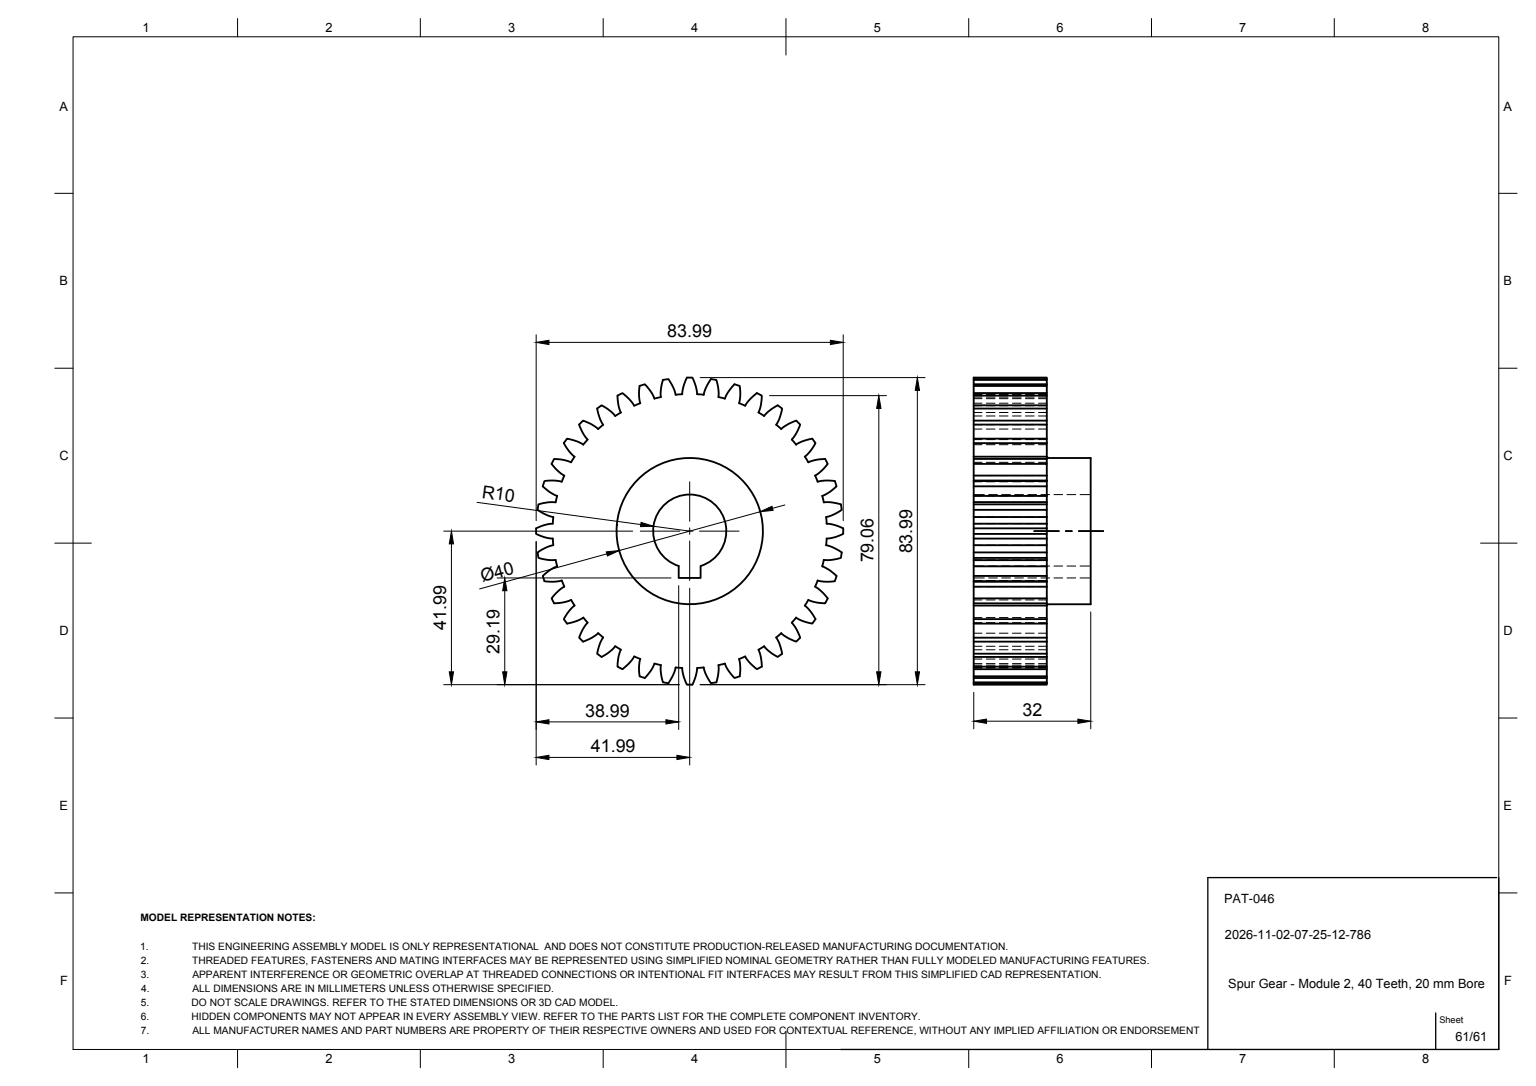
ISO-10303-21;
HEADER;
/* Generated by software containing ST-Developer
 * from STEP Tools, Inc. (www.steptools.com) 
 */

FILE_DESCRIPTION(
/* description */ ('Gear mesh backlash fixture'),
/* implementation_level */ '2;1');

FILE_NAME(
/* name */ 'Spur Gear - Module 2, 40 Teeth, 20 mm Bore.step',
/* time_stamp */ '2026-10-28T03:26:00-07:00',
/* author */ (''),
/* organization */ (''),
/* preprocessor_version */ 'ST-DEVELOPER v20.2',
/* originating_system */ 'Autodesk Translation Framework v15.17.0.0',
/* authorisation */ '');

FILE_SCHEMA (('AUTOMOTIVE_DESIGN { 1 0 10303 214 3 1 1 }'));
ENDSEC;

DATA;
#10=MECHANICAL_DESIGN_GEOMETRIC_PRESENTATION_REPRESENTATION('',(#1079),#57900);
#51=(
BOUNDED_SURFACE()
B_SPLINE_SURFACE(5,1,((#39961,#39962),(#39963,#39964),(#39965,#39966),(#39967,
#39968),(#39969,#39970),(#39971,#39972),(#39973,#39974),(#39975,#39976),
(#39977,#39978),(#39979,#39980),(#39981,#39982),(#39983,#39984),(#39985,
#39986),(#39987,#39988),(#39989,#39990),(#39991,#39992),(#39993,#39994),
(#39995,#39996),(#39997,#39998),(#39999,#40000),(#40001,#40002),(#40003,
#40004),(#40005,#40006),(#40007,#40008),(#40009,#40010),(#40011,#40012),
(#40013,#40014),(#40015,#40016),(#40017,#40018),(#40019,#40020),(#40021,
#40022),(#40023,#40024),(#40025,#40026),(#40027,#40028),(#40029,#40030),
(#40031,#40032),(#40033,#40034),(#40035,#40036),(#40037,#40038),(#40039,
#40040),(#40041,#40042),(#40043,#40044),(#40045,#40046),(#40047,#40048),
(#40049,#40050),(#40051,#40052),(#40053,#40054),(#40055,#40056),(#40057,
#40058),(#40059,#40060),(#40061,#40062),(#40063,#40064),(#40065,#40066),
(#40067,#40068),(#40069,#40070),(#40071,#40072),(#40073,#40074),(#40075,
#40076),(#40077,#40078),(#40079,#40080),(#40081,#40082),(#40083,#40084),
(#40085,#40086),(#40087,#40088),(#40089,#40090),(#40091,#40092),(#40093,
#40094),(#40095,#40096),(#40097,#40098),(#40099,#40100)),.UNSPECIFIED.,
 .F.,.F.,.F.)
B_SPLINE_SURFACE_WITH_KNOTS((6,1,1,1,1,1,1,1,1,1,1,1,1,1,1,1,1,1,1,1,1,
1,1,1,1,1,1,1,1,1,1,1,1,1,1,1,1,1,1,1,1,1,1,1,1,1,1,1,1,1,1,1,1,1,1,1,1,
1,1,1,1,1,1,1,1,6),(2,2),(-1.,-0.984615384615383,-0.969230769230768,-0.953846153846152,
-0.938461538461537,-0.923076923076922,-0.907692307692306,-0.892307692307691,
-0.876923076923076,-0.86153846153846,-0.846153846153845,-0.83076923076923,
-0.815384615384614,-0.799999999999999,-0.784615384615384,-0.769230769230768,
-0.753846153846153,-0.738461538461538,-0.723076923076922,-0.707692307692307,
-0.692307692307692,-0.676923076923076,-0.661538461538461,-0.646153846153846,
-0.63076923076923,-0.615384615384615,-0.6,-0.584615384615384,-0.569230769230769,
-0.553846153846154,-0.538461538461538,-0.523076923076923,-0.507692307692308,
-0.492307692307692,-0.476923076923077,-0.461538461538462,-0.446153846153846,
-0.430769230769231,-0.415384615384615,-0.4,-0.384615384615385,-0.369230769230769,
-0.353846153846154,-0.338461538461538,-0.323076923076923,-0.307692307692308,
-0.292307692307692,-0.276923076923077,-0.261538461538462,-0.246153846153846,
-0.230769230769231,-0.215384615384615,-0.2,-0.184615384615385,-0.169230769230769,
-0.153846153846154,-0.138461538461538,-0.123076923076923,-0.107692307692308,
-0.0923076923076923,-0.0769230769230769,-0.0615384615384615,-0.0461538461538462,
-0.0307692307692308,-0.0153846153846154,0.),(-1.,1.),.UNSPECIFIED.)
GEOMETRIC_REPRESENTATION_ITEM()
RATIONAL_B_SPLINE_SURFACE(((1.,1.),(1.,1.),(1.,1.),(1.,1.),(1.,1.),(1.,
1.),(1.,1.),(1.,1.),(1.,1.),(1.,1.),(1.,1.),(1.,1.),(1.,1.),(1.,1.),(1.,
1.),(1.,1.),(1.,1.),(1.,1.),(1.,1.),(1.,1.),(1.,1.),(1.,1.),(1.,1.),(1.,
1.),(1.,1.),(1.,1.),(1.,1.),(1.,1.),(1.,1.),(1.,1.),(1.,1.),(1.,1.),(1.,
1.),(1.,1.),(1.,1.),(1.,1.),(1.,1.),(1.,1.),(1.,1.),(1.,1.),(1.,1.),(1.,
1.),(1.,1.),(1.,1.),(1.,1.),(1.,1.),(1.,1.),(1.,1.),(1.,1.),(1.,1.),(1.,
1.),(1.,1.),(1.,1.),(1.,1.),(1.,1.),(1.,1.),(1.,1.),(1.,1.),(1.,1.),(1.,
1.),(1.,1.),(1.,1.),(1.,1.),(1.,1.),(1.,1.),(1.,1.),(1.,1.),(1.,1.),(1.,
1.),(1.,1.)))
REPRESENTATION_ITEM('')
SURFACE()
);
#52=(
BOUNDED_SURFACE()
B_SPLINE_SURFACE(5,1,((#40180,#40181),(#40182,#40183),(#40184,#40185),(#40186,
#40187),(#40188,#40189),(#40190,#40191),(#40192,#40193),(#40194,#40195),
(#40196,#40197),(#40198,#40199),(#40200,#40201),(#40202,#40203),(#40204,
#40205),(#40206,#40207),(#40208,#40209),(#40210,#40211),(#40212,#40213),
(#40214,#40215),(#40216,#40217),(#40218,#40219),(#40220,#40221),(#40222,
#40223),(#40224,#40225),(#40226,#40227),(#40228,#40229),(#40230,#40231),
(#40232,#40233),(#40234,#40235),(#40236,#40237),(#40238,#40239),(#40240,
#40241),(#40242,#40243),(#40244,#40245),(#40246,#40247),(#40248,#40249),
(#40250,#40251),(#40252,#40253),(#40254,#40255),(#40256,#40257),(#40258,
#40259),(#40260,#40261),(#40262,#40263),(#40264,#40265),(#40266,#40267),
(#40268,#40269),(#40270,#40271),(#40272,#40273),(#40274,#40275),(#40276,
#40277),(#40278,#40279),(#40280,#40281),(#40282,#40283),(#40284,#40285),
(#40286,#40287),(#40288,#40289),(#40290,#40291),(#40292,#40293),(#40294,
#40295),(#40296,#40297),(#40298,#40299),(#40300,#40301),(#40302,#40303),
(#40304,#40305),(#40306,#40307),(#40308,#40309),(#40310,#40311),(#40312,
#40313),(#40314,#40315),(#40316,#40317),(#40318,#40319)),.UNSPECIFIED.,
 .F.,.F.,.F.)
B_SPLINE_SURFACE_WITH_KNOTS((6,1,1,1,1,1,1,1,1,1,1,1,1,1,1,1,1,1,1,1,1,
1,1,1,1,1,1,1,1,1,1,1,1,1,1,1,1,1,1,1,1,1,1,1,1,1,1,1,1,1,1,1,1,1,1,1,1,
1,1,1,1,1,1,1,1,6),(2,2),(-1.,-0.984615384615383,-0.969230769230768,-0.953846153846152,
-0.938461538461537,-0.923076923076922,-0.907692307692306,-0.892307692307691,
-0.876923076923076,-0.86153846153846,-0.846153846153845,-0.83076923076923,
-0.815384615384614,-0.799999999999999,-0.784615384615384,-0.769230769230768,
-0.753846153846153,-0.738461538461538,-0.723076923076922,-0.707692307692307,
-0.692307692307692,-0.676923076923076,-0.661538461538461,-0.646153846153846,
-0.63076923076923,-0.615384615384615,-0.6,-0.584615384615384,-0.569230769230769,
-0.553846153846154,-0.538461538461538,-0.523076923076923,-0.507692307692308,
-0.492307692307692,-0.476923076923077,-0.461538461538462,-0.446153846153846,
-0.430769230769231,-0.415384615384615,-0.4,-0.384615384615385,-0.369230769230769,
-0.353846153846154,-0.338461538461538,-0.323076923076923,-0.307692307692308,
-0.292307692307692,-0.276923076923077,-0.261538461538462,-0.246153846153846,
-0.230769230769231,-0.215384615384615,-0.2,-0.184615384615385,-0.169230769230769,
-0.153846153846154,-0.138461538461538,-0.123076923076923,-0.107692307692308,
-0.0923076923076923,-0.0769230769230769,-0.0615384615384615,-0.0461538461538462,
-0.0307692307692308,-0.0153846153846154,0.),(-1.,1.),.UNSPECIFIED.)
GEOMETRIC_REPRESENTATION_ITEM()
RATIONAL_B_SPLINE_SURFACE(((1.,1.),(1.,1.),(1.,1.),(1.,1.),(1.,1.),(1.,
1.),(1.,1.),(1.,1.),(1.,1.),(1.,1.),(1.,1.),(1.,1.),(1.,1.),(1.,1.),(1.,
1.),(1.,1.),(1.,1.),(1.,1.),(1.,1.),(1.,1.),(1.,1.),(1.,1.),(1.,1.),(1.,
1.),(1.,1.),(1.,1.),(1.,1.),(1.,1.),(1.,1.),(1.,1.),(1.,1.),(1.,1.),(1.,
1.),(1.,1.),(1.,1.),(1.,1.),(1.,1.),(1.,1.),(1.,1.),(1.,1.),(1.,1.),(1.,
1.),(1.,1.),(1.,1.),(1.,1.),(1.,1.),(1.,1.),(1.,1.),(1.,1.),(1.,1.),(1.,
1.),(1.,1.),(1.,1.),(1.,1.),(1.,1.),(1.,1.),(1.,1.),(1.,1.),(1.,1.),(1.,
1.),(1.,1.),(1.,1.),(1.,1.),(1.,1.),(1.,1.),(1.,1.),(1.,1.),(1.,1.),(1.,
1.),(1.,1.)))
REPRESENTATION_ITEM('')
SURFACE()
);
#53=(
BOUNDED_SURFACE()
B_SPLINE_SURFACE(5,1,((#40410,#40411),(#40412,#40413),(#40414,#40415),(#40416,
#40417),(#40418,#40419),(#40420,#40421),(#40422,#40423),(#40424,#40425),
(#40426,#40427),(#40428,#40429),(#40430,#40431),(#40432,#40433),(#40434,
#40435),(#40436,#40437),(#40438,#40439),(#40440,#40441),(#40442,#40443),
(#40444,#40445),(#40446,#40447),(#40448,#40449),(#40450,#40451),(#40452,
#40453),(#40454,#40455),(#40456,#40457),(#40458,#40459),(#40460,#40461),
(#40462,#40463),(#40464,#40465),(#40466,#40467),(#40468,#40469),(#40470,
#40471),(#40472,#40473),(#40474,#40475),(#40476,#40477),(#40478,#40479),
(#40480,#40481),(#40482,#40483),(#40484,#40485),(#40486,#40487),(#40488,
#40489),(#40490,#40491),(#40492,#40493),(#40494,#40495),(#40496,#40497),
(#40498,#40499),(#40500,#40501),(#40502,#40503),(#40504,#40505),(#40506,
#40507),(#40508,#40509),(#40510,#40511),(#40512,#40513),(#40514,#40515),
(#40516,#40517),(#40518,#40519),(#40520,#40521),(#40522,#40523),(#40524,
#40525),(#40526,#40527),(#40528,#40529),(#40530,#40531),(#40532,#40533),
(#40534,#40535),(#40536,#40537),(#40538,#40539),(#40540,#40541),(#40542,
#40543),(#40544,#40545),(#40546,#40547),(#40548,#40549)),.UNSPECIFIED.,
 .F.,.F.,.F.)
B_SPLINE_SURFACE_WITH_KNOTS((6,1,1,1,1,1,1,1,1,1,1,1,1,1,1,1,1,1,1,1,1,
1,1,1,1,1,1,1,1,1,1,1,1,1,1,1,1,1,1,1,1,1,1,1,1,1,1,1,1,1,1,1,1,1,1,1,1,
1,1,1,1,1,1,1,1,6),(2,2),(-1.,-0.984615384615383,-0.969230769230768,-0.953846153846152,
-0.938461538461537,-0.923076923076922,-0.907692307692306,-0.892307692307691,
-0.876923076923076,-0.86153846153846,-0.846153846153845,-0.83076923076923,
-0.815384615384614,-0.799999999999999,-0.784615384615384,-0.769230769230768,
-0.753846153846153,-0.738461538461538,-0.723076923076922,-0.707692307692307,
-0.692307692307692,-0.676923076923076,-0.661538461538461,-0.646153846153846,
-0.63076923076923,-0.615384615384615,-0.6,-0.584615384615384,-0.569230769230769,
-0.553846153846154,-0.538461538461538,-0.523076923076923,-0.507692307692308,
-0.492307692307692,-0.476923076923077,-0.461538461538462,-0.446153846153846,
-0.430769230769231,-0.415384615384615,-0.4,-0.384615384615385,-0.369230769230769,
-0.353846153846154,-0.338461538461538,-0.323076923076923,-0.307692307692308,
-0.292307692307692,-0.276923076923077,-0.261538461538462,-0.246153846153846,
-0.230769230769231,-0.215384615384615,-0.2,-0.184615384615385,-0.169230769230769,
-0.153846153846154,-0.138461538461538,-0.123076923076923,-0.107692307692308,
-0.0923076923076923,-0.0769230769230769,-0.0615384615384615,-0.0461538461538462,
-0.0307692307692308,-0.0153846153846154,0.),(-1.,1.),.UNSPECIFIED.)
GEOMETRIC_REPRESENTATION_ITEM()
RATIONAL_B_SPLINE_SURFACE(((1.,1.),(1.,1.),(1.,1.),(1.,1.),(1.,1.),(1.,
1.),(1.,1.),(1.,1.),(1.,1.),(1.,1.),(1.,1.),(1.,1.),(1.,1.),(1.,1.),(1.,
1.),(1.,1.),(1.,1.),(1.,1.),(1.,1.),(1.,1.),(1.,1.),(1.,1.),(1.,1.),(1.,
1.),(1.,1.),(1.,1.),(1.,1.),(1.,1.),(1.,1.),(1.,1.),(1.,1.),(1.,1.),(1.,
1.),(1.,1.),(1.,1.),(1.,1.),(1.,1.),(1.,1.),(1.,1.),(1.,1.),(1.,1.),(1.,
1.),(1.,1.),(1.,1.),(1.,1.),(1.,1.),(1.,1.),(1.,1.),(1.,1.),(1.,1.),(1.,
1.),(1.,1.),(1.,1.),(1.,1.),(1.,1.),(1.,1.),(1.,1.),(1.,1.),(1.,1.),(1.,
1.),(1.,1.),(1.,1.),(1.,1.),(1.,1.),(1.,1.),(1.,1.),(1.,1.),(1.,1.),(1.,
1.),(1.,1.)))
REPRESENTATION_ITEM('')
SURFACE()
);
#54=(
BOUNDED_SURFACE()
B_SPLINE_SURFACE(5,1,((#40622,#40623),(#40624,#40625),(#40626,#40627),(#40628,
#40629),(#40630,#40631),(#40632,#40633),(#40634,#40635),(#40636,#40637),
(#40638,#40639),(#40640,#40641),(#40642,#40643),(#40644,#40645),(#40646,
#40647),(#40648,#40649),(#40650,#40651),(#40652,#40653),(#40654,#40655),
(#40656,#40657),(#40658,#40659),(#40660,#40661),(#40662,#40663),(#40664,
#40665),(#40666,#40667),(#40668,#40669),(#40670,#40671),(#40672,#40673),
(#40674,#40675),(#40676,#40677),(#40678,#40679),(#40680,#40681),(#40682,
#40683),(#40684,#40685),(#40686,#40687),(#40688,#40689),(#40690,#40691),
(#40692,#40693),(#40694,#40695),(#40696,#40697),(#40698,#40699),(#40700,
#40701),(#40702,#40703),(#40704,#40705),(#40706,#40707),(#40708,#40709),
(#40710,#40711),(#40712,#40713),(#40714,#40715),(#40716,#40717),(#40718,
#40719),(#40720,#40721),(#40722,#40723),(#40724,#40725),(#40726,#40727),
(#40728,#40729),(#40730,#40731),(#40732,#40733),(#40734,#40735),(#40736,
#40737),(#40738,#40739),(#40740,#40741),(#40742,#40743),(#40744,#40745),
(#40746,#40747),(#40748,#40749),(#40750,#40751),(#40752,#40753),(#40754,
#40755),(#40756,#40757),(#40758,#40759),(#40760,#40761)),.UNSPECIFIED.,
 .F.,.F.,.F.)
B_SPLINE_SURFACE_WITH_KNOTS((6,1,1,1,1,1,1,1,1,1,1,1,1,1,1,1,1,1,1,1,1,
1,1,1,1,1,1,1,1,1,1,1,1,1,1,1,1,1,1,1,1,1,1,1,1,1,1,1,1,1,1,1,1,1,1,1,1,
1,1,1,1,1,1,1,1,6),(2,2),(-1.,-0.984615384615383,-0.969230769230768,-0.953846153846152,
-0.938461538461537,-0.923076923076922,-0.907692307692306,-0.892307692307691,
-0.876923076923076,-0.86153846153846,-0.846153846153845,-0.83076923076923,
-0.815384615384614,-0.799999999999999,-0.784615384615384,-0.769230769230768,
-0.753846153846153,-0.738461538461538,-0.723076923076922,-0.707692307692307,
-0.692307692307692,-0.676923076923076,-0.661538461538461,-0.646153846153846,
-0.63076923076923,-0.615384615384615,-0.6,-0.584615384615384,-0.569230769230769,
-0.553846153846154,-0.538461538461538,-0.523076923076923,-0.507692307692308,
-0.492307692307692,-0.476923076923077,-0.461538461538462,-0.446153846153846,
-0.430769230769231,-0.415384615384615,-0.4,-0.384615384615385,-0.369230769230769,
-0.353846153846154,-0.338461538461538,-0.323076923076923,-0.307692307692308,
-0.292307692307692,-0.276923076923077,-0.261538461538462,-0.246153846153846,
-0.230769230769231,-0.215384615384615,-0.2,-0.184615384615385,-0.169230769230769,
-0.153846153846154,-0.138461538461538,-0.123076923076923,-0.107692307692308,
-0.0923076923076923,-0.0769230769230769,-0.0615384615384615,-0.0461538461538462,
-0.0307692307692308,-0.0153846153846154,0.),(-1.,1.),.UNSPECIFIED.)
GEOMETRIC_REPRESENTATION_ITEM()
RATIONAL_B_SPLINE_SURFACE(((1.,1.),(1.,1.),(1.,1.),(1.,1.),(1.,1.),(1.,
1.),(1.,1.),(1.,1.),(1.,1.),(1.,1.),(1.,1.),(1.,1.),(1.,1.),(1.,1.),(1.,
1.),(1.,1.),(1.,1.),(1.,1.),(1.,1.),(1.,1.),(1.,1.),(1.,1.),(1.,1.),(1.,
1.),(1.,1.),(1.,1.),(1.,1.),(1.,1.),(1.,1.),(1.,1.),(1.,1.),(1.,1.),(1.,
1.),(1.,1.),(1.,1.),(1.,1.),(1.,1.),(1.,1.),(1.,1.),(1.,1.),(1.,1.),(1.,
1.),(1.,1.),(1.,1.),(1.,1.),(1.,1.),(1.,1.),(1.,1.),(1.,1.),(1.,1.),(1.,
1.),(1.,1.),(1.,1.),(1.,1.),(1.,1.),(1.,1.),(1.,1.),(1.,1.),(1.,1.),(1.,
1.),(1.,1.),(1.,1.),(1.,1.),(1.,1.),(1.,1.),(1.,1.),(1.,1.),(1.,1.),(1.,
1.),(1.,1.)))
REPRESENTATION_ITEM('')
SURFACE()
);
#55=(
BOUNDED_SURFACE()
B_SPLINE_SURFACE(5,1,((#40852,#40853),(#40854,#40855),(#40856,#40857),(#40858,
#40859),(#40860,#40861),(#40862,#40863),(#40864,#40865),(#40866,#40867),
(#40868,#40869),(#40870,#40871),(#40872,#40873),(#40874,#40875),(#40876,
#40877),(#40878,#40879),(#40880,#40881),(#40882,#40883),(#40884,#40885),
(#40886,#40887),(#40888,#40889),(#40890,#40891),(#40892,#40893),(#40894,
#40895),(#40896,#40897),(#40898,#40899),(#40900,#40901),(#40902,#40903),
(#40904,#40905),(#40906,#40907),(#40908,#40909),(#40910,#40911),(#40912,
#40913),(#40914,#40915),(#40916,#40917),(#40918,#40919),(#40920,#40921),
(#40922,#40923),(#40924,#40925),(#40926,#40927),(#40928,#40929),(#40930,
#40931),(#40932,#40933),(#40934,#40935),(#40936,#40937),(#40938,#40939),
(#40940,#40941),(#40942,#40943),(#40944,#40945),(#40946,#40947),(#40948,
#40949),(#40950,#40951),(#40952,#40953),(#40954,#40955),(#40956,#40957),
(#40958,#40959),(#40960,#40961),(#40962,#40963),(#40964,#40965),(#40966,
#40967),(#40968,#40969),(#40970,#40971),(#40972,#40973),(#40974,#40975),
(#40976,#40977),(#40978,#40979),(#40980,#40981),(#40982,#40983),(#40984,
#40985),(#40986,#40987),(#40988,#40989),(#40990,#40991)),.UNSPECIFIED.,
 .F.,.F.,.F.)
B_SPLINE_SURFACE_WITH_KNOTS((6,1,1,1,1,1,1,1,1,1,1,1,1,1,1,1,1,1,1,1,1,
1,1,1,1,1,1,1,1,1,1,1,1,1,1,1,1,1,1,1,1,1,1,1,1,1,1,1,1,1,1,1,1,1,1,1,1,
1,1,1,1,1,1,1,1,6),(2,2),(-1.,-0.984615384615383,-0.969230769230768,-0.953846153846152,
-0.938461538461537,-0.923076923076922,-0.907692307692306,-0.892307692307691,
-0.876923076923076,-0.86153846153846,-0.846153846153845,-0.83076923076923,
-0.815384615384614,-0.799999999999999,-0.784615384615384,-0.769230769230768,
-0.753846153846153,-0.738461538461538,-0.723076923076922,-0.707692307692307,
-0.692307692307692,-0.676923076923076,-0.661538461538461,-0.646153846153846,
-0.63076923076923,-0.615384615384615,-0.6,-0.584615384615384,-0.569230769230769,
-0.553846153846154,-0.538461538461538,-0.523076923076923,-0.507692307692308,
-0.492307692307692,-0.476923076923077,-0.461538461538462,-0.446153846153846,
-0.430769230769231,-0.415384615384615,-0.4,-0.384615384615385,-0.369230769230769,
-0.353846153846154,-0.338461538461538,-0.323076923076923,-0.307692307692308,
-0.292307692307692,-0.276923076923077,-0.261538461538462,-0.246153846153846,
-0.230769230769231,-0.215384615384615,-0.2,-0.184615384615385,-0.169230769230769,
-0.153846153846154,-0.138461538461538,-0.123076923076923,-0.107692307692308,
-0.0923076923076923,-0.0769230769230769,-0.0615384615384615,-0.0461538461538462,
-0.0307692307692308,-0.0153846153846154,0.),(-1.,1.),.UNSPECIFIED.)
GEOMETRIC_REPRESENTATION_ITEM()
RATIONAL_B_SPLINE_SURFACE(((1.,1.),(1.,1.),(1.,1.),(1.,1.),(1.,1.),(1.,
1.),(1.,1.),(1.,1.),(1.,1.),(1.,1.),(1.,1.),(1.,1.),(1.,1.),(1.,1.),(1.,
1.),(1.,1.),(1.,1.),(1.,1.),(1.,1.),(1.,1.),(1.,1.),(1.,1.),(1.,1.),(1.,
1.),(1.,1.),(1.,1.),(1.,1.),(1.,1.),(1.,1.),(1.,1.),(1.,1.),(1.,1.),(1.,
1.),(1.,1.),(1.,1.),(1.,1.),(1.,1.),(1.,1.),(1.,1.),(1.,1.),(1.,1.),(1.,
1.),(1.,1.),(1.,1.),(1.,1.),(1.,1.),(1.,1.),(1.,1.),(1.,1.),(1.,1.),(1.,
1.),(1.,1.),(1.,1.),(1.,1.),(1.,1.),(1.,1.),(1.,1.),(1.,1.),(1.,1.),(1.,
1.),(1.,1.),(1.,1.),(1.,1.),(1.,1.),(1.,1.),(1.,1.),(1.,1.),(1.,1.),(1.,
1.),(1.,1.)))
REPRESENTATION_ITEM('')
SURFACE()
);
#56=(
BOUNDED_SURFACE()
B_SPLINE_SURFACE(5,1,((#41064,#41065),(#41066,#41067),(#41068,#41069),(#41070,
#41071),(#41072,#41073),(#41074,#41075),(#41076,#41077),(#41078,#41079),
(#41080,#41081),(#41082,#41083),(#41084,#41085),(#41086,#41087),(#41088,
#41089),(#41090,#41091),(#41092,#41093),(#41094,#41095),(#41096,#41097),
(#41098,#41099),(#41100,#41101),(#41102,#41103),(#41104,#41105),(#41106,
#41107),(#41108,#41109),(#41110,#41111),(#41112,#41113),(#41114,#41115),
(#41116,#41117),(#41118,#41119),(#41120,#41121),(#41122,#41123),(#41124,
#41125),(#41126,#41127),(#41128,#41129),(#41130,#41131),(#41132,#41133),
(#41134,#41135),(#41136,#41137),(#41138,#41139),(#41140,#41141),(#41142,
#41143),(#41144,#41145),(#41146,#41147),(#41148,#41149),(#41150,#41151),
(#41152,#41153),(#41154,#41155),(#41156,#41157),(#41158,#41159),(#41160,
#41161),(#41162,#41163),(#41164,#41165),(#41166,#41167),(#41168,#41169),
(#41170,#41171),(#41172,#41173),(#41174,#41175),(#41176,#41177),(#41178,
#41179),(#41180,#41181),(#41182,#41183),(#41184,#41185),(#41186,#41187),
(#41188,#41189),(#41190,#41191),(#41192,#41193),(#41194,#41195),(#41196,
#41197),(#41198,#41199),(#41200,#41201),(#41202,#41203)),.UNSPECIFIED.,
 .F.,.F.,.F.)
B_SPLINE_SURFACE_WITH_KNOTS((6,1,1,1,1,1,1,1,1,1,1,1,1,1,1,1,1,1,1,1,1,
1,1,1,1,1,1,1,1,1,1,1,1,1,1,1,1,1,1,1,1,1,1,1,1,1,1,1,1,1,1,1,1,1,1,1,1,
1,1,1,1,1,1,1,1,6),(2,2),(-1.,-0.984615384615383,-0.969230769230768,-0.953846153846152,
-0.938461538461537,-0.923076923076922,-0.907692307692306,-0.892307692307691,
-0.876923076923076,-0.86153846153846,-0.846153846153845,-0.83076923076923,
-0.815384615384614,-0.799999999999999,-0.784615384615384,-0.769230769230768,
-0.753846153846153,-0.738461538461538,-0.723076923076922,-0.707692307692307,
-0.692307692307692,-0.676923076923076,-0.661538461538461,-0.646153846153846,
-0.63076923076923,-0.615384615384615,-0.6,-0.584615384615384,-0.569230769230769,
-0.553846153846154,-0.538461538461538,-0.523076923076923,-0.507692307692308,
-0.492307692307692,-0.476923076923077,-0.461538461538462,-0.446153846153846,
-0.430769230769231,-0.415384615384615,-0.4,-0.384615384615385,-0.369230769230769,
-0.353846153846154,-0.338461538461538,-0.323076923076923,-0.307692307692308,
-0.292307692307692,-0.276923076923077,-0.261538461538462,-0.246153846153846,
-0.230769230769231,-0.215384615384615,-0.2,-0.184615384615385,-0.169230769230769,
-0.153846153846154,-0.138461538461538,-0.123076923076923,-0.107692307692308,
-0.0923076923076923,-0.0769230769230769,-0.0615384615384615,-0.0461538461538462,
-0.0307692307692308,-0.0153846153846154,0.),(-1.,1.),.UNSPECIFIED.)
GEOMETRIC_REPRESENTATION_ITEM()
RATIONAL_B_SPLINE_SURFACE(((1.,1.),(1.,1.),(1.,1.),(1.,1.),(1.,1.),(1.,
1.),(1.,1.),(1.,1.),(1.,1.),(1.,1.),(1.,1.),(1.,1.),(1.,1.),(1.,1.),(1.,
1.),(1.,1.),(1.,1.),(1.,1.),(1.,1.),(1.,1.),(1.,1.),(1.,1.),(1.,1.),(1.,
1.),(1.,1.),(1.,1.),(1.,1.),(1.,1.),(1.,1.),(1.,1.),(1.,1.),(1.,1.),(1.,
1.),(1.,1.),(1.,1.),(1.,1.),(1.,1.),(1.,1.),(1.,1.),(1.,1.),(1.,1.),(1.,
1.),(1.,1.),(1.,1.),(1.,1.),(1.,1.),(1.,1.),(1.,1.),(1.,1.),(1.,1.),(1.,
1.),(1.,1.),(1.,1.),(1.,1.),(1.,1.),(1.,1.),(1.,1.),(1.,1.),(1.,1.),(1.,
1.),(1.,1.),(1.,1.),(1.,1.),(1.,1.),(1.,1.),(1.,1.),(1.,1.),(1.,1.),(1.,
1.),(1.,1.)))
REPRESENTATION_ITEM('')
SURFACE()
);
#57=(
BOUNDED_SURFACE()
B_SPLINE_SURFACE(5,1,((#41294,#41295),(#41296,#41297),(#41298,#41299),(#41300,
#41301),(#41302,#41303),(#41304,#41305),(#41306,#41307),(#41308,#41309),
(#41310,#41311),(#41312,#41313),(#41314,#41315),(#41316,#41317),(#41318,
#41319),(#41320,#41321),(#41322,#41323),(#41324,#41325),(#41326,#41327),
(#41328,#41329),(#41330,#41331),(#41332,#41333),(#41334,#41335),(#41336,
#41337),(#41338,#41339),(#41340,#41341),(#41342,#41343),(#41344,#41345),
(#41346,#41347),(#41348,#41349),(#41350,#41351),(#41352,#41353),(#41354,
#41355),(#41356,#41357),(#41358,#41359),(#41360,#41361),(#41362,#41363),
(#41364,#41365),(#41366,#41367),(#41368,#41369),(#41370,#41371),(#41372,
#41373),(#41374,#41375),(#41376,#41377),(#41378,#41379),(#41380,#41381),
(#41382,#41383),(#41384,#41385),(#41386,#41387),(#41388,#41389),(#41390,
#41391),(#41392,#41393),(#41394,#41395),(#41396,#41397),(#41398,#41399),
(#41400,#41401),(#41402,#41403),(#41404,#41405),(#41406,#41407),(#41408,
#41409),(#41410,#41411),(#41412,#41413),(#41414,#41415),(#41416,#41417),
(#41418,#41419),(#41420,#41421),(#41422,#41423),(#41424,#41425),(#41426,
#41427),(#41428,#41429),(#41430,#41431),(#41432,#41433)),.UNSPECIFIED.,
 .F.,.F.,.F.)
B_SPLINE_SURFACE_WITH_KNOTS((6,1,1,1,1,1,1,1,1,1,1,1,1,1,1,1,1,1,1,1,1,
1,1,1,1,1,1,1,1,1,1,1,1,1,1,1,1,1,1,1,1,1,1,1,1,1,1,1,1,1,1,1,1,1,1,1,1,
1,1,1,1,1,1,1,1,6),(2,2),(-1.,-0.984615384615383,-0.969230769230768,-0.953846153846152,
-0.938461538461537,-0.923076923076922,-0.907692307692306,-0.892307692307691,
-0.876923076923076,-0.86153846153846,-0.846153846153845,-0.83076923076923,
-0.815384615384614,-0.799999999999999,-0.784615384615384,-0.769230769230768,
-0.753846153846153,-0.738461538461538,-0.723076923076922,-0.707692307692307,
-0.692307692307692,-0.676923076923076,-0.661538461538461,-0.646153846153846,
-0.63076923076923,-0.615384615384615,-0.6,-0.584615384615384,-0.569230769230769,
-0.553846153846154,-0.538461538461538,-0.523076923076923,-0.507692307692308,
-0.492307692307692,-0.476923076923077,-0.461538461538462,-0.446153846153846,
-0.430769230769231,-0.415384615384615,-0.4,-0.384615384615385,-0.369230769230769,
-0.353846153846154,-0.338461538461538,-0.323076923076923,-0.307692307692308,
-0.292307692307692,-0.276923076923077,-0.261538461538462,-0.246153846153846,
-0.230769230769231,-0.215384615384615,-0.2,-0.184615384615385,-0.169230769230769,
-0.153846153846154,-0.138461538461538,-0.123076923076923,-0.107692307692308,
-0.0923076923076923,-0.0769230769230769,-0.0615384615384615,-0.0461538461538462,
-0.0307692307692308,-0.0153846153846154,0.),(-1.,1.),.UNSPECIFIED.)
GEOMETRIC_REPRESENTATION_ITEM()
RATIONAL_B_SPLINE_SURFACE(((1.,1.),(1.,1.),(1.,1.),(1.,1.),(1.,1.),(1.,
1.),(1.,1.),(1.,1.),(1.,1.),(1.,1.),(1.,1.),(1.,1.),(1.,1.),(1.,1.),(1.,
1.),(1.,1.),(1.,1.),(1.,1.),(1.,1.),(1.,1.),(1.,1.),(1.,1.),(1.,1.),(1.,
1.),(1.,1.),(1.,1.),(1.,1.),(1.,1.),(1.,1.),(1.,1.),(1.,1.),(1.,1.),(1.,
1.),(1.,1.),(1.,1.),(1.,1.),(1.,1.),(1.,1.),(1.,1.),(1.,1.),(1.,1.),(1.,
1.),(1.,1.),(1.,1.),(1.,1.),(1.,1.),(1.,1.),(1.,1.),(1.,1.),(1.,1.),(1.,
1.),(1.,1.),(1.,1.),(1.,1.),(1.,1.),(1.,1.),(1.,1.),(1.,1.),(1.,1.),(1.,
1.),(1.,1.),(1.,1.),(1.,1.),(1.,1.),(1.,1.),(1.,1.),(1.,1.),(1.,1.),(1.,
1.),(1.,1.)))
REPRESENTATION_ITEM('')
SURFACE()
);
#58=(
BOUNDED_SURFACE()
B_SPLINE_SURFACE(5,1,((#41506,#41507),(#41508,#41509),(#41510,#41511),(#41512,
#41513),(#41514,#41515),(#41516,#41517),(#41518,#41519),(#41520,#41521),
(#41522,#41523),(#41524,#41525),(#41526,#41527),(#41528,#41529),(#41530,
#41531),(#41532,#41533),(#41534,#41535),(#41536,#41537),(#41538,#41539),
(#41540,#41541),(#41542,#41543),(#41544,#41545),(#41546,#41547),(#41548,
#41549),(#41550,#41551),(#41552,#41553),(#41554,#41555),(#41556,#41557),
(#41558,#41559),(#41560,#41561),(#41562,#41563),(#41564,#41565),(#41566,
#41567),(#41568,#41569),(#41570,#41571),(#41572,#41573),(#41574,#41575),
(#41576,#41577),(#41578,#41579),(#41580,#41581),(#41582,#41583),(#41584,
#41585),(#41586,#41587),(#41588,#41589),(#41590,#41591),(#41592,#41593),
(#41594,#41595),(#41596,#41597),(#41598,#41599),(#41600,#41601),(#41602,
#41603),(#41604,#41605),(#41606,#41607),(#41608,#41609),(#41610,#41611),
(#41612,#41613),(#41614,#41615),(#41616,#41617),(#41618,#41619),(#41620,
#41621),(#41622,#41623),(#41624,#41625),(#41626,#41627),(#41628,#41629),
(#41630,#41631),(#41632,#41633),(#41634,#41635),(#41636,#41637),(#41638,
#41639),(#41640,#41641),(#41642,#41643),(#41644,#41645)),.UNSPECIFIED.,
 .F.,.F.,.F.)
B_SPLINE_SURFACE_WITH_KNOTS((6,1,1,1,1,1,1,1,1,1,1,1,1,1,1,1,1,1,1,1,1,
1,1,1,1,1,1,1,1,1,1,1,1,1,1,1,1,1,1,1,1,1,1,1,1,1,1,1,1,1,1,1,1,1,1,1,1,
1,1,1,1,1,1,1,1,6),(2,2),(-1.,-0.984615384615383,-0.969230769230768,-0.953846153846152,
-0.938461538461537,-0.923076923076922,-0.907692307692306,-0.892307692307691,
-0.876923076923076,-0.86153846153846,-0.846153846153845,-0.83076923076923,
-0.815384615384614,-0.799999999999999,-0.784615384615384,-0.769230769230768,
-0.753846153846153,-0.738461538461538,-0.723076923076922,-0.707692307692307,
-0.692307692307692,-0.676923076923076,-0.661538461538461,-0.646153846153846,
-0.63076923076923,-0.615384615384615,-0.6,-0.584615384615384,-0.569230769230769,
-0.553846153846154,-0.538461538461538,-0.523076923076923,-0.507692307692308,
-0.492307692307692,-0.476923076923077,-0.461538461538462,-0.446153846153846,
-0.430769230769231,-0.415384615384615,-0.4,-0.384615384615385,-0.369230769230769,
-0.353846153846154,-0.338461538461538,-0.323076923076923,-0.307692307692308,
-0.292307692307692,-0.276923076923077,-0.261538461538462,-0.246153846153846,
-0.230769230769231,-0.215384615384615,-0.2,-0.184615384615385,-0.169230769230769,
-0.153846153846154,-0.138461538461538,-0.123076923076923,-0.107692307692308,
-0.0923076923076923,-0.0769230769230769,-0.0615384615384615,-0.0461538461538462,
-0.0307692307692308,-0.0153846153846154,0.),(-1.,1.),.UNSPECIFIED.)
GEOMETRIC_REPRESENTATION_ITEM()
RATIONAL_B_SPLINE_SURFACE(((1.,1.),(1.,1.),(1.,1.),(1.,1.),(1.,1.),(1.,
1.),(1.,1.),(1.,1.),(1.,1.),(1.,1.),(1.,1.),(1.,1.),(1.,1.),(1.,1.),(1.,
1.),(1.,1.),(1.,1.),(1.,1.),(1.,1.),(1.,1.),(1.,1.),(1.,1.),(1.,1.),(1.,
1.),(1.,1.),(1.,1.),(1.,1.),(1.,1.),(1.,1.),(1.,1.),(1.,1.),(1.,1.),(1.,
1.),(1.,1.),(1.,1.),(1.,1.),(1.,1.),(1.,1.),(1.,1.),(1.,1.),(1.,1.),(1.,
1.),(1.,1.),(1.,1.),(1.,1.),(1.,1.),(1.,1.),(1.,1.),(1.,1.),(1.,1.),(1.,
1.),(1.,1.),(1.,1.),(1.,1.),(1.,1.),(1.,1.),(1.,1.),(1.,1.),(1.,1.),(1.,
1.),(1.,1.),(1.,1.),(1.,1.),(1.,1.),(1.,1.),(1.,1.),(1.,1.),(1.,1.),(1.,
1.),(1.,1.)))
REPRESENTATION_ITEM('')
SURFACE()
);
#59=(
BOUNDED_SURFACE()
B_SPLINE_SURFACE(5,1,((#41736,#41737),(#41738,#41739),(#41740,#41741),(#41742,
#41743),(#41744,#41745),(#41746,#41747),(#41748,#41749),(#41750,#41751),
(#41752,#41753),(#41754,#41755),(#41756,#41757),(#41758,#41759),(#41760,
#41761),(#41762,#41763),(#41764,#41765),(#41766,#41767),(#41768,#41769),
(#41770,#41771),(#41772,#41773),(#41774,#41775),(#41776,#41777),(#41778,
#41779),(#41780,#41781),(#41782,#41783),(#41784,#41785),(#41786,#41787),
(#41788,#41789),(#41790,#41791),(#41792,#41793),(#41794,#41795),(#41796,
#41797),(#41798,#41799),(#41800,#41801),(#41802,#41803),(#41804,#41805),
(#41806,#41807),(#41808,#41809),(#41810,#41811),(#41812,#41813),(#41814,
#41815),(#41816,#41817),(#41818,#41819),(#41820,#41821),(#41822,#41823),
(#41824,#41825),(#41826,#41827),(#41828,#41829),(#41830,#41831),(#41832,
#41833),(#41834,#41835),(#41836,#41837),(#41838,#41839),(#41840,#41841),
(#41842,#41843),(#41844,#41845),(#41846,#41847),(#41848,#41849),(#41850,
#41851),(#41852,#41853),(#41854,#41855),(#41856,#41857),(#41858,#41859),
(#41860,#41861),(#41862,#41863),(#41864,#41865),(#41866,#41867),(#41868,
#41869),(#41870,#41871),(#41872,#41873),(#41874,#41875)),.UNSPECIFIED.,
 .F.,.F.,.F.)
B_SPLINE_SURFACE_WITH_KNOTS((6,1,1,1,1,1,1,1,1,1,1,1,1,1,1,1,1,1,1,1,1,
1,1,1,1,1,1,1,1,1,1,1,1,1,1,1,1,1,1,1,1,1,1,1,1,1,1,1,1,1,1,1,1,1,1,1,1,
1,1,1,1,1,1,1,1,6),(2,2),(-1.,-0.984615384615383,-0.969230769230768,-0.953846153846152,
-0.938461538461537,-0.923076923076922,-0.907692307692306,-0.892307692307691,
-0.876923076923076,-0.86153846153846,-0.846153846153845,-0.83076923076923,
-0.815384615384614,-0.799999999999999,-0.784615384615384,-0.769230769230768,
-0.753846153846153,-0.738461538461538,-0.723076923076922,-0.707692307692307,
-0.692307692307692,-0.676923076923076,-0.661538461538461,-0.646153846153846,
-0.63076923076923,-0.615384615384615,-0.6,-0.584615384615384,-0.569230769230769,
-0.553846153846154,-0.538461538461538,-0.523076923076923,-0.507692307692308,
-0.492307692307692,-0.476923076923077,-0.461538461538462,-0.446153846153846,
-0.430769230769231,-0.415384615384615,-0.4,-0.384615384615385,-0.369230769230769,
-0.353846153846154,-0.338461538461538,-0.323076923076923,-0.307692307692308,
-0.292307692307692,-0.276923076923077,-0.261538461538462,-0.246153846153846,
-0.230769230769231,-0.215384615384615,-0.2,-0.184615384615385,-0.169230769230769,
-0.153846153846154,-0.138461538461538,-0.123076923076923,-0.107692307692308,
-0.0923076923076923,-0.0769230769230769,-0.0615384615384615,-0.0461538461538462,
-0.0307692307692308,-0.0153846153846154,0.),(-1.,1.),.UNSPECIFIED.)
GEOMETRIC_REPRESENTATION_ITEM()
RATIONAL_B_SPLINE_SURFACE(((1.,1.),(1.,1.),(1.,1.),(1.,1.),(1.,1.),(1.,
1.),(1.,1.),(1.,1.),(1.,1.),(1.,1.),(1.,1.),(1.,1.),(1.,1.),(1.,1.),(1.,
1.),(1.,1.),(1.,1.),(1.,1.),(1.,1.),(1.,1.),(1.,1.),(1.,1.),(1.,1.),(1.,
1.),(1.,1.),(1.,1.),(1.,1.),(1.,1.),(1.,1.),(1.,1.),(1.,1.),(1.,1.),(1.,
1.),(1.,1.),(1.,1.),(1.,1.),(1.,1.),(1.,1.),(1.,1.),(1.,1.),(1.,1.),(1.,
1.),(1.,1.),(1.,1.),(1.,1.),(1.,1.),(1.,1.),(1.,1.),(1.,1.),(1.,1.),(1.,
1.),(1.,1.),(1.,1.),(1.,1.),(1.,1.),(1.,1.),(1.,1.),(1.,1.),(1.,1.),(1.,
1.),(1.,1.),(1.,1.),(1.,1.),(1.,1.),(1.,1.),(1.,1.),(1.,1.),(1.,1.),(1.,
1.),(1.,1.)))
REPRESENTATION_ITEM('')
SURFACE()
);
#60=(
BOUNDED_SURFACE()
B_SPLINE_SURFACE(5,1,((#41948,#41949),(#41950,#41951),(#41952,#41953),(#41954,
#41955),(#41956,#41957),(#41958,#41959),(#41960,#41961),(#41962,#41963),
(#41964,#41965),(#41966,#41967),(#41968,#41969),(#41970,#41971),(#41972,
#41973),(#41974,#41975),(#41976,#41977),(#41978,#41979),(#41980,#41981),
(#41982,#41983),(#41984,#41985),(#41986,#41987),(#41988,#41989),(#41990,
#41991),(#41992,#41993),(#41994,#41995),(#41996,#41997),(#41998,#41999),
(#42000,#42001),(#42002,#42003),(#42004,#42005),(#42006,#42007),(#42008,
#42009),(#42010,#42011),(#42012,#42013),(#42014,#42015),(#42016,#42017),
(#42018,#42019),(#42020,#42021),(#42022,#42023),(#42024,#42025),(#42026,
#42027),(#42028,#42029),(#42030,#42031),(#42032,#42033),(#42034,#42035),
(#42036,#42037),(#42038,#42039),(#42040,#42041),(#42042,#42043),(#42044,
#42045),(#42046,#42047),(#42048,#42049),(#42050,#42051),(#42052,#42053),
(#42054,#42055),(#42056,#42057),(#42058,#42059),(#42060,#42061),(#42062,
#42063),(#42064,#42065),(#42066,#42067),(#42068,#42069),(#42070,#42071),
(#42072,#42073),(#42074,#42075),(#42076,#42077),(#42078,#42079),(#42080,
#42081),(#42082,#42083),(#42084,#42085),(#42086,#42087)),.UNSPECIFIED.,
 .F.,.F.,.F.)
B_SPLINE_SURFACE_WITH_KNOTS((6,1,1,1,1,1,1,1,1,1,1,1,1,1,1,1,1,1,1,1,1,
1,1,1,1,1,1,1,1,1,1,1,1,1,1,1,1,1,1,1,1,1,1,1,1,1,1,1,1,1,1,1,1,1,1,1,1,
1,1,1,1,1,1,1,1,6),(2,2),(-1.,-0.984615384615383,-0.969230769230768,-0.953846153846152,
-0.938461538461537,-0.923076923076922,-0.907692307692306,-0.892307692307691,
-0.876923076923076,-0.86153846153846,-0.846153846153845,-0.83076923076923,
-0.815384615384614,-0.799999999999999,-0.784615384615384,-0.769230769230768,
-0.753846153846153,-0.738461538461538,-0.723076923076922,-0.707692307692307,
-0.692307692307692,-0.676923076923076,-0.661538461538461,-0.646153846153846,
-0.63076923076923,-0.615384615384615,-0.6,-0.584615384615384,-0.569230769230769,
-0.553846153846154,-0.538461538461538,-0.523076923076923,-0.507692307692308,
-0.492307692307692,-0.476923076923077,-0.461538461538462,-0.446153846153846,
-0.430769230769231,-0.415384615384615,-0.4,-0.384615384615385,-0.369230769230769,
-0.353846153846154,-0.338461538461538,-0.323076923076923,-0.307692307692308,
-0.292307692307692,-0.276923076923077,-0.261538461538462,-0.246153846153846,
-0.230769230769231,-0.215384615384615,-0.2,-0.184615384615385,-0.169230769230769,
-0.153846153846154,-0.138461538461538,-0.123076923076923,-0.107692307692308,
-0.0923076923076923,-0.0769230769230769,-0.0615384615384615,-0.0461538461538462,
-0.0307692307692308,-0.0153846153846154,0.),(-1.,1.),.UNSPECIFIED.)
GEOMETRIC_REPRESENTATION_ITEM()
RATIONAL_B_SPLINE_SURFACE(((1.,1.),(1.,1.),(1.,1.),(1.,1.),(1.,1.),(1.,
1.),(1.,1.),(1.,1.),(1.,1.),(1.,1.),(1.,1.),(1.,1.),(1.,1.),(1.,1.),(1.,
1.),(1.,1.),(1.,1.),(1.,1.),(1.,1.),(1.,1.),(1.,1.),(1.,1.),(1.,1.),(1.,
1.),(1.,1.),(1.,1.),(1.,1.),(1.,1.),(1.,1.),(1.,1.),(1.,1.),(1.,1.),(1.,
1.),(1.,1.),(1.,1.),(1.,1.),(1.,1.),(1.,1.),(1.,1.),(1.,1.),(1.,1.),(1.,
1.),(1.,1.),(1.,1.),(1.,1.),(1.,1.),(1.,1.),(1.,1.),(1.,1.),(1.,1.),(1.,
1.),(1.,1.),(1.,1.),(1.,1.),(1.,1.),(1.,1.),(1.,1.),(1.,1.),(1.,1.),(1.,
1.),(1.,1.),(1.,1.),(1.,1.),(1.,1.),(1.,1.),(1.,1.),(1.,1.),(1.,1.),(1.,
1.),(1.,1.)))
REPRESENTATION_ITEM('')
SURFACE()
);
#61=(
BOUNDED_SURFACE()
B_SPLINE_SURFACE(5,1,((#42178,#42179),(#42180,#42181),(#42182,#42183),(#42184,
#42185),(#42186,#42187),(#42188,#42189),(#42190,#42191),(#42192,#42193),
(#42194,#42195),(#42196,#42197),(#42198,#42199),(#42200,#42201),(#42202,
#42203),(#42204,#42205),(#42206,#42207),(#42208,#42209),(#42210,#42211),
(#42212,#42213),(#42214,#42215),(#42216,#42217),(#42218,#42219),(#42220,
#42221),(#42222,#42223),(#42224,#42225),(#42226,#42227),(#42228,#42229),
(#42230,#42231),(#42232,#42233),(#42234,#42235),(#42236,#42237),(#42238,
#42239),(#42240,#42241),(#42242,#42243),(#42244,#42245),(#42246,#42247),
(#42248,#42249),(#42250,#42251),(#42252,#42253),(#42254,#42255),(#42256,
#42257),(#42258,#42259),(#42260,#42261),(#42262,#42263),(#42264,#42265),
(#42266,#42267),(#42268,#42269),(#42270,#42271),(#42272,#42273),(#42274,
#42275),(#42276,#42277),(#42278,#42279),(#42280,#42281),(#42282,#42283),
(#42284,#42285),(#42286,#42287),(#42288,#42289),(#42290,#42291),(#42292,
#42293),(#42294,#42295),(#42296,#42297),(#42298,#42299),(#42300,#42301),
(#42302,#42303),(#42304,#42305),(#42306,#42307),(#42308,#42309),(#42310,
#42311),(#42312,#42313),(#42314,#42315),(#42316,#42317)),.UNSPECIFIED.,
 .F.,.F.,.F.)
B_SPLINE_SURFACE_WITH_KNOTS((6,1,1,1,1,1,1,1,1,1,1,1,1,1,1,1,1,1,1,1,1,
1,1,1,1,1,1,1,1,1,1,1,1,1,1,1,1,1,1,1,1,1,1,1,1,1,1,1,1,1,1,1,1,1,1,1,1,
1,1,1,1,1,1,1,1,6),(2,2),(-1.,-0.984615384615383,-0.969230769230768,-0.953846153846152,
-0.938461538461537,-0.923076923076922,-0.907692307692306,-0.892307692307691,
-0.876923076923076,-0.86153846153846,-0.846153846153845,-0.83076923076923,
-0.815384615384614,-0.799999999999999,-0.784615384615384,-0.769230769230768,
-0.753846153846153,-0.738461538461538,-0.723076923076922,-0.707692307692307,
-0.692307692307692,-0.676923076923076,-0.661538461538461,-0.646153846153846,
-0.63076923076923,-0.615384615384615,-0.6,-0.584615384615384,-0.569230769230769,
-0.553846153846154,-0.538461538461538,-0.523076923076923,-0.507692307692308,
-0.492307692307692,-0.476923076923077,-0.461538461538462,-0.446153846153846,
-0.430769230769231,-0.415384615384615,-0.4,-0.384615384615385,-0.369230769230769,
-0.353846153846154,-0.338461538461538,-0.323076923076923,-0.307692307692308,
-0.292307692307692,-0.276923076923077,-0.261538461538462,-0.246153846153846,
-0.230769230769231,-0.215384615384615,-0.2,-0.184615384615385,-0.169230769230769,
-0.153846153846154,-0.138461538461538,-0.123076923076923,-0.107692307692308,
-0.0923076923076923,-0.0769230769230769,-0.0615384615384615,-0.0461538461538462,
-0.0307692307692308,-0.0153846153846154,0.),(-1.,1.),.UNSPECIFIED.)
GEOMETRIC_REPRESENTATION_ITEM()
RATIONAL_B_SPLINE_SURFACE(((1.,1.),(1.,1.),(1.,1.),(1.,1.),(1.,1.),(1.,
1.),(1.,1.),(1.,1.),(1.,1.),(1.,1.),(1.,1.),(1.,1.),(1.,1.),(1.,1.),(1.,
1.),(1.,1.),(1.,1.),(1.,1.),(1.,1.),(1.,1.),(1.,1.),(1.,1.),(1.,1.),(1.,
1.),(1.,1.),(1.,1.),(1.,1.),(1.,1.),(1.,1.),(1.,1.),(1.,1.),(1.,1.),(1.,
1.),(1.,1.),(1.,1.),(1.,1.),(1.,1.),(1.,1.),(1.,1.),(1.,1.),(1.,1.),(1.,
1.),(1.,1.),(1.,1.),(1.,1.),(1.,1.),(1.,1.),(1.,1.),(1.,1.),(1.,1.),(1.,
1.),(1.,1.),(1.,1.),(1.,1.),(1.,1.),(1.,1.),(1.,1.),(1.,1.),(1.,1.),(1.,
1.),(1.,1.),(1.,1.),(1.,1.),(1.,1.),(1.,1.),(1.,1.),(1.,1.),(1.,1.),(1.,
1.),(1.,1.)))
REPRESENTATION_ITEM('')
SURFACE()
);
#62=(
BOUNDED_SURFACE()
B_SPLINE_SURFACE(5,1,((#42390,#42391),(#42392,#42393),(#42394,#42395),(#42396,
#42397),(#42398,#42399),(#42400,#42401),(#42402,#42403),(#42404,#42405),
(#42406,#42407),(#42408,#42409),(#42410,#42411),(#42412,#42413),(#42414,
#42415),(#42416,#42417),(#42418,#42419),(#42420,#42421),(#42422,#42423),
(#42424,#42425),(#42426,#42427),(#42428,#42429),(#42430,#42431),(#42432,
#42433),(#42434,#42435),(#42436,#42437),(#42438,#42439),(#42440,#42441),
(#42442,#42443),(#42444,#42445),(#42446,#42447),(#42448,#42449),(#42450,
#42451),(#42452,#42453),(#42454,#42455),(#42456,#42457),(#42458,#42459),
(#42460,#42461),(#42462,#42463),(#42464,#42465),(#42466,#42467),(#42468,
#42469),(#42470,#42471),(#42472,#42473),(#42474,#42475),(#42476,#42477),
(#42478,#42479),(#42480,#42481),(#42482,#42483),(#42484,#42485),(#42486,
#42487),(#42488,#42489),(#42490,#42491),(#42492,#42493),(#42494,#42495),
(#42496,#42497),(#42498,#42499),(#42500,#42501),(#42502,#42503),(#42504,
#42505),(#42506,#42507),(#42508,#42509),(#42510,#42511),(#42512,#42513),
(#42514,#42515),(#42516,#42517),(#42518,#42519),(#42520,#42521),(#42522,
#42523),(#42524,#42525),(#42526,#42527),(#42528,#42529)),.UNSPECIFIED.,
 .F.,.F.,.F.)
B_SPLINE_SURFACE_WITH_KNOTS((6,1,1,1,1,1,1,1,1,1,1,1,1,1,1,1,1,1,1,1,1,
1,1,1,1,1,1,1,1,1,1,1,1,1,1,1,1,1,1,1,1,1,1,1,1,1,1,1,1,1,1,1,1,1,1,1,1,
1,1,1,1,1,1,1,1,6),(2,2),(-1.,-0.984615384615383,-0.969230769230768,-0.953846153846152,
-0.938461538461537,-0.923076923076922,-0.907692307692306,-0.892307692307691,
-0.876923076923076,-0.86153846153846,-0.846153846153845,-0.83076923076923,
-0.815384615384614,-0.799999999999999,-0.784615384615384,-0.769230769230768,
-0.753846153846153,-0.738461538461538,-0.723076923076922,-0.707692307692307,
-0.692307692307692,-0.676923076923076,-0.661538461538461,-0.646153846153846,
-0.63076923076923,-0.615384615384615,-0.6,-0.584615384615384,-0.569230769230769,
-0.553846153846154,-0.538461538461538,-0.523076923076923,-0.507692307692308,
-0.492307692307692,-0.476923076923077,-0.461538461538462,-0.446153846153846,
-0.430769230769231,-0.415384615384615,-0.4,-0.384615384615385,-0.369230769230769,
-0.353846153846154,-0.338461538461538,-0.323076923076923,-0.307692307692308,
-0.292307692307692,-0.276923076923077,-0.261538461538462,-0.246153846153846,
-0.230769230769231,-0.215384615384615,-0.2,-0.184615384615385,-0.169230769230769,
-0.153846153846154,-0.138461538461538,-0.123076923076923,-0.107692307692308,
-0.0923076923076923,-0.0769230769230769,-0.0615384615384615,-0.0461538461538462,
-0.0307692307692308,-0.0153846153846154,0.),(-1.,1.),.UNSPECIFIED.)
GEOMETRIC_REPRESENTATION_ITEM()
RATIONAL_B_SPLINE_SURFACE(((1.,1.),(1.,1.),(1.,1.),(1.,1.),(1.,1.),(1.,
1.),(1.,1.),(1.,1.),(1.,1.),(1.,1.),(1.,1.),(1.,1.),(1.,1.),(1.,1.),(1.,
1.),(1.,1.),(1.,1.),(1.,1.),(1.,1.),(1.,1.),(1.,1.),(1.,1.),(1.,1.),(1.,
1.),(1.,1.),(1.,1.),(1.,1.),(1.,1.),(1.,1.),(1.,1.),(1.,1.),(1.,1.),(1.,
1.),(1.,1.),(1.,1.),(1.,1.),(1.,1.),(1.,1.),(1.,1.),(1.,1.),(1.,1.),(1.,
1.),(1.,1.),(1.,1.),(1.,1.),(1.,1.),(1.,1.),(1.,1.),(1.,1.),(1.,1.),(1.,
1.),(1.,1.),(1.,1.),(1.,1.),(1.,1.),(1.,1.),(1.,1.),(1.,1.),(1.,1.),(1.,
1.),(1.,1.),(1.,1.),(1.,1.),(1.,1.),(1.,1.),(1.,1.),(1.,1.),(1.,1.),(1.,
1.),(1.,1.)))
REPRESENTATION_ITEM('')
SURFACE()
);
#63=(
BOUNDED_SURFACE()
B_SPLINE_SURFACE(5,1,((#42620,#42621),(#42622,#42623),(#42624,#42625),(#42626,
#42627),(#42628,#42629),(#42630,#42631),(#42632,#42633),(#42634,#42635),
(#42636,#42637),(#42638,#42639),(#42640,#42641),(#42642,#42643),(#42644,
#42645),(#42646,#42647),(#42648,#42649),(#42650,#42651),(#42652,#42653),
(#42654,#42655),(#42656,#42657),(#42658,#42659),(#42660,#42661),(#42662,
#42663),(#42664,#42665),(#42666,#42667),(#42668,#42669),(#42670,#42671),
(#42672,#42673),(#42674,#42675),(#42676,#42677),(#42678,#42679),(#42680,
#42681),(#42682,#42683),(#42684,#42685),(#42686,#42687),(#42688,#42689),
(#42690,#42691),(#42692,#42693),(#42694,#42695),(#42696,#42697),(#42698,
#42699),(#42700,#42701),(#42702,#42703),(#42704,#42705),(#42706,#42707),
(#42708,#42709),(#42710,#42711),(#42712,#42713),(#42714,#42715),(#42716,
#42717),(#42718,#42719),(#42720,#42721),(#42722,#42723),(#42724,#42725),
(#42726,#42727),(#42728,#42729),(#42730,#42731),(#42732,#42733),(#42734,
#42735),(#42736,#42737),(#42738,#42739),(#42740,#42741),(#42742,#42743),
(#42744,#42745),(#42746,#42747),(#42748,#42749),(#42750,#42751),(#42752,
#42753),(#42754,#42755),(#42756,#42757),(#42758,#42759)),.UNSPECIFIED.,
 .F.,.F.,.F.)
B_SPLINE_SURFACE_WITH_KNOTS((6,1,1,1,1,1,1,1,1,1,1,1,1,1,1,1,1,1,1,1,1,
1,1,1,1,1,1,1,1,1,1,1,1,1,1,1,1,1,1,1,1,1,1,1,1,1,1,1,1,1,1,1,1,1,1,1,1,
1,1,1,1,1,1,1,1,6),(2,2),(-1.,-0.984615384615383,-0.969230769230768,-0.953846153846152,
-0.938461538461537,-0.923076923076922,-0.907692307692306,-0.892307692307691,
-0.876923076923076,-0.86153846153846,-0.846153846153845,-0.83076923076923,
-0.815384615384614,-0.799999999999999,-0.784615384615384,-0.769230769230768,
-0.753846153846153,-0.738461538461538,-0.723076923076922,-0.707692307692307,
-0.692307692307692,-0.676923076923076,-0.661538461538461,-0.646153846153846,
-0.63076923076923,-0.615384615384615,-0.6,-0.584615384615384,-0.569230769230769,
-0.553846153846154,-0.538461538461538,-0.523076923076923,-0.507692307692308,
-0.492307692307692,-0.476923076923077,-0.461538461538462,-0.446153846153846,
-0.430769230769231,-0.415384615384615,-0.4,-0.384615384615385,-0.369230769230769,
-0.353846153846154,-0.338461538461538,-0.323076923076923,-0.307692307692308,
-0.292307692307692,-0.276923076923077,-0.261538461538462,-0.246153846153846,
-0.230769230769231,-0.215384615384615,-0.2,-0.184615384615385,-0.169230769230769,
-0.153846153846154,-0.138461538461538,-0.123076923076923,-0.107692307692308,
-0.0923076923076923,-0.0769230769230769,-0.0615384615384615,-0.0461538461538462,
-0.0307692307692308,-0.0153846153846154,0.),(-1.,1.),.UNSPECIFIED.)
GEOMETRIC_REPRESENTATION_ITEM()
RATIONAL_B_SPLINE_SURFACE(((1.,1.),(1.,1.),(1.,1.),(1.,1.),(1.,1.),(1.,
1.),(1.,1.),(1.,1.),(1.,1.),(1.,1.),(1.,1.),(1.,1.),(1.,1.),(1.,1.),(1.,
1.),(1.,1.),(1.,1.),(1.,1.),(1.,1.),(1.,1.),(1.,1.),(1.,1.),(1.,1.),(1.,
1.),(1.,1.),(1.,1.),(1.,1.),(1.,1.),(1.,1.),(1.,1.),(1.,1.),(1.,1.),(1.,
1.),(1.,1.),(1.,1.),(1.,1.),(1.,1.),(1.,1.),(1.,1.),(1.,1.),(1.,1.),(1.,
1.),(1.,1.),(1.,1.),(1.,1.),(1.,1.),(1.,1.),(1.,1.),(1.,1.),(1.,1.),(1.,
1.),(1.,1.),(1.,1.),(1.,1.),(1.,1.),(1.,1.),(1.,1.),(1.,1.),(1.,1.),(1.,
1.),(1.,1.),(1.,1.),(1.,1.),(1.,1.),(1.,1.),(1.,1.),(1.,1.),(1.,1.),(1.,
1.),(1.,1.)))
REPRESENTATION_ITEM('')
SURFACE()
);
#64=(
BOUNDED_SURFACE()
B_SPLINE_SURFACE(5,1,((#42832,#42833),(#42834,#42835),(#42836,#42837),(#42838,
#42839),(#42840,#42841),(#42842,#42843),(#42844,#42845),(#42846,#42847),
(#42848,#42849),(#42850,#42851),(#42852,#42853),(#42854,#42855),(#42856,
#42857),(#42858,#42859),(#42860,#42861),(#42862,#42863),(#42864,#42865),
(#42866,#42867),(#42868,#42869),(#42870,#42871),(#42872,#42873),(#42874,
#42875),(#42876,#42877),(#42878,#42879),(#42880,#42881),(#42882,#42883),
(#42884,#42885),(#42886,#42887),(#42888,#42889),(#42890,#42891),(#42892,
#42893),(#42894,#42895),(#42896,#42897),(#42898,#42899),(#42900,#42901),
(#42902,#42903),(#42904,#42905),(#42906,#42907),(#42908,#42909),(#42910,
#42911),(#42912,#42913),(#42914,#42915),(#42916,#42917),(#42918,#42919),
(#42920,#42921),(#42922,#42923),(#42924,#42925),(#42926,#42927),(#42928,
#42929),(#42930,#42931),(#42932,#42933),(#42934,#42935),(#42936,#42937),
(#42938,#42939),(#42940,#42941),(#42942,#42943),(#42944,#42945),(#42946,
#42947),(#42948,#42949),(#42950,#42951),(#42952,#42953),(#42954,#42955),
(#42956,#42957),(#42958,#42959),(#42960,#42961),(#42962,#42963),(#42964,
#42965),(#42966,#42967),(#42968,#42969),(#42970,#42971)),.UNSPECIFIED.,
 .F.,.F.,.F.)
B_SPLINE_SURFACE_WITH_KNOTS((6,1,1,1,1,1,1,1,1,1,1,1,1,1,1,1,1,1,1,1,1,
1,1,1,1,1,1,1,1,1,1,1,1,1,1,1,1,1,1,1,1,1,1,1,1,1,1,1,1,1,1,1,1,1,1,1,1,
1,1,1,1,1,1,1,1,6),(2,2),(-1.,-0.984615384615383,-0.969230769230768,-0.953846153846152,
-0.938461538461537,-0.923076923076922,-0.907692307692306,-0.892307692307691,
-0.876923076923076,-0.86153846153846,-0.846153846153845,-0.83076923076923,
-0.815384615384614,-0.799999999999999,-0.784615384615384,-0.769230769230768,
-0.753846153846153,-0.738461538461538,-0.723076923076922,-0.707692307692307,
-0.692307692307692,-0.676923076923076,-0.661538461538461,-0.646153846153846,
-0.63076923076923,-0.615384615384615,-0.6,-0.584615384615384,-0.569230769230769,
-0.553846153846154,-0.538461538461538,-0.523076923076923,-0.507692307692308,
-0.492307692307692,-0.476923076923077,-0.461538461538462,-0.446153846153846,
-0.430769230769231,-0.415384615384615,-0.4,-0.384615384615385,-0.369230769230769,
-0.353846153846154,-0.338461538461538,-0.323076923076923,-0.307692307692308,
-0.292307692307692,-0.276923076923077,-0.261538461538462,-0.246153846153846,
-0.230769230769231,-0.215384615384615,-0.2,-0.184615384615385,-0.169230769230769,
-0.153846153846154,-0.138461538461538,-0.123076923076923,-0.107692307692308,
-0.0923076923076923,-0.0769230769230769,-0.0615384615384615,-0.0461538461538462,
-0.0307692307692308,-0.0153846153846154,0.),(-1.,1.),.UNSPECIFIED.)
GEOMETRIC_REPRESENTATION_ITEM()
RATIONAL_B_SPLINE_SURFACE(((1.,1.),(1.,1.),(1.,1.),(1.,1.),(1.,1.),(1.,
1.),(1.,1.),(1.,1.),(1.,1.),(1.,1.),(1.,1.),(1.,1.),(1.,1.),(1.,1.),(1.,
1.),(1.,1.),(1.,1.),(1.,1.),(1.,1.),(1.,1.),(1.,1.),(1.,1.),(1.,1.),(1.,
1.),(1.,1.),(1.,1.),(1.,1.),(1.,1.),(1.,1.),(1.,1.),(1.,1.),(1.,1.),(1.,
1.),(1.,1.),(1.,1.),(1.,1.),(1.,1.),(1.,1.),(1.,1.),(1.,1.),(1.,1.),(1.,
1.),(1.,1.),(1.,1.),(1.,1.),(1.,1.),(1.,1.),(1.,1.),(1.,1.),(1.,1.),(1.,
1.),(1.,1.),(1.,1.),(1.,1.),(1.,1.),(1.,1.),(1.,1.),(1.,1.),(1.,1.),(1.,
1.),(1.,1.),(1.,1.),(1.,1.),(1.,1.),(1.,1.),(1.,1.),(1.,1.),(1.,1.),(1.,
1.),(1.,1.)))
REPRESENTATION_ITEM('')
SURFACE()
);
#65=(
BOUNDED_SURFACE()
B_SPLINE_SURFACE(5,1,((#43062,#43063),(#43064,#43065),(#43066,#43067),(#43068,
#43069),(#43070,#43071),(#43072,#43073),(#43074,#43075),(#43076,#43077),
(#43078,#43079),(#43080,#43081),(#43082,#43083),(#43084,#43085),(#43086,
#43087),(#43088,#43089),(#43090,#43091),(#43092,#43093),(#43094,#43095),
(#43096,#43097),(#43098,#43099),(#43100,#43101),(#43102,#43103),(#43104,
#43105),(#43106,#43107),(#43108,#43109),(#43110,#43111),(#43112,#43113),
(#43114,#43115),(#43116,#43117),(#43118,#43119),(#43120,#43121),(#43122,
#43123),(#43124,#43125),(#43126,#43127),(#43128,#43129),(#43130,#43131),
(#43132,#43133),(#43134,#43135),(#43136,#43137),(#43138,#43139),(#43140,
#43141),(#43142,#43143),(#43144,#43145),(#43146,#43147),(#43148,#43149),
(#43150,#43151),(#43152,#43153),(#43154,#43155),(#43156,#43157),(#43158,
#43159),(#43160,#43161),(#43162,#43163),(#43164,#43165),(#43166,#43167),
(#43168,#43169),(#43170,#43171),(#43172,#43173),(#43174,#43175),(#43176,
#43177),(#43178,#43179),(#43180,#43181),(#43182,#43183),(#43184,#43185),
(#43186,#43187),(#43188,#43189),(#43190,#43191),(#43192,#43193),(#43194,
#43195),(#43196,#43197),(#43198,#43199),(#43200,#43201)),.UNSPECIFIED.,
 .F.,.F.,.F.)
B_SPLINE_SURFACE_WITH_KNOTS((6,1,1,1,1,1,1,1,1,1,1,1,1,1,1,1,1,1,1,1,1,
1,1,1,1,1,1,1,1,1,1,1,1,1,1,1,1,1,1,1,1,1,1,1,1,1,1,1,1,1,1,1,1,1,1,1,1,
1,1,1,1,1,1,1,1,6),(2,2),(-1.,-0.984615384615383,-0.969230769230768,-0.953846153846152,
-0.938461538461537,-0.923076923076922,-0.907692307692306,-0.892307692307691,
-0.876923076923076,-0.86153846153846,-0.846153846153845,-0.83076923076923,
-0.815384615384614,-0.799999999999999,-0.784615384615384,-0.769230769230768,
-0.753846153846153,-0.738461538461538,-0.723076923076922,-0.707692307692307,
-0.692307692307692,-0.676923076923076,-0.661538461538461,-0.646153846153846,
-0.63076923076923,-0.615384615384615,-0.6,-0.584615384615384,-0.569230769230769,
-0.553846153846154,-0.538461538461538,-0.523076923076923,-0.507692307692308,
-0.492307692307692,-0.476923076923077,-0.461538461538462,-0.446153846153846,
-0.430769230769231,-0.415384615384615,-0.4,-0.384615384615385,-0.369230769230769,
-0.353846153846154,-0.338461538461538,-0.323076923076923,-0.307692307692308,
-0.292307692307692,-0.276923076923077,-0.261538461538462,-0.246153846153846,
-0.230769230769231,-0.215384615384615,-0.2,-0.184615384615385,-0.169230769230769,
-0.153846153846154,-0.138461538461538,-0.123076923076923,-0.107692307692308,
-0.0923076923076923,-0.0769230769230769,-0.0615384615384615,-0.0461538461538462,
-0.0307692307692308,-0.0153846153846154,0.),(-1.,1.),.UNSPECIFIED.)
GEOMETRIC_REPRESENTATION_ITEM()
RATIONAL_B_SPLINE_SURFACE(((1.,1.),(1.,1.),(1.,1.),(1.,1.),(1.,1.),(1.,
1.),(1.,1.),(1.,1.),(1.,1.),(1.,1.),(1.,1.),(1.,1.),(1.,1.),(1.,1.),(1.,
1.),(1.,1.),(1.,1.),(1.,1.),(1.,1.),(1.,1.),(1.,1.),(1.,1.),(1.,1.),(1.,
1.),(1.,1.),(1.,1.),(1.,1.),(1.,1.),(1.,1.),(1.,1.),(1.,1.),(1.,1.),(1.,
1.),(1.,1.),(1.,1.),(1.,1.),(1.,1.),(1.,1.),(1.,1.),(1.,1.),(1.,1.),(1.,
1.),(1.,1.),(1.,1.),(1.,1.),(1.,1.),(1.,1.),(1.,1.),(1.,1.),(1.,1.),(1.,
1.),(1.,1.),(1.,1.),(1.,1.),(1.,1.),(1.,1.),(1.,1.),(1.,1.),(1.,1.),(1.,
1.),(1.,1.),(1.,1.),(1.,1.),(1.,1.),(1.,1.),(1.,1.),(1.,1.),(1.,1.),(1.,
1.),(1.,1.)))
REPRESENTATION_ITEM('')
SURFACE()
);
#66=(
BOUNDED_SURFACE()
B_SPLINE_SURFACE(5,1,((#43274,#43275),(#43276,#43277),(#43278,#43279),(#43280,
#43281),(#43282,#43283),(#43284,#43285),(#43286,#43287),(#43288,#43289),
(#43290,#43291),(#43292,#43293),(#43294,#43295),(#43296,#43297),(#43298,
#43299),(#43300,#43301),(#43302,#43303),(#43304,#43305),(#43306,#43307),
(#43308,#43309),(#43310,#43311),(#43312,#43313),(#43314,#43315),(#43316,
#43317),(#43318,#43319),(#43320,#43321),(#43322,#43323),(#43324,#43325),
(#43326,#43327),(#43328,#43329),(#43330,#43331),(#43332,#43333),(#43334,
#43335),(#43336,#43337),(#43338,#43339),(#43340,#43341),(#43342,#43343),
(#43344,#43345),(#43346,#43347),(#43348,#43349),(#43350,#43351),(#43352,
#43353),(#43354,#43355),(#43356,#43357),(#43358,#43359),(#43360,#43361),
(#43362,#43363),(#43364,#43365),(#43366,#43367),(#43368,#43369),(#43370,
#43371),(#43372,#43373),(#43374,#43375),(#43376,#43377),(#43378,#43379),
(#43380,#43381),(#43382,#43383),(#43384,#43385),(#43386,#43387),(#43388,
#43389),(#43390,#43391),(#43392,#43393),(#43394,#43395),(#43396,#43397),
(#43398,#43399),(#43400,#43401),(#43402,#43403),(#43404,#43405),(#43406,
#43407),(#43408,#43409),(#43410,#43411),(#43412,#43413)),.UNSPECIFIED.,
 .F.,.F.,.F.)
B_SPLINE_SURFACE_WITH_KNOTS((6,1,1,1,1,1,1,1,1,1,1,1,1,1,1,1,1,1,1,1,1,
1,1,1,1,1,1,1,1,1,1,1,1,1,1,1,1,1,1,1,1,1,1,1,1,1,1,1,1,1,1,1,1,1,1,1,1,
1,1,1,1,1,1,1,1,6),(2,2),(-1.,-0.984615384615383,-0.969230769230768,-0.953846153846152,
-0.938461538461537,-0.923076923076922,-0.907692307692306,-0.892307692307691,
-0.876923076923076,-0.86153846153846,-0.846153846153845,-0.83076923076923,
-0.815384615384614,-0.799999999999999,-0.784615384615384,-0.769230769230768,
-0.753846153846153,-0.738461538461538,-0.723076923076922,-0.707692307692307,
-0.692307692307692,-0.676923076923076,-0.661538461538461,-0.646153846153846,
-0.63076923076923,-0.615384615384615,-0.6,-0.584615384615384,-0.569230769230769,
-0.553846153846154,-0.538461538461538,-0.523076923076923,-0.507692307692308,
-0.492307692307692,-0.476923076923077,-0.461538461538462,-0.446153846153846,
-0.430769230769231,-0.415384615384615,-0.4,-0.384615384615385,-0.369230769230769,
-0.353846153846154,-0.338461538461538,-0.323076923076923,-0.307692307692308,
-0.292307692307692,-0.276923076923077,-0.261538461538462,-0.246153846153846,
-0.230769230769231,-0.215384615384615,-0.2,-0.184615384615385,-0.169230769230769,
-0.153846153846154,-0.138461538461538,-0.123076923076923,-0.107692307692308,
-0.0923076923076923,-0.0769230769230769,-0.0615384615384615,-0.0461538461538462,
-0.0307692307692308,-0.0153846153846154,0.),(-1.,1.),.UNSPECIFIED.)
GEOMETRIC_REPRESENTATION_ITEM()
RATIONAL_B_SPLINE_SURFACE(((1.,1.),(1.,1.),(1.,1.),(1.,1.),(1.,1.),(1.,
1.),(1.,1.),(1.,1.),(1.,1.),(1.,1.),(1.,1.),(1.,1.),(1.,1.),(1.,1.),(1.,
1.),(1.,1.),(1.,1.),(1.,1.),(1.,1.),(1.,1.),(1.,1.),(1.,1.),(1.,1.),(1.,
1.),(1.,1.),(1.,1.),(1.,1.),(1.,1.),(1.,1.),(1.,1.),(1.,1.),(1.,1.),(1.,
1.),(1.,1.),(1.,1.),(1.,1.),(1.,1.),(1.,1.),(1.,1.),(1.,1.),(1.,1.),(1.,
1.),(1.,1.),(1.,1.),(1.,1.),(1.,1.),(1.,1.),(1.,1.),(1.,1.),(1.,1.),(1.,
1.),(1.,1.),(1.,1.),(1.,1.),(1.,1.),(1.,1.),(1.,1.),(1.,1.),(1.,1.),(1.,
1.),(1.,1.),(1.,1.),(1.,1.),(1.,1.),(1.,1.),(1.,1.),(1.,1.),(1.,1.),(1.,
1.),(1.,1.)))
REPRESENTATION_ITEM('')
SURFACE()
);
#67=(
BOUNDED_SURFACE()
B_SPLINE_SURFACE(5,1,((#43504,#43505),(#43506,#43507),(#43508,#43509),(#43510,
#43511),(#43512,#43513),(#43514,#43515),(#43516,#43517),(#43518,#43519),
(#43520,#43521),(#43522,#43523),(#43524,#43525),(#43526,#43527),(#43528,
#43529),(#43530,#43531),(#43532,#43533),(#43534,#43535),(#43536,#43537),
(#43538,#43539),(#43540,#43541),(#43542,#43543),(#43544,#43545),(#43546,
#43547),(#43548,#43549),(#43550,#43551),(#43552,#43553),(#43554,#43555),
(#43556,#43557),(#43558,#43559),(#43560,#43561),(#43562,#43563),(#43564,
#43565),(#43566,#43567),(#43568,#43569),(#43570,#43571),(#43572,#43573),
(#43574,#43575),(#43576,#43577),(#43578,#43579),(#43580,#43581),(#43582,
#43583),(#43584,#43585),(#43586,#43587),(#43588,#43589),(#43590,#43591),
(#43592,#43593),(#43594,#43595),(#43596,#43597),(#43598,#43599),(#43600,
#43601),(#43602,#43603),(#43604,#43605),(#43606,#43607),(#43608,#43609),
(#43610,#43611),(#43612,#43613),(#43614,#43615),(#43616,#43617),(#43618,
#43619),(#43620,#43621),(#43622,#43623),(#43624,#43625),(#43626,#43627),
(#43628,#43629),(#43630,#43631),(#43632,#43633),(#43634,#43635),(#43636,
#43637),(#43638,#43639),(#43640,#43641),(#43642,#43643)),.UNSPECIFIED.,
 .F.,.F.,.F.)
B_SPLINE_SURFACE_WITH_KNOTS((6,1,1,1,1,1,1,1,1,1,1,1,1,1,1,1,1,1,1,1,1,
1,1,1,1,1,1,1,1,1,1,1,1,1,1,1,1,1,1,1,1,1,1,1,1,1,1,1,1,1,1,1,1,1,1,1,1,
1,1,1,1,1,1,1,1,6),(2,2),(-1.,-0.984615384615383,-0.969230769230768,-0.953846153846152,
-0.938461538461537,-0.923076923076922,-0.907692307692306,-0.892307692307691,
-0.876923076923076,-0.86153846153846,-0.846153846153845,-0.83076923076923,
-0.815384615384614,-0.799999999999999,-0.784615384615384,-0.769230769230768,
-0.753846153846153,-0.738461538461538,-0.723076923076922,-0.707692307692307,
-0.692307692307692,-0.676923076923076,-0.661538461538461,-0.646153846153846,
-0.63076923076923,-0.615384615384615,-0.6,-0.584615384615384,-0.569230769230769,
-0.553846153846154,-0.538461538461538,-0.523076923076923,-0.507692307692308,
-0.492307692307692,-0.476923076923077,-0.461538461538462,-0.446153846153846,
-0.430769230769231,-0.415384615384615,-0.4,-0.384615384615385,-0.369230769230769,
-0.353846153846154,-0.338461538461538,-0.323076923076923,-0.307692307692308,
-0.292307692307692,-0.276923076923077,-0.261538461538462,-0.246153846153846,
-0.230769230769231,-0.215384615384615,-0.2,-0.184615384615385,-0.169230769230769,
-0.153846153846154,-0.138461538461538,-0.123076923076923,-0.107692307692308,
-0.0923076923076923,-0.0769230769230769,-0.0615384615384615,-0.0461538461538462,
-0.0307692307692308,-0.0153846153846154,0.),(-1.,1.),.UNSPECIFIED.)
GEOMETRIC_REPRESENTATION_ITEM()
RATIONAL_B_SPLINE_SURFACE(((1.,1.),(1.,1.),(1.,1.),(1.,1.),(1.,1.),(1.,
1.),(1.,1.),(1.,1.),(1.,1.),(1.,1.),(1.,1.),(1.,1.),(1.,1.),(1.,1.),(1.,
1.),(1.,1.),(1.,1.),(1.,1.),(1.,1.),(1.,1.),(1.,1.),(1.,1.),(1.,1.),(1.,
1.),(1.,1.),(1.,1.),(1.,1.),(1.,1.),(1.,1.),(1.,1.),(1.,1.),(1.,1.),(1.,
1.),(1.,1.),(1.,1.),(1.,1.),(1.,1.),(1.,1.),(1.,1.),(1.,1.),(1.,1.),(1.,
1.),(1.,1.),(1.,1.),(1.,1.),(1.,1.),(1.,1.),(1.,1.),(1.,1.),(1.,1.),(1.,
1.),(1.,1.),(1.,1.),(1.,1.),(1.,1.),(1.,1.),(1.,1.),(1.,1.),(1.,1.),(1.,
1.),(1.,1.),(1.,1.),(1.,1.),(1.,1.),(1.,1.),(1.,1.),(1.,1.),(1.,1.),(1.,
1.),(1.,1.)))
REPRESENTATION_ITEM('')
SURFACE()
);
#68=(
BOUNDED_SURFACE()
B_SPLINE_SURFACE(5,1,((#43716,#43717),(#43718,#43719),(#43720,#43721),(#43722,
#43723),(#43724,#43725),(#43726,#43727),(#43728,#43729),(#43730,#43731),
(#43732,#43733),(#43734,#43735),(#43736,#43737),(#43738,#43739),(#43740,
#43741),(#43742,#43743),(#43744,#43745),(#43746,#43747),(#43748,#43749),
(#43750,#43751),(#43752,#43753),(#43754,#43755),(#43756,#43757),(#43758,
#43759),(#43760,#43761),(#43762,#43763),(#43764,#43765),(#43766,#43767),
(#43768,#43769),(#43770,#43771),(#43772,#43773),(#43774,#43775),(#43776,
#43777),(#43778,#43779),(#43780,#43781),(#43782,#43783),(#43784,#43785),
(#43786,#43787),(#43788,#43789),(#43790,#43791),(#43792,#43793),(#43794,
#43795),(#43796,#43797),(#43798,#43799),(#43800,#43801),(#43802,#43803),
(#43804,#43805),(#43806,#43807),(#43808,#43809),(#43810,#43811),(#43812,
#43813),(#43814,#43815),(#43816,#43817),(#43818,#43819),(#43820,#43821),
(#43822,#43823),(#43824,#43825),(#43826,#43827),(#43828,#43829),(#43830,
#43831),(#43832,#43833),(#43834,#43835),(#43836,#43837),(#43838,#43839),
(#43840,#43841),(#43842,#43843),(#43844,#43845),(#43846,#43847),(#43848,
#43849),(#43850,#43851),(#43852,#43853),(#43854,#43855)),.UNSPECIFIED.,
 .F.,.F.,.F.)
B_SPLINE_SURFACE_WITH_KNOTS((6,1,1,1,1,1,1,1,1,1,1,1,1,1,1,1,1,1,1,1,1,
1,1,1,1,1,1,1,1,1,1,1,1,1,1,1,1,1,1,1,1,1,1,1,1,1,1,1,1,1,1,1,1,1,1,1,1,
1,1,1,1,1,1,1,1,6),(2,2),(-1.,-0.984615384615383,-0.969230769230768,-0.953846153846152,
-0.938461538461537,-0.923076923076922,-0.907692307692306,-0.892307692307691,
-0.876923076923076,-0.86153846153846,-0.846153846153845,-0.83076923076923,
-0.815384615384614,-0.799999999999999,-0.784615384615384,-0.769230769230768,
-0.753846153846153,-0.738461538461538,-0.723076923076922,-0.707692307692307,
-0.692307692307692,-0.676923076923076,-0.661538461538461,-0.646153846153846,
-0.63076923076923,-0.615384615384615,-0.6,-0.584615384615384,-0.569230769230769,
-0.553846153846154,-0.538461538461538,-0.523076923076923,-0.507692307692308,
-0.492307692307692,-0.476923076923077,-0.461538461538462,-0.446153846153846,
-0.430769230769231,-0.415384615384615,-0.4,-0.384615384615385,-0.369230769230769,
-0.353846153846154,-0.338461538461538,-0.323076923076923,-0.307692307692308,
-0.292307692307692,-0.276923076923077,-0.261538461538462,-0.246153846153846,
-0.230769230769231,-0.215384615384615,-0.2,-0.184615384615385,-0.169230769230769,
-0.153846153846154,-0.138461538461538,-0.123076923076923,-0.107692307692308,
-0.0923076923076923,-0.0769230769230769,-0.0615384615384615,-0.0461538461538462,
-0.0307692307692308,-0.0153846153846154,0.),(-1.,1.),.UNSPECIFIED.)
GEOMETRIC_REPRESENTATION_ITEM()
RATIONAL_B_SPLINE_SURFACE(((1.,1.),(1.,1.),(1.,1.),(1.,1.),(1.,1.),(1.,
1.),(1.,1.),(1.,1.),(1.,1.),(1.,1.),(1.,1.),(1.,1.),(1.,1.),(1.,1.),(1.,
1.),(1.,1.),(1.,1.),(1.,1.),(1.,1.),(1.,1.),(1.,1.),(1.,1.),(1.,1.),(1.,
1.),(1.,1.),(1.,1.),(1.,1.),(1.,1.),(1.,1.),(1.,1.),(1.,1.),(1.,1.),(1.,
1.),(1.,1.),(1.,1.),(1.,1.),(1.,1.),(1.,1.),(1.,1.),(1.,1.),(1.,1.),(1.,
1.),(1.,1.),(1.,1.),(1.,1.),(1.,1.),(1.,1.),(1.,1.),(1.,1.),(1.,1.),(1.,
1.),(1.,1.),(1.,1.),(1.,1.),(1.,1.),(1.,1.),(1.,1.),(1.,1.),(1.,1.),(1.,
1.),(1.,1.),(1.,1.),(1.,1.),(1.,1.),(1.,1.),(1.,1.),(1.,1.),(1.,1.),(1.,
1.),(1.,1.)))
REPRESENTATION_ITEM('')
SURFACE()
);
#69=(
BOUNDED_SURFACE()
B_SPLINE_SURFACE(5,1,((#43946,#43947),(#43948,#43949),(#43950,#43951),(#43952,
#43953),(#43954,#43955),(#43956,#43957),(#43958,#43959),(#43960,#43961),
(#43962,#43963),(#43964,#43965),(#43966,#43967),(#43968,#43969),(#43970,
#43971),(#43972,#43973),(#43974,#43975),(#43976,#43977),(#43978,#43979),
(#43980,#43981),(#43982,#43983),(#43984,#43985),(#43986,#43987),(#43988,
#43989),(#43990,#43991),(#43992,#43993),(#43994,#43995),(#43996,#43997),
(#43998,#43999),(#44000,#44001),(#44002,#44003),(#44004,#44005),(#44006,
#44007),(#44008,#44009),(#44010,#44011),(#44012,#44013),(#44014,#44015),
(#44016,#44017),(#44018,#44019),(#44020,#44021),(#44022,#44023),(#44024,
#44025),(#44026,#44027),(#44028,#44029),(#44030,#44031),(#44032,#44033),
(#44034,#44035),(#44036,#44037),(#44038,#44039),(#44040,#44041),(#44042,
#44043),(#44044,#44045),(#44046,#44047),(#44048,#44049),(#44050,#44051),
(#44052,#44053),(#44054,#44055),(#44056,#44057),(#44058,#44059),(#44060,
#44061),(#44062,#44063),(#44064,#44065),(#44066,#44067),(#44068,#44069),
(#44070,#44071),(#44072,#44073),(#44074,#44075),(#44076,#44077),(#44078,
#44079),(#44080,#44081),(#44082,#44083),(#44084,#44085)),.UNSPECIFIED.,
 .F.,.F.,.F.)
B_SPLINE_SURFACE_WITH_KNOTS((6,1,1,1,1,1,1,1,1,1,1,1,1,1,1,1,1,1,1,1,1,
1,1,1,1,1,1,1,1,1,1,1,1,1,1,1,1,1,1,1,1,1,1,1,1,1,1,1,1,1,1,1,1,1,1,1,1,
1,1,1,1,1,1,1,1,6),(2,2),(-1.,-0.984615384615383,-0.969230769230768,-0.953846153846152,
-0.938461538461537,-0.923076923076922,-0.907692307692306,-0.892307692307691,
-0.876923076923076,-0.86153846153846,-0.846153846153845,-0.83076923076923,
-0.815384615384614,-0.799999999999999,-0.784615384615384,-0.769230769230768,
-0.753846153846153,-0.738461538461538,-0.723076923076922,-0.707692307692307,
-0.692307692307692,-0.676923076923076,-0.661538461538461,-0.646153846153846,
-0.63076923076923,-0.615384615384615,-0.6,-0.584615384615384,-0.569230769230769,
-0.553846153846154,-0.538461538461538,-0.523076923076923,-0.507692307692308,
-0.492307692307692,-0.476923076923077,-0.461538461538462,-0.446153846153846,
-0.430769230769231,-0.415384615384615,-0.4,-0.384615384615385,-0.369230769230769,
-0.353846153846154,-0.338461538461538,-0.323076923076923,-0.307692307692308,
-0.292307692307692,-0.276923076923077,-0.261538461538462,-0.246153846153846,
-0.230769230769231,-0.215384615384615,-0.2,-0.184615384615385,-0.169230769230769,
-0.153846153846154,-0.138461538461538,-0.123076923076923,-0.107692307692308,
-0.0923076923076923,-0.0769230769230769,-0.0615384615384615,-0.0461538461538462,
-0.0307692307692308,-0.0153846153846154,0.),(-1.,1.),.UNSPECIFIED.)
GEOMETRIC_REPRESENTATION_ITEM()
RATIONAL_B_SPLINE_SURFACE(((1.,1.),(1.,1.),(1.,1.),(1.,1.),(1.,1.),(1.,
1.),(1.,1.),(1.,1.),(1.,1.),(1.,1.),(1.,1.),(1.,1.),(1.,1.),(1.,1.),(1.,
1.),(1.,1.),(1.,1.),(1.,1.),(1.,1.),(1.,1.),(1.,1.),(1.,1.),(1.,1.),(1.,
1.),(1.,1.),(1.,1.),(1.,1.),(1.,1.),(1.,1.),(1.,1.),(1.,1.),(1.,1.),(1.,
1.),(1.,1.),(1.,1.),(1.,1.),(1.,1.),(1.,1.),(1.,1.),(1.,1.),(1.,1.),(1.,
1.),(1.,1.),(1.,1.),(1.,1.),(1.,1.),(1.,1.),(1.,1.),(1.,1.),(1.,1.),(1.,
1.),(1.,1.),(1.,1.),(1.,1.),(1.,1.),(1.,1.),(1.,1.),(1.,1.),(1.,1.),(1.,
1.),(1.,1.),(1.,1.),(1.,1.),(1.,1.),(1.,1.),(1.,1.),(1.,1.),(1.,1.),(1.,
1.),(1.,1.)))
REPRESENTATION_ITEM('')
SURFACE()
);
#70=(
BOUNDED_SURFACE()
B_SPLINE_SURFACE(5,1,((#44158,#44159),(#44160,#44161),(#44162,#44163),(#44164,
#44165),(#44166,#44167),(#44168,#44169),(#44170,#44171),(#44172,#44173),
(#44174,#44175),(#44176,#44177),(#44178,#44179),(#44180,#44181),(#44182,
#44183),(#44184,#44185),(#44186,#44187),(#44188,#44189),(#44190,#44191),
(#44192,#44193),(#44194,#44195),(#44196,#44197),(#44198,#44199),(#44200,
#44201),(#44202,#44203),(#44204,#44205),(#44206,#44207),(#44208,#44209),
(#44210,#44211),(#44212,#44213),(#44214,#44215),(#44216,#44217),(#44218,
#44219),(#44220,#44221),(#44222,#44223),(#44224,#44225),(#44226,#44227),
(#44228,#44229),(#44230,#44231),(#44232,#44233),(#44234,#44235),(#44236,
#44237),(#44238,#44239),(#44240,#44241),(#44242,#44243),(#44244,#44245),
(#44246,#44247),(#44248,#44249),(#44250,#44251),(#44252,#44253),(#44254,
#44255),(#44256,#44257),(#44258,#44259),(#44260,#44261),(#44262,#44263),
(#44264,#44265),(#44266,#44267),(#44268,#44269),(#44270,#44271),(#44272,
#44273),(#44274,#44275),(#44276,#44277),(#44278,#44279),(#44280,#44281),
(#44282,#44283),(#44284,#44285),(#44286,#44287),(#44288,#44289),(#44290,
#44291),(#44292,#44293),(#44294,#44295),(#44296,#44297)),.UNSPECIFIED.,
 .F.,.F.,.F.)
B_SPLINE_SURFACE_WITH_KNOTS((6,1,1,1,1,1,1,1,1,1,1,1,1,1,1,1,1,1,1,1,1,
1,1,1,1,1,1,1,1,1,1,1,1,1,1,1,1,1,1,1,1,1,1,1,1,1,1,1,1,1,1,1,1,1,1,1,1,
1,1,1,1,1,1,1,1,6),(2,2),(-1.,-0.984615384615383,-0.969230769230768,-0.953846153846152,
-0.938461538461537,-0.923076923076922,-0.907692307692306,-0.892307692307691,
-0.876923076923076,-0.86153846153846,-0.846153846153845,-0.83076923076923,
-0.815384615384614,-0.799999999999999,-0.784615384615384,-0.769230769230768,
-0.753846153846153,-0.738461538461538,-0.723076923076922,-0.707692307692307,
-0.692307692307692,-0.676923076923076,-0.661538461538461,-0.646153846153846,
-0.63076923076923,-0.615384615384615,-0.6,-0.584615384615384,-0.569230769230769,
-0.553846153846154,-0.538461538461538,-0.523076923076923,-0.507692307692308,
-0.492307692307692,-0.476923076923077,-0.461538461538462,-0.446153846153846,
-0.430769230769231,-0.415384615384615,-0.4,-0.384615384615385,-0.369230769230769,
-0.353846153846154,-0.338461538461538,-0.323076923076923,-0.307692307692308,
-0.292307692307692,-0.276923076923077,-0.261538461538462,-0.246153846153846,
-0.230769230769231,-0.215384615384615,-0.2,-0.184615384615385,-0.169230769230769,
-0.153846153846154,-0.138461538461538,-0.123076923076923,-0.107692307692308,
-0.0923076923076923,-0.0769230769230769,-0.0615384615384615,-0.0461538461538462,
-0.0307692307692308,-0.0153846153846154,0.),(-1.,1.),.UNSPECIFIED.)
GEOMETRIC_REPRESENTATION_ITEM()
RATIONAL_B_SPLINE_SURFACE(((1.,1.),(1.,1.),(1.,1.),(1.,1.),(1.,1.),(1.,
1.),(1.,1.),(1.,1.),(1.,1.),(1.,1.),(1.,1.),(1.,1.),(1.,1.),(1.,1.),(1.,
1.),(1.,1.),(1.,1.),(1.,1.),(1.,1.),(1.,1.),(1.,1.),(1.,1.),(1.,1.),(1.,
1.),(1.,1.),(1.,1.),(1.,1.),(1.,1.),(1.,1.),(1.,1.),(1.,1.),(1.,1.),(1.,
1.),(1.,1.),(1.,1.),(1.,1.),(1.,1.),(1.,1.),(1.,1.),(1.,1.),(1.,1.),(1.,
1.),(1.,1.),(1.,1.),(1.,1.),(1.,1.),(1.,1.),(1.,1.),(1.,1.),(1.,1.),(1.,
1.),(1.,1.),(1.,1.),(1.,1.),(1.,1.),(1.,1.),(1.,1.),(1.,1.),(1.,1.),(1.,
1.),(1.,1.),(1.,1.),(1.,1.),(1.,1.),(1.,1.),(1.,1.),(1.,1.),(1.,1.),(1.,
1.),(1.,1.)))
REPRESENTATION_ITEM('')
SURFACE()
);
#71=(
BOUNDED_SURFACE()
B_SPLINE_SURFACE(5,1,((#44388,#44389),(#44390,#44391),(#44392,#44393),(#44394,
#44395),(#44396,#44397),(#44398,#44399),(#44400,#44401),(#44402,#44403),
(#44404,#44405),(#44406,#44407),(#44408,#44409),(#44410,#44411),(#44412,
#44413),(#44414,#44415),(#44416,#44417),(#44418,#44419),(#44420,#44421),
(#44422,#44423),(#44424,#44425),(#44426,#44427),(#44428,#44429),(#44430,
#44431),(#44432,#44433),(#44434,#44435),(#44436,#44437),(#44438,#44439),
(#44440,#44441),(#44442,#44443),(#44444,#44445),(#44446,#44447),(#44448,
#44449),(#44450,#44451),(#44452,#44453),(#44454,#44455),(#44456,#44457),
(#44458,#44459),(#44460,#44461),(#44462,#44463),(#44464,#44465),(#44466,
#44467),(#44468,#44469),(#44470,#44471),(#44472,#44473),(#44474,#44475),
(#44476,#44477),(#44478,#44479),(#44480,#44481),(#44482,#44483),(#44484,
#44485),(#44486,#44487),(#44488,#44489),(#44490,#44491),(#44492,#44493),
(#44494,#44495),(#44496,#44497),(#44498,#44499),(#44500,#44501),(#44502,
#44503),(#44504,#44505),(#44506,#44507),(#44508,#44509),(#44510,#44511),
(#44512,#44513),(#44514,#44515),(#44516,#44517),(#44518,#44519),(#44520,
#44521),(#44522,#44523),(#44524,#44525),(#44526,#44527)),.UNSPECIFIED.,
 .F.,.F.,.F.)
B_SPLINE_SURFACE_WITH_KNOTS((6,1,1,1,1,1,1,1,1,1,1,1,1,1,1,1,1,1,1,1,1,
1,1,1,1,1,1,1,1,1,1,1,1,1,1,1,1,1,1,1,1,1,1,1,1,1,1,1,1,1,1,1,1,1,1,1,1,
1,1,1,1,1,1,1,1,6),(2,2),(-1.,-0.984615384615383,-0.969230769230768,-0.953846153846152,
-0.938461538461537,-0.923076923076922,-0.907692307692306,-0.892307692307691,
-0.876923076923076,-0.86153846153846,-0.846153846153845,-0.83076923076923,
-0.815384615384614,-0.799999999999999,-0.784615384615384,-0.769230769230768,
-0.753846153846153,-0.738461538461538,-0.723076923076922,-0.707692307692307,
-0.692307692307692,-0.676923076923076,-0.661538461538461,-0.646153846153846,
-0.63076923076923,-0.615384615384615,-0.6,-0.584615384615384,-0.569230769230769,
-0.553846153846154,-0.538461538461538,-0.523076923076923,-0.507692307692308,
-0.492307692307692,-0.476923076923077,-0.461538461538462,-0.446153846153846,
-0.430769230769231,-0.415384615384615,-0.4,-0.384615384615385,-0.369230769230769,
-0.353846153846154,-0.338461538461538,-0.323076923076923,-0.307692307692308,
-0.292307692307692,-0.276923076923077,-0.261538461538462,-0.246153846153846,
-0.230769230769231,-0.215384615384615,-0.2,-0.184615384615385,-0.169230769230769,
-0.153846153846154,-0.138461538461538,-0.123076923076923,-0.107692307692308,
-0.0923076923076923,-0.0769230769230769,-0.0615384615384615,-0.0461538461538462,
-0.0307692307692308,-0.0153846153846154,0.),(-1.,1.),.UNSPECIFIED.)
GEOMETRIC_REPRESENTATION_ITEM()
RATIONAL_B_SPLINE_SURFACE(((1.,1.),(1.,1.),(1.,1.),(1.,1.),(1.,1.),(1.,
1.),(1.,1.),(1.,1.),(1.,1.),(1.,1.),(1.,1.),(1.,1.),(1.,1.),(1.,1.),(1.,
1.),(1.,1.),(1.,1.),(1.,1.),(1.,1.),(1.,1.),(1.,1.),(1.,1.),(1.,1.),(1.,
1.),(1.,1.),(1.,1.),(1.,1.),(1.,1.),(1.,1.),(1.,1.),(1.,1.),(1.,1.),(1.,
1.),(1.,1.),(1.,1.),(1.,1.),(1.,1.),(1.,1.),(1.,1.),(1.,1.),(1.,1.),(1.,
1.),(1.,1.),(1.,1.),(1.,1.),(1.,1.),(1.,1.),(1.,1.),(1.,1.),(1.,1.),(1.,
1.),(1.,1.),(1.,1.),(1.,1.),(1.,1.),(1.,1.),(1.,1.),(1.,1.),(1.,1.),(1.,
1.),(1.,1.),(1.,1.),(1.,1.),(1.,1.),(1.,1.),(1.,1.),(1.,1.),(1.,1.),(1.,
1.),(1.,1.)))
REPRESENTATION_ITEM('')
SURFACE()
);
#72=(
BOUNDED_SURFACE()
B_SPLINE_SURFACE(5,1,((#44600,#44601),(#44602,#44603),(#44604,#44605),(#44606,
#44607),(#44608,#44609),(#44610,#44611),(#44612,#44613),(#44614,#44615),
(#44616,#44617),(#44618,#44619),(#44620,#44621),(#44622,#44623),(#44624,
#44625),(#44626,#44627),(#44628,#44629),(#44630,#44631),(#44632,#44633),
(#44634,#44635),(#44636,#44637),(#44638,#44639),(#44640,#44641),(#44642,
#44643),(#44644,#44645),(#44646,#44647),(#44648,#44649),(#44650,#44651),
(#44652,#44653),(#44654,#44655),(#44656,#44657),(#44658,#44659),(#44660,
#44661),(#44662,#44663),(#44664,#44665),(#44666,#44667),(#44668,#44669),
(#44670,#44671),(#44672,#44673),(#44674,#44675),(#44676,#44677),(#44678,
#44679),(#44680,#44681),(#44682,#44683),(#44684,#44685),(#44686,#44687),
(#44688,#44689),(#44690,#44691),(#44692,#44693),(#44694,#44695),(#44696,
#44697),(#44698,#44699),(#44700,#44701),(#44702,#44703),(#44704,#44705),
(#44706,#44707),(#44708,#44709),(#44710,#44711),(#44712,#44713),(#44714,
#44715),(#44716,#44717),(#44718,#44719),(#44720,#44721),(#44722,#44723),
(#44724,#44725),(#44726,#44727),(#44728,#44729),(#44730,#44731),(#44732,
#44733),(#44734,#44735),(#44736,#44737),(#44738,#44739)),.UNSPECIFIED.,
 .F.,.F.,.F.)
B_SPLINE_SURFACE_WITH_KNOTS((6,1,1,1,1,1,1,1,1,1,1,1,1,1,1,1,1,1,1,1,1,
1,1,1,1,1,1,1,1,1,1,1,1,1,1,1,1,1,1,1,1,1,1,1,1,1,1,1,1,1,1,1,1,1,1,1,1,
1,1,1,1,1,1,1,1,6),(2,2),(-1.,-0.984615384615383,-0.969230769230768,-0.953846153846152,
-0.938461538461537,-0.923076923076922,-0.907692307692306,-0.892307692307691,
-0.876923076923076,-0.86153846153846,-0.846153846153845,-0.83076923076923,
-0.815384615384614,-0.799999999999999,-0.784615384615384,-0.769230769230768,
-0.753846153846153,-0.738461538461538,-0.723076923076922,-0.707692307692307,
-0.692307692307692,-0.676923076923076,-0.661538461538461,-0.646153846153846,
-0.63076923076923,-0.615384615384615,-0.6,-0.584615384615384,-0.569230769230769,
-0.553846153846154,-0.538461538461538,-0.523076923076923,-0.507692307692308,
-0.492307692307692,-0.476923076923077,-0.461538461538462,-0.446153846153846,
-0.430769230769231,-0.415384615384615,-0.4,-0.384615384615385,-0.369230769230769,
-0.353846153846154,-0.338461538461538,-0.323076923076923,-0.307692307692308,
-0.292307692307692,-0.276923076923077,-0.261538461538462,-0.246153846153846,
-0.230769230769231,-0.215384615384615,-0.2,-0.184615384615385,-0.169230769230769,
-0.153846153846154,-0.138461538461538,-0.123076923076923,-0.107692307692308,
-0.0923076923076923,-0.0769230769230769,-0.0615384615384615,-0.0461538461538462,
-0.0307692307692308,-0.0153846153846154,0.),(-1.,1.),.UNSPECIFIED.)
GEOMETRIC_REPRESENTATION_ITEM()
RATIONAL_B_SPLINE_SURFACE(((1.,1.),(1.,1.),(1.,1.),(1.,1.),(1.,1.),(1.,
1.),(1.,1.),(1.,1.),(1.,1.),(1.,1.),(1.,1.),(1.,1.),(1.,1.),(1.,1.),(1.,
1.),(1.,1.),(1.,1.),(1.,1.),(1.,1.),(1.,1.),(1.,1.),(1.,1.),(1.,1.),(1.,
1.),(1.,1.),(1.,1.),(1.,1.),(1.,1.),(1.,1.),(1.,1.),(1.,1.),(1.,1.),(1.,
1.),(1.,1.),(1.,1.),(1.,1.),(1.,1.),(1.,1.),(1.,1.),(1.,1.),(1.,1.),(1.,
1.),(1.,1.),(1.,1.),(1.,1.),(1.,1.),(1.,1.),(1.,1.),(1.,1.),(1.,1.),(1.,
1.),(1.,1.),(1.,1.),(1.,1.),(1.,1.),(1.,1.),(1.,1.),(1.,1.),(1.,1.),(1.,
1.),(1.,1.),(1.,1.),(1.,1.),(1.,1.),(1.,1.),(1.,1.),(1.,1.),(1.,1.),(1.,
1.),(1.,1.)))
REPRESENTATION_ITEM('')
SURFACE()
);
#73=(
BOUNDED_SURFACE()
B_SPLINE_SURFACE(5,1,((#44830,#44831),(#44832,#44833),(#44834,#44835),(#44836,
#44837),(#44838,#44839),(#44840,#44841),(#44842,#44843),(#44844,#44845),
(#44846,#44847),(#44848,#44849),(#44850,#44851),(#44852,#44853),(#44854,
#44855),(#44856,#44857),(#44858,#44859),(#44860,#44861),(#44862,#44863),
(#44864,#44865),(#44866,#44867),(#44868,#44869),(#44870,#44871),(#44872,
#44873),(#44874,#44875),(#44876,#44877),(#44878,#44879),(#44880,#44881),
(#44882,#44883),(#44884,#44885),(#44886,#44887),(#44888,#44889),(#44890,
#44891),(#44892,#44893),(#44894,#44895),(#44896,#44897),(#44898,#44899),
(#44900,#44901),(#44902,#44903),(#44904,#44905),(#44906,#44907),(#44908,
#44909),(#44910,#44911),(#44912,#44913),(#44914,#44915),(#44916,#44917),
(#44918,#44919),(#44920,#44921),(#44922,#44923),(#44924,#44925),(#44926,
#44927),(#44928,#44929),(#44930,#44931),(#44932,#44933),(#44934,#44935),
(#44936,#44937),(#44938,#44939),(#44940,#44941),(#44942,#44943),(#44944,
#44945),(#44946,#44947),(#44948,#44949),(#44950,#44951),(#44952,#44953),
(#44954,#44955),(#44956,#44957),(#44958,#44959),(#44960,#44961),(#44962,
#44963),(#44964,#44965),(#44966,#44967),(#44968,#44969)),.UNSPECIFIED.,
 .F.,.F.,.F.)
B_SPLINE_SURFACE_WITH_KNOTS((6,1,1,1,1,1,1,1,1,1,1,1,1,1,1,1,1,1,1,1,1,
1,1,1,1,1,1,1,1,1,1,1,1,1,1,1,1,1,1,1,1,1,1,1,1,1,1,1,1,1,1,1,1,1,1,1,1,
1,1,1,1,1,1,1,1,6),(2,2),(-1.,-0.984615384615383,-0.969230769230768,-0.953846153846152,
-0.938461538461537,-0.923076923076922,-0.907692307692306,-0.892307692307691,
-0.876923076923076,-0.86153846153846,-0.846153846153845,-0.83076923076923,
-0.815384615384614,-0.799999999999999,-0.784615384615384,-0.769230769230768,
-0.753846153846153,-0.738461538461538,-0.723076923076922,-0.707692307692307,
-0.692307692307692,-0.676923076923076,-0.661538461538461,-0.646153846153846,
-0.63076923076923,-0.615384615384615,-0.6,-0.584615384615384,-0.569230769230769,
-0.553846153846154,-0.538461538461538,-0.523076923076923,-0.507692307692308,
-0.492307692307692,-0.476923076923077,-0.461538461538462,-0.446153846153846,
-0.430769230769231,-0.415384615384615,-0.4,-0.384615384615385,-0.369230769230769,
-0.353846153846154,-0.338461538461538,-0.323076923076923,-0.307692307692308,
-0.292307692307692,-0.276923076923077,-0.261538461538462,-0.246153846153846,
-0.230769230769231,-0.215384615384615,-0.2,-0.184615384615385,-0.169230769230769,
-0.153846153846154,-0.138461538461538,-0.123076923076923,-0.107692307692308,
-0.0923076923076923,-0.0769230769230769,-0.0615384615384615,-0.0461538461538462,
-0.0307692307692308,-0.0153846153846154,0.),(-1.,1.),.UNSPECIFIED.)
GEOMETRIC_REPRESENTATION_ITEM()
RATIONAL_B_SPLINE_SURFACE(((1.,1.),(1.,1.),(1.,1.),(1.,1.),(1.,1.),(1.,
1.),(1.,1.),(1.,1.),(1.,1.),(1.,1.),(1.,1.),(1.,1.),(1.,1.),(1.,1.),(1.,
1.),(1.,1.),(1.,1.),(1.,1.),(1.,1.),(1.,1.),(1.,1.),(1.,1.),(1.,1.),(1.,
1.),(1.,1.),(1.,1.),(1.,1.),(1.,1.),(1.,1.),(1.,1.),(1.,1.),(1.,1.),(1.,
1.),(1.,1.),(1.,1.),(1.,1.),(1.,1.),(1.,1.),(1.,1.),(1.,1.),(1.,1.),(1.,
1.),(1.,1.),(1.,1.),(1.,1.),(1.,1.),(1.,1.),(1.,1.),(1.,1.),(1.,1.),(1.,
1.),(1.,1.),(1.,1.),(1.,1.),(1.,1.),(1.,1.),(1.,1.),(1.,1.),(1.,1.),(1.,
1.),(1.,1.),(1.,1.),(1.,1.),(1.,1.),(1.,1.),(1.,1.),(1.,1.),(1.,1.),(1.,
1.),(1.,1.)))
REPRESENTATION_ITEM('')
SURFACE()
);
#74=(
BOUNDED_SURFACE()
B_SPLINE_SURFACE(5,1,((#45042,#45043),(#45044,#45045),(#45046,#45047),(#45048,
#45049),(#45050,#45051),(#45052,#45053),(#45054,#45055),(#45056,#45057),
(#45058,#45059),(#45060,#45061),(#45062,#45063),(#45064,#45065),(#45066,
#45067),(#45068,#45069),(#45070,#45071),(#45072,#45073),(#45074,#45075),
(#45076,#45077),(#45078,#45079),(#45080,#45081),(#45082,#45083),(#45084,
#45085),(#45086,#45087),(#45088,#45089),(#45090,#45091),(#45092,#45093),
(#45094,#45095),(#45096,#45097),(#45098,#45099),(#45100,#45101),(#45102,
#45103),(#45104,#45105),(#45106,#45107),(#45108,#45109),(#45110,#45111),
(#45112,#45113),(#45114,#45115),(#45116,#45117),(#45118,#45119),(#45120,
#45121),(#45122,#45123),(#45124,#45125),(#45126,#45127),(#45128,#45129),
(#45130,#45131),(#45132,#45133),(#45134,#45135),(#45136,#45137),(#45138,
#45139),(#45140,#45141),(#45142,#45143),(#45144,#45145),(#45146,#45147),
(#45148,#45149),(#45150,#45151),(#45152,#45153),(#45154,#45155),(#45156,
#45157),(#45158,#45159),(#45160,#45161),(#45162,#45163),(#45164,#45165),
(#45166,#45167),(#45168,#45169),(#45170,#45171),(#45172,#45173),(#45174,
#45175),(#45176,#45177),(#45178,#45179),(#45180,#45181)),.UNSPECIFIED.,
 .F.,.F.,.F.)
B_SPLINE_SURFACE_WITH_KNOTS((6,1,1,1,1,1,1,1,1,1,1,1,1,1,1,1,1,1,1,1,1,
1,1,1,1,1,1,1,1,1,1,1,1,1,1,1,1,1,1,1,1,1,1,1,1,1,1,1,1,1,1,1,1,1,1,1,1,
1,1,1,1,1,1,1,1,6),(2,2),(-1.,-0.984615384615383,-0.969230769230768,-0.953846153846152,
-0.938461538461537,-0.923076923076922,-0.907692307692306,-0.892307692307691,
-0.876923076923076,-0.86153846153846,-0.846153846153845,-0.83076923076923,
-0.815384615384614,-0.799999999999999,-0.784615384615384,-0.769230769230768,
-0.753846153846153,-0.738461538461538,-0.723076923076922,-0.707692307692307,
-0.692307692307692,-0.676923076923076,-0.661538461538461,-0.646153846153846,
-0.63076923076923,-0.615384615384615,-0.6,-0.584615384615384,-0.569230769230769,
-0.553846153846154,-0.538461538461538,-0.523076923076923,-0.507692307692308,
-0.492307692307692,-0.476923076923077,-0.461538461538462,-0.446153846153846,
-0.430769230769231,-0.415384615384615,-0.4,-0.384615384615385,-0.369230769230769,
-0.353846153846154,-0.338461538461538,-0.323076923076923,-0.307692307692308,
-0.292307692307692,-0.276923076923077,-0.261538461538462,-0.246153846153846,
-0.230769230769231,-0.215384615384615,-0.2,-0.184615384615385,-0.169230769230769,
-0.153846153846154,-0.138461538461538,-0.123076923076923,-0.107692307692308,
-0.0923076923076923,-0.0769230769230769,-0.0615384615384615,-0.0461538461538462,
-0.0307692307692308,-0.0153846153846154,0.),(-1.,1.),.UNSPECIFIED.)
GEOMETRIC_REPRESENTATION_ITEM()
RATIONAL_B_SPLINE_SURFACE(((1.,1.),(1.,1.),(1.,1.),(1.,1.),(1.,1.),(1.,
1.),(1.,1.),(1.,1.),(1.,1.),(1.,1.),(1.,1.),(1.,1.),(1.,1.),(1.,1.),(1.,
1.),(1.,1.),(1.,1.),(1.,1.),(1.,1.),(1.,1.),(1.,1.),(1.,1.),(1.,1.),(1.,
1.),(1.,1.),(1.,1.),(1.,1.),(1.,1.),(1.,1.),(1.,1.),(1.,1.),(1.,1.),(1.,
1.),(1.,1.),(1.,1.),(1.,1.),(1.,1.),(1.,1.),(1.,1.),(1.,1.),(1.,1.),(1.,
1.),(1.,1.),(1.,1.),(1.,1.),(1.,1.),(1.,1.),(1.,1.),(1.,1.),(1.,1.),(1.,
1.),(1.,1.),(1.,1.),(1.,1.),(1.,1.),(1.,1.),(1.,1.),(1.,1.),(1.,1.),(1.,
1.),(1.,1.),(1.,1.),(1.,1.),(1.,1.),(1.,1.),(1.,1.),(1.,1.),(1.,1.),(1.,
1.),(1.,1.)))
REPRESENTATION_ITEM('')
SURFACE()
);
#75=(
BOUNDED_SURFACE()
B_SPLINE_SURFACE(5,1,((#45272,#45273),(#45274,#45275),(#45276,#45277),(#45278,
#45279),(#45280,#45281),(#45282,#45283),(#45284,#45285),(#45286,#45287),
(#45288,#45289),(#45290,#45291),(#45292,#45293),(#45294,#45295),(#45296,
#45297),(#45298,#45299),(#45300,#45301),(#45302,#45303),(#45304,#45305),
(#45306,#45307),(#45308,#45309),(#45310,#45311),(#45312,#45313),(#45314,
#45315),(#45316,#45317),(#45318,#45319),(#45320,#45321),(#45322,#45323),
(#45324,#45325),(#45326,#45327),(#45328,#45329),(#45330,#45331),(#45332,
#45333),(#45334,#45335),(#45336,#45337),(#45338,#45339),(#45340,#45341),
(#45342,#45343),(#45344,#45345),(#45346,#45347),(#45348,#45349),(#45350,
#45351),(#45352,#45353),(#45354,#45355),(#45356,#45357),(#45358,#45359),
(#45360,#45361),(#45362,#45363),(#45364,#45365),(#45366,#45367),(#45368,
#45369),(#45370,#45371),(#45372,#45373),(#45374,#45375),(#45376,#45377),
(#45378,#45379),(#45380,#45381),(#45382,#45383),(#45384,#45385),(#45386,
#45387),(#45388,#45389),(#45390,#45391),(#45392,#45393),(#45394,#45395),
(#45396,#45397),(#45398,#45399),(#45400,#45401),(#45402,#45403),(#45404,
#45405),(#45406,#45407),(#45408,#45409),(#45410,#45411)),.UNSPECIFIED.,
 .F.,.F.,.F.)
B_SPLINE_SURFACE_WITH_KNOTS((6,1,1,1,1,1,1,1,1,1,1,1,1,1,1,1,1,1,1,1,1,
1,1,1,1,1,1,1,1,1,1,1,1,1,1,1,1,1,1,1,1,1,1,1,1,1,1,1,1,1,1,1,1,1,1,1,1,
1,1,1,1,1,1,1,1,6),(2,2),(-1.,-0.984615384615383,-0.969230769230768,-0.953846153846152,
-0.938461538461537,-0.923076923076922,-0.907692307692306,-0.892307692307691,
-0.876923076923076,-0.86153846153846,-0.846153846153845,-0.83076923076923,
-0.815384615384614,-0.799999999999999,-0.784615384615384,-0.769230769230768,
-0.753846153846153,-0.738461538461538,-0.723076923076922,-0.707692307692307,
-0.692307692307692,-0.676923076923076,-0.661538461538461,-0.646153846153846,
-0.63076923076923,-0.615384615384615,-0.6,-0.584615384615384,-0.569230769230769,
-0.553846153846154,-0.538461538461538,-0.523076923076923,-0.507692307692308,
-0.492307692307692,-0.476923076923077,-0.461538461538462,-0.446153846153846,
-0.430769230769231,-0.415384615384615,-0.4,-0.384615384615385,-0.369230769230769,
-0.353846153846154,-0.338461538461538,-0.323076923076923,-0.307692307692308,
-0.292307692307692,-0.276923076923077,-0.261538461538462,-0.246153846153846,
-0.230769230769231,-0.215384615384615,-0.2,-0.184615384615385,-0.169230769230769,
-0.153846153846154,-0.138461538461538,-0.123076923076923,-0.107692307692308,
-0.0923076923076923,-0.0769230769230769,-0.0615384615384615,-0.0461538461538462,
-0.0307692307692308,-0.0153846153846154,0.),(-1.,1.),.UNSPECIFIED.)
GEOMETRIC_REPRESENTATION_ITEM()
RATIONAL_B_SPLINE_SURFACE(((1.,1.),(1.,1.),(1.,1.),(1.,1.),(1.,1.),(1.,
1.),(1.,1.),(1.,1.),(1.,1.),(1.,1.),(1.,1.),(1.,1.),(1.,1.),(1.,1.),(1.,
1.),(1.,1.),(1.,1.),(1.,1.),(1.,1.),(1.,1.),(1.,1.),(1.,1.),(1.,1.),(1.,
1.),(1.,1.),(1.,1.),(1.,1.),(1.,1.),(1.,1.),(1.,1.),(1.,1.),(1.,1.),(1.,
1.),(1.,1.),(1.,1.),(1.,1.),(1.,1.),(1.,1.),(1.,1.),(1.,1.),(1.,1.),(1.,
1.),(1.,1.),(1.,1.),(1.,1.),(1.,1.),(1.,1.),(1.,1.),(1.,1.),(1.,1.),(1.,
1.),(1.,1.),(1.,1.),(1.,1.),(1.,1.),(1.,1.),(1.,1.),(1.,1.),(1.,1.),(1.,
1.),(1.,1.),(1.,1.),(1.,1.),(1.,1.),(1.,1.),(1.,1.),(1.,1.),(1.,1.),(1.,
1.),(1.,1.)))
REPRESENTATION_ITEM('')
SURFACE()
);
#76=(
BOUNDED_SURFACE()
B_SPLINE_SURFACE(5,1,((#45484,#45485),(#45486,#45487),(#45488,#45489),(#45490,
#45491),(#45492,#45493),(#45494,#45495),(#45496,#45497),(#45498,#45499),
(#45500,#45501),(#45502,#45503),(#45504,#45505),(#45506,#45507),(#45508,
#45509),(#45510,#45511),(#45512,#45513),(#45514,#45515),(#45516,#45517),
(#45518,#45519),(#45520,#45521),(#45522,#45523),(#45524,#45525),(#45526,
#45527),(#45528,#45529),(#45530,#45531),(#45532,#45533),(#45534,#45535),
(#45536,#45537),(#45538,#45539),(#45540,#45541),(#45542,#45543),(#45544,
#45545),(#45546,#45547),(#45548,#45549),(#45550,#45551),(#45552,#45553),
(#45554,#45555),(#45556,#45557),(#45558,#45559),(#45560,#45561),(#45562,
#45563),(#45564,#45565),(#45566,#45567),(#45568,#45569),(#45570,#45571),
(#45572,#45573),(#45574,#45575),(#45576,#45577),(#45578,#45579),(#45580,
#45581),(#45582,#45583),(#45584,#45585),(#45586,#45587),(#45588,#45589),
(#45590,#45591),(#45592,#45593),(#45594,#45595),(#45596,#45597),(#45598,
#45599),(#45600,#45601),(#45602,#45603),(#45604,#45605),(#45606,#45607),
(#45608,#45609),(#45610,#45611),(#45612,#45613),(#45614,#45615),(#45616,
#45617),(#45618,#45619),(#45620,#45621),(#45622,#45623)),.UNSPECIFIED.,
 .F.,.F.,.F.)
B_SPLINE_SURFACE_WITH_KNOTS((6,1,1,1,1,1,1,1,1,1,1,1,1,1,1,1,1,1,1,1,1,
1,1,1,1,1,1,1,1,1,1,1,1,1,1,1,1,1,1,1,1,1,1,1,1,1,1,1,1,1,1,1,1,1,1,1,1,
1,1,1,1,1,1,1,1,6),(2,2),(-1.,-0.984615384615383,-0.969230769230768,-0.953846153846152,
-0.938461538461537,-0.923076923076922,-0.907692307692306,-0.892307692307691,
-0.876923076923076,-0.86153846153846,-0.846153846153845,-0.83076923076923,
-0.815384615384614,-0.799999999999999,-0.784615384615384,-0.769230769230768,
-0.753846153846153,-0.738461538461538,-0.723076923076922,-0.707692307692307,
-0.692307692307692,-0.676923076923076,-0.661538461538461,-0.646153846153846,
-0.63076923076923,-0.615384615384615,-0.6,-0.584615384615384,-0.569230769230769,
-0.553846153846154,-0.538461538461538,-0.523076923076923,-0.507692307692308,
-0.492307692307692,-0.476923076923077,-0.461538461538462,-0.446153846153846,
-0.430769230769231,-0.415384615384615,-0.4,-0.384615384615385,-0.369230769230769,
-0.353846153846154,-0.338461538461538,-0.323076923076923,-0.307692307692308,
-0.292307692307692,-0.276923076923077,-0.261538461538462,-0.246153846153846,
-0.230769230769231,-0.215384615384615,-0.2,-0.184615384615385,-0.169230769230769,
-0.153846153846154,-0.138461538461538,-0.123076923076923,-0.107692307692308,
-0.0923076923076923,-0.0769230769230769,-0.0615384615384615,-0.0461538461538462,
-0.0307692307692308,-0.0153846153846154,0.),(-1.,1.),.UNSPECIFIED.)
GEOMETRIC_REPRESENTATION_ITEM()
RATIONAL_B_SPLINE_SURFACE(((1.,1.),(1.,1.),(1.,1.),(1.,1.),(1.,1.),(1.,
1.),(1.,1.),(1.,1.),(1.,1.),(1.,1.),(1.,1.),(1.,1.),(1.,1.),(1.,1.),(1.,
1.),(1.,1.),(1.,1.),(1.,1.),(1.,1.),(1.,1.),(1.,1.),(1.,1.),(1.,1.),(1.,
1.),(1.,1.),(1.,1.),(1.,1.),(1.,1.),(1.,1.),(1.,1.),(1.,1.),(1.,1.),(1.,
1.),(1.,1.),(1.,1.),(1.,1.),(1.,1.),(1.,1.),(1.,1.),(1.,1.),(1.,1.),(1.,
1.),(1.,1.),(1.,1.),(1.,1.),(1.,1.),(1.,1.),(1.,1.),(1.,1.),(1.,1.),(1.,
1.),(1.,1.),(1.,1.),(1.,1.),(1.,1.),(1.,1.),(1.,1.),(1.,1.),(1.,1.),(1.,
1.),(1.,1.),(1.,1.),(1.,1.),(1.,1.),(1.,1.),(1.,1.),(1.,1.),(1.,1.),(1.,
1.),(1.,1.)))
REPRESENTATION_ITEM('')
SURFACE()
);
#77=(
BOUNDED_SURFACE()
B_SPLINE_SURFACE(5,1,((#45714,#45715),(#45716,#45717),(#45718,#45719),(#45720,
#45721),(#45722,#45723),(#45724,#45725),(#45726,#45727),(#45728,#45729),
(#45730,#45731),(#45732,#45733),(#45734,#45735),(#45736,#45737),(#45738,
#45739),(#45740,#45741),(#45742,#45743),(#45744,#45745),(#45746,#45747),
(#45748,#45749),(#45750,#45751),(#45752,#45753),(#45754,#45755),(#45756,
#45757),(#45758,#45759),(#45760,#45761),(#45762,#45763),(#45764,#45765),
(#45766,#45767),(#45768,#45769),(#45770,#45771),(#45772,#45773),(#45774,
#45775),(#45776,#45777),(#45778,#45779),(#45780,#45781),(#45782,#45783),
(#45784,#45785),(#45786,#45787),(#45788,#45789),(#45790,#45791),(#45792,
#45793),(#45794,#45795),(#45796,#45797),(#45798,#45799),(#45800,#45801),
(#45802,#45803),(#45804,#45805),(#45806,#45807),(#45808,#45809),(#45810,
#45811),(#45812,#45813),(#45814,#45815),(#45816,#45817),(#45818,#45819),
(#45820,#45821),(#45822,#45823),(#45824,#45825),(#45826,#45827),(#45828,
#45829),(#45830,#45831),(#45832,#45833),(#45834,#45835),(#45836,#45837),
(#45838,#45839),(#45840,#45841),(#45842,#45843),(#45844,#45845),(#45846,
#45847),(#45848,#45849),(#45850,#45851),(#45852,#45853)),.UNSPECIFIED.,
 .F.,.F.,.F.)
B_SPLINE_SURFACE_WITH_KNOTS((6,1,1,1,1,1,1,1,1,1,1,1,1,1,1,1,1,1,1,1,1,
1,1,1,1,1,1,1,1,1,1,1,1,1,1,1,1,1,1,1,1,1,1,1,1,1,1,1,1,1,1,1,1,1,1,1,1,
1,1,1,1,1,1,1,1,6),(2,2),(-1.,-0.984615384615383,-0.969230769230768,-0.953846153846152,
-0.938461538461537,-0.923076923076922,-0.907692307692306,-0.892307692307691,
-0.876923076923076,-0.86153846153846,-0.846153846153845,-0.83076923076923,
-0.815384615384614,-0.799999999999999,-0.784615384615384,-0.769230769230768,
-0.753846153846153,-0.738461538461538,-0.723076923076922,-0.707692307692307,
-0.692307692307692,-0.676923076923076,-0.661538461538461,-0.646153846153846,
-0.63076923076923,-0.615384615384615,-0.6,-0.584615384615384,-0.569230769230769,
-0.553846153846154,-0.538461538461538,-0.523076923076923,-0.507692307692308,
-0.492307692307692,-0.476923076923077,-0.461538461538462,-0.446153846153846,
-0.430769230769231,-0.415384615384615,-0.4,-0.384615384615385,-0.369230769230769,
-0.353846153846154,-0.338461538461538,-0.323076923076923,-0.307692307692308,
-0.292307692307692,-0.276923076923077,-0.261538461538462,-0.246153846153846,
-0.230769230769231,-0.215384615384615,-0.2,-0.184615384615385,-0.169230769230769,
-0.153846153846154,-0.138461538461538,-0.123076923076923,-0.107692307692308,
-0.0923076923076923,-0.0769230769230769,-0.0615384615384615,-0.0461538461538462,
-0.0307692307692308,-0.0153846153846154,0.),(-1.,1.),.UNSPECIFIED.)
GEOMETRIC_REPRESENTATION_ITEM()
RATIONAL_B_SPLINE_SURFACE(((1.,1.),(1.,1.),(1.,1.),(1.,1.),(1.,1.),(1.,
1.),(1.,1.),(1.,1.),(1.,1.),(1.,1.),(1.,1.),(1.,1.),(1.,1.),(1.,1.),(1.,
1.),(1.,1.),(1.,1.),(1.,1.),(1.,1.),(1.,1.),(1.,1.),(1.,1.),(1.,1.),(1.,
1.),(1.,1.),(1.,1.),(1.,1.),(1.,1.),(1.,1.),(1.,1.),(1.,1.),(1.,1.),(1.,
1.),(1.,1.),(1.,1.),(1.,1.),(1.,1.),(1.,1.),(1.,1.),(1.,1.),(1.,1.),(1.,
1.),(1.,1.),(1.,1.),(1.,1.),(1.,1.),(1.,1.),(1.,1.),(1.,1.),(1.,1.),(1.,
1.),(1.,1.),(1.,1.),(1.,1.),(1.,1.),(1.,1.),(1.,1.),(1.,1.),(1.,1.),(1.,
1.),(1.,1.),(1.,1.),(1.,1.),(1.,1.),(1.,1.),(1.,1.),(1.,1.),(1.,1.),(1.,
1.),(1.,1.)))
REPRESENTATION_ITEM('')
SURFACE()
);
#78=(
BOUNDED_SURFACE()
B_SPLINE_SURFACE(5,1,((#45926,#45927),(#45928,#45929),(#45930,#45931),(#45932,
#45933),(#45934,#45935),(#45936,#45937),(#45938,#45939),(#45940,#45941),
(#45942,#45943),(#45944,#45945),(#45946,#45947),(#45948,#45949),(#45950,
#45951),(#45952,#45953),(#45954,#45955),(#45956,#45957),(#45958,#45959),
(#45960,#45961),(#45962,#45963),(#45964,#45965),(#45966,#45967),(#45968,
#45969),(#45970,#45971),(#45972,#45973),(#45974,#45975),(#45976,#45977),
(#45978,#45979),(#45980,#45981),(#45982,#45983),(#45984,#45985),(#45986,
#45987),(#45988,#45989),(#45990,#45991),(#45992,#45993),(#45994,#45995),
(#45996,#45997),(#45998,#45999),(#46000,#46001),(#46002,#46003),(#46004,
#46005),(#46006,#46007),(#46008,#46009),(#46010,#46011),(#46012,#46013),
(#46014,#46015),(#46016,#46017),(#46018,#46019),(#46020,#46021),(#46022,
#46023),(#46024,#46025),(#46026,#46027),(#46028,#46029),(#46030,#46031),
(#46032,#46033),(#46034,#46035),(#46036,#46037),(#46038,#46039),(#46040,
#46041),(#46042,#46043),(#46044,#46045),(#46046,#46047),(#46048,#46049),
(#46050,#46051),(#46052,#46053),(#46054,#46055),(#46056,#46057),(#46058,
#46059),(#46060,#46061),(#46062,#46063),(#46064,#46065)),.UNSPECIFIED.,
 .F.,.F.,.F.)
B_SPLINE_SURFACE_WITH_KNOTS((6,1,1,1,1,1,1,1,1,1,1,1,1,1,1,1,1,1,1,1,1,
1,1,1,1,1,1,1,1,1,1,1,1,1,1,1,1,1,1,1,1,1,1,1,1,1,1,1,1,1,1,1,1,1,1,1,1,
1,1,1,1,1,1,1,1,6),(2,2),(-1.,-0.984615384615383,-0.969230769230768,-0.953846153846152,
-0.938461538461537,-0.923076923076922,-0.907692307692306,-0.892307692307691,
-0.876923076923076,-0.86153846153846,-0.846153846153845,-0.83076923076923,
-0.815384615384614,-0.799999999999999,-0.784615384615384,-0.769230769230768,
-0.753846153846153,-0.738461538461538,-0.723076923076922,-0.707692307692307,
-0.692307692307692,-0.676923076923076,-0.661538461538461,-0.646153846153846,
-0.63076923076923,-0.615384615384615,-0.6,-0.584615384615384,-0.569230769230769,
-0.553846153846154,-0.538461538461538,-0.523076923076923,-0.507692307692308,
-0.492307692307692,-0.476923076923077,-0.461538461538462,-0.446153846153846,
-0.430769230769231,-0.415384615384615,-0.4,-0.384615384615385,-0.369230769230769,
-0.353846153846154,-0.338461538461538,-0.323076923076923,-0.307692307692308,
-0.292307692307692,-0.276923076923077,-0.261538461538462,-0.246153846153846,
-0.230769230769231,-0.215384615384615,-0.2,-0.184615384615385,-0.169230769230769,
-0.153846153846154,-0.138461538461538,-0.123076923076923,-0.107692307692308,
-0.0923076923076923,-0.0769230769230769,-0.0615384615384615,-0.0461538461538462,
-0.0307692307692308,-0.0153846153846154,0.),(-1.,1.),.UNSPECIFIED.)
GEOMETRIC_REPRESENTATION_ITEM()
RATIONAL_B_SPLINE_SURFACE(((1.,1.),(1.,1.),(1.,1.),(1.,1.),(1.,1.),(1.,
1.),(1.,1.),(1.,1.),(1.,1.),(1.,1.),(1.,1.),(1.,1.),(1.,1.),(1.,1.),(1.,
1.),(1.,1.),(1.,1.),(1.,1.),(1.,1.),(1.,1.),(1.,1.),(1.,1.),(1.,1.),(1.,
1.),(1.,1.),(1.,1.),(1.,1.),(1.,1.),(1.,1.),(1.,1.),(1.,1.),(1.,1.),(1.,
1.),(1.,1.),(1.,1.),(1.,1.),(1.,1.),(1.,1.),(1.,1.),(1.,1.),(1.,1.),(1.,
1.),(1.,1.),(1.,1.),(1.,1.),(1.,1.),(1.,1.),(1.,1.),(1.,1.),(1.,1.),(1.,
1.),(1.,1.),(1.,1.),(1.,1.),(1.,1.),(1.,1.),(1.,1.),(1.,1.),(1.,1.),(1.,
1.),(1.,1.),(1.,1.),(1.,1.),(1.,1.),(1.,1.),(1.,1.),(1.,1.),(1.,1.),(1.,
1.),(1.,1.)))
REPRESENTATION_ITEM('')
SURFACE()
);
#79=(
BOUNDED_SURFACE()
B_SPLINE_SURFACE(5,1,((#46156,#46157),(#46158,#46159),(#46160,#46161),(#46162,
#46163),(#46164,#46165),(#46166,#46167),(#46168,#46169),(#46170,#46171),
(#46172,#46173),(#46174,#46175),(#46176,#46177),(#46178,#46179),(#46180,
#46181),(#46182,#46183),(#46184,#46185),(#46186,#46187),(#46188,#46189),
(#46190,#46191),(#46192,#46193),(#46194,#46195),(#46196,#46197),(#46198,
#46199),(#46200,#46201),(#46202,#46203),(#46204,#46205),(#46206,#46207),
(#46208,#46209),(#46210,#46211),(#46212,#46213),(#46214,#46215),(#46216,
#46217),(#46218,#46219),(#46220,#46221),(#46222,#46223),(#46224,#46225),
(#46226,#46227),(#46228,#46229),(#46230,#46231),(#46232,#46233),(#46234,
#46235),(#46236,#46237),(#46238,#46239),(#46240,#46241),(#46242,#46243),
(#46244,#46245),(#46246,#46247),(#46248,#46249),(#46250,#46251),(#46252,
#46253),(#46254,#46255),(#46256,#46257),(#46258,#46259),(#46260,#46261),
(#46262,#46263),(#46264,#46265),(#46266,#46267),(#46268,#46269),(#46270,
#46271),(#46272,#46273),(#46274,#46275),(#46276,#46277),(#46278,#46279),
(#46280,#46281),(#46282,#46283),(#46284,#46285),(#46286,#46287),(#46288,
#46289),(#46290,#46291),(#46292,#46293),(#46294,#46295)),.UNSPECIFIED.,
 .F.,.F.,.F.)
B_SPLINE_SURFACE_WITH_KNOTS((6,1,1,1,1,1,1,1,1,1,1,1,1,1,1,1,1,1,1,1,1,
1,1,1,1,1,1,1,1,1,1,1,1,1,1,1,1,1,1,1,1,1,1,1,1,1,1,1,1,1,1,1,1,1,1,1,1,
1,1,1,1,1,1,1,1,6),(2,2),(-1.,-0.984615384615383,-0.969230769230768,-0.953846153846152,
-0.938461538461537,-0.923076923076922,-0.907692307692306,-0.892307692307691,
-0.876923076923076,-0.86153846153846,-0.846153846153845,-0.83076923076923,
-0.815384615384614,-0.799999999999999,-0.784615384615384,-0.769230769230768,
-0.753846153846153,-0.738461538461538,-0.723076923076922,-0.707692307692307,
-0.692307692307692,-0.676923076923076,-0.661538461538461,-0.646153846153846,
-0.63076923076923,-0.615384615384615,-0.6,-0.584615384615384,-0.569230769230769,
-0.553846153846154,-0.538461538461538,-0.523076923076923,-0.507692307692308,
-0.492307692307692,-0.476923076923077,-0.461538461538462,-0.446153846153846,
-0.430769230769231,-0.415384615384615,-0.4,-0.384615384615385,-0.369230769230769,
-0.353846153846154,-0.338461538461538,-0.323076923076923,-0.307692307692308,
-0.292307692307692,-0.276923076923077,-0.261538461538462,-0.246153846153846,
-0.230769230769231,-0.215384615384615,-0.2,-0.184615384615385,-0.169230769230769,
-0.153846153846154,-0.138461538461538,-0.123076923076923,-0.107692307692308,
-0.0923076923076923,-0.0769230769230769,-0.0615384615384615,-0.0461538461538462,
-0.0307692307692308,-0.0153846153846154,0.),(-1.,1.),.UNSPECIFIED.)
GEOMETRIC_REPRESENTATION_ITEM()
RATIONAL_B_SPLINE_SURFACE(((1.,1.),(1.,1.),(1.,1.),(1.,1.),(1.,1.),(1.,
1.),(1.,1.),(1.,1.),(1.,1.),(1.,1.),(1.,1.),(1.,1.),(1.,1.),(1.,1.),(1.,
1.),(1.,1.),(1.,1.),(1.,1.),(1.,1.),(1.,1.),(1.,1.),(1.,1.),(1.,1.),(1.,
1.),(1.,1.),(1.,1.),(1.,1.),(1.,1.),(1.,1.),(1.,1.),(1.,1.),(1.,1.),(1.,
1.),(1.,1.),(1.,1.),(1.,1.),(1.,1.),(1.,1.),(1.,1.),(1.,1.),(1.,1.),(1.,
1.),(1.,1.),(1.,1.),(1.,1.),(1.,1.),(1.,1.),(1.,1.),(1.,1.),(1.,1.),(1.,
1.),(1.,1.),(1.,1.),(1.,1.),(1.,1.),(1.,1.),(1.,1.),(1.,1.),(1.,1.),(1.,
1.),(1.,1.),(1.,1.),(1.,1.),(1.,1.),(1.,1.),(1.,1.),(1.,1.),(1.,1.),(1.,
1.),(1.,1.)))
REPRESENTATION_ITEM('')
SURFACE()
);
#80=(
BOUNDED_SURFACE()
B_SPLINE_SURFACE(5,1,((#46368,#46369),(#46370,#46371),(#46372,#46373),(#46374,
#46375),(#46376,#46377),(#46378,#46379),(#46380,#46381),(#46382,#46383),
(#46384,#46385),(#46386,#46387),(#46388,#46389),(#46390,#46391),(#46392,
#46393),(#46394,#46395),(#46396,#46397),(#46398,#46399),(#46400,#46401),
(#46402,#46403),(#46404,#46405),(#46406,#46407),(#46408,#46409),(#46410,
#46411),(#46412,#46413),(#46414,#46415),(#46416,#46417),(#46418,#46419),
(#46420,#46421),(#46422,#46423),(#46424,#46425),(#46426,#46427),(#46428,
#46429),(#46430,#46431),(#46432,#46433),(#46434,#46435),(#46436,#46437),
(#46438,#46439),(#46440,#46441),(#46442,#46443),(#46444,#46445),(#46446,
#46447),(#46448,#46449),(#46450,#46451),(#46452,#46453),(#46454,#46455),
(#46456,#46457),(#46458,#46459),(#46460,#46461),(#46462,#46463),(#46464,
#46465),(#46466,#46467),(#46468,#46469),(#46470,#46471),(#46472,#46473),
(#46474,#46475),(#46476,#46477),(#46478,#46479),(#46480,#46481),(#46482,
#46483),(#46484,#46485),(#46486,#46487),(#46488,#46489),(#46490,#46491),
(#46492,#46493),(#46494,#46495),(#46496,#46497),(#46498,#46499),(#46500,
#46501),(#46502,#46503),(#46504,#46505),(#46506,#46507)),.UNSPECIFIED.,
 .F.,.F.,.F.)
B_SPLINE_SURFACE_WITH_KNOTS((6,1,1,1,1,1,1,1,1,1,1,1,1,1,1,1,1,1,1,1,1,
1,1,1,1,1,1,1,1,1,1,1,1,1,1,1,1,1,1,1,1,1,1,1,1,1,1,1,1,1,1,1,1,1,1,1,1,
1,1,1,1,1,1,1,1,6),(2,2),(-1.,-0.984615384615383,-0.969230769230768,-0.953846153846152,
-0.938461538461537,-0.923076923076922,-0.907692307692306,-0.892307692307691,
-0.876923076923076,-0.86153846153846,-0.846153846153845,-0.83076923076923,
-0.815384615384614,-0.799999999999999,-0.784615384615384,-0.769230769230768,
-0.753846153846153,-0.738461538461538,-0.723076923076922,-0.707692307692307,
-0.692307692307692,-0.676923076923076,-0.661538461538461,-0.646153846153846,
-0.63076923076923,-0.615384615384615,-0.6,-0.584615384615384,-0.569230769230769,
-0.553846153846154,-0.538461538461538,-0.523076923076923,-0.507692307692308,
-0.492307692307692,-0.476923076923077,-0.461538461538462,-0.446153846153846,
-0.430769230769231,-0.415384615384615,-0.4,-0.384615384615385,-0.369230769230769,
-0.353846153846154,-0.338461538461538,-0.323076923076923,-0.307692307692308,
-0.292307692307692,-0.276923076923077,-0.261538461538462,-0.246153846153846,
-0.230769230769231,-0.215384615384615,-0.2,-0.184615384615385,-0.169230769230769,
-0.153846153846154,-0.138461538461538,-0.123076923076923,-0.107692307692308,
-0.0923076923076923,-0.0769230769230769,-0.0615384615384615,-0.0461538461538462,
-0.0307692307692308,-0.0153846153846154,0.),(-1.,1.),.UNSPECIFIED.)
GEOMETRIC_REPRESENTATION_ITEM()
RATIONAL_B_SPLINE_SURFACE(((1.,1.),(1.,1.),(1.,1.),(1.,1.),(1.,1.),(1.,
1.),(1.,1.),(1.,1.),(1.,1.),(1.,1.),(1.,1.),(1.,1.),(1.,1.),(1.,1.),(1.,
1.),(1.,1.),(1.,1.),(1.,1.),(1.,1.),(1.,1.),(1.,1.),(1.,1.),(1.,1.),(1.,
1.),(1.,1.),(1.,1.),(1.,1.),(1.,1.),(1.,1.),(1.,1.),(1.,1.),(1.,1.),(1.,
1.),(1.,1.),(1.,1.),(1.,1.),(1.,1.),(1.,1.),(1.,1.),(1.,1.),(1.,1.),(1.,
1.),(1.,1.),(1.,1.),(1.,1.),(1.,1.),(1.,1.),(1.,1.),(1.,1.),(1.,1.),(1.,
1.),(1.,1.),(1.,1.),(1.,1.),(1.,1.),(1.,1.),(1.,1.),(1.,1.),(1.,1.),(1.,
1.),(1.,1.),(1.,1.),(1.,1.),(1.,1.),(1.,1.),(1.,1.),(1.,1.),(1.,1.),(1.,
1.),(1.,1.)))
REPRESENTATION_ITEM('')
SURFACE()
);
#81=(
BOUNDED_SURFACE()
B_SPLINE_SURFACE(5,1,((#46598,#46599),(#46600,#46601),(#46602,#46603),(#46604,
#46605),(#46606,#46607),(#46608,#46609),(#46610,#46611),(#46612,#46613),
(#46614,#46615),(#46616,#46617),(#46618,#46619),(#46620,#46621),(#46622,
#46623),(#46624,#46625),(#46626,#46627),(#46628,#46629),(#46630,#46631),
(#46632,#46633),(#46634,#46635),(#46636,#46637),(#46638,#46639),(#46640,
#46641),(#46642,#46643),(#46644,#46645),(#46646,#46647),(#46648,#46649),
(#46650,#46651),(#46652,#46653),(#46654,#46655),(#46656,#46657),(#46658,
#46659),(#46660,#46661),(#46662,#46663),(#46664,#46665),(#46666,#46667),
(#46668,#46669),(#46670,#46671),(#46672,#46673),(#46674,#46675),(#46676,
#46677),(#46678,#46679),(#46680,#46681),(#46682,#46683),(#46684,#46685),
(#46686,#46687),(#46688,#46689),(#46690,#46691),(#46692,#46693),(#46694,
#46695),(#46696,#46697),(#46698,#46699),(#46700,#46701),(#46702,#46703),
(#46704,#46705),(#46706,#46707),(#46708,#46709),(#46710,#46711),(#46712,
#46713),(#46714,#46715),(#46716,#46717),(#46718,#46719),(#46720,#46721),
(#46722,#46723),(#46724,#46725),(#46726,#46727),(#46728,#46729),(#46730,
#46731),(#46732,#46733),(#46734,#46735),(#46736,#46737)),.UNSPECIFIED.,
 .F.,.F.,.F.)
B_SPLINE_SURFACE_WITH_KNOTS((6,1,1,1,1,1,1,1,1,1,1,1,1,1,1,1,1,1,1,1,1,
1,1,1,1,1,1,1,1,1,1,1,1,1,1,1,1,1,1,1,1,1,1,1,1,1,1,1,1,1,1,1,1,1,1,1,1,
1,1,1,1,1,1,1,1,6),(2,2),(-1.,-0.984615384615383,-0.969230769230768,-0.953846153846152,
-0.938461538461537,-0.923076923076922,-0.907692307692306,-0.892307692307691,
-0.876923076923076,-0.86153846153846,-0.846153846153845,-0.83076923076923,
-0.815384615384614,-0.799999999999999,-0.784615384615384,-0.769230769230768,
-0.753846153846153,-0.738461538461538,-0.723076923076922,-0.707692307692307,
-0.692307692307692,-0.676923076923076,-0.661538461538461,-0.646153846153846,
-0.63076923076923,-0.615384615384615,-0.6,-0.584615384615384,-0.569230769230769,
-0.553846153846154,-0.538461538461538,-0.523076923076923,-0.507692307692308,
-0.492307692307692,-0.476923076923077,-0.461538461538462,-0.446153846153846,
-0.430769230769231,-0.415384615384615,-0.4,-0.384615384615385,-0.369230769230769,
-0.353846153846154,-0.338461538461538,-0.323076923076923,-0.307692307692308,
-0.292307692307692,-0.276923076923077,-0.261538461538462,-0.246153846153846,
-0.230769230769231,-0.215384615384615,-0.2,-0.184615384615385,-0.169230769230769,
-0.153846153846154,-0.138461538461538,-0.123076923076923,-0.107692307692308,
-0.0923076923076923,-0.0769230769230769,-0.0615384615384615,-0.0461538461538462,
-0.0307692307692308,-0.0153846153846154,0.),(-1.,1.),.UNSPECIFIED.)
GEOMETRIC_REPRESENTATION_ITEM()
RATIONAL_B_SPLINE_SURFACE(((1.,1.),(1.,1.),(1.,1.),(1.,1.),(1.,1.),(1.,
1.),(1.,1.),(1.,1.),(1.,1.),(1.,1.),(1.,1.),(1.,1.),(1.,1.),(1.,1.),(1.,
1.),(1.,1.),(1.,1.),(1.,1.),(1.,1.),(1.,1.),(1.,1.),(1.,1.),(1.,1.),(1.,
1.),(1.,1.),(1.,1.),(1.,1.),(1.,1.),(1.,1.),(1.,1.),(1.,1.),(1.,1.),(1.,
1.),(1.,1.),(1.,1.),(1.,1.),(1.,1.),(1.,1.),(1.,1.),(1.,1.),(1.,1.),(1.,
1.),(1.,1.),(1.,1.),(1.,1.),(1.,1.),(1.,1.),(1.,1.),(1.,1.),(1.,1.),(1.,
1.),(1.,1.),(1.,1.),(1.,1.),(1.,1.),(1.,1.),(1.,1.),(1.,1.),(1.,1.),(1.,
1.),(1.,1.),(1.,1.),(1.,1.),(1.,1.),(1.,1.),(1.,1.),(1.,1.),(1.,1.),(1.,
1.),(1.,1.)))
REPRESENTATION_ITEM('')
SURFACE()
);
#82=(
BOUNDED_SURFACE()
B_SPLINE_SURFACE(5,1,((#46810,#46811),(#46812,#46813),(#46814,#46815),(#46816,
#46817),(#46818,#46819),(#46820,#46821),(#46822,#46823),(#46824,#46825),
(#46826,#46827),(#46828,#46829),(#46830,#46831),(#46832,#46833),(#46834,
#46835),(#46836,#46837),(#46838,#46839),(#46840,#46841),(#46842,#46843),
(#46844,#46845),(#46846,#46847),(#46848,#46849),(#46850,#46851),(#46852,
#46853),(#46854,#46855),(#46856,#46857),(#46858,#46859),(#46860,#46861),
(#46862,#46863),(#46864,#46865),(#46866,#46867),(#46868,#46869),(#46870,
#46871),(#46872,#46873),(#46874,#46875),(#46876,#46877),(#46878,#46879),
(#46880,#46881),(#46882,#46883),(#46884,#46885),(#46886,#46887),(#46888,
#46889),(#46890,#46891),(#46892,#46893),(#46894,#46895),(#46896,#46897),
(#46898,#46899),(#46900,#46901),(#46902,#46903),(#46904,#46905),(#46906,
#46907),(#46908,#46909),(#46910,#46911),(#46912,#46913),(#46914,#46915),
(#46916,#46917),(#46918,#46919),(#46920,#46921),(#46922,#46923),(#46924,
#46925),(#46926,#46927),(#46928,#46929),(#46930,#46931),(#46932,#46933),
(#46934,#46935),(#46936,#46937),(#46938,#46939),(#46940,#46941),(#46942,
#46943),(#46944,#46945),(#46946,#46947),(#46948,#46949)),.UNSPECIFIED.,
 .F.,.F.,.F.)
B_SPLINE_SURFACE_WITH_KNOTS((6,1,1,1,1,1,1,1,1,1,1,1,1,1,1,1,1,1,1,1,1,
1,1,1,1,1,1,1,1,1,1,1,1,1,1,1,1,1,1,1,1,1,1,1,1,1,1,1,1,1,1,1,1,1,1,1,1,
1,1,1,1,1,1,1,1,6),(2,2),(-1.,-0.984615384615383,-0.969230769230768,-0.953846153846152,
-0.938461538461537,-0.923076923076922,-0.907692307692306,-0.892307692307691,
-0.876923076923076,-0.86153846153846,-0.846153846153845,-0.83076923076923,
-0.815384615384614,-0.799999999999999,-0.784615384615384,-0.769230769230768,
-0.753846153846153,-0.738461538461538,-0.723076923076922,-0.707692307692307,
-0.692307692307692,-0.676923076923076,-0.661538461538461,-0.646153846153846,
-0.63076923076923,-0.615384615384615,-0.6,-0.584615384615384,-0.569230769230769,
-0.553846153846154,-0.538461538461538,-0.523076923076923,-0.507692307692308,
-0.492307692307692,-0.476923076923077,-0.461538461538462,-0.446153846153846,
-0.430769230769231,-0.415384615384615,-0.4,-0.384615384615385,-0.369230769230769,
-0.353846153846154,-0.338461538461538,-0.323076923076923,-0.307692307692308,
-0.292307692307692,-0.276923076923077,-0.261538461538462,-0.246153846153846,
-0.230769230769231,-0.215384615384615,-0.2,-0.184615384615385,-0.169230769230769,
-0.153846153846154,-0.138461538461538,-0.123076923076923,-0.107692307692308,
-0.0923076923076923,-0.0769230769230769,-0.0615384615384615,-0.0461538461538462,
-0.0307692307692308,-0.0153846153846154,0.),(-1.,1.),.UNSPECIFIED.)
GEOMETRIC_REPRESENTATION_ITEM()
RATIONAL_B_SPLINE_SURFACE(((1.,1.),(1.,1.),(1.,1.),(1.,1.),(1.,1.),(1.,
1.),(1.,1.),(1.,1.),(1.,1.),(1.,1.),(1.,1.),(1.,1.),(1.,1.),(1.,1.),(1.,
1.),(1.,1.),(1.,1.),(1.,1.),(1.,1.),(1.,1.),(1.,1.),(1.,1.),(1.,1.),(1.,
1.),(1.,1.),(1.,1.),(1.,1.),(1.,1.),(1.,1.),(1.,1.),(1.,1.),(1.,1.),(1.,
1.),(1.,1.),(1.,1.),(1.,1.),(1.,1.),(1.,1.),(1.,1.),(1.,1.),(1.,1.),(1.,
1.),(1.,1.),(1.,1.),(1.,1.),(1.,1.),(1.,1.),(1.,1.),(1.,1.),(1.,1.),(1.,
1.),(1.,1.),(1.,1.),(1.,1.),(1.,1.),(1.,1.),(1.,1.),(1.,1.),(1.,1.),(1.,
1.),(1.,1.),(1.,1.),(1.,1.),(1.,1.),(1.,1.),(1.,1.),(1.,1.),(1.,1.),(1.,
1.),(1.,1.)))
REPRESENTATION_ITEM('')
SURFACE()
);
#83=(
BOUNDED_SURFACE()
B_SPLINE_SURFACE(5,1,((#47040,#47041),(#47042,#47043),(#47044,#47045),(#47046,
#47047),(#47048,#47049),(#47050,#47051),(#47052,#47053),(#47054,#47055),
(#47056,#47057),(#47058,#47059),(#47060,#47061),(#47062,#47063),(#47064,
#47065),(#47066,#47067),(#47068,#47069),(#47070,#47071),(#47072,#47073),
(#47074,#47075),(#47076,#47077),(#47078,#47079),(#47080,#47081),(#47082,
#47083),(#47084,#47085),(#47086,#47087),(#47088,#47089),(#47090,#47091),
(#47092,#47093),(#47094,#47095),(#47096,#47097),(#47098,#47099),(#47100,
#47101),(#47102,#47103),(#47104,#47105),(#47106,#47107),(#47108,#47109),
(#47110,#47111),(#47112,#47113),(#47114,#47115),(#47116,#47117),(#47118,
#47119),(#47120,#47121),(#47122,#47123),(#47124,#47125),(#47126,#47127),
(#47128,#47129),(#47130,#47131),(#47132,#47133),(#47134,#47135),(#47136,
#47137),(#47138,#47139),(#47140,#47141),(#47142,#47143),(#47144,#47145),
(#47146,#47147),(#47148,#47149),(#47150,#47151),(#47152,#47153),(#47154,
#47155),(#47156,#47157),(#47158,#47159),(#47160,#47161),(#47162,#47163),
(#47164,#47165),(#47166,#47167),(#47168,#47169),(#47170,#47171),(#47172,
#47173),(#47174,#47175),(#47176,#47177),(#47178,#47179)),.UNSPECIFIED.,
 .F.,.F.,.F.)
B_SPLINE_SURFACE_WITH_KNOTS((6,1,1,1,1,1,1,1,1,1,1,1,1,1,1,1,1,1,1,1,1,
1,1,1,1,1,1,1,1,1,1,1,1,1,1,1,1,1,1,1,1,1,1,1,1,1,1,1,1,1,1,1,1,1,1,1,1,
1,1,1,1,1,1,1,1,6),(2,2),(-1.,-0.984615384615383,-0.969230769230768,-0.953846153846152,
-0.938461538461537,-0.923076923076922,-0.907692307692306,-0.892307692307691,
-0.876923076923076,-0.86153846153846,-0.846153846153845,-0.83076923076923,
-0.815384615384614,-0.799999999999999,-0.784615384615384,-0.769230769230768,
-0.753846153846153,-0.738461538461538,-0.723076923076922,-0.707692307692307,
-0.692307692307692,-0.676923076923076,-0.661538461538461,-0.646153846153846,
-0.63076923076923,-0.615384615384615,-0.6,-0.584615384615384,-0.569230769230769,
-0.553846153846154,-0.538461538461538,-0.523076923076923,-0.507692307692308,
-0.492307692307692,-0.476923076923077,-0.461538461538462,-0.446153846153846,
-0.430769230769231,-0.415384615384615,-0.4,-0.384615384615385,-0.369230769230769,
-0.353846153846154,-0.338461538461538,-0.323076923076923,-0.307692307692308,
-0.292307692307692,-0.276923076923077,-0.261538461538462,-0.246153846153846,
-0.230769230769231,-0.215384615384615,-0.2,-0.184615384615385,-0.169230769230769,
-0.153846153846154,-0.138461538461538,-0.123076923076923,-0.107692307692308,
-0.0923076923076923,-0.0769230769230769,-0.0615384615384615,-0.0461538461538462,
-0.0307692307692308,-0.0153846153846154,0.),(-1.,1.),.UNSPECIFIED.)
GEOMETRIC_REPRESENTATION_ITEM()
RATIONAL_B_SPLINE_SURFACE(((1.,1.),(1.,1.),(1.,1.),(1.,1.),(1.,1.),(1.,
1.),(1.,1.),(1.,1.),(1.,1.),(1.,1.),(1.,1.),(1.,1.),(1.,1.),(1.,1.),(1.,
1.),(1.,1.),(1.,1.),(1.,1.),(1.,1.),(1.,1.),(1.,1.),(1.,1.),(1.,1.),(1.,
1.),(1.,1.),(1.,1.),(1.,1.),(1.,1.),(1.,1.),(1.,1.),(1.,1.),(1.,1.),(1.,
1.),(1.,1.),(1.,1.),(1.,1.),(1.,1.),(1.,1.),(1.,1.),(1.,1.),(1.,1.),(1.,
1.),(1.,1.),(1.,1.),(1.,1.),(1.,1.),(1.,1.),(1.,1.),(1.,1.),(1.,1.),(1.,
1.),(1.,1.),(1.,1.),(1.,1.),(1.,1.),(1.,1.),(1.,1.),(1.,1.),(1.,1.),(1.,
1.),(1.,1.),(1.,1.),(1.,1.),(1.,1.),(1.,1.),(1.,1.),(1.,1.),(1.,1.),(1.,
1.),(1.,1.)))
REPRESENTATION_ITEM('')
SURFACE()
);
#84=(
BOUNDED_SURFACE()
B_SPLINE_SURFACE(5,1,((#47252,#47253),(#47254,#47255),(#47256,#47257),(#47258,
#47259),(#47260,#47261),(#47262,#47263),(#47264,#47265),(#47266,#47267),
(#47268,#47269),(#47270,#47271),(#47272,#47273),(#47274,#47275),(#47276,
#47277),(#47278,#47279),(#47280,#47281),(#47282,#47283),(#47284,#47285),
(#47286,#47287),(#47288,#47289),(#47290,#47291),(#47292,#47293),(#47294,
#47295),(#47296,#47297),(#47298,#47299),(#47300,#47301),(#47302,#47303),
(#47304,#47305),(#47306,#47307),(#47308,#47309),(#47310,#47311),(#47312,
#47313),(#47314,#47315),(#47316,#47317),(#47318,#47319),(#47320,#47321),
(#47322,#47323),(#47324,#47325),(#47326,#47327),(#47328,#47329),(#47330,
#47331),(#47332,#47333),(#47334,#47335),(#47336,#47337),(#47338,#47339),
(#47340,#47341),(#47342,#47343),(#47344,#47345),(#47346,#47347),(#47348,
#47349),(#47350,#47351),(#47352,#47353),(#47354,#47355),(#47356,#47357),
(#47358,#47359),(#47360,#47361),(#47362,#47363),(#47364,#47365),(#47366,
#47367),(#47368,#47369),(#47370,#47371),(#47372,#47373),(#47374,#47375),
(#47376,#47377),(#47378,#47379),(#47380,#47381),(#47382,#47383),(#47384,
#47385),(#47386,#47387),(#47388,#47389),(#47390,#47391)),.UNSPECIFIED.,
 .F.,.F.,.F.)
B_SPLINE_SURFACE_WITH_KNOTS((6,1,1,1,1,1,1,1,1,1,1,1,1,1,1,1,1,1,1,1,1,
1,1,1,1,1,1,1,1,1,1,1,1,1,1,1,1,1,1,1,1,1,1,1,1,1,1,1,1,1,1,1,1,1,1,1,1,
1,1,1,1,1,1,1,1,6),(2,2),(-1.,-0.984615384615383,-0.969230769230768,-0.953846153846152,
-0.938461538461537,-0.923076923076922,-0.907692307692306,-0.892307692307691,
-0.876923076923076,-0.86153846153846,-0.846153846153845,-0.83076923076923,
-0.815384615384614,-0.799999999999999,-0.784615384615384,-0.769230769230768,
-0.753846153846153,-0.738461538461538,-0.723076923076922,-0.707692307692307,
-0.692307692307692,-0.676923076923076,-0.661538461538461,-0.646153846153846,
-0.63076923076923,-0.615384615384615,-0.6,-0.584615384615384,-0.569230769230769,
-0.553846153846154,-0.538461538461538,-0.523076923076923,-0.507692307692308,
-0.492307692307692,-0.476923076923077,-0.461538461538462,-0.446153846153846,
-0.430769230769231,-0.415384615384615,-0.4,-0.384615384615385,-0.369230769230769,
-0.353846153846154,-0.338461538461538,-0.323076923076923,-0.307692307692308,
-0.292307692307692,-0.276923076923077,-0.261538461538462,-0.246153846153846,
-0.230769230769231,-0.215384615384615,-0.2,-0.184615384615385,-0.169230769230769,
-0.153846153846154,-0.138461538461538,-0.123076923076923,-0.107692307692308,
-0.0923076923076923,-0.0769230769230769,-0.0615384615384615,-0.0461538461538462,
-0.0307692307692308,-0.0153846153846154,0.),(-1.,1.),.UNSPECIFIED.)
GEOMETRIC_REPRESENTATION_ITEM()
RATIONAL_B_SPLINE_SURFACE(((1.,1.),(1.,1.),(1.,1.),(1.,1.),(1.,1.),(1.,
1.),(1.,1.),(1.,1.),(1.,1.),(1.,1.),(1.,1.),(1.,1.),(1.,1.),(1.,1.),(1.,
1.),(1.,1.),(1.,1.),(1.,1.),(1.,1.),(1.,1.),(1.,1.),(1.,1.),(1.,1.),(1.,
1.),(1.,1.),(1.,1.),(1.,1.),(1.,1.),(1.,1.),(1.,1.),(1.,1.),(1.,1.),(1.,
1.),(1.,1.),(1.,1.),(1.,1.),(1.,1.),(1.,1.),(1.,1.),(1.,1.),(1.,1.),(1.,
1.),(1.,1.),(1.,1.),(1.,1.),(1.,1.),(1.,1.),(1.,1.),(1.,1.),(1.,1.),(1.,
1.),(1.,1.),(1.,1.),(1.,1.),(1.,1.),(1.,1.),(1.,1.),(1.,1.),(1.,1.),(1.,
1.),(1.,1.),(1.,1.),(1.,1.),(1.,1.),(1.,1.),(1.,1.),(1.,1.),(1.,1.),(1.,
1.),(1.,1.)))
REPRESENTATION_ITEM('')
SURFACE()
);
#85=(
BOUNDED_SURFACE()
B_SPLINE_SURFACE(5,1,((#47482,#47483),(#47484,#47485),(#47486,#47487),(#47488,
#47489),(#47490,#47491),(#47492,#47493),(#47494,#47495),(#47496,#47497),
(#47498,#47499),(#47500,#47501),(#47502,#47503),(#47504,#47505),(#47506,
#47507),(#47508,#47509),(#47510,#47511),(#47512,#47513),(#47514,#47515),
(#47516,#47517),(#47518,#47519),(#47520,#47521),(#47522,#47523),(#47524,
#47525),(#47526,#47527),(#47528,#47529),(#47530,#47531),(#47532,#47533),
(#47534,#47535),(#47536,#47537),(#47538,#47539),(#47540,#47541),(#47542,
#47543),(#47544,#47545),(#47546,#47547),(#47548,#47549),(#47550,#47551),
(#47552,#47553),(#47554,#47555),(#47556,#47557),(#47558,#47559),(#47560,
#47561),(#47562,#47563),(#47564,#47565),(#47566,#47567),(#47568,#47569),
(#47570,#47571),(#47572,#47573),(#47574,#47575),(#47576,#47577),(#47578,
#47579),(#47580,#47581),(#47582,#47583),(#47584,#47585),(#47586,#47587),
(#47588,#47589),(#47590,#47591),(#47592,#47593),(#47594,#47595),(#47596,
#47597),(#47598,#47599),(#47600,#47601),(#47602,#47603),(#47604,#47605),
(#47606,#47607),(#47608,#47609),(#47610,#47611),(#47612,#47613),(#47614,
#47615),(#47616,#47617),(#47618,#47619),(#47620,#47621)),.UNSPECIFIED.,
 .F.,.F.,.F.)
B_SPLINE_SURFACE_WITH_KNOTS((6,1,1,1,1,1,1,1,1,1,1,1,1,1,1,1,1,1,1,1,1,
1,1,1,1,1,1,1,1,1,1,1,1,1,1,1,1,1,1,1,1,1,1,1,1,1,1,1,1,1,1,1,1,1,1,1,1,
1,1,1,1,1,1,1,1,6),(2,2),(-1.,-0.984615384615383,-0.969230769230768,-0.953846153846152,
-0.938461538461537,-0.923076923076922,-0.907692307692306,-0.892307692307691,
-0.876923076923076,-0.86153846153846,-0.846153846153845,-0.83076923076923,
-0.815384615384614,-0.799999999999999,-0.784615384615384,-0.769230769230768,
-0.753846153846153,-0.738461538461538,-0.723076923076922,-0.707692307692307,
-0.692307692307692,-0.676923076923076,-0.661538461538461,-0.646153846153846,
-0.63076923076923,-0.615384615384615,-0.6,-0.584615384615384,-0.569230769230769,
-0.553846153846154,-0.538461538461538,-0.523076923076923,-0.507692307692308,
-0.492307692307692,-0.476923076923077,-0.461538461538462,-0.446153846153846,
-0.430769230769231,-0.415384615384615,-0.4,-0.384615384615385,-0.369230769230769,
-0.353846153846154,-0.338461538461538,-0.323076923076923,-0.307692307692308,
-0.292307692307692,-0.276923076923077,-0.261538461538462,-0.246153846153846,
-0.230769230769231,-0.215384615384615,-0.2,-0.184615384615385,-0.169230769230769,
-0.153846153846154,-0.138461538461538,-0.123076923076923,-0.107692307692308,
-0.0923076923076923,-0.0769230769230769,-0.0615384615384615,-0.0461538461538462,
-0.0307692307692308,-0.0153846153846154,0.),(-1.,1.),.UNSPECIFIED.)
GEOMETRIC_REPRESENTATION_ITEM()
RATIONAL_B_SPLINE_SURFACE(((1.,1.),(1.,1.),(1.,1.),(1.,1.),(1.,1.),(1.,
1.),(1.,1.),(1.,1.),(1.,1.),(1.,1.),(1.,1.),(1.,1.),(1.,1.),(1.,1.),(1.,
1.),(1.,1.),(1.,1.),(1.,1.),(1.,1.),(1.,1.),(1.,1.),(1.,1.),(1.,1.),(1.,
1.),(1.,1.),(1.,1.),(1.,1.),(1.,1.),(1.,1.),(1.,1.),(1.,1.),(1.,1.),(1.,
1.),(1.,1.),(1.,1.),(1.,1.),(1.,1.),(1.,1.),(1.,1.),(1.,1.),(1.,1.),(1.,
1.),(1.,1.),(1.,1.),(1.,1.),(1.,1.),(1.,1.),(1.,1.),(1.,1.),(1.,1.),(1.,
1.),(1.,1.),(1.,1.),(1.,1.),(1.,1.),(1.,1.),(1.,1.),(1.,1.),(1.,1.),(1.,
1.),(1.,1.),(1.,1.),(1.,1.),(1.,1.),(1.,1.),(1.,1.),(1.,1.),(1.,1.),(1.,
1.),(1.,1.)))
REPRESENTATION_ITEM('')
SURFACE()
);
#86=(
BOUNDED_SURFACE()
B_SPLINE_SURFACE(5,1,((#47694,#47695),(#47696,#47697),(#47698,#47699),(#47700,
#47701),(#47702,#47703),(#47704,#47705),(#47706,#47707),(#47708,#47709),
(#47710,#47711),(#47712,#47713),(#47714,#47715),(#47716,#47717),(#47718,
#47719),(#47720,#47721),(#47722,#47723),(#47724,#47725),(#47726,#47727),
(#47728,#47729),(#47730,#47731),(#47732,#47733),(#47734,#47735),(#47736,
#47737),(#47738,#47739),(#47740,#47741),(#47742,#47743),(#47744,#47745),
(#47746,#47747),(#47748,#47749),(#47750,#47751),(#47752,#47753),(#47754,
#47755),(#47756,#47757),(#47758,#47759),(#47760,#47761),(#47762,#47763),
(#47764,#47765),(#47766,#47767),(#47768,#47769),(#47770,#47771),(#47772,
#47773),(#47774,#47775),(#47776,#47777),(#47778,#47779),(#47780,#47781),
(#47782,#47783),(#47784,#47785),(#47786,#47787),(#47788,#47789),(#47790,
#47791),(#47792,#47793),(#47794,#47795),(#47796,#47797),(#47798,#47799),
(#47800,#47801),(#47802,#47803),(#47804,#47805),(#47806,#47807),(#47808,
#47809),(#47810,#47811),(#47812,#47813),(#47814,#47815),(#47816,#47817),
(#47818,#47819),(#47820,#47821),(#47822,#47823),(#47824,#47825),(#47826,
#47827),(#47828,#47829),(#47830,#47831),(#47832,#47833)),.UNSPECIFIED.,
 .F.,.F.,.F.)
B_SPLINE_SURFACE_WITH_KNOTS((6,1,1,1,1,1,1,1,1,1,1,1,1,1,1,1,1,1,1,1,1,
1,1,1,1,1,1,1,1,1,1,1,1,1,1,1,1,1,1,1,1,1,1,1,1,1,1,1,1,1,1,1,1,1,1,1,1,
1,1,1,1,1,1,1,1,6),(2,2),(-1.,-0.984615384615383,-0.969230769230768,-0.953846153846152,
-0.938461538461537,-0.923076923076922,-0.907692307692306,-0.892307692307691,
-0.876923076923076,-0.86153846153846,-0.846153846153845,-0.83076923076923,
-0.815384615384614,-0.799999999999999,-0.784615384615384,-0.769230769230768,
-0.753846153846153,-0.738461538461538,-0.723076923076922,-0.707692307692307,
-0.692307692307692,-0.676923076923076,-0.661538461538461,-0.646153846153846,
-0.63076923076923,-0.615384615384615,-0.6,-0.584615384615384,-0.569230769230769,
-0.553846153846154,-0.538461538461538,-0.523076923076923,-0.507692307692308,
-0.492307692307692,-0.476923076923077,-0.461538461538462,-0.446153846153846,
-0.430769230769231,-0.415384615384615,-0.4,-0.384615384615385,-0.369230769230769,
-0.353846153846154,-0.338461538461538,-0.323076923076923,-0.307692307692308,
-0.292307692307692,-0.276923076923077,-0.261538461538462,-0.246153846153846,
-0.230769230769231,-0.215384615384615,-0.2,-0.184615384615385,-0.169230769230769,
-0.153846153846154,-0.138461538461538,-0.123076923076923,-0.107692307692308,
-0.0923076923076923,-0.0769230769230769,-0.0615384615384615,-0.0461538461538462,
-0.0307692307692308,-0.0153846153846154,0.),(-1.,1.),.UNSPECIFIED.)
GEOMETRIC_REPRESENTATION_ITEM()
RATIONAL_B_SPLINE_SURFACE(((1.,1.),(1.,1.),(1.,1.),(1.,1.),(1.,1.),(1.,
1.),(1.,1.),(1.,1.),(1.,1.),(1.,1.),(1.,1.),(1.,1.),(1.,1.),(1.,1.),(1.,
1.),(1.,1.),(1.,1.),(1.,1.),(1.,1.),(1.,1.),(1.,1.),(1.,1.),(1.,1.),(1.,
1.),(1.,1.),(1.,1.),(1.,1.),(1.,1.),(1.,1.),(1.,1.),(1.,1.),(1.,1.),(1.,
1.),(1.,1.),(1.,1.),(1.,1.),(1.,1.),(1.,1.),(1.,1.),(1.,1.),(1.,1.),(1.,
1.),(1.,1.),(1.,1.),(1.,1.),(1.,1.),(1.,1.),(1.,1.),(1.,1.),(1.,1.),(1.,
1.),(1.,1.),(1.,1.),(1.,1.),(1.,1.),(1.,1.),(1.,1.),(1.,1.),(1.,1.),(1.,
1.),(1.,1.),(1.,1.),(1.,1.),(1.,1.),(1.,1.),(1.,1.),(1.,1.),(1.,1.),(1.,
1.),(1.,1.)))
REPRESENTATION_ITEM('')
SURFACE()
);
#87=(
BOUNDED_SURFACE()
B_SPLINE_SURFACE(5,1,((#47924,#47925),(#47926,#47927),(#47928,#47929),(#47930,
#47931),(#47932,#47933),(#47934,#47935),(#47936,#47937),(#47938,#47939),
(#47940,#47941),(#47942,#47943),(#47944,#47945),(#47946,#47947),(#47948,
#47949),(#47950,#47951),(#47952,#47953),(#47954,#47955),(#47956,#47957),
(#47958,#47959),(#47960,#47961),(#47962,#47963),(#47964,#47965),(#47966,
#47967),(#47968,#47969),(#47970,#47971),(#47972,#47973),(#47974,#47975),
(#47976,#47977),(#47978,#47979),(#47980,#47981),(#47982,#47983),(#47984,
#47985),(#47986,#47987),(#47988,#47989),(#47990,#47991),(#47992,#47993),
(#47994,#47995),(#47996,#47997),(#47998,#47999),(#48000,#48001),(#48002,
#48003),(#48004,#48005),(#48006,#48007),(#48008,#48009),(#48010,#48011),
(#48012,#48013),(#48014,#48015),(#48016,#48017),(#48018,#48019),(#48020,
#48021),(#48022,#48023),(#48024,#48025),(#48026,#48027),(#48028,#48029),
(#48030,#48031),(#48032,#48033),(#48034,#48035),(#48036,#48037),(#48038,
#48039),(#48040,#48041),(#48042,#48043),(#48044,#48045),(#48046,#48047),
(#48048,#48049),(#48050,#48051),(#48052,#48053),(#48054,#48055),(#48056,
#48057),(#48058,#48059),(#48060,#48061),(#48062,#48063)),.UNSPECIFIED.,
 .F.,.F.,.F.)
B_SPLINE_SURFACE_WITH_KNOTS((6,1,1,1,1,1,1,1,1,1,1,1,1,1,1,1,1,1,1,1,1,
1,1,1,1,1,1,1,1,1,1,1,1,1,1,1,1,1,1,1,1,1,1,1,1,1,1,1,1,1,1,1,1,1,1,1,1,
1,1,1,1,1,1,1,1,6),(2,2),(-1.,-0.984615384615383,-0.969230769230768,-0.953846153846152,
-0.938461538461537,-0.923076923076922,-0.907692307692306,-0.892307692307691,
-0.876923076923076,-0.86153846153846,-0.846153846153845,-0.83076923076923,
-0.815384615384614,-0.799999999999999,-0.784615384615384,-0.769230769230768,
-0.753846153846153,-0.738461538461538,-0.723076923076922,-0.707692307692307,
-0.692307692307692,-0.676923076923076,-0.661538461538461,-0.646153846153846,
-0.63076923076923,-0.615384615384615,-0.6,-0.584615384615384,-0.569230769230769,
-0.553846153846154,-0.538461538461538,-0.523076923076923,-0.507692307692308,
-0.492307692307692,-0.476923076923077,-0.461538461538462,-0.446153846153846,
-0.430769230769231,-0.415384615384615,-0.4,-0.384615384615385,-0.369230769230769,
-0.353846153846154,-0.338461538461538,-0.323076923076923,-0.307692307692308,
-0.292307692307692,-0.276923076923077,-0.261538461538462,-0.246153846153846,
-0.230769230769231,-0.215384615384615,-0.2,-0.184615384615385,-0.169230769230769,
-0.153846153846154,-0.138461538461538,-0.123076923076923,-0.107692307692308,
-0.0923076923076923,-0.0769230769230769,-0.0615384615384615,-0.0461538461538462,
-0.0307692307692308,-0.0153846153846154,0.),(-1.,1.),.UNSPECIFIED.)
GEOMETRIC_REPRESENTATION_ITEM()
RATIONAL_B_SPLINE_SURFACE(((1.,1.),(1.,1.),(1.,1.),(1.,1.),(1.,1.),(1.,
1.),(1.,1.),(1.,1.),(1.,1.),(1.,1.),(1.,1.),(1.,1.),(1.,1.),(1.,1.),(1.,
1.),(1.,1.),(1.,1.),(1.,1.),(1.,1.),(1.,1.),(1.,1.),(1.,1.),(1.,1.),(1.,
1.),(1.,1.),(1.,1.),(1.,1.),(1.,1.),(1.,1.),(1.,1.),(1.,1.),(1.,1.),(1.,
1.),(1.,1.),(1.,1.),(1.,1.),(1.,1.),(1.,1.),(1.,1.),(1.,1.),(1.,1.),(1.,
1.),(1.,1.),(1.,1.),(1.,1.),(1.,1.),(1.,1.),(1.,1.),(1.,1.),(1.,1.),(1.,
1.),(1.,1.),(1.,1.),(1.,1.),(1.,1.),(1.,1.),(1.,1.),(1.,1.),(1.,1.),(1.,
1.),(1.,1.),(1.,1.),(1.,1.),(1.,1.),(1.,1.),(1.,1.),(1.,1.),(1.,1.),(1.,
1.),(1.,1.)))
REPRESENTATION_ITEM('')
SURFACE()
);
#88=(
BOUNDED_SURFACE()
B_SPLINE_SURFACE(5,1,((#48136,#48137),(#48138,#48139),(#48140,#48141),(#48142,
#48143),(#48144,#48145),(#48146,#48147),(#48148,#48149),(#48150,#48151),
(#48152,#48153),(#48154,#48155),(#48156,#48157),(#48158,#48159),(#48160,
#48161),(#48162,#48163),(#48164,#48165),(#48166,#48167),(#48168,#48169),
(#48170,#48171),(#48172,#48173),(#48174,#48175),(#48176,#48177),(#48178,
#48179),(#48180,#48181),(#48182,#48183),(#48184,#48185),(#48186,#48187),
(#48188,#48189),(#48190,#48191),(#48192,#48193),(#48194,#48195),(#48196,
#48197),(#48198,#48199),(#48200,#48201),(#48202,#48203),(#48204,#48205),
(#48206,#48207),(#48208,#48209),(#48210,#48211),(#48212,#48213),(#48214,
#48215),(#48216,#48217),(#48218,#48219),(#48220,#48221),(#48222,#48223),
(#48224,#48225),(#48226,#48227),(#48228,#48229),(#48230,#48231),(#48232,
#48233),(#48234,#48235),(#48236,#48237),(#48238,#48239),(#48240,#48241),
(#48242,#48243),(#48244,#48245),(#48246,#48247),(#48248,#48249),(#48250,
#48251),(#48252,#48253),(#48254,#48255),(#48256,#48257),(#48258,#48259),
(#48260,#48261),(#48262,#48263),(#48264,#48265),(#48266,#48267),(#48268,
#48269),(#48270,#48271),(#48272,#48273),(#48274,#48275)),.UNSPECIFIED.,
 .F.,.F.,.F.)
B_SPLINE_SURFACE_WITH_KNOTS((6,1,1,1,1,1,1,1,1,1,1,1,1,1,1,1,1,1,1,1,1,
1,1,1,1,1,1,1,1,1,1,1,1,1,1,1,1,1,1,1,1,1,1,1,1,1,1,1,1,1,1,1,1,1,1,1,1,
1,1,1,1,1,1,1,1,6),(2,2),(-1.,-0.984615384615383,-0.969230769230768,-0.953846153846152,
-0.938461538461537,-0.923076923076922,-0.907692307692306,-0.892307692307691,
-0.876923076923076,-0.86153846153846,-0.846153846153845,-0.83076923076923,
-0.815384615384614,-0.799999999999999,-0.784615384615384,-0.769230769230768,
-0.753846153846153,-0.738461538461538,-0.723076923076922,-0.707692307692307,
-0.692307692307692,-0.676923076923076,-0.661538461538461,-0.646153846153846,
-0.63076923076923,-0.615384615384615,-0.6,-0.584615384615384,-0.569230769230769,
-0.553846153846154,-0.538461538461538,-0.523076923076923,-0.507692307692308,
-0.492307692307692,-0.476923076923077,-0.461538461538462,-0.446153846153846,
-0.430769230769231,-0.415384615384615,-0.4,-0.384615384615385,-0.369230769230769,
-0.353846153846154,-0.338461538461538,-0.323076923076923,-0.307692307692308,
-0.292307692307692,-0.276923076923077,-0.261538461538462,-0.246153846153846,
-0.230769230769231,-0.215384615384615,-0.2,-0.184615384615385,-0.169230769230769,
-0.153846153846154,-0.138461538461538,-0.123076923076923,-0.107692307692308,
-0.0923076923076923,-0.0769230769230769,-0.0615384615384615,-0.0461538461538462,
-0.0307692307692308,-0.0153846153846154,0.),(-1.,1.),.UNSPECIFIED.)
GEOMETRIC_REPRESENTATION_ITEM()
RATIONAL_B_SPLINE_SURFACE(((1.,1.),(1.,1.),(1.,1.),(1.,1.),(1.,1.),(1.,
1.),(1.,1.),(1.,1.),(1.,1.),(1.,1.),(1.,1.),(1.,1.),(1.,1.),(1.,1.),(1.,
1.),(1.,1.),(1.,1.),(1.,1.),(1.,1.),(1.,1.),(1.,1.),(1.,1.),(1.,1.),(1.,
1.),(1.,1.),(1.,1.),(1.,1.),(1.,1.),(1.,1.),(1.,1.),(1.,1.),(1.,1.),(1.,
1.),(1.,1.),(1.,1.),(1.,1.),(1.,1.),(1.,1.),(1.,1.),(1.,1.),(1.,1.),(1.,
1.),(1.,1.),(1.,1.),(1.,1.),(1.,1.),(1.,1.),(1.,1.),(1.,1.),(1.,1.),(1.,
1.),(1.,1.),(1.,1.),(1.,1.),(1.,1.),(1.,1.),(1.,1.),(1.,1.),(1.,1.),(1.,
1.),(1.,1.),(1.,1.),(1.,1.),(1.,1.),(1.,1.),(1.,1.),(1.,1.),(1.,1.),(1.,
1.),(1.,1.)))
REPRESENTATION_ITEM('')
SURFACE()
);
#89=(
BOUNDED_SURFACE()
B_SPLINE_SURFACE(5,1,((#48366,#48367),(#48368,#48369),(#48370,#48371),(#48372,
#48373),(#48374,#48375),(#48376,#48377),(#48378,#48379),(#48380,#48381),
(#48382,#48383),(#48384,#48385),(#48386,#48387),(#48388,#48389),(#48390,
#48391),(#48392,#48393),(#48394,#48395),(#48396,#48397),(#48398,#48399),
(#48400,#48401),(#48402,#48403),(#48404,#48405),(#48406,#48407),(#48408,
#48409),(#48410,#48411),(#48412,#48413),(#48414,#48415),(#48416,#48417),
(#48418,#48419),(#48420,#48421),(#48422,#48423),(#48424,#48425),(#48426,
#48427),(#48428,#48429),(#48430,#48431),(#48432,#48433),(#48434,#48435),
(#48436,#48437),(#48438,#48439),(#48440,#48441),(#48442,#48443),(#48444,
#48445),(#48446,#48447),(#48448,#48449),(#48450,#48451),(#48452,#48453),
(#48454,#48455),(#48456,#48457),(#48458,#48459),(#48460,#48461),(#48462,
#48463),(#48464,#48465),(#48466,#48467),(#48468,#48469),(#48470,#48471),
(#48472,#48473),(#48474,#48475),(#48476,#48477),(#48478,#48479),(#48480,
#48481),(#48482,#48483),(#48484,#48485),(#48486,#48487),(#48488,#48489),
(#48490,#48491),(#48492,#48493),(#48494,#48495),(#48496,#48497),(#48498,
#48499),(#48500,#48501),(#48502,#48503),(#48504,#48505)),.UNSPECIFIED.,
 .F.,.F.,.F.)
B_SPLINE_SURFACE_WITH_KNOTS((6,1,1,1,1,1,1,1,1,1,1,1,1,1,1,1,1,1,1,1,1,
1,1,1,1,1,1,1,1,1,1,1,1,1,1,1,1,1,1,1,1,1,1,1,1,1,1,1,1,1,1,1,1,1,1,1,1,
1,1,1,1,1,1,1,1,6),(2,2),(-1.,-0.984615384615383,-0.969230769230768,-0.953846153846152,
-0.938461538461537,-0.923076923076922,-0.907692307692306,-0.892307692307691,
-0.876923076923076,-0.86153846153846,-0.846153846153845,-0.83076923076923,
-0.815384615384614,-0.799999999999999,-0.784615384615384,-0.769230769230768,
-0.753846153846153,-0.738461538461538,-0.723076923076922,-0.707692307692307,
-0.692307692307692,-0.676923076923076,-0.661538461538461,-0.646153846153846,
-0.63076923076923,-0.615384615384615,-0.6,-0.584615384615384,-0.569230769230769,
-0.553846153846154,-0.538461538461538,-0.523076923076923,-0.507692307692308,
-0.492307692307692,-0.476923076923077,-0.461538461538462,-0.446153846153846,
-0.430769230769231,-0.415384615384615,-0.4,-0.384615384615385,-0.369230769230769,
-0.353846153846154,-0.338461538461538,-0.323076923076923,-0.307692307692308,
-0.292307692307692,-0.276923076923077,-0.261538461538462,-0.246153846153846,
-0.230769230769231,-0.215384615384615,-0.2,-0.184615384615385,-0.169230769230769,
-0.153846153846154,-0.138461538461538,-0.123076923076923,-0.107692307692308,
-0.0923076923076923,-0.0769230769230769,-0.0615384615384615,-0.0461538461538462,
-0.0307692307692308,-0.0153846153846154,0.),(-1.,1.),.UNSPECIFIED.)
GEOMETRIC_REPRESENTATION_ITEM()
RATIONAL_B_SPLINE_SURFACE(((1.,1.),(1.,1.),(1.,1.),(1.,1.),(1.,1.),(1.,
1.),(1.,1.),(1.,1.),(1.,1.),(1.,1.),(1.,1.),(1.,1.),(1.,1.),(1.,1.),(1.,
1.),(1.,1.),(1.,1.),(1.,1.),(1.,1.),(1.,1.),(1.,1.),(1.,1.),(1.,1.),(1.,
1.),(1.,1.),(1.,1.),(1.,1.),(1.,1.),(1.,1.),(1.,1.),(1.,1.),(1.,1.),(1.,
1.),(1.,1.),(1.,1.),(1.,1.),(1.,1.),(1.,1.),(1.,1.),(1.,1.),(1.,1.),(1.,
1.),(1.,1.),(1.,1.),(1.,1.),(1.,1.),(1.,1.),(1.,1.),(1.,1.),(1.,1.),(1.,
1.),(1.,1.),(1.,1.),(1.,1.),(1.,1.),(1.,1.),(1.,1.),(1.,1.),(1.,1.),(1.,
1.),(1.,1.),(1.,1.),(1.,1.),(1.,1.),(1.,1.),(1.,1.),(1.,1.),(1.,1.),(1.,
1.),(1.,1.)))
REPRESENTATION_ITEM('')
SURFACE()
);
#90=(
BOUNDED_SURFACE()
B_SPLINE_SURFACE(5,1,((#48578,#48579),(#48580,#48581),(#48582,#48583),(#48584,
#48585),(#48586,#48587),(#48588,#48589),(#48590,#48591),(#48592,#48593),
(#48594,#48595),(#48596,#48597),(#48598,#48599),(#48600,#48601),(#48602,
#48603),(#48604,#48605),(#48606,#48607),(#48608,#48609),(#48610,#48611),
(#48612,#48613),(#48614,#48615),(#48616,#48617),(#48618,#48619),(#48620,
#48621),(#48622,#48623),(#48624,#48625),(#48626,#48627),(#48628,#48629),
(#48630,#48631),(#48632,#48633),(#48634,#48635),(#48636,#48637),(#48638,
#48639),(#48640,#48641),(#48642,#48643),(#48644,#48645),(#48646,#48647),
(#48648,#48649),(#48650,#48651),(#48652,#48653),(#48654,#48655),(#48656,
#48657),(#48658,#48659),(#48660,#48661),(#48662,#48663),(#48664,#48665),
(#48666,#48667),(#48668,#48669),(#48670,#48671),(#48672,#48673),(#48674,
#48675),(#48676,#48677),(#48678,#48679),(#48680,#48681),(#48682,#48683),
(#48684,#48685),(#48686,#48687),(#48688,#48689),(#48690,#48691),(#48692,
#48693),(#48694,#48695),(#48696,#48697),(#48698,#48699),(#48700,#48701),
(#48702,#48703),(#48704,#48705),(#48706,#48707),(#48708,#48709),(#48710,
#48711),(#48712,#48713),(#48714,#48715),(#48716,#48717)),.UNSPECIFIED.,
 .F.,.F.,.F.)
B_SPLINE_SURFACE_WITH_KNOTS((6,1,1,1,1,1,1,1,1,1,1,1,1,1,1,1,1,1,1,1,1,
1,1,1,1,1,1,1,1,1,1,1,1,1,1,1,1,1,1,1,1,1,1,1,1,1,1,1,1,1,1,1,1,1,1,1,1,
1,1,1,1,1,1,1,1,6),(2,2),(-1.,-0.984615384615383,-0.969230769230768,-0.953846153846152,
-0.938461538461537,-0.923076923076922,-0.907692307692306,-0.892307692307691,
-0.876923076923076,-0.86153846153846,-0.846153846153845,-0.83076923076923,
-0.815384615384614,-0.799999999999999,-0.784615384615384,-0.769230769230768,
-0.753846153846153,-0.738461538461538,-0.723076923076922,-0.707692307692307,
-0.692307692307692,-0.676923076923076,-0.661538461538461,-0.646153846153846,
-0.63076923076923,-0.615384615384615,-0.6,-0.584615384615384,-0.569230769230769,
-0.553846153846154,-0.538461538461538,-0.523076923076923,-0.507692307692308,
-0.492307692307692,-0.476923076923077,-0.461538461538462,-0.446153846153846,
-0.430769230769231,-0.415384615384615,-0.4,-0.384615384615385,-0.369230769230769,
-0.353846153846154,-0.338461538461538,-0.323076923076923,-0.307692307692308,
-0.292307692307692,-0.276923076923077,-0.261538461538462,-0.246153846153846,
-0.230769230769231,-0.215384615384615,-0.2,-0.184615384615385,-0.169230769230769,
-0.153846153846154,-0.138461538461538,-0.123076923076923,-0.107692307692308,
-0.0923076923076923,-0.0769230769230769,-0.0615384615384615,-0.0461538461538462,
-0.0307692307692308,-0.0153846153846154,0.),(-1.,1.),.UNSPECIFIED.)
GEOMETRIC_REPRESENTATION_ITEM()
RATIONAL_B_SPLINE_SURFACE(((1.,1.),(1.,1.),(1.,1.),(1.,1.),(1.,1.),(1.,
1.),(1.,1.),(1.,1.),(1.,1.),(1.,1.),(1.,1.),(1.,1.),(1.,1.),(1.,1.),(1.,
1.),(1.,1.),(1.,1.),(1.,1.),(1.,1.),(1.,1.),(1.,1.),(1.,1.),(1.,1.),(1.,
1.),(1.,1.),(1.,1.),(1.,1.),(1.,1.),(1.,1.),(1.,1.),(1.,1.),(1.,1.),(1.,
1.),(1.,1.),(1.,1.),(1.,1.),(1.,1.),(1.,1.),(1.,1.),(1.,1.),(1.,1.),(1.,
1.),(1.,1.),(1.,1.),(1.,1.),(1.,1.),(1.,1.),(1.,1.),(1.,1.),(1.,1.),(1.,
1.),(1.,1.),(1.,1.),(1.,1.),(1.,1.),(1.,1.),(1.,1.),(1.,1.),(1.,1.),(1.,
1.),(1.,1.),(1.,1.),(1.,1.),(1.,1.),(1.,1.),(1.,1.),(1.,1.),(1.,1.),(1.,
1.),(1.,1.)))
REPRESENTATION_ITEM('')
SURFACE()
);
#91=(
BOUNDED_SURFACE()
B_SPLINE_SURFACE(5,1,((#48808,#48809),(#48810,#48811),(#48812,#48813),(#48814,
#48815),(#48816,#48817),(#48818,#48819),(#48820,#48821),(#48822,#48823),
(#48824,#48825),(#48826,#48827),(#48828,#48829),(#48830,#48831),(#48832,
#48833),(#48834,#48835),(#48836,#48837),(#48838,#48839),(#48840,#48841),
(#48842,#48843),(#48844,#48845),(#48846,#48847),(#48848,#48849),(#48850,
#48851),(#48852,#48853),(#48854,#48855),(#48856,#48857),(#48858,#48859),
(#48860,#48861),(#48862,#48863),(#48864,#48865),(#48866,#48867),(#48868,
#48869),(#48870,#48871),(#48872,#48873),(#48874,#48875),(#48876,#48877),
(#48878,#48879),(#48880,#48881),(#48882,#48883),(#48884,#48885),(#48886,
#48887),(#48888,#48889),(#48890,#48891),(#48892,#48893),(#48894,#48895),
(#48896,#48897),(#48898,#48899),(#48900,#48901),(#48902,#48903),(#48904,
#48905),(#48906,#48907),(#48908,#48909),(#48910,#48911),(#48912,#48913),
(#48914,#48915),(#48916,#48917),(#48918,#48919),(#48920,#48921),(#48922,
#48923),(#48924,#48925),(#48926,#48927),(#48928,#48929),(#48930,#48931),
(#48932,#48933),(#48934,#48935),(#48936,#48937),(#48938,#48939),(#48940,
#48941),(#48942,#48943),(#48944,#48945),(#48946,#48947)),.UNSPECIFIED.,
 .F.,.F.,.F.)
B_SPLINE_SURFACE_WITH_KNOTS((6,1,1,1,1,1,1,1,1,1,1,1,1,1,1,1,1,1,1,1,1,
1,1,1,1,1,1,1,1,1,1,1,1,1,1,1,1,1,1,1,1,1,1,1,1,1,1,1,1,1,1,1,1,1,1,1,1,
1,1,1,1,1,1,1,1,6),(2,2),(-1.,-0.984615384615383,-0.969230769230768,-0.953846153846152,
-0.938461538461537,-0.923076923076922,-0.907692307692306,-0.892307692307691,
-0.876923076923076,-0.86153846153846,-0.846153846153845,-0.83076923076923,
-0.815384615384614,-0.799999999999999,-0.784615384615384,-0.769230769230768,
-0.753846153846153,-0.738461538461538,-0.723076923076922,-0.707692307692307,
-0.692307692307692,-0.676923076923076,-0.661538461538461,-0.646153846153846,
-0.63076923076923,-0.615384615384615,-0.6,-0.584615384615384,-0.569230769230769,
-0.553846153846154,-0.538461538461538,-0.523076923076923,-0.507692307692308,
-0.492307692307692,-0.476923076923077,-0.461538461538462,-0.446153846153846,
-0.430769230769231,-0.415384615384615,-0.4,-0.384615384615385,-0.369230769230769,
-0.353846153846154,-0.338461538461538,-0.323076923076923,-0.307692307692308,
-0.292307692307692,-0.276923076923077,-0.261538461538462,-0.246153846153846,
-0.230769230769231,-0.215384615384615,-0.2,-0.184615384615385,-0.169230769230769,
-0.153846153846154,-0.138461538461538,-0.123076923076923,-0.107692307692308,
-0.0923076923076923,-0.0769230769230769,-0.0615384615384615,-0.0461538461538462,
-0.0307692307692308,-0.0153846153846154,0.),(-1.,1.),.UNSPECIFIED.)
GEOMETRIC_REPRESENTATION_ITEM()
RATIONAL_B_SPLINE_SURFACE(((1.,1.),(1.,1.),(1.,1.),(1.,1.),(1.,1.),(1.,
1.),(1.,1.),(1.,1.),(1.,1.),(1.,1.),(1.,1.),(1.,1.),(1.,1.),(1.,1.),(1.,
1.),(1.,1.),(1.,1.),(1.,1.),(1.,1.),(1.,1.),(1.,1.),(1.,1.),(1.,1.),(1.,
1.),(1.,1.),(1.,1.),(1.,1.),(1.,1.),(1.,1.),(1.,1.),(1.,1.),(1.,1.),(1.,
1.),(1.,1.),(1.,1.),(1.,1.),(1.,1.),(1.,1.),(1.,1.),(1.,1.),(1.,1.),(1.,
1.),(1.,1.),(1.,1.),(1.,1.),(1.,1.),(1.,1.),(1.,1.),(1.,1.),(1.,1.),(1.,
1.),(1.,1.),(1.,1.),(1.,1.),(1.,1.),(1.,1.),(1.,1.),(1.,1.),(1.,1.),(1.,
1.),(1.,1.),(1.,1.),(1.,1.),(1.,1.),(1.,1.),(1.,1.),(1.,1.),(1.,1.),(1.,
1.),(1.,1.)))
REPRESENTATION_ITEM('')
SURFACE()
);
#92=(
BOUNDED_SURFACE()
B_SPLINE_SURFACE(5,1,((#49020,#49021),(#49022,#49023),(#49024,#49025),(#49026,
#49027),(#49028,#49029),(#49030,#49031),(#49032,#49033),(#49034,#49035),
(#49036,#49037),(#49038,#49039),(#49040,#49041),(#49042,#49043),(#49044,
#49045),(#49046,#49047),(#49048,#49049),(#49050,#49051),(#49052,#49053),
(#49054,#49055),(#49056,#49057),(#49058,#49059),(#49060,#49061),(#49062,
#49063),(#49064,#49065),(#49066,#49067),(#49068,#49069),(#49070,#49071),
(#49072,#49073),(#49074,#49075),(#49076,#49077),(#49078,#49079),(#49080,
#49081),(#49082,#49083),(#49084,#49085),(#49086,#49087),(#49088,#49089),
(#49090,#49091),(#49092,#49093),(#49094,#49095),(#49096,#49097),(#49098,
#49099),(#49100,#49101),(#49102,#49103),(#49104,#49105),(#49106,#49107),
(#49108,#49109),(#49110,#49111),(#49112,#49113),(#49114,#49115),(#49116,
#49117),(#49118,#49119),(#49120,#49121),(#49122,#49123),(#49124,#49125),
(#49126,#49127),(#49128,#49129),(#49130,#49131),(#49132,#49133),(#49134,
#49135),(#49136,#49137),(#49138,#49139),(#49140,#49141),(#49142,#49143),
(#49144,#49145),(#49146,#49147),(#49148,#49149),(#49150,#49151),(#49152,
#49153),(#49154,#49155),(#49156,#49157),(#49158,#49159)),.UNSPECIFIED.,
 .F.,.F.,.F.)
B_SPLINE_SURFACE_WITH_KNOTS((6,1,1,1,1,1,1,1,1,1,1,1,1,1,1,1,1,1,1,1,1,
1,1,1,1,1,1,1,1,1,1,1,1,1,1,1,1,1,1,1,1,1,1,1,1,1,1,1,1,1,1,1,1,1,1,1,1,
1,1,1,1,1,1,1,1,6),(2,2),(-1.,-0.984615384615383,-0.969230769230768,-0.953846153846152,
-0.938461538461537,-0.923076923076922,-0.907692307692306,-0.892307692307691,
-0.876923076923076,-0.86153846153846,-0.846153846153845,-0.83076923076923,
-0.815384615384614,-0.799999999999999,-0.784615384615384,-0.769230769230768,
-0.753846153846153,-0.738461538461538,-0.723076923076922,-0.707692307692307,
-0.692307692307692,-0.676923076923076,-0.661538461538461,-0.646153846153846,
-0.63076923076923,-0.615384615384615,-0.6,-0.584615384615384,-0.569230769230769,
-0.553846153846154,-0.538461538461538,-0.523076923076923,-0.507692307692308,
-0.492307692307692,-0.476923076923077,-0.461538461538462,-0.446153846153846,
-0.430769230769231,-0.415384615384615,-0.4,-0.384615384615385,-0.369230769230769,
-0.353846153846154,-0.338461538461538,-0.323076923076923,-0.307692307692308,
-0.292307692307692,-0.276923076923077,-0.261538461538462,-0.246153846153846,
-0.230769230769231,-0.215384615384615,-0.2,-0.184615384615385,-0.169230769230769,
-0.153846153846154,-0.138461538461538,-0.123076923076923,-0.107692307692308,
-0.0923076923076923,-0.0769230769230769,-0.0615384615384615,-0.0461538461538462,
-0.0307692307692308,-0.0153846153846154,0.),(-1.,1.),.UNSPECIFIED.)
GEOMETRIC_REPRESENTATION_ITEM()
RATIONAL_B_SPLINE_SURFACE(((1.,1.),(1.,1.),(1.,1.),(1.,1.),(1.,1.),(1.,
1.),(1.,1.),(1.,1.),(1.,1.),(1.,1.),(1.,1.),(1.,1.),(1.,1.),(1.,1.),(1.,
1.),(1.,1.),(1.,1.),(1.,1.),(1.,1.),(1.,1.),(1.,1.),(1.,1.),(1.,1.),(1.,
1.),(1.,1.),(1.,1.),(1.,1.),(1.,1.),(1.,1.),(1.,1.),(1.,1.),(1.,1.),(1.,
1.),(1.,1.),(1.,1.),(1.,1.),(1.,1.),(1.,1.),(1.,1.),(1.,1.),(1.,1.),(1.,
1.),(1.,1.),(1.,1.),(1.,1.),(1.,1.),(1.,1.),(1.,1.),(1.,1.),(1.,1.),(1.,
1.),(1.,1.),(1.,1.),(1.,1.),(1.,1.),(1.,1.),(1.,1.),(1.,1.),(1.,1.),(1.,
1.),(1.,1.),(1.,1.),(1.,1.),(1.,1.),(1.,1.),(1.,1.),(1.,1.),(1.,1.),(1.,
1.),(1.,1.)))
REPRESENTATION_ITEM('')
SURFACE()
);
#93=(
BOUNDED_SURFACE()
B_SPLINE_SURFACE(5,1,((#49250,#49251),(#49252,#49253),(#49254,#49255),(#49256,
#49257),(#49258,#49259),(#49260,#49261),(#49262,#49263),(#49264,#49265),
(#49266,#49267),(#49268,#49269),(#49270,#49271),(#49272,#49273),(#49274,
#49275),(#49276,#49277),(#49278,#49279),(#49280,#49281),(#49282,#49283),
(#49284,#49285),(#49286,#49287),(#49288,#49289),(#49290,#49291),(#49292,
#49293),(#49294,#49295),(#49296,#49297),(#49298,#49299),(#49300,#49301),
(#49302,#49303),(#49304,#49305),(#49306,#49307),(#49308,#49309),(#49310,
#49311),(#49312,#49313),(#49314,#49315),(#49316,#49317),(#49318,#49319),
(#49320,#49321),(#49322,#49323),(#49324,#49325),(#49326,#49327),(#49328,
#49329),(#49330,#49331),(#49332,#49333),(#49334,#49335),(#49336,#49337),
(#49338,#49339),(#49340,#49341),(#49342,#49343),(#49344,#49345),(#49346,
#49347),(#49348,#49349),(#49350,#49351),(#49352,#49353),(#49354,#49355),
(#49356,#49357),(#49358,#49359),(#49360,#49361),(#49362,#49363),(#49364,
#49365),(#49366,#49367),(#49368,#49369),(#49370,#49371),(#49372,#49373),
(#49374,#49375),(#49376,#49377),(#49378,#49379),(#49380,#49381),(#49382,
#49383),(#49384,#49385),(#49386,#49387),(#49388,#49389)),.UNSPECIFIED.,
 .F.,.F.,.F.)
B_SPLINE_SURFACE_WITH_KNOTS((6,1,1,1,1,1,1,1,1,1,1,1,1,1,1,1,1,1,1,1,1,
1,1,1,1,1,1,1,1,1,1,1,1,1,1,1,1,1,1,1,1,1,1,1,1,1,1,1,1,1,1,1,1,1,1,1,1,
1,1,1,1,1,1,1,1,6),(2,2),(-1.,-0.984615384615383,-0.969230769230768,-0.953846153846152,
-0.938461538461537,-0.923076923076922,-0.907692307692306,-0.892307692307691,
-0.876923076923076,-0.86153846153846,-0.846153846153845,-0.83076923076923,
-0.815384615384614,-0.799999999999999,-0.784615384615384,-0.769230769230768,
-0.753846153846153,-0.738461538461538,-0.723076923076922,-0.707692307692307,
-0.692307692307692,-0.676923076923076,-0.661538461538461,-0.646153846153846,
-0.63076923076923,-0.615384615384615,-0.6,-0.584615384615384,-0.569230769230769,
-0.553846153846154,-0.538461538461538,-0.523076923076923,-0.507692307692308,
-0.492307692307692,-0.476923076923077,-0.461538461538462,-0.446153846153846,
-0.430769230769231,-0.415384615384615,-0.4,-0.384615384615385,-0.369230769230769,
-0.353846153846154,-0.338461538461538,-0.323076923076923,-0.307692307692308,
-0.292307692307692,-0.276923076923077,-0.261538461538462,-0.246153846153846,
-0.230769230769231,-0.215384615384615,-0.2,-0.184615384615385,-0.169230769230769,
-0.153846153846154,-0.138461538461538,-0.123076923076923,-0.107692307692308,
-0.0923076923076923,-0.0769230769230769,-0.0615384615384615,-0.0461538461538462,
-0.0307692307692308,-0.0153846153846154,0.),(-1.,1.),.UNSPECIFIED.)
GEOMETRIC_REPRESENTATION_ITEM()
RATIONAL_B_SPLINE_SURFACE(((1.,1.),(1.,1.),(1.,1.),(1.,1.),(1.,1.),(1.,
1.),(1.,1.),(1.,1.),(1.,1.),(1.,1.),(1.,1.),(1.,1.),(1.,1.),(1.,1.),(1.,
1.),(1.,1.),(1.,1.),(1.,1.),(1.,1.),(1.,1.),(1.,1.),(1.,1.),(1.,1.),(1.,
1.),(1.,1.),(1.,1.),(1.,1.),(1.,1.),(1.,1.),(1.,1.),(1.,1.),(1.,1.),(1.,
1.),(1.,1.),(1.,1.),(1.,1.),(1.,1.),(1.,1.),(1.,1.),(1.,1.),(1.,1.),(1.,
1.),(1.,1.),(1.,1.),(1.,1.),(1.,1.),(1.,1.),(1.,1.),(1.,1.),(1.,1.),(1.,
1.),(1.,1.),(1.,1.),(1.,1.),(1.,1.),(1.,1.),(1.,1.),(1.,1.),(1.,1.),(1.,
1.),(1.,1.),(1.,1.),(1.,1.),(1.,1.),(1.,1.),(1.,1.),(1.,1.),(1.,1.),(1.,
1.),(1.,1.)))
REPRESENTATION_ITEM('')
SURFACE()
);
#94=(
BOUNDED_SURFACE()
B_SPLINE_SURFACE(5,1,((#49462,#49463),(#49464,#49465),(#49466,#49467),(#49468,
#49469),(#49470,#49471),(#49472,#49473),(#49474,#49475),(#49476,#49477),
(#49478,#49479),(#49480,#49481),(#49482,#49483),(#49484,#49485),(#49486,
#49487),(#49488,#49489),(#49490,#49491),(#49492,#49493),(#49494,#49495),
(#49496,#49497),(#49498,#49499),(#49500,#49501),(#49502,#49503),(#49504,
#49505),(#49506,#49507),(#49508,#49509),(#49510,#49511),(#49512,#49513),
(#49514,#49515),(#49516,#49517),(#49518,#49519),(#49520,#49521),(#49522,
#49523),(#49524,#49525),(#49526,#49527),(#49528,#49529),(#49530,#49531),
(#49532,#49533),(#49534,#49535),(#49536,#49537),(#49538,#49539),(#49540,
#49541),(#49542,#49543),(#49544,#49545),(#49546,#49547),(#49548,#49549),
(#49550,#49551),(#49552,#49553),(#49554,#49555),(#49556,#49557),(#49558,
#49559),(#49560,#49561),(#49562,#49563),(#49564,#49565),(#49566,#49567),
(#49568,#49569),(#49570,#49571),(#49572,#49573),(#49574,#49575),(#49576,
#49577),(#49578,#49579),(#49580,#49581),(#49582,#49583),(#49584,#49585),
(#49586,#49587),(#49588,#49589),(#49590,#49591),(#49592,#49593),(#49594,
#49595),(#49596,#49597),(#49598,#49599),(#49600,#49601)),.UNSPECIFIED.,
 .F.,.F.,.F.)
B_SPLINE_SURFACE_WITH_KNOTS((6,1,1,1,1,1,1,1,1,1,1,1,1,1,1,1,1,1,1,1,1,
1,1,1,1,1,1,1,1,1,1,1,1,1,1,1,1,1,1,1,1,1,1,1,1,1,1,1,1,1,1,1,1,1,1,1,1,
1,1,1,1,1,1,1,1,6),(2,2),(-1.,-0.984615384615383,-0.969230769230768,-0.953846153846152,
-0.938461538461537,-0.923076923076922,-0.907692307692306,-0.892307692307691,
-0.876923076923076,-0.86153846153846,-0.846153846153845,-0.83076923076923,
-0.815384615384614,-0.799999999999999,-0.784615384615384,-0.769230769230768,
-0.753846153846153,-0.738461538461538,-0.723076923076922,-0.707692307692307,
-0.692307692307692,-0.676923076923076,-0.661538461538461,-0.646153846153846,
-0.63076923076923,-0.615384615384615,-0.6,-0.584615384615384,-0.569230769230769,
-0.553846153846154,-0.538461538461538,-0.523076923076923,-0.507692307692308,
-0.492307692307692,-0.476923076923077,-0.461538461538462,-0.446153846153846,
-0.430769230769231,-0.415384615384615,-0.4,-0.384615384615385,-0.369230769230769,
-0.353846153846154,-0.338461538461538,-0.323076923076923,-0.307692307692308,
-0.292307692307692,-0.276923076923077,-0.261538461538462,-0.246153846153846,
-0.230769230769231,-0.215384615384615,-0.2,-0.184615384615385,-0.169230769230769,
-0.153846153846154,-0.138461538461538,-0.123076923076923,-0.107692307692308,
-0.0923076923076923,-0.0769230769230769,-0.0615384615384615,-0.0461538461538462,
-0.0307692307692308,-0.0153846153846154,0.),(-1.,1.),.UNSPECIFIED.)
GEOMETRIC_REPRESENTATION_ITEM()
RATIONAL_B_SPLINE_SURFACE(((1.,1.),(1.,1.),(1.,1.),(1.,1.),(1.,1.),(1.,
1.),(1.,1.),(1.,1.),(1.,1.),(1.,1.),(1.,1.),(1.,1.),(1.,1.),(1.,1.),(1.,
1.),(1.,1.),(1.,1.),(1.,1.),(1.,1.),(1.,1.),(1.,1.),(1.,1.),(1.,1.),(1.,
1.),(1.,1.),(1.,1.),(1.,1.),(1.,1.),(1.,1.),(1.,1.),(1.,1.),(1.,1.),(1.,
1.),(1.,1.),(1.,1.),(1.,1.),(1.,1.),(1.,1.),(1.,1.),(1.,1.),(1.,1.),(1.,
1.),(1.,1.),(1.,1.),(1.,1.),(1.,1.),(1.,1.),(1.,1.),(1.,1.),(1.,1.),(1.,
1.),(1.,1.),(1.,1.),(1.,1.),(1.,1.),(1.,1.),(1.,1.),(1.,1.),(1.,1.),(1.,
1.),(1.,1.),(1.,1.),(1.,1.),(1.,1.),(1.,1.),(1.,1.),(1.,1.),(1.,1.),(1.,
1.),(1.,1.)))
REPRESENTATION_ITEM('')
SURFACE()
);
#95=(
BOUNDED_SURFACE()
B_SPLINE_SURFACE(5,1,((#49692,#49693),(#49694,#49695),(#49696,#49697),(#49698,
#49699),(#49700,#49701),(#49702,#49703),(#49704,#49705),(#49706,#49707),
(#49708,#49709),(#49710,#49711),(#49712,#49713),(#49714,#49715),(#49716,
#49717),(#49718,#49719),(#49720,#49721),(#49722,#49723),(#49724,#49725),
(#49726,#49727),(#49728,#49729),(#49730,#49731),(#49732,#49733),(#49734,
#49735),(#49736,#49737),(#49738,#49739),(#49740,#49741),(#49742,#49743),
(#49744,#49745),(#49746,#49747),(#49748,#49749),(#49750,#49751),(#49752,
#49753),(#49754,#49755),(#49756,#49757),(#49758,#49759),(#49760,#49761),
(#49762,#49763),(#49764,#49765),(#49766,#49767),(#49768,#49769),(#49770,
#49771),(#49772,#49773),(#49774,#49775),(#49776,#49777),(#49778,#49779),
(#49780,#49781),(#49782,#49783),(#49784,#49785),(#49786,#49787),(#49788,
#49789),(#49790,#49791),(#49792,#49793),(#49794,#49795),(#49796,#49797),
(#49798,#49799),(#49800,#49801),(#49802,#49803),(#49804,#49805),(#49806,
#49807),(#49808,#49809),(#49810,#49811),(#49812,#49813),(#49814,#49815),
(#49816,#49817),(#49818,#49819),(#49820,#49821),(#49822,#49823),(#49824,
#49825),(#49826,#49827),(#49828,#49829),(#49830,#49831)),.UNSPECIFIED.,
 .F.,.F.,.F.)
B_SPLINE_SURFACE_WITH_KNOTS((6,1,1,1,1,1,1,1,1,1,1,1,1,1,1,1,1,1,1,1,1,
1,1,1,1,1,1,1,1,1,1,1,1,1,1,1,1,1,1,1,1,1,1,1,1,1,1,1,1,1,1,1,1,1,1,1,1,
1,1,1,1,1,1,1,1,6),(2,2),(-1.,-0.984615384615383,-0.969230769230768,-0.953846153846152,
-0.938461538461537,-0.923076923076922,-0.907692307692306,-0.892307692307691,
-0.876923076923076,-0.86153846153846,-0.846153846153845,-0.83076923076923,
-0.815384615384614,-0.799999999999999,-0.784615384615384,-0.769230769230768,
-0.753846153846153,-0.738461538461538,-0.723076923076922,-0.707692307692307,
-0.692307692307692,-0.676923076923076,-0.661538461538461,-0.646153846153846,
-0.63076923076923,-0.615384615384615,-0.6,-0.584615384615384,-0.569230769230769,
-0.553846153846154,-0.538461538461538,-0.523076923076923,-0.507692307692308,
-0.492307692307692,-0.476923076923077,-0.461538461538462,-0.446153846153846,
-0.430769230769231,-0.415384615384615,-0.4,-0.384615384615385,-0.369230769230769,
-0.353846153846154,-0.338461538461538,-0.323076923076923,-0.307692307692308,
-0.292307692307692,-0.276923076923077,-0.261538461538462,-0.246153846153846,
-0.230769230769231,-0.215384615384615,-0.2,-0.184615384615385,-0.169230769230769,
-0.153846153846154,-0.138461538461538,-0.123076923076923,-0.107692307692308,
-0.0923076923076923,-0.0769230769230769,-0.0615384615384615,-0.0461538461538462,
-0.0307692307692308,-0.0153846153846154,0.),(-1.,1.),.UNSPECIFIED.)
GEOMETRIC_REPRESENTATION_ITEM()
RATIONAL_B_SPLINE_SURFACE(((1.,1.),(1.,1.),(1.,1.),(1.,1.),(1.,1.),(1.,
1.),(1.,1.),(1.,1.),(1.,1.),(1.,1.),(1.,1.),(1.,1.),(1.,1.),(1.,1.),(1.,
1.),(1.,1.),(1.,1.),(1.,1.),(1.,1.),(1.,1.),(1.,1.),(1.,1.),(1.,1.),(1.,
1.),(1.,1.),(1.,1.),(1.,1.),(1.,1.),(1.,1.),(1.,1.),(1.,1.),(1.,1.),(1.,
1.),(1.,1.),(1.,1.),(1.,1.),(1.,1.),(1.,1.),(1.,1.),(1.,1.),(1.,1.),(1.,
1.),(1.,1.),(1.,1.),(1.,1.),(1.,1.),(1.,1.),(1.,1.),(1.,1.),(1.,1.),(1.,
1.),(1.,1.),(1.,1.),(1.,1.),(1.,1.),(1.,1.),(1.,1.),(1.,1.),(1.,1.),(1.,
1.),(1.,1.),(1.,1.),(1.,1.),(1.,1.),(1.,1.),(1.,1.),(1.,1.),(1.,1.),(1.,
1.),(1.,1.)))
REPRESENTATION_ITEM('')
SURFACE()
);
#96=(
BOUNDED_SURFACE()
B_SPLINE_SURFACE(5,1,((#49904,#49905),(#49906,#49907),(#49908,#49909),(#49910,
#49911),(#49912,#49913),(#49914,#49915),(#49916,#49917),(#49918,#49919),
(#49920,#49921),(#49922,#49923),(#49924,#49925),(#49926,#49927),(#49928,
#49929),(#49930,#49931),(#49932,#49933),(#49934,#49935),(#49936,#49937),
(#49938,#49939),(#49940,#49941),(#49942,#49943),(#49944,#49945),(#49946,
#49947),(#49948,#49949),(#49950,#49951),(#49952,#49953),(#49954,#49955),
(#49956,#49957),(#49958,#49959),(#49960,#49961),(#49962,#49963),(#49964,
#49965),(#49966,#49967),(#49968,#49969),(#49970,#49971),(#49972,#49973),
(#49974,#49975),(#49976,#49977),(#49978,#49979),(#49980,#49981),(#49982,
#49983),(#49984,#49985),(#49986,#49987),(#49988,#49989),(#49990,#49991),
(#49992,#49993),(#49994,#49995),(#49996,#49997),(#49998,#49999),(#50000,
#50001),(#50002,#50003),(#50004,#50005),(#50006,#50007),(#50008,#50009),
(#50010,#50011),(#50012,#50013),(#50014,#50015),(#50016,#50017),(#50018,
#50019),(#50020,#50021),(#50022,#50023),(#50024,#50025),(#50026,#50027),
(#50028,#50029),(#50030,#50031),(#50032,#50033),(#50034,#50035),(#50036,
#50037),(#50038,#50039),(#50040,#50041),(#50042,#50043)),.UNSPECIFIED.,
 .F.,.F.,.F.)
B_SPLINE_SURFACE_WITH_KNOTS((6,1,1,1,1,1,1,1,1,1,1,1,1,1,1,1,1,1,1,1,1,
1,1,1,1,1,1,1,1,1,1,1,1,1,1,1,1,1,1,1,1,1,1,1,1,1,1,1,1,1,1,1,1,1,1,1,1,
1,1,1,1,1,1,1,1,6),(2,2),(-1.,-0.984615384615383,-0.969230769230768,-0.953846153846152,
-0.938461538461537,-0.923076923076922,-0.907692307692306,-0.892307692307691,
-0.876923076923076,-0.86153846153846,-0.846153846153845,-0.83076923076923,
-0.815384615384614,-0.799999999999999,-0.784615384615384,-0.769230769230768,
-0.753846153846153,-0.738461538461538,-0.723076923076922,-0.707692307692307,
-0.692307692307692,-0.676923076923076,-0.661538461538461,-0.646153846153846,
-0.63076923076923,-0.615384615384615,-0.6,-0.584615384615384,-0.569230769230769,
-0.553846153846154,-0.538461538461538,-0.523076923076923,-0.507692307692308,
-0.492307692307692,-0.476923076923077,-0.461538461538462,-0.446153846153846,
-0.430769230769231,-0.415384615384615,-0.4,-0.384615384615385,-0.369230769230769,
-0.353846153846154,-0.338461538461538,-0.323076923076923,-0.307692307692308,
-0.292307692307692,-0.276923076923077,-0.261538461538462,-0.246153846153846,
-0.230769230769231,-0.215384615384615,-0.2,-0.184615384615385,-0.169230769230769,
-0.153846153846154,-0.138461538461538,-0.123076923076923,-0.107692307692308,
-0.0923076923076923,-0.0769230769230769,-0.0615384615384615,-0.0461538461538462,
-0.0307692307692308,-0.0153846153846154,0.),(-1.,1.),.UNSPECIFIED.)
GEOMETRIC_REPRESENTATION_ITEM()
RATIONAL_B_SPLINE_SURFACE(((1.,1.),(1.,1.),(1.,1.),(1.,1.),(1.,1.),(1.,
1.),(1.,1.),(1.,1.),(1.,1.),(1.,1.),(1.,1.),(1.,1.),(1.,1.),(1.,1.),(1.,
1.),(1.,1.),(1.,1.),(1.,1.),(1.,1.),(1.,1.),(1.,1.),(1.,1.),(1.,1.),(1.,
1.),(1.,1.),(1.,1.),(1.,1.),(1.,1.),(1.,1.),(1.,1.),(1.,1.),(1.,1.),(1.,
1.),(1.,1.),(1.,1.),(1.,1.),(1.,1.),(1.,1.),(1.,1.),(1.,1.),(1.,1.),(1.,
1.),(1.,1.),(1.,1.),(1.,1.),(1.,1.),(1.,1.),(1.,1.),(1.,1.),(1.,1.),(1.,
1.),(1.,1.),(1.,1.),(1.,1.),(1.,1.),(1.,1.),(1.,1.),(1.,1.),(1.,1.),(1.,
1.),(1.,1.),(1.,1.),(1.,1.),(1.,1.),(1.,1.),(1.,1.),(1.,1.),(1.,1.),(1.,
1.),(1.,1.)))
REPRESENTATION_ITEM('')
SURFACE()
);
#97=(
BOUNDED_SURFACE()
B_SPLINE_SURFACE(5,1,((#50134,#50135),(#50136,#50137),(#50138,#50139),(#50140,
#50141),(#50142,#50143),(#50144,#50145),(#50146,#50147),(#50148,#50149),
(#50150,#50151),(#50152,#50153),(#50154,#50155),(#50156,#50157),(#50158,
#50159),(#50160,#50161),(#50162,#50163),(#50164,#50165),(#50166,#50167),
(#50168,#50169),(#50170,#50171),(#50172,#50173),(#50174,#50175),(#50176,
#50177),(#50178,#50179),(#50180,#50181),(#50182,#50183),(#50184,#50185),
(#50186,#50187),(#50188,#50189),(#50190,#50191),(#50192,#50193),(#50194,
#50195),(#50196,#50197),(#50198,#50199),(#50200,#50201),(#50202,#50203),
(#50204,#50205),(#50206,#50207),(#50208,#50209),(#50210,#50211),(#50212,
#50213),(#50214,#50215),(#50216,#50217),(#50218,#50219),(#50220,#50221),
(#50222,#50223),(#50224,#50225),(#50226,#50227),(#50228,#50229),(#50230,
#50231),(#50232,#50233),(#50234,#50235),(#50236,#50237),(#50238,#50239),
(#50240,#50241),(#50242,#50243),(#50244,#50245),(#50246,#50247),(#50248,
#50249),(#50250,#50251),(#50252,#50253),(#50254,#50255),(#50256,#50257),
(#50258,#50259),(#50260,#50261),(#50262,#50263),(#50264,#50265),(#50266,
#50267),(#50268,#50269),(#50270,#50271),(#50272,#50273)),.UNSPECIFIED.,
 .F.,.F.,.F.)
B_SPLINE_SURFACE_WITH_KNOTS((6,1,1,1,1,1,1,1,1,1,1,1,1,1,1,1,1,1,1,1,1,
1,1,1,1,1,1,1,1,1,1,1,1,1,1,1,1,1,1,1,1,1,1,1,1,1,1,1,1,1,1,1,1,1,1,1,1,
1,1,1,1,1,1,1,1,6),(2,2),(-1.,-0.984615384615383,-0.969230769230768,-0.953846153846152,
-0.938461538461537,-0.923076923076922,-0.907692307692306,-0.892307692307691,
-0.876923076923076,-0.86153846153846,-0.846153846153845,-0.83076923076923,
-0.815384615384614,-0.799999999999999,-0.784615384615384,-0.769230769230768,
-0.753846153846153,-0.738461538461538,-0.723076923076922,-0.707692307692307,
-0.692307692307692,-0.676923076923076,-0.661538461538461,-0.646153846153846,
-0.63076923076923,-0.615384615384615,-0.6,-0.584615384615384,-0.569230769230769,
-0.553846153846154,-0.538461538461538,-0.523076923076923,-0.507692307692308,
-0.492307692307692,-0.476923076923077,-0.461538461538462,-0.446153846153846,
-0.430769230769231,-0.415384615384615,-0.4,-0.384615384615385,-0.369230769230769,
-0.353846153846154,-0.338461538461538,-0.323076923076923,-0.307692307692308,
-0.292307692307692,-0.276923076923077,-0.261538461538462,-0.246153846153846,
-0.230769230769231,-0.215384615384615,-0.2,-0.184615384615385,-0.169230769230769,
-0.153846153846154,-0.138461538461538,-0.123076923076923,-0.107692307692308,
-0.0923076923076923,-0.0769230769230769,-0.0615384615384615,-0.0461538461538462,
-0.0307692307692308,-0.0153846153846154,0.),(-1.,1.),.UNSPECIFIED.)
GEOMETRIC_REPRESENTATION_ITEM()
RATIONAL_B_SPLINE_SURFACE(((1.,1.),(1.,1.),(1.,1.),(1.,1.),(1.,1.),(1.,
1.),(1.,1.),(1.,1.),(1.,1.),(1.,1.),(1.,1.),(1.,1.),(1.,1.),(1.,1.),(1.,
1.),(1.,1.),(1.,1.),(1.,1.),(1.,1.),(1.,1.),(1.,1.),(1.,1.),(1.,1.),(1.,
1.),(1.,1.),(1.,1.),(1.,1.),(1.,1.),(1.,1.),(1.,1.),(1.,1.),(1.,1.),(1.,
1.),(1.,1.),(1.,1.),(1.,1.),(1.,1.),(1.,1.),(1.,1.),(1.,1.),(1.,1.),(1.,
1.),(1.,1.),(1.,1.),(1.,1.),(1.,1.),(1.,1.),(1.,1.),(1.,1.),(1.,1.),(1.,
1.),(1.,1.),(1.,1.),(1.,1.),(1.,1.),(1.,1.),(1.,1.),(1.,1.),(1.,1.),(1.,
1.),(1.,1.),(1.,1.),(1.,1.),(1.,1.),(1.,1.),(1.,1.),(1.,1.),(1.,1.),(1.,
1.),(1.,1.)))
REPRESENTATION_ITEM('')
SURFACE()
);
#98=(
BOUNDED_SURFACE()
B_SPLINE_SURFACE(5,1,((#50346,#50347),(#50348,#50349),(#50350,#50351),(#50352,
#50353),(#50354,#50355),(#50356,#50357),(#50358,#50359),(#50360,#50361),
(#50362,#50363),(#50364,#50365),(#50366,#50367),(#50368,#50369),(#50370,
#50371),(#50372,#50373),(#50374,#50375),(#50376,#50377),(#50378,#50379),
(#50380,#50381),(#50382,#50383),(#50384,#50385),(#50386,#50387),(#50388,
#50389),(#50390,#50391),(#50392,#50393),(#50394,#50395),(#50396,#50397),
(#50398,#50399),(#50400,#50401),(#50402,#50403),(#50404,#50405),(#50406,
#50407),(#50408,#50409),(#50410,#50411),(#50412,#50413),(#50414,#50415),
(#50416,#50417),(#50418,#50419),(#50420,#50421),(#50422,#50423),(#50424,
#50425),(#50426,#50427),(#50428,#50429),(#50430,#50431),(#50432,#50433),
(#50434,#50435),(#50436,#50437),(#50438,#50439),(#50440,#50441),(#50442,
#50443),(#50444,#50445),(#50446,#50447),(#50448,#50449),(#50450,#50451),
(#50452,#50453),(#50454,#50455),(#50456,#50457),(#50458,#50459),(#50460,
#50461),(#50462,#50463),(#50464,#50465),(#50466,#50467),(#50468,#50469),
(#50470,#50471),(#50472,#50473),(#50474,#50475),(#50476,#50477),(#50478,
#50479),(#50480,#50481),(#50482,#50483),(#50484,#50485)),.UNSPECIFIED.,
 .F.,.F.,.F.)
B_SPLINE_SURFACE_WITH_KNOTS((6,1,1,1,1,1,1,1,1,1,1,1,1,1,1,1,1,1,1,1,1,
1,1,1,1,1,1,1,1,1,1,1,1,1,1,1,1,1,1,1,1,1,1,1,1,1,1,1,1,1,1,1,1,1,1,1,1,
1,1,1,1,1,1,1,1,6),(2,2),(-1.,-0.984615384615383,-0.969230769230768,-0.953846153846152,
-0.938461538461537,-0.923076923076922,-0.907692307692306,-0.892307692307691,
-0.876923076923076,-0.86153846153846,-0.846153846153845,-0.83076923076923,
-0.815384615384614,-0.799999999999999,-0.784615384615384,-0.769230769230768,
-0.753846153846153,-0.738461538461538,-0.723076923076922,-0.707692307692307,
-0.692307692307692,-0.676923076923076,-0.661538461538461,-0.646153846153846,
-0.63076923076923,-0.615384615384615,-0.6,-0.584615384615384,-0.569230769230769,
-0.553846153846154,-0.538461538461538,-0.523076923076923,-0.507692307692308,
-0.492307692307692,-0.476923076923077,-0.461538461538462,-0.446153846153846,
-0.430769230769231,-0.415384615384615,-0.4,-0.384615384615385,-0.369230769230769,
-0.353846153846154,-0.338461538461538,-0.323076923076923,-0.307692307692308,
-0.292307692307692,-0.276923076923077,-0.261538461538462,-0.246153846153846,
-0.230769230769231,-0.215384615384615,-0.2,-0.184615384615385,-0.169230769230769,
-0.153846153846154,-0.138461538461538,-0.123076923076923,-0.107692307692308,
-0.0923076923076923,-0.0769230769230769,-0.0615384615384615,-0.0461538461538462,
-0.0307692307692308,-0.0153846153846154,0.),(-1.,1.),.UNSPECIFIED.)
GEOMETRIC_REPRESENTATION_ITEM()
RATIONAL_B_SPLINE_SURFACE(((1.,1.),(1.,1.),(1.,1.),(1.,1.),(1.,1.),(1.,
1.),(1.,1.),(1.,1.),(1.,1.),(1.,1.),(1.,1.),(1.,1.),(1.,1.),(1.,1.),(1.,
1.),(1.,1.),(1.,1.),(1.,1.),(1.,1.),(1.,1.),(1.,1.),(1.,1.),(1.,1.),(1.,
1.),(1.,1.),(1.,1.),(1.,1.),(1.,1.),(1.,1.),(1.,1.),(1.,1.),(1.,1.),(1.,
1.),(1.,1.),(1.,1.),(1.,1.),(1.,1.),(1.,1.),(1.,1.),(1.,1.),(1.,1.),(1.,
1.),(1.,1.),(1.,1.),(1.,1.),(1.,1.),(1.,1.),(1.,1.),(1.,1.),(1.,1.),(1.,
1.),(1.,1.),(1.,1.),(1.,1.),(1.,1.),(1.,1.),(1.,1.),(1.,1.),(1.,1.),(1.,
1.),(1.,1.),(1.,1.),(1.,1.),(1.,1.),(1.,1.),(1.,1.),(1.,1.),(1.,1.),(1.,
1.),(1.,1.)))
REPRESENTATION_ITEM('')
SURFACE()
);
#99=(
BOUNDED_SURFACE()
B_SPLINE_SURFACE(5,1,((#50576,#50577),(#50578,#50579),(#50580,#50581),(#50582,
#50583),(#50584,#50585),(#50586,#50587),(#50588,#50589),(#50590,#50591),
(#50592,#50593),(#50594,#50595),(#50596,#50597),(#50598,#50599),(#50600,
#50601),(#50602,#50603),(#50604,#50605),(#50606,#50607),(#50608,#50609),
(#50610,#50611),(#50612,#50613),(#50614,#50615),(#50616,#50617),(#50618,
#50619),(#50620,#50621),(#50622,#50623),(#50624,#50625),(#50626,#50627),
(#50628,#50629),(#50630,#50631),(#50632,#50633),(#50634,#50635),(#50636,
#50637),(#50638,#50639),(#50640,#50641),(#50642,#50643),(#50644,#50645),
(#50646,#50647),(#50648,#50649),(#50650,#50651),(#50652,#50653),(#50654,
#50655),(#50656,#50657),(#50658,#50659),(#50660,#50661),(#50662,#50663),
(#50664,#50665),(#50666,#50667),(#50668,#50669),(#50670,#50671),(#50672,
#50673),(#50674,#50675),(#50676,#50677),(#50678,#50679),(#50680,#50681),
(#50682,#50683),(#50684,#50685),(#50686,#50687),(#50688,#50689),(#50690,
#50691),(#50692,#50693),(#50694,#50695),(#50696,#50697),(#50698,#50699),
(#50700,#50701),(#50702,#50703),(#50704,#50705),(#50706,#50707),(#50708,
#50709),(#50710,#50711),(#50712,#50713),(#50714,#50715)),.UNSPECIFIED.,
 .F.,.F.,.F.)
B_SPLINE_SURFACE_WITH_KNOTS((6,1,1,1,1,1,1,1,1,1,1,1,1,1,1,1,1,1,1,1,1,
1,1,1,1,1,1,1,1,1,1,1,1,1,1,1,1,1,1,1,1,1,1,1,1,1,1,1,1,1,1,1,1,1,1,1,1,
1,1,1,1,1,1,1,1,6),(2,2),(-1.,-0.984615384615383,-0.969230769230768,-0.953846153846152,
-0.938461538461537,-0.923076923076922,-0.907692307692306,-0.892307692307691,
-0.876923076923076,-0.86153846153846,-0.846153846153845,-0.83076923076923,
-0.815384615384614,-0.799999999999999,-0.784615384615384,-0.769230769230768,
-0.753846153846153,-0.738461538461538,-0.723076923076922,-0.707692307692307,
-0.692307692307692,-0.676923076923076,-0.661538461538461,-0.646153846153846,
-0.63076923076923,-0.615384615384615,-0.6,-0.584615384615384,-0.569230769230769,
-0.553846153846154,-0.538461538461538,-0.523076923076923,-0.507692307692308,
-0.492307692307692,-0.476923076923077,-0.461538461538462,-0.446153846153846,
-0.430769230769231,-0.415384615384615,-0.4,-0.384615384615385,-0.369230769230769,
-0.353846153846154,-0.338461538461538,-0.323076923076923,-0.307692307692308,
-0.292307692307692,-0.276923076923077,-0.261538461538462,-0.246153846153846,
-0.230769230769231,-0.215384615384615,-0.2,-0.184615384615385,-0.169230769230769,
-0.153846153846154,-0.138461538461538,-0.123076923076923,-0.107692307692308,
-0.0923076923076923,-0.0769230769230769,-0.0615384615384615,-0.0461538461538462,
-0.0307692307692308,-0.0153846153846154,0.),(-1.,1.),.UNSPECIFIED.)
GEOMETRIC_REPRESENTATION_ITEM()
RATIONAL_B_SPLINE_SURFACE(((1.,1.),(1.,1.),(1.,1.),(1.,1.),(1.,1.),(1.,
1.),(1.,1.),(1.,1.),(1.,1.),(1.,1.),(1.,1.),(1.,1.),(1.,1.),(1.,1.),(1.,
1.),(1.,1.),(1.,1.),(1.,1.),(1.,1.),(1.,1.),(1.,1.),(1.,1.),(1.,1.),(1.,
1.),(1.,1.),(1.,1.),(1.,1.),(1.,1.),(1.,1.),(1.,1.),(1.,1.),(1.,1.),(1.,
1.),(1.,1.),(1.,1.),(1.,1.),(1.,1.),(1.,1.),(1.,1.),(1.,1.),(1.,1.),(1.,
1.),(1.,1.),(1.,1.),(1.,1.),(1.,1.),(1.,1.),(1.,1.),(1.,1.),(1.,1.),(1.,
1.),(1.,1.),(1.,1.),(1.,1.),(1.,1.),(1.,1.),(1.,1.),(1.,1.),(1.,1.),(1.,
1.),(1.,1.),(1.,1.),(1.,1.),(1.,1.),(1.,1.),(1.,1.),(1.,1.),(1.,1.),(1.,
1.),(1.,1.)))
REPRESENTATION_ITEM('')
SURFACE()
);
#100=(
BOUNDED_SURFACE()
B_SPLINE_SURFACE(5,1,((#50788,#50789),(#50790,#50791),(#50792,#50793),(#50794,
#50795),(#50796,#50797),(#50798,#50799),(#50800,#50801),(#50802,#50803),
(#50804,#50805),(#50806,#50807),(#50808,#50809),(#50810,#50811),(#50812,
#50813),(#50814,#50815),(#50816,#50817),(#50818,#50819),(#50820,#50821),
(#50822,#50823),(#50824,#50825),(#50826,#50827),(#50828,#50829),(#50830,
#50831),(#50832,#50833),(#50834,#50835),(#50836,#50837),(#50838,#50839),
(#50840,#50841),(#50842,#50843),(#50844,#50845),(#50846,#50847),(#50848,
#50849),(#50850,#50851),(#50852,#50853),(#50854,#50855),(#50856,#50857),
(#50858,#50859),(#50860,#50861),(#50862,#50863),(#50864,#50865),(#50866,
#50867),(#50868,#50869),(#50870,#50871),(#50872,#50873),(#50874,#50875),
(#50876,#50877),(#50878,#50879),(#50880,#50881),(#50882,#50883),(#50884,
#50885),(#50886,#50887),(#50888,#50889),(#50890,#50891),(#50892,#50893),
(#50894,#50895),(#50896,#50897),(#50898,#50899),(#50900,#50901),(#50902,
#50903),(#50904,#50905),(#50906,#50907),(#50908,#50909),(#50910,#50911),
(#50912,#50913),(#50914,#50915),(#50916,#50917),(#50918,#50919),(#50920,
#50921),(#50922,#50923),(#50924,#50925),(#50926,#50927)),.UNSPECIFIED.,
 .F.,.F.,.F.)
B_SPLINE_SURFACE_WITH_KNOTS((6,1,1,1,1,1,1,1,1,1,1,1,1,1,1,1,1,1,1,1,1,
1,1,1,1,1,1,1,1,1,1,1,1,1,1,1,1,1,1,1,1,1,1,1,1,1,1,1,1,1,1,1,1,1,1,1,1,
1,1,1,1,1,1,1,1,6),(2,2),(-1.,-0.984615384615383,-0.969230769230768,-0.953846153846152,
-0.938461538461537,-0.923076923076922,-0.907692307692306,-0.892307692307691,
-0.876923076923076,-0.86153846153846,-0.846153846153845,-0.83076923076923,
-0.815384615384614,-0.799999999999999,-0.784615384615384,-0.769230769230768,
-0.753846153846153,-0.738461538461538,-0.723076923076922,-0.707692307692307,
-0.692307692307692,-0.676923076923076,-0.661538461538461,-0.646153846153846,
-0.63076923076923,-0.615384615384615,-0.6,-0.584615384615384,-0.569230769230769,
-0.553846153846154,-0.538461538461538,-0.523076923076923,-0.507692307692308,
-0.492307692307692,-0.476923076923077,-0.461538461538462,-0.446153846153846,
-0.430769230769231,-0.415384615384615,-0.4,-0.384615384615385,-0.369230769230769,
-0.353846153846154,-0.338461538461538,-0.323076923076923,-0.307692307692308,
-0.292307692307692,-0.276923076923077,-0.261538461538462,-0.246153846153846,
-0.230769230769231,-0.215384615384615,-0.2,-0.184615384615385,-0.169230769230769,
-0.153846153846154,-0.138461538461538,-0.123076923076923,-0.107692307692308,
-0.0923076923076923,-0.0769230769230769,-0.0615384615384615,-0.0461538461538462,
-0.0307692307692308,-0.0153846153846154,0.),(-1.,1.),.UNSPECIFIED.)
GEOMETRIC_REPRESENTATION_ITEM()
RATIONAL_B_SPLINE_SURFACE(((1.,1.),(1.,1.),(1.,1.),(1.,1.),(1.,1.),(1.,
1.),(1.,1.),(1.,1.),(1.,1.),(1.,1.),(1.,1.),(1.,1.),(1.,1.),(1.,1.),(1.,
1.),(1.,1.),(1.,1.),(1.,1.),(1.,1.),(1.,1.),(1.,1.),(1.,1.),(1.,1.),(1.,
1.),(1.,1.),(1.,1.),(1.,1.),(1.,1.),(1.,1.),(1.,1.),(1.,1.),(1.,1.),(1.,
1.),(1.,1.),(1.,1.),(1.,1.),(1.,1.),(1.,1.),(1.,1.),(1.,1.),(1.,1.),(1.,
1.),(1.,1.),(1.,1.),(1.,1.),(1.,1.),(1.,1.),(1.,1.),(1.,1.),(1.,1.),(1.,
1.),(1.,1.),(1.,1.),(1.,1.),(1.,1.),(1.,1.),(1.,1.),(1.,1.),(1.,1.),(1.,
1.),(1.,1.),(1.,1.),(1.,1.),(1.,1.),(1.,1.),(1.,1.),(1.,1.),(1.,1.),(1.,
1.),(1.,1.)))
REPRESENTATION_ITEM('')
SURFACE()
);
#101=(
BOUNDED_SURFACE()
B_SPLINE_SURFACE(5,1,((#51018,#51019),(#51020,#51021),(#51022,#51023),(#51024,
#51025),(#51026,#51027),(#51028,#51029),(#51030,#51031),(#51032,#51033),
(#51034,#51035),(#51036,#51037),(#51038,#51039),(#51040,#51041),(#51042,
#51043),(#51044,#51045),(#51046,#51047),(#51048,#51049),(#51050,#51051),
(#51052,#51053),(#51054,#51055),(#51056,#51057),(#51058,#51059),(#51060,
#51061),(#51062,#51063),(#51064,#51065),(#51066,#51067),(#51068,#51069),
(#51070,#51071),(#51072,#51073),(#51074,#51075),(#51076,#51077),(#51078,
#51079),(#51080,#51081),(#51082,#51083),(#51084,#51085),(#51086,#51087),
(#51088,#51089),(#51090,#51091),(#51092,#51093),(#51094,#51095),(#51096,
#51097),(#51098,#51099),(#51100,#51101),(#51102,#51103),(#51104,#51105),
(#51106,#51107),(#51108,#51109),(#51110,#51111),(#51112,#51113),(#51114,
#51115),(#51116,#51117),(#51118,#51119),(#51120,#51121),(#51122,#51123),
(#51124,#51125),(#51126,#51127),(#51128,#51129),(#51130,#51131),(#51132,
#51133),(#51134,#51135),(#51136,#51137),(#51138,#51139),(#51140,#51141),
(#51142,#51143),(#51144,#51145),(#51146,#51147),(#51148,#51149),(#51150,
#51151),(#51152,#51153),(#51154,#51155),(#51156,#51157)),.UNSPECIFIED.,
 .F.,.F.,.F.)
B_SPLINE_SURFACE_WITH_KNOTS((6,1,1,1,1,1,1,1,1,1,1,1,1,1,1,1,1,1,1,1,1,
1,1,1,1,1,1,1,1,1,1,1,1,1,1,1,1,1,1,1,1,1,1,1,1,1,1,1,1,1,1,1,1,1,1,1,1,
1,1,1,1,1,1,1,1,6),(2,2),(-1.,-0.984615384615383,-0.969230769230768,-0.953846153846152,
-0.938461538461537,-0.923076923076922,-0.907692307692306,-0.892307692307691,
-0.876923076923076,-0.86153846153846,-0.846153846153845,-0.83076923076923,
-0.815384615384614,-0.799999999999999,-0.784615384615384,-0.769230769230768,
-0.753846153846153,-0.738461538461538,-0.723076923076922,-0.707692307692307,
-0.692307692307692,-0.676923076923076,-0.661538461538461,-0.646153846153846,
-0.63076923076923,-0.615384615384615,-0.6,-0.584615384615384,-0.569230769230769,
-0.553846153846154,-0.538461538461538,-0.523076923076923,-0.507692307692308,
-0.492307692307692,-0.476923076923077,-0.461538461538462,-0.446153846153846,
-0.430769230769231,-0.415384615384615,-0.4,-0.384615384615385,-0.369230769230769,
-0.353846153846154,-0.338461538461538,-0.323076923076923,-0.307692307692308,
-0.292307692307692,-0.276923076923077,-0.261538461538462,-0.246153846153846,
-0.230769230769231,-0.215384615384615,-0.2,-0.184615384615385,-0.169230769230769,
-0.153846153846154,-0.138461538461538,-0.123076923076923,-0.107692307692308,
-0.0923076923076923,-0.0769230769230769,-0.0615384615384615,-0.0461538461538462,
-0.0307692307692308,-0.0153846153846154,0.),(-1.,1.),.UNSPECIFIED.)
GEOMETRIC_REPRESENTATION_ITEM()
RATIONAL_B_SPLINE_SURFACE(((1.,1.),(1.,1.),(1.,1.),(1.,1.),(1.,1.),(1.,
1.),(1.,1.),(1.,1.),(1.,1.),(1.,1.),(1.,1.),(1.,1.),(1.,1.),(1.,1.),(1.,
1.),(1.,1.),(1.,1.),(1.,1.),(1.,1.),(1.,1.),(1.,1.),(1.,1.),(1.,1.),(1.,
1.),(1.,1.),(1.,1.),(1.,1.),(1.,1.),(1.,1.),(1.,1.),(1.,1.),(1.,1.),(1.,
1.),(1.,1.),(1.,1.),(1.,1.),(1.,1.),(1.,1.),(1.,1.),(1.,1.),(1.,1.),(1.,
1.),(1.,1.),(1.,1.),(1.,1.),(1.,1.),(1.,1.),(1.,1.),(1.,1.),(1.,1.),(1.,
1.),(1.,1.),(1.,1.),(1.,1.),(1.,1.),(1.,1.),(1.,1.),(1.,1.),(1.,1.),(1.,
1.),(1.,1.),(1.,1.),(1.,1.),(1.,1.),(1.,1.),(1.,1.),(1.,1.),(1.,1.),(1.,
1.),(1.,1.)))
REPRESENTATION_ITEM('')
SURFACE()
);
#102=(
BOUNDED_SURFACE()
B_SPLINE_SURFACE(5,1,((#51230,#51231),(#51232,#51233),(#51234,#51235),(#51236,
#51237),(#51238,#51239),(#51240,#51241),(#51242,#51243),(#51244,#51245),
(#51246,#51247),(#51248,#51249),(#51250,#51251),(#51252,#51253),(#51254,
#51255),(#51256,#51257),(#51258,#51259),(#51260,#51261),(#51262,#51263),
(#51264,#51265),(#51266,#51267),(#51268,#51269),(#51270,#51271),(#51272,
#51273),(#51274,#51275),(#51276,#51277),(#51278,#51279),(#51280,#51281),
(#51282,#51283),(#51284,#51285),(#51286,#51287),(#51288,#51289),(#51290,
#51291),(#51292,#51293),(#51294,#51295),(#51296,#51297),(#51298,#51299),
(#51300,#51301),(#51302,#51303),(#51304,#51305),(#51306,#51307),(#51308,
#51309),(#51310,#51311),(#51312,#51313),(#51314,#51315),(#51316,#51317),
(#51318,#51319),(#51320,#51321),(#51322,#51323),(#51324,#51325),(#51326,
#51327),(#51328,#51329),(#51330,#51331),(#51332,#51333),(#51334,#51335),
(#51336,#51337),(#51338,#51339),(#51340,#51341),(#51342,#51343),(#51344,
#51345),(#51346,#51347),(#51348,#51349),(#51350,#51351),(#51352,#51353),
(#51354,#51355),(#51356,#51357),(#51358,#51359),(#51360,#51361),(#51362,
#51363),(#51364,#51365),(#51366,#51367),(#51368,#51369)),.UNSPECIFIED.,
 .F.,.F.,.F.)
B_SPLINE_SURFACE_WITH_KNOTS((6,1,1,1,1,1,1,1,1,1,1,1,1,1,1,1,1,1,1,1,1,
1,1,1,1,1,1,1,1,1,1,1,1,1,1,1,1,1,1,1,1,1,1,1,1,1,1,1,1,1,1,1,1,1,1,1,1,
1,1,1,1,1,1,1,1,6),(2,2),(-1.,-0.984615384615383,-0.969230769230768,-0.953846153846152,
-0.938461538461537,-0.923076923076922,-0.907692307692306,-0.892307692307691,
-0.876923076923076,-0.86153846153846,-0.846153846153845,-0.83076923076923,
-0.815384615384614,-0.799999999999999,-0.784615384615384,-0.769230769230768,
-0.753846153846153,-0.738461538461538,-0.723076923076922,-0.707692307692307,
-0.692307692307692,-0.676923076923076,-0.661538461538461,-0.646153846153846,
-0.63076923076923,-0.615384615384615,-0.6,-0.584615384615384,-0.569230769230769,
-0.553846153846154,-0.538461538461538,-0.523076923076923,-0.507692307692308,
-0.492307692307692,-0.476923076923077,-0.461538461538462,-0.446153846153846,
-0.430769230769231,-0.415384615384615,-0.4,-0.384615384615385,-0.369230769230769,
-0.353846153846154,-0.338461538461538,-0.323076923076923,-0.307692307692308,
-0.292307692307692,-0.276923076923077,-0.261538461538462,-0.246153846153846,
-0.230769230769231,-0.215384615384615,-0.2,-0.184615384615385,-0.169230769230769,
-0.153846153846154,-0.138461538461538,-0.123076923076923,-0.107692307692308,
-0.0923076923076923,-0.0769230769230769,-0.0615384615384615,-0.0461538461538462,
-0.0307692307692308,-0.0153846153846154,0.),(-1.,1.),.UNSPECIFIED.)
GEOMETRIC_REPRESENTATION_ITEM()
RATIONAL_B_SPLINE_SURFACE(((1.,1.),(1.,1.),(1.,1.),(1.,1.),(1.,1.),(1.,
1.),(1.,1.),(1.,1.),(1.,1.),(1.,1.),(1.,1.),(1.,1.),(1.,1.),(1.,1.),(1.,
1.),(1.,1.),(1.,1.),(1.,1.),(1.,1.),(1.,1.),(1.,1.),(1.,1.),(1.,1.),(1.,
1.),(1.,1.),(1.,1.),(1.,1.),(1.,1.),(1.,1.),(1.,1.),(1.,1.),(1.,1.),(1.,
1.),(1.,1.),(1.,1.),(1.,1.),(1.,1.),(1.,1.),(1.,1.),(1.,1.),(1.,1.),(1.,
1.),(1.,1.),(1.,1.),(1.,1.),(1.,1.),(1.,1.),(1.,1.),(1.,1.),(1.,1.),(1.,
1.),(1.,1.),(1.,1.),(1.,1.),(1.,1.),(1.,1.),(1.,1.),(1.,1.),(1.,1.),(1.,
1.),(1.,1.),(1.,1.),(1.,1.),(1.,1.),(1.,1.),(1.,1.),(1.,1.),(1.,1.),(1.,
1.),(1.,1.)))
REPRESENTATION_ITEM('')
SURFACE()
);
#103=(
BOUNDED_SURFACE()
B_SPLINE_SURFACE(5,1,((#51460,#51461),(#51462,#51463),(#51464,#51465),(#51466,
#51467),(#51468,#51469),(#51470,#51471),(#51472,#51473),(#51474,#51475),
(#51476,#51477),(#51478,#51479),(#51480,#51481),(#51482,#51483),(#51484,
#51485),(#51486,#51487),(#51488,#51489),(#51490,#51491),(#51492,#51493),
(#51494,#51495),(#51496,#51497),(#51498,#51499),(#51500,#51501),(#51502,
#51503),(#51504,#51505),(#51506,#51507),(#51508,#51509),(#51510,#51511),
(#51512,#51513),(#51514,#51515),(#51516,#51517),(#51518,#51519),(#51520,
#51521),(#51522,#51523),(#51524,#51525),(#51526,#51527),(#51528,#51529),
(#51530,#51531),(#51532,#51533),(#51534,#51535),(#51536,#51537),(#51538,
#51539),(#51540,#51541),(#51542,#51543),(#51544,#51545),(#51546,#51547),
(#51548,#51549),(#51550,#51551),(#51552,#51553),(#51554,#51555),(#51556,
#51557),(#51558,#51559),(#51560,#51561),(#51562,#51563),(#51564,#51565),
(#51566,#51567),(#51568,#51569),(#51570,#51571),(#51572,#51573),(#51574,
#51575),(#51576,#51577),(#51578,#51579),(#51580,#51581),(#51582,#51583),
(#51584,#51585),(#51586,#51587),(#51588,#51589),(#51590,#51591),(#51592,
#51593),(#51594,#51595),(#51596,#51597),(#51598,#51599)),.UNSPECIFIED.,
 .F.,.F.,.F.)
B_SPLINE_SURFACE_WITH_KNOTS((6,1,1,1,1,1,1,1,1,1,1,1,1,1,1,1,1,1,1,1,1,
1,1,1,1,1,1,1,1,1,1,1,1,1,1,1,1,1,1,1,1,1,1,1,1,1,1,1,1,1,1,1,1,1,1,1,1,
1,1,1,1,1,1,1,1,6),(2,2),(-1.,-0.984615384615383,-0.969230769230768,-0.953846153846152,
-0.938461538461537,-0.923076923076922,-0.907692307692306,-0.892307692307691,
-0.876923076923076,-0.86153846153846,-0.846153846153845,-0.83076923076923,
-0.815384615384614,-0.799999999999999,-0.784615384615384,-0.769230769230768,
-0.753846153846153,-0.738461538461538,-0.723076923076922,-0.707692307692307,
-0.692307692307692,-0.676923076923076,-0.661538461538461,-0.646153846153846,
-0.63076923076923,-0.615384615384615,-0.6,-0.584615384615384,-0.569230769230769,
-0.553846153846154,-0.538461538461538,-0.523076923076923,-0.507692307692308,
-0.492307692307692,-0.476923076923077,-0.461538461538462,-0.446153846153846,
-0.430769230769231,-0.415384615384615,-0.4,-0.384615384615385,-0.369230769230769,
-0.353846153846154,-0.338461538461538,-0.323076923076923,-0.307692307692308,
-0.292307692307692,-0.276923076923077,-0.261538461538462,-0.246153846153846,
-0.230769230769231,-0.215384615384615,-0.2,-0.184615384615385,-0.169230769230769,
-0.153846153846154,-0.138461538461538,-0.123076923076923,-0.107692307692308,
-0.0923076923076923,-0.0769230769230769,-0.0615384615384615,-0.0461538461538462,
-0.0307692307692308,-0.0153846153846154,0.),(-1.,1.),.UNSPECIFIED.)
GEOMETRIC_REPRESENTATION_ITEM()
RATIONAL_B_SPLINE_SURFACE(((1.,1.),(1.,1.),(1.,1.),(1.,1.),(1.,1.),(1.,
1.),(1.,1.),(1.,1.),(1.,1.),(1.,1.),(1.,1.),(1.,1.),(1.,1.),(1.,1.),(1.,
1.),(1.,1.),(1.,1.),(1.,1.),(1.,1.),(1.,1.),(1.,1.),(1.,1.),(1.,1.),(1.,
1.),(1.,1.),(1.,1.),(1.,1.),(1.,1.),(1.,1.),(1.,1.),(1.,1.),(1.,1.),(1.,
1.),(1.,1.),(1.,1.),(1.,1.),(1.,1.),(1.,1.),(1.,1.),(1.,1.),(1.,1.),(1.,
1.),(1.,1.),(1.,1.),(1.,1.),(1.,1.),(1.,1.),(1.,1.),(1.,1.),(1.,1.),(1.,
1.),(1.,1.),(1.,1.),(1.,1.),(1.,1.),(1.,1.),(1.,1.),(1.,1.),(1.,1.),(1.,
1.),(1.,1.),(1.,1.),(1.,1.),(1.,1.),(1.,1.),(1.,1.),(1.,1.),(1.,1.),(1.,
1.),(1.,1.)))
REPRESENTATION_ITEM('')
SURFACE()
);
#104=(
BOUNDED_SURFACE()
B_SPLINE_SURFACE(5,1,((#51672,#51673),(#51674,#51675),(#51676,#51677),(#51678,
#51679),(#51680,#51681),(#51682,#51683),(#51684,#51685),(#51686,#51687),
(#51688,#51689),(#51690,#51691),(#51692,#51693),(#51694,#51695),(#51696,
#51697),(#51698,#51699),(#51700,#51701),(#51702,#51703),(#51704,#51705),
(#51706,#51707),(#51708,#51709),(#51710,#51711),(#51712,#51713),(#51714,
#51715),(#51716,#51717),(#51718,#51719),(#51720,#51721),(#51722,#51723),
(#51724,#51725),(#51726,#51727),(#51728,#51729),(#51730,#51731),(#51732,
#51733),(#51734,#51735),(#51736,#51737),(#51738,#51739),(#51740,#51741),
(#51742,#51743),(#51744,#51745),(#51746,#51747),(#51748,#51749),(#51750,
#51751),(#51752,#51753),(#51754,#51755),(#51756,#51757),(#51758,#51759),
(#51760,#51761),(#51762,#51763),(#51764,#51765),(#51766,#51767),(#51768,
#51769),(#51770,#51771),(#51772,#51773),(#51774,#51775),(#51776,#51777),
(#51778,#51779),(#51780,#51781),(#51782,#51783),(#51784,#51785),(#51786,
#51787),(#51788,#51789),(#51790,#51791),(#51792,#51793),(#51794,#51795),
(#51796,#51797),(#51798,#51799),(#51800,#51801),(#51802,#51803),(#51804,
#51805),(#51806,#51807),(#51808,#51809),(#51810,#51811)),.UNSPECIFIED.,
 .F.,.F.,.F.)
B_SPLINE_SURFACE_WITH_KNOTS((6,1,1,1,1,1,1,1,1,1,1,1,1,1,1,1,1,1,1,1,1,
1,1,1,1,1,1,1,1,1,1,1,1,1,1,1,1,1,1,1,1,1,1,1,1,1,1,1,1,1,1,1,1,1,1,1,1,
1,1,1,1,1,1,1,1,6),(2,2),(-1.,-0.984615384615383,-0.969230769230768,-0.953846153846152,
-0.938461538461537,-0.923076923076922,-0.907692307692306,-0.892307692307691,
-0.876923076923076,-0.86153846153846,-0.846153846153845,-0.83076923076923,
-0.815384615384614,-0.799999999999999,-0.784615384615384,-0.769230769230768,
-0.753846153846153,-0.738461538461538,-0.723076923076922,-0.707692307692307,
-0.692307692307692,-0.676923076923076,-0.661538461538461,-0.646153846153846,
-0.63076923076923,-0.615384615384615,-0.6,-0.584615384615384,-0.569230769230769,
-0.553846153846154,-0.538461538461538,-0.523076923076923,-0.507692307692308,
-0.492307692307692,-0.476923076923077,-0.461538461538462,-0.446153846153846,
-0.430769230769231,-0.415384615384615,-0.4,-0.384615384615385,-0.369230769230769,
-0.353846153846154,-0.338461538461538,-0.323076923076923,-0.307692307692308,
-0.292307692307692,-0.276923076923077,-0.261538461538462,-0.246153846153846,
-0.230769230769231,-0.215384615384615,-0.2,-0.184615384615385,-0.169230769230769,
-0.153846153846154,-0.138461538461538,-0.123076923076923,-0.107692307692308,
-0.0923076923076923,-0.0769230769230769,-0.0615384615384615,-0.0461538461538462,
-0.0307692307692308,-0.0153846153846154,0.),(-1.,1.),.UNSPECIFIED.)
GEOMETRIC_REPRESENTATION_ITEM()
RATIONAL_B_SPLINE_SURFACE(((1.,1.),(1.,1.),(1.,1.),(1.,1.),(1.,1.),(1.,
1.),(1.,1.),(1.,1.),(1.,1.),(1.,1.),(1.,1.),(1.,1.),(1.,1.),(1.,1.),(1.,
1.),(1.,1.),(1.,1.),(1.,1.),(1.,1.),(1.,1.),(1.,1.),(1.,1.),(1.,1.),(1.,
1.),(1.,1.),(1.,1.),(1.,1.),(1.,1.),(1.,1.),(1.,1.),(1.,1.),(1.,1.),(1.,
1.),(1.,1.),(1.,1.),(1.,1.),(1.,1.),(1.,1.),(1.,1.),(1.,1.),(1.,1.),(1.,
1.),(1.,1.),(1.,1.),(1.,1.),(1.,1.),(1.,1.),(1.,1.),(1.,1.),(1.,1.),(1.,
1.),(1.,1.),(1.,1.),(1.,1.),(1.,1.),(1.,1.),(1.,1.),(1.,1.),(1.,1.),(1.,
1.),(1.,1.),(1.,1.),(1.,1.),(1.,1.),(1.,1.),(1.,1.),(1.,1.),(1.,1.),(1.,
1.),(1.,1.)))
REPRESENTATION_ITEM('')
SURFACE()
);
#105=(
BOUNDED_SURFACE()
B_SPLINE_SURFACE(5,1,((#51902,#51903),(#51904,#51905),(#51906,#51907),(#51908,
#51909),(#51910,#51911),(#51912,#51913),(#51914,#51915),(#51916,#51917),
(#51918,#51919),(#51920,#51921),(#51922,#51923),(#51924,#51925),(#51926,
#51927),(#51928,#51929),(#51930,#51931),(#51932,#51933),(#51934,#51935),
(#51936,#51937),(#51938,#51939),(#51940,#51941),(#51942,#51943),(#51944,
#51945),(#51946,#51947),(#51948,#51949),(#51950,#51951),(#51952,#51953),
(#51954,#51955),(#51956,#51957),(#51958,#51959),(#51960,#51961),(#51962,
#51963),(#51964,#51965),(#51966,#51967),(#51968,#51969),(#51970,#51971),
(#51972,#51973),(#51974,#51975),(#51976,#51977),(#51978,#51979),(#51980,
#51981),(#51982,#51983),(#51984,#51985),(#51986,#51987),(#51988,#51989),
(#51990,#51991),(#51992,#51993),(#51994,#51995),(#51996,#51997),(#51998,
#51999),(#52000,#52001),(#52002,#52003),(#52004,#52005),(#52006,#52007),
(#52008,#52009),(#52010,#52011),(#52012,#52013),(#52014,#52015),(#52016,
#52017),(#52018,#52019),(#52020,#52021),(#52022,#52023),(#52024,#52025),
(#52026,#52027),(#52028,#52029),(#52030,#52031),(#52032,#52033),(#52034,
#52035),(#52036,#52037),(#52038,#52039),(#52040,#52041)),.UNSPECIFIED.,
 .F.,.F.,.F.)
B_SPLINE_SURFACE_WITH_KNOTS((6,1,1,1,1,1,1,1,1,1,1,1,1,1,1,1,1,1,1,1,1,
1,1,1,1,1,1,1,1,1,1,1,1,1,1,1,1,1,1,1,1,1,1,1,1,1,1,1,1,1,1,1,1,1,1,1,1,
1,1,1,1,1,1,1,1,6),(2,2),(-1.,-0.984615384615383,-0.969230769230768,-0.953846153846152,
-0.938461538461537,-0.923076923076922,-0.907692307692306,-0.892307692307691,
-0.876923076923076,-0.86153846153846,-0.846153846153845,-0.83076923076923,
-0.815384615384614,-0.799999999999999,-0.784615384615384,-0.769230769230768,
-0.753846153846153,-0.738461538461538,-0.723076923076922,-0.707692307692307,
-0.692307692307692,-0.676923076923076,-0.661538461538461,-0.646153846153846,
-0.63076923076923,-0.615384615384615,-0.6,-0.584615384615384,-0.569230769230769,
-0.553846153846154,-0.538461538461538,-0.523076923076923,-0.507692307692308,
-0.492307692307692,-0.476923076923077,-0.461538461538462,-0.446153846153846,
-0.430769230769231,-0.415384615384615,-0.4,-0.384615384615385,-0.369230769230769,
-0.353846153846154,-0.338461538461538,-0.323076923076923,-0.307692307692308,
-0.292307692307692,-0.276923076923077,-0.261538461538462,-0.246153846153846,
-0.230769230769231,-0.215384615384615,-0.2,-0.184615384615385,-0.169230769230769,
-0.153846153846154,-0.138461538461538,-0.123076923076923,-0.107692307692308,
-0.0923076923076923,-0.0769230769230769,-0.0615384615384615,-0.0461538461538462,
-0.0307692307692308,-0.0153846153846154,0.),(-1.,1.),.UNSPECIFIED.)
GEOMETRIC_REPRESENTATION_ITEM()
RATIONAL_B_SPLINE_SURFACE(((1.,1.),(1.,1.),(1.,1.),(1.,1.),(1.,1.),(1.,
1.),(1.,1.),(1.,1.),(1.,1.),(1.,1.),(1.,1.),(1.,1.),(1.,1.),(1.,1.),(1.,
1.),(1.,1.),(1.,1.),(1.,1.),(1.,1.),(1.,1.),(1.,1.),(1.,1.),(1.,1.),(1.,
1.),(1.,1.),(1.,1.),(1.,1.),(1.,1.),(1.,1.),(1.,1.),(1.,1.),(1.,1.),(1.,
1.),(1.,1.),(1.,1.),(1.,1.),(1.,1.),(1.,1.),(1.,1.),(1.,1.),(1.,1.),(1.,
1.),(1.,1.),(1.,1.),(1.,1.),(1.,1.),(1.,1.),(1.,1.),(1.,1.),(1.,1.),(1.,
1.),(1.,1.),(1.,1.),(1.,1.),(1.,1.),(1.,1.),(1.,1.),(1.,1.),(1.,1.),(1.,
1.),(1.,1.),(1.,1.),(1.,1.),(1.,1.),(1.,1.),(1.,1.),(1.,1.),(1.,1.),(1.,
1.),(1.,1.)))
REPRESENTATION_ITEM('')
SURFACE()
);
#106=(
BOUNDED_SURFACE()
B_SPLINE_SURFACE(5,1,((#52114,#52115),(#52116,#52117),(#52118,#52119),(#52120,
#52121),(#52122,#52123),(#52124,#52125),(#52126,#52127),(#52128,#52129),
(#52130,#52131),(#52132,#52133),(#52134,#52135),(#52136,#52137),(#52138,
#52139),(#52140,#52141),(#52142,#52143),(#52144,#52145),(#52146,#52147),
(#52148,#52149),(#52150,#52151),(#52152,#52153),(#52154,#52155),(#52156,
#52157),(#52158,#52159),(#52160,#52161),(#52162,#52163),(#52164,#52165),
(#52166,#52167),(#52168,#52169),(#52170,#52171),(#52172,#52173),(#52174,
#52175),(#52176,#52177),(#52178,#52179),(#52180,#52181),(#52182,#52183),
(#52184,#52185),(#52186,#52187),(#52188,#52189),(#52190,#52191),(#52192,
#52193),(#52194,#52195),(#52196,#52197),(#52198,#52199),(#52200,#52201),
(#52202,#52203),(#52204,#52205),(#52206,#52207),(#52208,#52209),(#52210,
#52211),(#52212,#52213),(#52214,#52215),(#52216,#52217),(#52218,#52219),
(#52220,#52221),(#52222,#52223),(#52224,#52225),(#52226,#52227),(#52228,
#52229),(#52230,#52231),(#52232,#52233),(#52234,#52235),(#52236,#52237),
(#52238,#52239),(#52240,#52241),(#52242,#52243),(#52244,#52245),(#52246,
#52247),(#52248,#52249),(#52250,#52251),(#52252,#52253)),.UNSPECIFIED.,
 .F.,.F.,.F.)
B_SPLINE_SURFACE_WITH_KNOTS((6,1,1,1,1,1,1,1,1,1,1,1,1,1,1,1,1,1,1,1,1,
1,1,1,1,1,1,1,1,1,1,1,1,1,1,1,1,1,1,1,1,1,1,1,1,1,1,1,1,1,1,1,1,1,1,1,1,
1,1,1,1,1,1,1,1,6),(2,2),(-1.,-0.984615384615383,-0.969230769230768,-0.953846153846152,
-0.938461538461537,-0.923076923076922,-0.907692307692306,-0.892307692307691,
-0.876923076923076,-0.86153846153846,-0.846153846153845,-0.83076923076923,
-0.815384615384614,-0.799999999999999,-0.784615384615384,-0.769230769230768,
-0.753846153846153,-0.738461538461538,-0.723076923076922,-0.707692307692307,
-0.692307692307692,-0.676923076923076,-0.661538461538461,-0.646153846153846,
-0.63076923076923,-0.615384615384615,-0.6,-0.584615384615384,-0.569230769230769,
-0.553846153846154,-0.538461538461538,-0.523076923076923,-0.507692307692308,
-0.492307692307692,-0.476923076923077,-0.461538461538462,-0.446153846153846,
-0.430769230769231,-0.415384615384615,-0.4,-0.384615384615385,-0.369230769230769,
-0.353846153846154,-0.338461538461538,-0.323076923076923,-0.307692307692308,
-0.292307692307692,-0.276923076923077,-0.261538461538462,-0.246153846153846,
-0.230769230769231,-0.215384615384615,-0.2,-0.184615384615385,-0.169230769230769,
-0.153846153846154,-0.138461538461538,-0.123076923076923,-0.107692307692308,
-0.0923076923076923,-0.0769230769230769,-0.0615384615384615,-0.0461538461538462,
-0.0307692307692308,-0.0153846153846154,0.),(-1.,1.),.UNSPECIFIED.)
GEOMETRIC_REPRESENTATION_ITEM()
RATIONAL_B_SPLINE_SURFACE(((1.,1.),(1.,1.),(1.,1.),(1.,1.),(1.,1.),(1.,
1.),(1.,1.),(1.,1.),(1.,1.),(1.,1.),(1.,1.),(1.,1.),(1.,1.),(1.,1.),(1.,
1.),(1.,1.),(1.,1.),(1.,1.),(1.,1.),(1.,1.),(1.,1.),(1.,1.),(1.,1.),(1.,
1.),(1.,1.),(1.,1.),(1.,1.),(1.,1.),(1.,1.),(1.,1.),(1.,1.),(1.,1.),(1.,
1.),(1.,1.),(1.,1.),(1.,1.),(1.,1.),(1.,1.),(1.,1.),(1.,1.),(1.,1.),(1.,
1.),(1.,1.),(1.,1.),(1.,1.),(1.,1.),(1.,1.),(1.,1.),(1.,1.),(1.,1.),(1.,
1.),(1.,1.),(1.,1.),(1.,1.),(1.,1.),(1.,1.),(1.,1.),(1.,1.),(1.,1.),(1.,
1.),(1.,1.),(1.,1.),(1.,1.),(1.,1.),(1.,1.),(1.,1.),(1.,1.),(1.,1.),(1.,
1.),(1.,1.)))
REPRESENTATION_ITEM('')
SURFACE()
);
#107=(
BOUNDED_SURFACE()
B_SPLINE_SURFACE(5,1,((#52344,#52345),(#52346,#52347),(#52348,#52349),(#52350,
#52351),(#52352,#52353),(#52354,#52355),(#52356,#52357),(#52358,#52359),
(#52360,#52361),(#52362,#52363),(#52364,#52365),(#52366,#52367),(#52368,
#52369),(#52370,#52371),(#52372,#52373),(#52374,#52375),(#52376,#52377),
(#52378,#52379),(#52380,#52381),(#52382,#52383),(#52384,#52385),(#52386,
#52387),(#52388,#52389),(#52390,#52391),(#52392,#52393),(#52394,#52395),
(#52396,#52397),(#52398,#52399),(#52400,#52401),(#52402,#52403),(#52404,
#52405),(#52406,#52407),(#52408,#52409),(#52410,#52411),(#52412,#52413),
(#52414,#52415),(#52416,#52417),(#52418,#52419),(#52420,#52421),(#52422,
#52423),(#52424,#52425),(#52426,#52427),(#52428,#52429),(#52430,#52431),
(#52432,#52433),(#52434,#52435),(#52436,#52437),(#52438,#52439),(#52440,
#52441),(#52442,#52443),(#52444,#52445),(#52446,#52447),(#52448,#52449),
(#52450,#52451),(#52452,#52453),(#52454,#52455),(#52456,#52457),(#52458,
#52459),(#52460,#52461),(#52462,#52463),(#52464,#52465),(#52466,#52467),
(#52468,#52469),(#52470,#52471),(#52472,#52473),(#52474,#52475),(#52476,
#52477),(#52478,#52479),(#52480,#52481),(#52482,#52483)),.UNSPECIFIED.,
 .F.,.F.,.F.)
B_SPLINE_SURFACE_WITH_KNOTS((6,1,1,1,1,1,1,1,1,1,1,1,1,1,1,1,1,1,1,1,1,
1,1,1,1,1,1,1,1,1,1,1,1,1,1,1,1,1,1,1,1,1,1,1,1,1,1,1,1,1,1,1,1,1,1,1,1,
1,1,1,1,1,1,1,1,6),(2,2),(-1.,-0.984615384615383,-0.969230769230768,-0.953846153846152,
-0.938461538461537,-0.923076923076922,-0.907692307692306,-0.892307692307691,
-0.876923076923076,-0.86153846153846,-0.846153846153845,-0.83076923076923,
-0.815384615384614,-0.799999999999999,-0.784615384615384,-0.769230769230768,
-0.753846153846153,-0.738461538461538,-0.723076923076922,-0.707692307692307,
-0.692307692307692,-0.676923076923076,-0.661538461538461,-0.646153846153846,
-0.63076923076923,-0.615384615384615,-0.6,-0.584615384615384,-0.569230769230769,
-0.553846153846154,-0.538461538461538,-0.523076923076923,-0.507692307692308,
-0.492307692307692,-0.476923076923077,-0.461538461538462,-0.446153846153846,
-0.430769230769231,-0.415384615384615,-0.4,-0.384615384615385,-0.369230769230769,
-0.353846153846154,-0.338461538461538,-0.323076923076923,-0.307692307692308,
-0.292307692307692,-0.276923076923077,-0.261538461538462,-0.246153846153846,
-0.230769230769231,-0.215384615384615,-0.2,-0.184615384615385,-0.169230769230769,
-0.153846153846154,-0.138461538461538,-0.123076923076923,-0.107692307692308,
-0.0923076923076923,-0.0769230769230769,-0.0615384615384615,-0.0461538461538462,
-0.0307692307692308,-0.0153846153846154,0.),(-1.,1.),.UNSPECIFIED.)
GEOMETRIC_REPRESENTATION_ITEM()
RATIONAL_B_SPLINE_SURFACE(((1.,1.),(1.,1.),(1.,1.),(1.,1.),(1.,1.),(1.,
1.),(1.,1.),(1.,1.),(1.,1.),(1.,1.),(1.,1.),(1.,1.),(1.,1.),(1.,1.),(1.,
1.),(1.,1.),(1.,1.),(1.,1.),(1.,1.),(1.,1.),(1.,1.),(1.,1.),(1.,1.),(1.,
1.),(1.,1.),(1.,1.),(1.,1.),(1.,1.),(1.,1.),(1.,1.),(1.,1.),(1.,1.),(1.,
1.),(1.,1.),(1.,1.),(1.,1.),(1.,1.),(1.,1.),(1.,1.),(1.,1.),(1.,1.),(1.,
1.),(1.,1.),(1.,1.),(1.,1.),(1.,1.),(1.,1.),(1.,1.),(1.,1.),(1.,1.),(1.,
1.),(1.,1.),(1.,1.),(1.,1.),(1.,1.),(1.,1.),(1.,1.),(1.,1.),(1.,1.),(1.,
1.),(1.,1.),(1.,1.),(1.,1.),(1.,1.),(1.,1.),(1.,1.),(1.,1.),(1.,1.),(1.,
1.),(1.,1.)))
REPRESENTATION_ITEM('')
SURFACE()
);
#108=(
BOUNDED_SURFACE()
B_SPLINE_SURFACE(5,1,((#52556,#52557),(#52558,#52559),(#52560,#52561),(#52562,
#52563),(#52564,#52565),(#52566,#52567),(#52568,#52569),(#52570,#52571),
(#52572,#52573),(#52574,#52575),(#52576,#52577),(#52578,#52579),(#52580,
#52581),(#52582,#52583),(#52584,#52585),(#52586,#52587),(#52588,#52589),
(#52590,#52591),(#52592,#52593),(#52594,#52595),(#52596,#52597),(#52598,
#52599),(#52600,#52601),(#52602,#52603),(#52604,#52605),(#52606,#52607),
(#52608,#52609),(#52610,#52611),(#52612,#52613),(#52614,#52615),(#52616,
#52617),(#52618,#52619),(#52620,#52621),(#52622,#52623),(#52624,#52625),
(#52626,#52627),(#52628,#52629),(#52630,#52631),(#52632,#52633),(#52634,
#52635),(#52636,#52637),(#52638,#52639),(#52640,#52641),(#52642,#52643),
(#52644,#52645),(#52646,#52647),(#52648,#52649),(#52650,#52651),(#52652,
#52653),(#52654,#52655),(#52656,#52657),(#52658,#52659),(#52660,#52661),
(#52662,#52663),(#52664,#52665),(#52666,#52667),(#52668,#52669),(#52670,
#52671),(#52672,#52673),(#52674,#52675),(#52676,#52677),(#52678,#52679),
(#52680,#52681),(#52682,#52683),(#52684,#52685),(#52686,#52687),(#52688,
#52689),(#52690,#52691),(#52692,#52693),(#52694,#52695)),.UNSPECIFIED.,
 .F.,.F.,.F.)
B_SPLINE_SURFACE_WITH_KNOTS((6,1,1,1,1,1,1,1,1,1,1,1,1,1,1,1,1,1,1,1,1,
1,1,1,1,1,1,1,1,1,1,1,1,1,1,1,1,1,1,1,1,1,1,1,1,1,1,1,1,1,1,1,1,1,1,1,1,
1,1,1,1,1,1,1,1,6),(2,2),(-1.,-0.984615384615383,-0.969230769230768,-0.953846153846152,
-0.938461538461537,-0.923076923076922,-0.907692307692306,-0.892307692307691,
-0.876923076923076,-0.86153846153846,-0.846153846153845,-0.83076923076923,
-0.815384615384614,-0.799999999999999,-0.784615384615384,-0.769230769230768,
-0.753846153846153,-0.738461538461538,-0.723076923076922,-0.707692307692307,
-0.692307692307692,-0.676923076923076,-0.661538461538461,-0.646153846153846,
-0.63076923076923,-0.615384615384615,-0.6,-0.584615384615384,-0.569230769230769,
-0.553846153846154,-0.538461538461538,-0.523076923076923,-0.507692307692308,
-0.492307692307692,-0.476923076923077,-0.461538461538462,-0.446153846153846,
-0.430769230769231,-0.415384615384615,-0.4,-0.384615384615385,-0.369230769230769,
-0.353846153846154,-0.338461538461538,-0.323076923076923,-0.307692307692308,
-0.292307692307692,-0.276923076923077,-0.261538461538462,-0.246153846153846,
-0.230769230769231,-0.215384615384615,-0.2,-0.184615384615385,-0.169230769230769,
-0.153846153846154,-0.138461538461538,-0.123076923076923,-0.107692307692308,
-0.0923076923076923,-0.0769230769230769,-0.0615384615384615,-0.0461538461538462,
-0.0307692307692308,-0.0153846153846154,0.),(-1.,1.),.UNSPECIFIED.)
GEOMETRIC_REPRESENTATION_ITEM()
RATIONAL_B_SPLINE_SURFACE(((1.,1.),(1.,1.),(1.,1.),(1.,1.),(1.,1.),(1.,
1.),(1.,1.),(1.,1.),(1.,1.),(1.,1.),(1.,1.),(1.,1.),(1.,1.),(1.,1.),(1.,
1.),(1.,1.),(1.,1.),(1.,1.),(1.,1.),(1.,1.),(1.,1.),(1.,1.),(1.,1.),(1.,
1.),(1.,1.),(1.,1.),(1.,1.),(1.,1.),(1.,1.),(1.,1.),(1.,1.),(1.,1.),(1.,
1.),(1.,1.),(1.,1.),(1.,1.),(1.,1.),(1.,1.),(1.,1.),(1.,1.),(1.,1.),(1.,
1.),(1.,1.),(1.,1.),(1.,1.),(1.,1.),(1.,1.),(1.,1.),(1.,1.),(1.,1.),(1.,
1.),(1.,1.),(1.,1.),(1.,1.),(1.,1.),(1.,1.),(1.,1.),(1.,1.),(1.,1.),(1.,
1.),(1.,1.),(1.,1.),(1.,1.),(1.,1.),(1.,1.),(1.,1.),(1.,1.),(1.,1.),(1.,
1.),(1.,1.)))
REPRESENTATION_ITEM('')
SURFACE()
);
#109=(
BOUNDED_SURFACE()
B_SPLINE_SURFACE(5,1,((#52786,#52787),(#52788,#52789),(#52790,#52791),(#52792,
#52793),(#52794,#52795),(#52796,#52797),(#52798,#52799),(#52800,#52801),
(#52802,#52803),(#52804,#52805),(#52806,#52807),(#52808,#52809),(#52810,
#52811),(#52812,#52813),(#52814,#52815),(#52816,#52817),(#52818,#52819),
(#52820,#52821),(#52822,#52823),(#52824,#52825),(#52826,#52827),(#52828,
#52829),(#52830,#52831),(#52832,#52833),(#52834,#52835),(#52836,#52837),
(#52838,#52839),(#52840,#52841),(#52842,#52843),(#52844,#52845),(#52846,
#52847),(#52848,#52849),(#52850,#52851),(#52852,#52853),(#52854,#52855),
(#52856,#52857),(#52858,#52859),(#52860,#52861),(#52862,#52863),(#52864,
#52865),(#52866,#52867),(#52868,#52869),(#52870,#52871),(#52872,#52873),
(#52874,#52875),(#52876,#52877),(#52878,#52879),(#52880,#52881),(#52882,
#52883),(#52884,#52885),(#52886,#52887),(#52888,#52889),(#52890,#52891),
(#52892,#52893),(#52894,#52895),(#52896,#52897),(#52898,#52899),(#52900,
#52901),(#52902,#52903),(#52904,#52905),(#52906,#52907),(#52908,#52909),
(#52910,#52911),(#52912,#52913),(#52914,#52915),(#52916,#52917),(#52918,
#52919),(#52920,#52921),(#52922,#52923),(#52924,#52925)),.UNSPECIFIED.,
 .F.,.F.,.F.)
B_SPLINE_SURFACE_WITH_KNOTS((6,1,1,1,1,1,1,1,1,1,1,1,1,1,1,1,1,1,1,1,1,
1,1,1,1,1,1,1,1,1,1,1,1,1,1,1,1,1,1,1,1,1,1,1,1,1,1,1,1,1,1,1,1,1,1,1,1,
1,1,1,1,1,1,1,1,6),(2,2),(-1.,-0.984615384615383,-0.969230769230768,-0.953846153846152,
-0.938461538461537,-0.923076923076922,-0.907692307692306,-0.892307692307691,
-0.876923076923076,-0.86153846153846,-0.846153846153845,-0.83076923076923,
-0.815384615384614,-0.799999999999999,-0.784615384615384,-0.769230769230768,
-0.753846153846153,-0.738461538461538,-0.723076923076922,-0.707692307692307,
-0.692307692307692,-0.676923076923076,-0.661538461538461,-0.646153846153846,
-0.63076923076923,-0.615384615384615,-0.6,-0.584615384615384,-0.569230769230769,
-0.553846153846154,-0.538461538461538,-0.523076923076923,-0.507692307692308,
-0.492307692307692,-0.476923076923077,-0.461538461538462,-0.446153846153846,
-0.430769230769231,-0.415384615384615,-0.4,-0.384615384615385,-0.369230769230769,
-0.353846153846154,-0.338461538461538,-0.323076923076923,-0.307692307692308,
-0.292307692307692,-0.276923076923077,-0.261538461538462,-0.246153846153846,
-0.230769230769231,-0.215384615384615,-0.2,-0.184615384615385,-0.169230769230769,
-0.153846153846154,-0.138461538461538,-0.123076923076923,-0.107692307692308,
-0.0923076923076923,-0.0769230769230769,-0.0615384615384615,-0.0461538461538462,
-0.0307692307692308,-0.0153846153846154,0.),(-1.,1.),.UNSPECIFIED.)
GEOMETRIC_REPRESENTATION_ITEM()
RATIONAL_B_SPLINE_SURFACE(((1.,1.),(1.,1.),(1.,1.),(1.,1.),(1.,1.),(1.,
1.),(1.,1.),(1.,1.),(1.,1.),(1.,1.),(1.,1.),(1.,1.),(1.,1.),(1.,1.),(1.,
1.),(1.,1.),(1.,1.),(1.,1.),(1.,1.),(1.,1.),(1.,1.),(1.,1.),(1.,1.),(1.,
1.),(1.,1.),(1.,1.),(1.,1.),(1.,1.),(1.,1.),(1.,1.),(1.,1.),(1.,1.),(1.,
1.),(1.,1.),(1.,1.),(1.,1.),(1.,1.),(1.,1.),(1.,1.),(1.,1.),(1.,1.),(1.,
1.),(1.,1.),(1.,1.),(1.,1.),(1.,1.),(1.,1.),(1.,1.),(1.,1.),(1.,1.),(1.,
1.),(1.,1.),(1.,1.),(1.,1.),(1.,1.),(1.,1.),(1.,1.),(1.,1.),(1.,1.),(1.,
1.),(1.,1.),(1.,1.),(1.,1.),(1.,1.),(1.,1.),(1.,1.),(1.,1.),(1.,1.),(1.,
1.),(1.,1.)))
REPRESENTATION_ITEM('')
SURFACE()
);
#110=(
BOUNDED_SURFACE()
B_SPLINE_SURFACE(5,1,((#52998,#52999),(#53000,#53001),(#53002,#53003),(#53004,
#53005),(#53006,#53007),(#53008,#53009),(#53010,#53011),(#53012,#53013),
(#53014,#53015),(#53016,#53017),(#53018,#53019),(#53020,#53021),(#53022,
#53023),(#53024,#53025),(#53026,#53027),(#53028,#53029),(#53030,#53031),
(#53032,#53033),(#53034,#53035),(#53036,#53037),(#53038,#53039),(#53040,
#53041),(#53042,#53043),(#53044,#53045),(#53046,#53047),(#53048,#53049),
(#53050,#53051),(#53052,#53053),(#53054,#53055),(#53056,#53057),(#53058,
#53059),(#53060,#53061),(#53062,#53063),(#53064,#53065),(#53066,#53067),
(#53068,#53069),(#53070,#53071),(#53072,#53073),(#53074,#53075),(#53076,
#53077),(#53078,#53079),(#53080,#53081),(#53082,#53083),(#53084,#53085),
(#53086,#53087),(#53088,#53089),(#53090,#53091),(#53092,#53093),(#53094,
#53095),(#53096,#53097),(#53098,#53099),(#53100,#53101),(#53102,#53103),
(#53104,#53105),(#53106,#53107),(#53108,#53109),(#53110,#53111),(#53112,
#53113),(#53114,#53115),(#53116,#53117),(#53118,#53119),(#53120,#53121),
(#53122,#53123),(#53124,#53125),(#53126,#53127),(#53128,#53129),(#53130,
#53131),(#53132,#53133),(#53134,#53135),(#53136,#53137)),.UNSPECIFIED.,
 .F.,.F.,.F.)
B_SPLINE_SURFACE_WITH_KNOTS((6,1,1,1,1,1,1,1,1,1,1,1,1,1,1,1,1,1,1,1,1,
1,1,1,1,1,1,1,1,1,1,1,1,1,1,1,1,1,1,1,1,1,1,1,1,1,1,1,1,1,1,1,1,1,1,1,1,
1,1,1,1,1,1,1,1,6),(2,2),(-1.,-0.984615384615383,-0.969230769230768,-0.953846153846152,
-0.938461538461537,-0.923076923076922,-0.907692307692306,-0.892307692307691,
-0.876923076923076,-0.86153846153846,-0.846153846153845,-0.83076923076923,
-0.815384615384614,-0.799999999999999,-0.784615384615384,-0.769230769230768,
-0.753846153846153,-0.738461538461538,-0.723076923076922,-0.707692307692307,
-0.692307692307692,-0.676923076923076,-0.661538461538461,-0.646153846153846,
-0.63076923076923,-0.615384615384615,-0.6,-0.584615384615384,-0.569230769230769,
-0.553846153846154,-0.538461538461538,-0.523076923076923,-0.507692307692308,
-0.492307692307692,-0.476923076923077,-0.461538461538462,-0.446153846153846,
-0.430769230769231,-0.415384615384615,-0.4,-0.384615384615385,-0.369230769230769,
-0.353846153846154,-0.338461538461538,-0.323076923076923,-0.307692307692308,
-0.292307692307692,-0.276923076923077,-0.261538461538462,-0.246153846153846,
-0.230769230769231,-0.215384615384615,-0.2,-0.184615384615385,-0.169230769230769,
-0.153846153846154,-0.138461538461538,-0.123076923076923,-0.107692307692308,
-0.0923076923076923,-0.0769230769230769,-0.0615384615384615,-0.0461538461538462,
-0.0307692307692308,-0.0153846153846154,0.),(-1.,1.),.UNSPECIFIED.)
GEOMETRIC_REPRESENTATION_ITEM()
RATIONAL_B_SPLINE_SURFACE(((1.,1.),(1.,1.),(1.,1.),(1.,1.),(1.,1.),(1.,
1.),(1.,1.),(1.,1.),(1.,1.),(1.,1.),(1.,1.),(1.,1.),(1.,1.),(1.,1.),(1.,
1.),(1.,1.),(1.,1.),(1.,1.),(1.,1.),(1.,1.),(1.,1.),(1.,1.),(1.,1.),(1.,
1.),(1.,1.),(1.,1.),(1.,1.),(1.,1.),(1.,1.),(1.,1.),(1.,1.),(1.,1.),(1.,
1.),(1.,1.),(1.,1.),(1.,1.),(1.,1.),(1.,1.),(1.,1.),(1.,1.),(1.,1.),(1.,
1.),(1.,1.),(1.,1.),(1.,1.),(1.,1.),(1.,1.),(1.,1.),(1.,1.),(1.,1.),(1.,
1.),(1.,1.),(1.,1.),(1.,1.),(1.,1.),(1.,1.),(1.,1.),(1.,1.),(1.,1.),(1.,
1.),(1.,1.),(1.,1.),(1.,1.),(1.,1.),(1.,1.),(1.,1.),(1.,1.),(1.,1.),(1.,
1.),(1.,1.)))
REPRESENTATION_ITEM('')
SURFACE()
);
#111=(
BOUNDED_SURFACE()
B_SPLINE_SURFACE(5,1,((#53228,#53229),(#53230,#53231),(#53232,#53233),(#53234,
#53235),(#53236,#53237),(#53238,#53239),(#53240,#53241),(#53242,#53243),
(#53244,#53245),(#53246,#53247),(#53248,#53249),(#53250,#53251),(#53252,
#53253),(#53254,#53255),(#53256,#53257),(#53258,#53259),(#53260,#53261),
(#53262,#53263),(#53264,#53265),(#53266,#53267),(#53268,#53269),(#53270,
#53271),(#53272,#53273),(#53274,#53275),(#53276,#53277),(#53278,#53279),
(#53280,#53281),(#53282,#53283),(#53284,#53285),(#53286,#53287),(#53288,
#53289),(#53290,#53291),(#53292,#53293),(#53294,#53295),(#53296,#53297),
(#53298,#53299),(#53300,#53301),(#53302,#53303),(#53304,#53305),(#53306,
#53307),(#53308,#53309),(#53310,#53311),(#53312,#53313),(#53314,#53315),
(#53316,#53317),(#53318,#53319),(#53320,#53321),(#53322,#53323),(#53324,
#53325),(#53326,#53327),(#53328,#53329),(#53330,#53331),(#53332,#53333),
(#53334,#53335),(#53336,#53337),(#53338,#53339),(#53340,#53341),(#53342,
#53343),(#53344,#53345),(#53346,#53347),(#53348,#53349),(#53350,#53351),
(#53352,#53353),(#53354,#53355),(#53356,#53357),(#53358,#53359),(#53360,
#53361),(#53362,#53363),(#53364,#53365),(#53366,#53367)),.UNSPECIFIED.,
 .F.,.F.,.F.)
B_SPLINE_SURFACE_WITH_KNOTS((6,1,1,1,1,1,1,1,1,1,1,1,1,1,1,1,1,1,1,1,1,
1,1,1,1,1,1,1,1,1,1,1,1,1,1,1,1,1,1,1,1,1,1,1,1,1,1,1,1,1,1,1,1,1,1,1,1,
1,1,1,1,1,1,1,1,6),(2,2),(-1.,-0.984615384615383,-0.969230769230768,-0.953846153846152,
-0.938461538461537,-0.923076923076922,-0.907692307692306,-0.892307692307691,
-0.876923076923076,-0.86153846153846,-0.846153846153845,-0.83076923076923,
-0.815384615384614,-0.799999999999999,-0.784615384615384,-0.769230769230768,
-0.753846153846153,-0.738461538461538,-0.723076923076922,-0.707692307692307,
-0.692307692307692,-0.676923076923076,-0.661538461538461,-0.646153846153846,
-0.63076923076923,-0.615384615384615,-0.6,-0.584615384615384,-0.569230769230769,
-0.553846153846154,-0.538461538461538,-0.523076923076923,-0.507692307692308,
-0.492307692307692,-0.476923076923077,-0.461538461538462,-0.446153846153846,
-0.430769230769231,-0.415384615384615,-0.4,-0.384615384615385,-0.369230769230769,
-0.353846153846154,-0.338461538461538,-0.323076923076923,-0.307692307692308,
-0.292307692307692,-0.276923076923077,-0.261538461538462,-0.246153846153846,
-0.230769230769231,-0.215384615384615,-0.2,-0.184615384615385,-0.169230769230769,
-0.153846153846154,-0.138461538461538,-0.123076923076923,-0.107692307692308,
-0.0923076923076923,-0.0769230769230769,-0.0615384615384615,-0.0461538461538462,
-0.0307692307692308,-0.0153846153846154,0.),(-1.,1.),.UNSPECIFIED.)
GEOMETRIC_REPRESENTATION_ITEM()
RATIONAL_B_SPLINE_SURFACE(((1.,1.),(1.,1.),(1.,1.),(1.,1.),(1.,1.),(1.,
1.),(1.,1.),(1.,1.),(1.,1.),(1.,1.),(1.,1.),(1.,1.),(1.,1.),(1.,1.),(1.,
1.),(1.,1.),(1.,1.),(1.,1.),(1.,1.),(1.,1.),(1.,1.),(1.,1.),(1.,1.),(1.,
1.),(1.,1.),(1.,1.),(1.,1.),(1.,1.),(1.,1.),(1.,1.),(1.,1.),(1.,1.),(1.,
1.),(1.,1.),(1.,1.),(1.,1.),(1.,1.),(1.,1.),(1.,1.),(1.,1.),(1.,1.),(1.,
1.),(1.,1.),(1.,1.),(1.,1.),(1.,1.),(1.,1.),(1.,1.),(1.,1.),(1.,1.),(1.,
1.),(1.,1.),(1.,1.),(1.,1.),(1.,1.),(1.,1.),(1.,1.),(1.,1.),(1.,1.),(1.,
1.),(1.,1.),(1.,1.),(1.,1.),(1.,1.),(1.,1.),(1.,1.),(1.,1.),(1.,1.),(1.,
1.),(1.,1.)))
REPRESENTATION_ITEM('')
SURFACE()
);
#112=(
BOUNDED_SURFACE()
B_SPLINE_SURFACE(5,1,((#53440,#53441),(#53442,#53443),(#53444,#53445),(#53446,
#53447),(#53448,#53449),(#53450,#53451),(#53452,#53453),(#53454,#53455),
(#53456,#53457),(#53458,#53459),(#53460,#53461),(#53462,#53463),(#53464,
#53465),(#53466,#53467),(#53468,#53469),(#53470,#53471),(#53472,#53473),
(#53474,#53475),(#53476,#53477),(#53478,#53479),(#53480,#53481),(#53482,
#53483),(#53484,#53485),(#53486,#53487),(#53488,#53489),(#53490,#53491),
(#53492,#53493),(#53494,#53495),(#53496,#53497),(#53498,#53499),(#53500,
#53501),(#53502,#53503),(#53504,#53505),(#53506,#53507),(#53508,#53509),
(#53510,#53511),(#53512,#53513),(#53514,#53515),(#53516,#53517),(#53518,
#53519),(#53520,#53521),(#53522,#53523),(#53524,#53525),(#53526,#53527),
(#53528,#53529),(#53530,#53531),(#53532,#53533),(#53534,#53535),(#53536,
#53537),(#53538,#53539),(#53540,#53541),(#53542,#53543),(#53544,#53545),
(#53546,#53547),(#53548,#53549),(#53550,#53551),(#53552,#53553),(#53554,
#53555),(#53556,#53557),(#53558,#53559),(#53560,#53561),(#53562,#53563),
(#53564,#53565),(#53566,#53567),(#53568,#53569),(#53570,#53571),(#53572,
#53573),(#53574,#53575),(#53576,#53577),(#53578,#53579)),.UNSPECIFIED.,
 .F.,.F.,.F.)
B_SPLINE_SURFACE_WITH_KNOTS((6,1,1,1,1,1,1,1,1,1,1,1,1,1,1,1,1,1,1,1,1,
1,1,1,1,1,1,1,1,1,1,1,1,1,1,1,1,1,1,1,1,1,1,1,1,1,1,1,1,1,1,1,1,1,1,1,1,
1,1,1,1,1,1,1,1,6),(2,2),(-1.,-0.984615384615383,-0.969230769230768,-0.953846153846152,
-0.938461538461537,-0.923076923076922,-0.907692307692306,-0.892307692307691,
-0.876923076923076,-0.86153846153846,-0.846153846153845,-0.83076923076923,
-0.815384615384614,-0.799999999999999,-0.784615384615384,-0.769230769230768,
-0.753846153846153,-0.738461538461538,-0.723076923076922,-0.707692307692307,
-0.692307692307692,-0.676923076923076,-0.661538461538461,-0.646153846153846,
-0.63076923076923,-0.615384615384615,-0.6,-0.584615384615384,-0.569230769230769,
-0.553846153846154,-0.538461538461538,-0.523076923076923,-0.507692307692308,
-0.492307692307692,-0.476923076923077,-0.461538461538462,-0.446153846153846,
-0.430769230769231,-0.415384615384615,-0.4,-0.384615384615385,-0.369230769230769,
-0.353846153846154,-0.338461538461538,-0.323076923076923,-0.307692307692308,
-0.292307692307692,-0.276923076923077,-0.261538461538462,-0.246153846153846,
-0.230769230769231,-0.215384615384615,-0.2,-0.184615384615385,-0.169230769230769,
-0.153846153846154,-0.138461538461538,-0.123076923076923,-0.107692307692308,
-0.0923076923076923,-0.0769230769230769,-0.0615384615384615,-0.0461538461538462,
-0.0307692307692308,-0.0153846153846154,0.),(-1.,1.),.UNSPECIFIED.)
GEOMETRIC_REPRESENTATION_ITEM()
RATIONAL_B_SPLINE_SURFACE(((1.,1.),(1.,1.),(1.,1.),(1.,1.),(1.,1.),(1.,
1.),(1.,1.),(1.,1.),(1.,1.),(1.,1.),(1.,1.),(1.,1.),(1.,1.),(1.,1.),(1.,
1.),(1.,1.),(1.,1.),(1.,1.),(1.,1.),(1.,1.),(1.,1.),(1.,1.),(1.,1.),(1.,
1.),(1.,1.),(1.,1.),(1.,1.),(1.,1.),(1.,1.),(1.,1.),(1.,1.),(1.,1.),(1.,
1.),(1.,1.),(1.,1.),(1.,1.),(1.,1.),(1.,1.),(1.,1.),(1.,1.),(1.,1.),(1.,
1.),(1.,1.),(1.,1.),(1.,1.),(1.,1.),(1.,1.),(1.,1.),(1.,1.),(1.,1.),(1.,
1.),(1.,1.),(1.,1.),(1.,1.),(1.,1.),(1.,1.),(1.,1.),(1.,1.),(1.,1.),(1.,
1.),(1.,1.),(1.,1.),(1.,1.),(1.,1.),(1.,1.),(1.,1.),(1.,1.),(1.,1.),(1.,
1.),(1.,1.)))
REPRESENTATION_ITEM('')
SURFACE()
);
#113=(
BOUNDED_SURFACE()
B_SPLINE_SURFACE(5,1,((#53670,#53671),(#53672,#53673),(#53674,#53675),(#53676,
#53677),(#53678,#53679),(#53680,#53681),(#53682,#53683),(#53684,#53685),
(#53686,#53687),(#53688,#53689),(#53690,#53691),(#53692,#53693),(#53694,
#53695),(#53696,#53697),(#53698,#53699),(#53700,#53701),(#53702,#53703),
(#53704,#53705),(#53706,#53707),(#53708,#53709),(#53710,#53711),(#53712,
#53713),(#53714,#53715),(#53716,#53717),(#53718,#53719),(#53720,#53721),
(#53722,#53723),(#53724,#53725),(#53726,#53727),(#53728,#53729),(#53730,
#53731),(#53732,#53733),(#53734,#53735),(#53736,#53737),(#53738,#53739),
(#53740,#53741),(#53742,#53743),(#53744,#53745),(#53746,#53747),(#53748,
#53749),(#53750,#53751),(#53752,#53753),(#53754,#53755),(#53756,#53757),
(#53758,#53759),(#53760,#53761),(#53762,#53763),(#53764,#53765),(#53766,
#53767),(#53768,#53769),(#53770,#53771),(#53772,#53773),(#53774,#53775),
(#53776,#53777),(#53778,#53779),(#53780,#53781),(#53782,#53783),(#53784,
#53785),(#53786,#53787),(#53788,#53789),(#53790,#53791),(#53792,#53793),
(#53794,#53795),(#53796,#53797),(#53798,#53799),(#53800,#53801),(#53802,
#53803),(#53804,#53805),(#53806,#53807),(#53808,#53809)),.UNSPECIFIED.,
 .F.,.F.,.F.)
B_SPLINE_SURFACE_WITH_KNOTS((6,1,1,1,1,1,1,1,1,1,1,1,1,1,1,1,1,1,1,1,1,
1,1,1,1,1,1,1,1,1,1,1,1,1,1,1,1,1,1,1,1,1,1,1,1,1,1,1,1,1,1,1,1,1,1,1,1,
1,1,1,1,1,1,1,1,6),(2,2),(-1.,-0.984615384615383,-0.969230769230768,-0.953846153846152,
-0.938461538461537,-0.923076923076922,-0.907692307692306,-0.892307692307691,
-0.876923076923076,-0.86153846153846,-0.846153846153845,-0.83076923076923,
-0.815384615384614,-0.799999999999999,-0.784615384615384,-0.769230769230768,
-0.753846153846153,-0.738461538461538,-0.723076923076922,-0.707692307692307,
-0.692307692307692,-0.676923076923076,-0.661538461538461,-0.646153846153846,
-0.63076923076923,-0.615384615384615,-0.6,-0.584615384615384,-0.569230769230769,
-0.553846153846154,-0.538461538461538,-0.523076923076923,-0.507692307692308,
-0.492307692307692,-0.476923076923077,-0.461538461538462,-0.446153846153846,
-0.430769230769231,-0.415384615384615,-0.4,-0.384615384615385,-0.369230769230769,
-0.353846153846154,-0.338461538461538,-0.323076923076923,-0.307692307692308,
-0.292307692307692,-0.276923076923077,-0.261538461538462,-0.246153846153846,
-0.230769230769231,-0.215384615384615,-0.2,-0.184615384615385,-0.169230769230769,
-0.153846153846154,-0.138461538461538,-0.123076923076923,-0.107692307692308,
-0.0923076923076923,-0.0769230769230769,-0.0615384615384615,-0.0461538461538462,
-0.0307692307692308,-0.0153846153846154,0.),(-1.,1.),.UNSPECIFIED.)
GEOMETRIC_REPRESENTATION_ITEM()
RATIONAL_B_SPLINE_SURFACE(((1.,1.),(1.,1.),(1.,1.),(1.,1.),(1.,1.),(1.,
1.),(1.,1.),(1.,1.),(1.,1.),(1.,1.),(1.,1.),(1.,1.),(1.,1.),(1.,1.),(1.,
1.),(1.,1.),(1.,1.),(1.,1.),(1.,1.),(1.,1.),(1.,1.),(1.,1.),(1.,1.),(1.,
1.),(1.,1.),(1.,1.),(1.,1.),(1.,1.),(1.,1.),(1.,1.),(1.,1.),(1.,1.),(1.,
1.),(1.,1.),(1.,1.),(1.,1.),(1.,1.),(1.,1.),(1.,1.),(1.,1.),(1.,1.),(1.,
1.),(1.,1.),(1.,1.),(1.,1.),(1.,1.),(1.,1.),(1.,1.),(1.,1.),(1.,1.),(1.,
1.),(1.,1.),(1.,1.),(1.,1.),(1.,1.),(1.,1.),(1.,1.),(1.,1.),(1.,1.),(1.,
1.),(1.,1.),(1.,1.),(1.,1.),(1.,1.),(1.,1.),(1.,1.),(1.,1.),(1.,1.),(1.,
1.),(1.,1.)))
REPRESENTATION_ITEM('')
SURFACE()
);
#114=(
BOUNDED_SURFACE()
B_SPLINE_SURFACE(5,1,((#53882,#53883),(#53884,#53885),(#53886,#53887),(#53888,
#53889),(#53890,#53891),(#53892,#53893),(#53894,#53895),(#53896,#53897),
(#53898,#53899),(#53900,#53901),(#53902,#53903),(#53904,#53905),(#53906,
#53907),(#53908,#53909),(#53910,#53911),(#53912,#53913),(#53914,#53915),
(#53916,#53917),(#53918,#53919),(#53920,#53921),(#53922,#53923),(#53924,
#53925),(#53926,#53927),(#53928,#53929),(#53930,#53931),(#53932,#53933),
(#53934,#53935),(#53936,#53937),(#53938,#53939),(#53940,#53941),(#53942,
#53943),(#53944,#53945),(#53946,#53947),(#53948,#53949),(#53950,#53951),
(#53952,#53953),(#53954,#53955),(#53956,#53957),(#53958,#53959),(#53960,
#53961),(#53962,#53963),(#53964,#53965),(#53966,#53967),(#53968,#53969),
(#53970,#53971),(#53972,#53973),(#53974,#53975),(#53976,#53977),(#53978,
#53979),(#53980,#53981),(#53982,#53983),(#53984,#53985),(#53986,#53987),
(#53988,#53989),(#53990,#53991),(#53992,#53993),(#53994,#53995),(#53996,
#53997),(#53998,#53999),(#54000,#54001),(#54002,#54003),(#54004,#54005),
(#54006,#54007),(#54008,#54009),(#54010,#54011),(#54012,#54013),(#54014,
#54015),(#54016,#54017),(#54018,#54019),(#54020,#54021)),.UNSPECIFIED.,
 .F.,.F.,.F.)
B_SPLINE_SURFACE_WITH_KNOTS((6,1,1,1,1,1,1,1,1,1,1,1,1,1,1,1,1,1,1,1,1,
1,1,1,1,1,1,1,1,1,1,1,1,1,1,1,1,1,1,1,1,1,1,1,1,1,1,1,1,1,1,1,1,1,1,1,1,
1,1,1,1,1,1,1,1,6),(2,2),(-1.,-0.984615384615383,-0.969230769230768,-0.953846153846152,
-0.938461538461537,-0.923076923076922,-0.907692307692306,-0.892307692307691,
-0.876923076923076,-0.86153846153846,-0.846153846153845,-0.83076923076923,
-0.815384615384614,-0.799999999999999,-0.784615384615384,-0.769230769230768,
-0.753846153846153,-0.738461538461538,-0.723076923076922,-0.707692307692307,
-0.692307692307692,-0.676923076923076,-0.661538461538461,-0.646153846153846,
-0.63076923076923,-0.615384615384615,-0.6,-0.584615384615384,-0.569230769230769,
-0.553846153846154,-0.538461538461538,-0.523076923076923,-0.507692307692308,
-0.492307692307692,-0.476923076923077,-0.461538461538462,-0.446153846153846,
-0.430769230769231,-0.415384615384615,-0.4,-0.384615384615385,-0.369230769230769,
-0.353846153846154,-0.338461538461538,-0.323076923076923,-0.307692307692308,
-0.292307692307692,-0.276923076923077,-0.261538461538462,-0.246153846153846,
-0.230769230769231,-0.215384615384615,-0.2,-0.184615384615385,-0.169230769230769,
-0.153846153846154,-0.138461538461538,-0.123076923076923,-0.107692307692308,
-0.0923076923076923,-0.0769230769230769,-0.0615384615384615,-0.0461538461538462,
-0.0307692307692308,-0.0153846153846154,0.),(-1.,1.),.UNSPECIFIED.)
GEOMETRIC_REPRESENTATION_ITEM()
RATIONAL_B_SPLINE_SURFACE(((1.,1.),(1.,1.),(1.,1.),(1.,1.),(1.,1.),(1.,
1.),(1.,1.),(1.,1.),(1.,1.),(1.,1.),(1.,1.),(1.,1.),(1.,1.),(1.,1.),(1.,
1.),(1.,1.),(1.,1.),(1.,1.),(1.,1.),(1.,1.),(1.,1.),(1.,1.),(1.,1.),(1.,
1.),(1.,1.),(1.,1.),(1.,1.),(1.,1.),(1.,1.),(1.,1.),(1.,1.),(1.,1.),(1.,
1.),(1.,1.),(1.,1.),(1.,1.),(1.,1.),(1.,1.),(1.,1.),(1.,1.),(1.,1.),(1.,
1.),(1.,1.),(1.,1.),(1.,1.),(1.,1.),(1.,1.),(1.,1.),(1.,1.),(1.,1.),(1.,
1.),(1.,1.),(1.,1.),(1.,1.),(1.,1.),(1.,1.),(1.,1.),(1.,1.),(1.,1.),(1.,
1.),(1.,1.),(1.,1.),(1.,1.),(1.,1.),(1.,1.),(1.,1.),(1.,1.),(1.,1.),(1.,
1.),(1.,1.)))
REPRESENTATION_ITEM('')
SURFACE()
);
#115=(
BOUNDED_SURFACE()
B_SPLINE_SURFACE(5,1,((#54112,#54113),(#54114,#54115),(#54116,#54117),(#54118,
#54119),(#54120,#54121),(#54122,#54123),(#54124,#54125),(#54126,#54127),
(#54128,#54129),(#54130,#54131),(#54132,#54133),(#54134,#54135),(#54136,
#54137),(#54138,#54139),(#54140,#54141),(#54142,#54143),(#54144,#54145),
(#54146,#54147),(#54148,#54149),(#54150,#54151),(#54152,#54153),(#54154,
#54155),(#54156,#54157),(#54158,#54159),(#54160,#54161),(#54162,#54163),
(#54164,#54165),(#54166,#54167),(#54168,#54169),(#54170,#54171),(#54172,
#54173),(#54174,#54175),(#54176,#54177),(#54178,#54179),(#54180,#54181),
(#54182,#54183),(#54184,#54185),(#54186,#54187),(#54188,#54189),(#54190,
#54191),(#54192,#54193),(#54194,#54195),(#54196,#54197),(#54198,#54199),
(#54200,#54201),(#54202,#54203),(#54204,#54205),(#54206,#54207),(#54208,
#54209),(#54210,#54211),(#54212,#54213),(#54214,#54215),(#54216,#54217),
(#54218,#54219),(#54220,#54221),(#54222,#54223),(#54224,#54225),(#54226,
#54227),(#54228,#54229),(#54230,#54231),(#54232,#54233),(#54234,#54235),
(#54236,#54237),(#54238,#54239),(#54240,#54241),(#54242,#54243),(#54244,
#54245),(#54246,#54247),(#54248,#54249),(#54250,#54251)),.UNSPECIFIED.,
 .F.,.F.,.F.)
B_SPLINE_SURFACE_WITH_KNOTS((6,1,1,1,1,1,1,1,1,1,1,1,1,1,1,1,1,1,1,1,1,
1,1,1,1,1,1,1,1,1,1,1,1,1,1,1,1,1,1,1,1,1,1,1,1,1,1,1,1,1,1,1,1,1,1,1,1,
1,1,1,1,1,1,1,1,6),(2,2),(-1.,-0.984615384615383,-0.969230769230768,-0.953846153846152,
-0.938461538461537,-0.923076923076922,-0.907692307692306,-0.892307692307691,
-0.876923076923076,-0.86153846153846,-0.846153846153845,-0.83076923076923,
-0.815384615384614,-0.799999999999999,-0.784615384615384,-0.769230769230768,
-0.753846153846153,-0.738461538461538,-0.723076923076922,-0.707692307692307,
-0.692307692307692,-0.676923076923076,-0.661538461538461,-0.646153846153846,
-0.63076923076923,-0.615384615384615,-0.6,-0.584615384615384,-0.569230769230769,
-0.553846153846154,-0.538461538461538,-0.523076923076923,-0.507692307692308,
-0.492307692307692,-0.476923076923077,-0.461538461538462,-0.446153846153846,
-0.430769230769231,-0.415384615384615,-0.4,-0.384615384615385,-0.369230769230769,
-0.353846153846154,-0.338461538461538,-0.323076923076923,-0.307692307692308,
-0.292307692307692,-0.276923076923077,-0.261538461538462,-0.246153846153846,
-0.230769230769231,-0.215384615384615,-0.2,-0.184615384615385,-0.169230769230769,
-0.153846153846154,-0.138461538461538,-0.123076923076923,-0.107692307692308,
-0.0923076923076923,-0.0769230769230769,-0.0615384615384615,-0.0461538461538462,
-0.0307692307692308,-0.0153846153846154,0.),(-1.,1.),.UNSPECIFIED.)
GEOMETRIC_REPRESENTATION_ITEM()
RATIONAL_B_SPLINE_SURFACE(((1.,1.),(1.,1.),(1.,1.),(1.,1.),(1.,1.),(1.,
1.),(1.,1.),(1.,1.),(1.,1.),(1.,1.),(1.,1.),(1.,1.),(1.,1.),(1.,1.),(1.,
1.),(1.,1.),(1.,1.),(1.,1.),(1.,1.),(1.,1.),(1.,1.),(1.,1.),(1.,1.),(1.,
1.),(1.,1.),(1.,1.),(1.,1.),(1.,1.),(1.,1.),(1.,1.),(1.,1.),(1.,1.),(1.,
1.),(1.,1.),(1.,1.),(1.,1.),(1.,1.),(1.,1.),(1.,1.),(1.,1.),(1.,1.),(1.,
1.),(1.,1.),(1.,1.),(1.,1.),(1.,1.),(1.,1.),(1.,1.),(1.,1.),(1.,1.),(1.,
1.),(1.,1.),(1.,1.),(1.,1.),(1.,1.),(1.,1.),(1.,1.),(1.,1.),(1.,1.),(1.,
1.),(1.,1.),(1.,1.),(1.,1.),(1.,1.),(1.,1.),(1.,1.),(1.,1.),(1.,1.),(1.,
1.),(1.,1.)))
REPRESENTATION_ITEM('')
SURFACE()
);
#116=(
BOUNDED_SURFACE()
B_SPLINE_SURFACE(5,1,((#54324,#54325),(#54326,#54327),(#54328,#54329),(#54330,
#54331),(#54332,#54333),(#54334,#54335),(#54336,#54337),(#54338,#54339),
(#54340,#54341),(#54342,#54343),(#54344,#54345),(#54346,#54347),(#54348,
#54349),(#54350,#54351),(#54352,#54353),(#54354,#54355),(#54356,#54357),
(#54358,#54359),(#54360,#54361),(#54362,#54363),(#54364,#54365),(#54366,
#54367),(#54368,#54369),(#54370,#54371),(#54372,#54373),(#54374,#54375),
(#54376,#54377),(#54378,#54379),(#54380,#54381),(#54382,#54383),(#54384,
#54385),(#54386,#54387),(#54388,#54389),(#54390,#54391),(#54392,#54393),
(#54394,#54395),(#54396,#54397),(#54398,#54399),(#54400,#54401),(#54402,
#54403),(#54404,#54405),(#54406,#54407),(#54408,#54409),(#54410,#54411),
(#54412,#54413),(#54414,#54415),(#54416,#54417),(#54418,#54419),(#54420,
#54421),(#54422,#54423),(#54424,#54425),(#54426,#54427),(#54428,#54429),
(#54430,#54431),(#54432,#54433),(#54434,#54435),(#54436,#54437),(#54438,
#54439),(#54440,#54441),(#54442,#54443),(#54444,#54445),(#54446,#54447),
(#54448,#54449),(#54450,#54451),(#54452,#54453),(#54454,#54455),(#54456,
#54457),(#54458,#54459),(#54460,#54461),(#54462,#54463)),.UNSPECIFIED.,
 .F.,.F.,.F.)
B_SPLINE_SURFACE_WITH_KNOTS((6,1,1,1,1,1,1,1,1,1,1,1,1,1,1,1,1,1,1,1,1,
1,1,1,1,1,1,1,1,1,1,1,1,1,1,1,1,1,1,1,1,1,1,1,1,1,1,1,1,1,1,1,1,1,1,1,1,
1,1,1,1,1,1,1,1,6),(2,2),(-1.,-0.984615384615383,-0.969230769230768,-0.953846153846152,
-0.938461538461537,-0.923076923076922,-0.907692307692306,-0.892307692307691,
-0.876923076923076,-0.86153846153846,-0.846153846153845,-0.83076923076923,
-0.815384615384614,-0.799999999999999,-0.784615384615384,-0.769230769230768,
-0.753846153846153,-0.738461538461538,-0.723076923076922,-0.707692307692307,
-0.692307692307692,-0.676923076923076,-0.661538461538461,-0.646153846153846,
-0.63076923076923,-0.615384615384615,-0.6,-0.584615384615384,-0.569230769230769,
-0.553846153846154,-0.538461538461538,-0.523076923076923,-0.507692307692308,
-0.492307692307692,-0.476923076923077,-0.461538461538462,-0.446153846153846,
-0.430769230769231,-0.415384615384615,-0.4,-0.384615384615385,-0.369230769230769,
-0.353846153846154,-0.338461538461538,-0.323076923076923,-0.307692307692308,
-0.292307692307692,-0.276923076923077,-0.261538461538462,-0.246153846153846,
-0.230769230769231,-0.215384615384615,-0.2,-0.184615384615385,-0.169230769230769,
-0.153846153846154,-0.138461538461538,-0.123076923076923,-0.107692307692308,
-0.0923076923076923,-0.0769230769230769,-0.0615384615384615,-0.0461538461538462,
-0.0307692307692308,-0.0153846153846154,0.),(-1.,1.),.UNSPECIFIED.)
GEOMETRIC_REPRESENTATION_ITEM()
RATIONAL_B_SPLINE_SURFACE(((1.,1.),(1.,1.),(1.,1.),(1.,1.),(1.,1.),(1.,
1.),(1.,1.),(1.,1.),(1.,1.),(1.,1.),(1.,1.),(1.,1.),(1.,1.),(1.,1.),(1.,
1.),(1.,1.),(1.,1.),(1.,1.),(1.,1.),(1.,1.),(1.,1.),(1.,1.),(1.,1.),(1.,
1.),(1.,1.),(1.,1.),(1.,1.),(1.,1.),(1.,1.),(1.,1.),(1.,1.),(1.,1.),(1.,
1.),(1.,1.),(1.,1.),(1.,1.),(1.,1.),(1.,1.),(1.,1.),(1.,1.),(1.,1.),(1.,
1.),(1.,1.),(1.,1.),(1.,1.),(1.,1.),(1.,1.),(1.,1.),(1.,1.),(1.,1.),(1.,
1.),(1.,1.),(1.,1.),(1.,1.),(1.,1.),(1.,1.),(1.,1.),(1.,1.),(1.,1.),(1.,
1.),(1.,1.),(1.,1.),(1.,1.),(1.,1.),(1.,1.),(1.,1.),(1.,1.),(1.,1.),(1.,
1.),(1.,1.)))
REPRESENTATION_ITEM('')
SURFACE()
);
#117=(
BOUNDED_SURFACE()
B_SPLINE_SURFACE(5,1,((#54554,#54555),(#54556,#54557),(#54558,#54559),(#54560,
#54561),(#54562,#54563),(#54564,#54565),(#54566,#54567),(#54568,#54569),
(#54570,#54571),(#54572,#54573),(#54574,#54575),(#54576,#54577),(#54578,
#54579),(#54580,#54581),(#54582,#54583),(#54584,#54585),(#54586,#54587),
(#54588,#54589),(#54590,#54591),(#54592,#54593),(#54594,#54595),(#54596,
#54597),(#54598,#54599),(#54600,#54601),(#54602,#54603),(#54604,#54605),
(#54606,#54607),(#54608,#54609),(#54610,#54611),(#54612,#54613),(#54614,
#54615),(#54616,#54617),(#54618,#54619),(#54620,#54621),(#54622,#54623),
(#54624,#54625),(#54626,#54627),(#54628,#54629),(#54630,#54631),(#54632,
#54633),(#54634,#54635),(#54636,#54637),(#54638,#54639),(#54640,#54641),
(#54642,#54643),(#54644,#54645),(#54646,#54647),(#54648,#54649),(#54650,
#54651),(#54652,#54653),(#54654,#54655),(#54656,#54657),(#54658,#54659),
(#54660,#54661),(#54662,#54663),(#54664,#54665),(#54666,#54667),(#54668,
#54669),(#54670,#54671),(#54672,#54673),(#54674,#54675),(#54676,#54677),
(#54678,#54679),(#54680,#54681),(#54682,#54683),(#54684,#54685),(#54686,
#54687),(#54688,#54689),(#54690,#54691),(#54692,#54693)),.UNSPECIFIED.,
 .F.,.F.,.F.)
B_SPLINE_SURFACE_WITH_KNOTS((6,1,1,1,1,1,1,1,1,1,1,1,1,1,1,1,1,1,1,1,1,
1,1,1,1,1,1,1,1,1,1,1,1,1,1,1,1,1,1,1,1,1,1,1,1,1,1,1,1,1,1,1,1,1,1,1,1,
1,1,1,1,1,1,1,1,6),(2,2),(-1.,-0.984615384615383,-0.969230769230768,-0.953846153846152,
-0.938461538461537,-0.923076923076922,-0.907692307692306,-0.892307692307691,
-0.876923076923076,-0.86153846153846,-0.846153846153845,-0.83076923076923,
-0.815384615384614,-0.799999999999999,-0.784615384615384,-0.769230769230768,
-0.753846153846153,-0.738461538461538,-0.723076923076922,-0.707692307692307,
-0.692307692307692,-0.676923076923076,-0.661538461538461,-0.646153846153846,
-0.63076923076923,-0.615384615384615,-0.6,-0.584615384615384,-0.569230769230769,
-0.553846153846154,-0.538461538461538,-0.523076923076923,-0.507692307692308,
-0.492307692307692,-0.476923076923077,-0.461538461538462,-0.446153846153846,
-0.430769230769231,-0.415384615384615,-0.4,-0.384615384615385,-0.369230769230769,
-0.353846153846154,-0.338461538461538,-0.323076923076923,-0.307692307692308,
-0.292307692307692,-0.276923076923077,-0.261538461538462,-0.246153846153846,
-0.230769230769231,-0.215384615384615,-0.2,-0.184615384615385,-0.169230769230769,
-0.153846153846154,-0.138461538461538,-0.123076923076923,-0.107692307692308,
-0.0923076923076923,-0.0769230769230769,-0.0615384615384615,-0.0461538461538462,
-0.0307692307692308,-0.0153846153846154,0.),(-1.,1.),.UNSPECIFIED.)
GEOMETRIC_REPRESENTATION_ITEM()
RATIONAL_B_SPLINE_SURFACE(((1.,1.),(1.,1.),(1.,1.),(1.,1.),(1.,1.),(1.,
1.),(1.,1.),(1.,1.),(1.,1.),(1.,1.),(1.,1.),(1.,1.),(1.,1.),(1.,1.),(1.,
1.),(1.,1.),(1.,1.),(1.,1.),(1.,1.),(1.,1.),(1.,1.),(1.,1.),(1.,1.),(1.,
1.),(1.,1.),(1.,1.),(1.,1.),(1.,1.),(1.,1.),(1.,1.),(1.,1.),(1.,1.),(1.,
1.),(1.,1.),(1.,1.),(1.,1.),(1.,1.),(1.,1.),(1.,1.),(1.,1.),(1.,1.),(1.,
1.),(1.,1.),(1.,1.),(1.,1.),(1.,1.),(1.,1.),(1.,1.),(1.,1.),(1.,1.),(1.,
1.),(1.,1.),(1.,1.),(1.,1.),(1.,1.),(1.,1.),(1.,1.),(1.,1.),(1.,1.),(1.,
1.),(1.,1.),(1.,1.),(1.,1.),(1.,1.),(1.,1.),(1.,1.),(1.,1.),(1.,1.),(1.,
1.),(1.,1.)))
REPRESENTATION_ITEM('')
SURFACE()
);
#118=(
BOUNDED_SURFACE()
B_SPLINE_SURFACE(5,1,((#54766,#54767),(#54768,#54769),(#54770,#54771),(#54772,
#54773),(#54774,#54775),(#54776,#54777),(#54778,#54779),(#54780,#54781),
(#54782,#54783),(#54784,#54785),(#54786,#54787),(#54788,#54789),(#54790,
#54791),(#54792,#54793),(#54794,#54795),(#54796,#54797),(#54798,#54799),
(#54800,#54801),(#54802,#54803),(#54804,#54805),(#54806,#54807),(#54808,
#54809),(#54810,#54811),(#54812,#54813),(#54814,#54815),(#54816,#54817),
(#54818,#54819),(#54820,#54821),(#54822,#54823),(#54824,#54825),(#54826,
#54827),(#54828,#54829),(#54830,#54831),(#54832,#54833),(#54834,#54835),
(#54836,#54837),(#54838,#54839),(#54840,#54841),(#54842,#54843),(#54844,
#54845),(#54846,#54847),(#54848,#54849),(#54850,#54851),(#54852,#54853),
(#54854,#54855),(#54856,#54857),(#54858,#54859),(#54860,#54861),(#54862,
#54863),(#54864,#54865),(#54866,#54867),(#54868,#54869),(#54870,#54871),
(#54872,#54873),(#54874,#54875),(#54876,#54877),(#54878,#54879),(#54880,
#54881),(#54882,#54883),(#54884,#54885),(#54886,#54887),(#54888,#54889),
(#54890,#54891),(#54892,#54893),(#54894,#54895),(#54896,#54897),(#54898,
#54899),(#54900,#54901),(#54902,#54903),(#54904,#54905)),.UNSPECIFIED.,
 .F.,.F.,.F.)
B_SPLINE_SURFACE_WITH_KNOTS((6,1,1,1,1,1,1,1,1,1,1,1,1,1,1,1,1,1,1,1,1,
1,1,1,1,1,1,1,1,1,1,1,1,1,1,1,1,1,1,1,1,1,1,1,1,1,1,1,1,1,1,1,1,1,1,1,1,
1,1,1,1,1,1,1,1,6),(2,2),(-1.,-0.984615384615383,-0.969230769230768,-0.953846153846152,
-0.938461538461537,-0.923076923076922,-0.907692307692306,-0.892307692307691,
-0.876923076923076,-0.86153846153846,-0.846153846153845,-0.83076923076923,
-0.815384615384614,-0.799999999999999,-0.784615384615384,-0.769230769230768,
-0.753846153846153,-0.738461538461538,-0.723076923076922,-0.707692307692307,
-0.692307692307692,-0.676923076923076,-0.661538461538461,-0.646153846153846,
-0.63076923076923,-0.615384615384615,-0.6,-0.584615384615384,-0.569230769230769,
-0.553846153846154,-0.538461538461538,-0.523076923076923,-0.507692307692308,
-0.492307692307692,-0.476923076923077,-0.461538461538462,-0.446153846153846,
-0.430769230769231,-0.415384615384615,-0.4,-0.384615384615385,-0.369230769230769,
-0.353846153846154,-0.338461538461538,-0.323076923076923,-0.307692307692308,
-0.292307692307692,-0.276923076923077,-0.261538461538462,-0.246153846153846,
-0.230769230769231,-0.215384615384615,-0.2,-0.184615384615385,-0.169230769230769,
-0.153846153846154,-0.138461538461538,-0.123076923076923,-0.107692307692308,
-0.0923076923076923,-0.0769230769230769,-0.0615384615384615,-0.0461538461538462,
-0.0307692307692308,-0.0153846153846154,0.),(-1.,1.),.UNSPECIFIED.)
GEOMETRIC_REPRESENTATION_ITEM()
RATIONAL_B_SPLINE_SURFACE(((1.,1.),(1.,1.),(1.,1.),(1.,1.),(1.,1.),(1.,
1.),(1.,1.),(1.,1.),(1.,1.),(1.,1.),(1.,1.),(1.,1.),(1.,1.),(1.,1.),(1.,
1.),(1.,1.),(1.,1.),(1.,1.),(1.,1.),(1.,1.),(1.,1.),(1.,1.),(1.,1.),(1.,
1.),(1.,1.),(1.,1.),(1.,1.),(1.,1.),(1.,1.),(1.,1.),(1.,1.),(1.,1.),(1.,
1.),(1.,1.),(1.,1.),(1.,1.),(1.,1.),(1.,1.),(1.,1.),(1.,1.),(1.,1.),(1.,
1.),(1.,1.),(1.,1.),(1.,1.),(1.,1.),(1.,1.),(1.,1.),(1.,1.),(1.,1.),(1.,
1.),(1.,1.),(1.,1.),(1.,1.),(1.,1.),(1.,1.),(1.,1.),(1.,1.),(1.,1.),(1.,
1.),(1.,1.),(1.,1.),(1.,1.),(1.,1.),(1.,1.),(1.,1.),(1.,1.),(1.,1.),(1.,
1.),(1.,1.)))
REPRESENTATION_ITEM('')
SURFACE()
);
#119=(
BOUNDED_SURFACE()
B_SPLINE_SURFACE(5,1,((#54996,#54997),(#54998,#54999),(#55000,#55001),(#55002,
#55003),(#55004,#55005),(#55006,#55007),(#55008,#55009),(#55010,#55011),
(#55012,#55013),(#55014,#55015),(#55016,#55017),(#55018,#55019),(#55020,
#55021),(#55022,#55023),(#55024,#55025),(#55026,#55027),(#55028,#55029),
(#55030,#55031),(#55032,#55033),(#55034,#55035),(#55036,#55037),(#55038,
#55039),(#55040,#55041),(#55042,#55043),(#55044,#55045),(#55046,#55047),
(#55048,#55049),(#55050,#55051),(#55052,#55053),(#55054,#55055),(#55056,
#55057),(#55058,#55059),(#55060,#55061),(#55062,#55063),(#55064,#55065),
(#55066,#55067),(#55068,#55069),(#55070,#55071),(#55072,#55073),(#55074,
#55075),(#55076,#55077),(#55078,#55079),(#55080,#55081),(#55082,#55083),
(#55084,#55085),(#55086,#55087),(#55088,#55089),(#55090,#55091),(#55092,
#55093),(#55094,#55095),(#55096,#55097),(#55098,#55099),(#55100,#55101),
(#55102,#55103),(#55104,#55105),(#55106,#55107),(#55108,#55109),(#55110,
#55111),(#55112,#55113),(#55114,#55115),(#55116,#55117),(#55118,#55119),
(#55120,#55121),(#55122,#55123),(#55124,#55125),(#55126,#55127),(#55128,
#55129),(#55130,#55131),(#55132,#55133),(#55134,#55135)),.UNSPECIFIED.,
 .F.,.F.,.F.)
B_SPLINE_SURFACE_WITH_KNOTS((6,1,1,1,1,1,1,1,1,1,1,1,1,1,1,1,1,1,1,1,1,
1,1,1,1,1,1,1,1,1,1,1,1,1,1,1,1,1,1,1,1,1,1,1,1,1,1,1,1,1,1,1,1,1,1,1,1,
1,1,1,1,1,1,1,1,6),(2,2),(-1.,-0.984615384615383,-0.969230769230768,-0.953846153846152,
-0.938461538461537,-0.923076923076922,-0.907692307692306,-0.892307692307691,
-0.876923076923076,-0.86153846153846,-0.846153846153845,-0.83076923076923,
-0.815384615384614,-0.799999999999999,-0.784615384615384,-0.769230769230768,
-0.753846153846153,-0.738461538461538,-0.723076923076922,-0.707692307692307,
-0.692307692307692,-0.676923076923076,-0.661538461538461,-0.646153846153846,
-0.63076923076923,-0.615384615384615,-0.6,-0.584615384615384,-0.569230769230769,
-0.553846153846154,-0.538461538461538,-0.523076923076923,-0.507692307692308,
-0.492307692307692,-0.476923076923077,-0.461538461538462,-0.446153846153846,
-0.430769230769231,-0.415384615384615,-0.4,-0.384615384615385,-0.369230769230769,
-0.353846153846154,-0.338461538461538,-0.323076923076923,-0.307692307692308,
-0.292307692307692,-0.276923076923077,-0.261538461538462,-0.246153846153846,
-0.230769230769231,-0.215384615384615,-0.2,-0.184615384615385,-0.169230769230769,
-0.153846153846154,-0.138461538461538,-0.123076923076923,-0.107692307692308,
-0.0923076923076923,-0.0769230769230769,-0.0615384615384615,-0.0461538461538462,
-0.0307692307692308,-0.0153846153846154,0.),(-1.,1.),.UNSPECIFIED.)
GEOMETRIC_REPRESENTATION_ITEM()
RATIONAL_B_SPLINE_SURFACE(((1.,1.),(1.,1.),(1.,1.),(1.,1.),(1.,1.),(1.,
1.),(1.,1.),(1.,1.),(1.,1.),(1.,1.),(1.,1.),(1.,1.),(1.,1.),(1.,1.),(1.,
1.),(1.,1.),(1.,1.),(1.,1.),(1.,1.),(1.,1.),(1.,1.),(1.,1.),(1.,1.),(1.,
1.),(1.,1.),(1.,1.),(1.,1.),(1.,1.),(1.,1.),(1.,1.),(1.,1.),(1.,1.),(1.,
1.),(1.,1.),(1.,1.),(1.,1.),(1.,1.),(1.,1.),(1.,1.),(1.,1.),(1.,1.),(1.,
1.),(1.,1.),(1.,1.),(1.,1.),(1.,1.),(1.,1.),(1.,1.),(1.,1.),(1.,1.),(1.,
1.),(1.,1.),(1.,1.),(1.,1.),(1.,1.),(1.,1.),(1.,1.),(1.,1.),(1.,1.),(1.,
1.),(1.,1.),(1.,1.),(1.,1.),(1.,1.),(1.,1.),(1.,1.),(1.,1.),(1.,1.),(1.,
1.),(1.,1.)))
REPRESENTATION_ITEM('')
SURFACE()
);
#120=(
BOUNDED_SURFACE()
B_SPLINE_SURFACE(5,1,((#55208,#55209),(#55210,#55211),(#55212,#55213),(#55214,
#55215),(#55216,#55217),(#55218,#55219),(#55220,#55221),(#55222,#55223),
(#55224,#55225),(#55226,#55227),(#55228,#55229),(#55230,#55231),(#55232,
#55233),(#55234,#55235),(#55236,#55237),(#55238,#55239),(#55240,#55241),
(#55242,#55243),(#55244,#55245),(#55246,#55247),(#55248,#55249),(#55250,
#55251),(#55252,#55253),(#55254,#55255),(#55256,#55257),(#55258,#55259),
(#55260,#55261),(#55262,#55263),(#55264,#55265),(#55266,#55267),(#55268,
#55269),(#55270,#55271),(#55272,#55273),(#55274,#55275),(#55276,#55277),
(#55278,#55279),(#55280,#55281),(#55282,#55283),(#55284,#55285),(#55286,
#55287),(#55288,#55289),(#55290,#55291),(#55292,#55293),(#55294,#55295),
(#55296,#55297),(#55298,#55299),(#55300,#55301),(#55302,#55303),(#55304,
#55305),(#55306,#55307),(#55308,#55309),(#55310,#55311),(#55312,#55313),
(#55314,#55315),(#55316,#55317),(#55318,#55319),(#55320,#55321),(#55322,
#55323),(#55324,#55325),(#55326,#55327),(#55328,#55329),(#55330,#55331),
(#55332,#55333),(#55334,#55335),(#55336,#55337),(#55338,#55339),(#55340,
#55341),(#55342,#55343),(#55344,#55345),(#55346,#55347)),.UNSPECIFIED.,
 .F.,.F.,.F.)
B_SPLINE_SURFACE_WITH_KNOTS((6,1,1,1,1,1,1,1,1,1,1,1,1,1,1,1,1,1,1,1,1,
1,1,1,1,1,1,1,1,1,1,1,1,1,1,1,1,1,1,1,1,1,1,1,1,1,1,1,1,1,1,1,1,1,1,1,1,
1,1,1,1,1,1,1,1,6),(2,2),(-1.,-0.984615384615383,-0.969230769230768,-0.953846153846152,
-0.938461538461537,-0.923076923076922,-0.907692307692306,-0.892307692307691,
-0.876923076923076,-0.86153846153846,-0.846153846153845,-0.83076923076923,
-0.815384615384614,-0.799999999999999,-0.784615384615384,-0.769230769230768,
-0.753846153846153,-0.738461538461538,-0.723076923076922,-0.707692307692307,
-0.692307692307692,-0.676923076923076,-0.661538461538461,-0.646153846153846,
-0.63076923076923,-0.615384615384615,-0.6,-0.584615384615384,-0.569230769230769,
-0.553846153846154,-0.538461538461538,-0.523076923076923,-0.507692307692308,
-0.492307692307692,-0.476923076923077,-0.461538461538462,-0.446153846153846,
-0.430769230769231,-0.415384615384615,-0.4,-0.384615384615385,-0.369230769230769,
-0.353846153846154,-0.338461538461538,-0.323076923076923,-0.307692307692308,
-0.292307692307692,-0.276923076923077,-0.261538461538462,-0.246153846153846,
-0.230769230769231,-0.215384615384615,-0.2,-0.184615384615385,-0.169230769230769,
-0.153846153846154,-0.138461538461538,-0.123076923076923,-0.107692307692308,
-0.0923076923076923,-0.0769230769230769,-0.0615384615384615,-0.0461538461538462,
-0.0307692307692308,-0.0153846153846154,0.),(-1.,1.),.UNSPECIFIED.)
GEOMETRIC_REPRESENTATION_ITEM()
RATIONAL_B_SPLINE_SURFACE(((1.,1.),(1.,1.),(1.,1.),(1.,1.),(1.,1.),(1.,
1.),(1.,1.),(1.,1.),(1.,1.),(1.,1.),(1.,1.),(1.,1.),(1.,1.),(1.,1.),(1.,
1.),(1.,1.),(1.,1.),(1.,1.),(1.,1.),(1.,1.),(1.,1.),(1.,1.),(1.,1.),(1.,
1.),(1.,1.),(1.,1.),(1.,1.),(1.,1.),(1.,1.),(1.,1.),(1.,1.),(1.,1.),(1.,
1.),(1.,1.),(1.,1.),(1.,1.),(1.,1.),(1.,1.),(1.,1.),(1.,1.),(1.,1.),(1.,
1.),(1.,1.),(1.,1.),(1.,1.),(1.,1.),(1.,1.),(1.,1.),(1.,1.),(1.,1.),(1.,
1.),(1.,1.),(1.,1.),(1.,1.),(1.,1.),(1.,1.),(1.,1.),(1.,1.),(1.,1.),(1.,
1.),(1.,1.),(1.,1.),(1.,1.),(1.,1.),(1.,1.),(1.,1.),(1.,1.),(1.,1.),(1.,
1.),(1.,1.)))
REPRESENTATION_ITEM('')
SURFACE()
);
#121=(
BOUNDED_SURFACE()
B_SPLINE_SURFACE(5,1,((#55438,#55439),(#55440,#55441),(#55442,#55443),(#55444,
#55445),(#55446,#55447),(#55448,#55449),(#55450,#55451),(#55452,#55453),
(#55454,#55455),(#55456,#55457),(#55458,#55459),(#55460,#55461),(#55462,
#55463),(#55464,#55465),(#55466,#55467),(#55468,#55469),(#55470,#55471),
(#55472,#55473),(#55474,#55475),(#55476,#55477),(#55478,#55479),(#55480,
#55481),(#55482,#55483),(#55484,#55485),(#55486,#55487),(#55488,#55489),
(#55490,#55491),(#55492,#55493),(#55494,#55495),(#55496,#55497),(#55498,
#55499),(#55500,#55501),(#55502,#55503),(#55504,#55505),(#55506,#55507),
(#55508,#55509),(#55510,#55511),(#55512,#55513),(#55514,#55515),(#55516,
#55517),(#55518,#55519),(#55520,#55521),(#55522,#55523),(#55524,#55525),
(#55526,#55527),(#55528,#55529),(#55530,#55531),(#55532,#55533),(#55534,
#55535),(#55536,#55537),(#55538,#55539),(#55540,#55541),(#55542,#55543),
(#55544,#55545),(#55546,#55547),(#55548,#55549),(#55550,#55551),(#55552,
#55553),(#55554,#55555),(#55556,#55557),(#55558,#55559),(#55560,#55561),
(#55562,#55563),(#55564,#55565),(#55566,#55567),(#55568,#55569),(#55570,
#55571),(#55572,#55573),(#55574,#55575),(#55576,#55577)),.UNSPECIFIED.,
 .F.,.F.,.F.)
B_SPLINE_SURFACE_WITH_KNOTS((6,1,1,1,1,1,1,1,1,1,1,1,1,1,1,1,1,1,1,1,1,
1,1,1,1,1,1,1,1,1,1,1,1,1,1,1,1,1,1,1,1,1,1,1,1,1,1,1,1,1,1,1,1,1,1,1,1,
1,1,1,1,1,1,1,1,6),(2,2),(-1.,-0.984615384615383,-0.969230769230768,-0.953846153846152,
-0.938461538461537,-0.923076923076922,-0.907692307692306,-0.892307692307691,
-0.876923076923076,-0.86153846153846,-0.846153846153845,-0.83076923076923,
-0.815384615384614,-0.799999999999999,-0.784615384615384,-0.769230769230768,
-0.753846153846153,-0.738461538461538,-0.723076923076922,-0.707692307692307,
-0.692307692307692,-0.676923076923076,-0.661538461538461,-0.646153846153846,
-0.63076923076923,-0.615384615384615,-0.6,-0.584615384615384,-0.569230769230769,
-0.553846153846154,-0.538461538461538,-0.523076923076923,-0.507692307692308,
-0.492307692307692,-0.476923076923077,-0.461538461538462,-0.446153846153846,
-0.430769230769231,-0.415384615384615,-0.4,-0.384615384615385,-0.369230769230769,
-0.353846153846154,-0.338461538461538,-0.323076923076923,-0.307692307692308,
-0.292307692307692,-0.276923076923077,-0.261538461538462,-0.246153846153846,
-0.230769230769231,-0.215384615384615,-0.2,-0.184615384615385,-0.169230769230769,
-0.153846153846154,-0.138461538461538,-0.123076923076923,-0.107692307692308,
-0.0923076923076923,-0.0769230769230769,-0.0615384615384615,-0.0461538461538462,
-0.0307692307692308,-0.0153846153846154,0.),(-1.,1.),.UNSPECIFIED.)
GEOMETRIC_REPRESENTATION_ITEM()
RATIONAL_B_SPLINE_SURFACE(((1.,1.),(1.,1.),(1.,1.),(1.,1.),(1.,1.),(1.,
1.),(1.,1.),(1.,1.),(1.,1.),(1.,1.),(1.,1.),(1.,1.),(1.,1.),(1.,1.),(1.,
1.),(1.,1.),(1.,1.),(1.,1.),(1.,1.),(1.,1.),(1.,1.),(1.,1.),(1.,1.),(1.,
1.),(1.,1.),(1.,1.),(1.,1.),(1.,1.),(1.,1.),(1.,1.),(1.,1.),(1.,1.),(1.,
1.),(1.,1.),(1.,1.),(1.,1.),(1.,1.),(1.,1.),(1.,1.),(1.,1.),(1.,1.),(1.,
1.),(1.,1.),(1.,1.),(1.,1.),(1.,1.),(1.,1.),(1.,1.),(1.,1.),(1.,1.),(1.,
1.),(1.,1.),(1.,1.),(1.,1.),(1.,1.),(1.,1.),(1.,1.),(1.,1.),(1.,1.),(1.,
1.),(1.,1.),(1.,1.),(1.,1.),(1.,1.),(1.,1.),(1.,1.),(1.,1.),(1.,1.),(1.,
1.),(1.,1.)))
REPRESENTATION_ITEM('')
SURFACE()
);
#122=(
BOUNDED_SURFACE()
B_SPLINE_SURFACE(5,1,((#55650,#55651),(#55652,#55653),(#55654,#55655),(#55656,
#55657),(#55658,#55659),(#55660,#55661),(#55662,#55663),(#55664,#55665),
(#55666,#55667),(#55668,#55669),(#55670,#55671),(#55672,#55673),(#55674,
#55675),(#55676,#55677),(#55678,#55679),(#55680,#55681),(#55682,#55683),
(#55684,#55685),(#55686,#55687),(#55688,#55689),(#55690,#55691),(#55692,
#55693),(#55694,#55695),(#55696,#55697),(#55698,#55699),(#55700,#55701),
(#55702,#55703),(#55704,#55705),(#55706,#55707),(#55708,#55709),(#55710,
#55711),(#55712,#55713),(#55714,#55715),(#55716,#55717),(#55718,#55719),
(#55720,#55721),(#55722,#55723),(#55724,#55725),(#55726,#55727),(#55728,
#55729),(#55730,#55731),(#55732,#55733),(#55734,#55735),(#55736,#55737),
(#55738,#55739),(#55740,#55741),(#55742,#55743),(#55744,#55745),(#55746,
#55747),(#55748,#55749),(#55750,#55751),(#55752,#55753),(#55754,#55755),
(#55756,#55757),(#55758,#55759),(#55760,#55761),(#55762,#55763),(#55764,
#55765),(#55766,#55767),(#55768,#55769),(#55770,#55771),(#55772,#55773),
(#55774,#55775),(#55776,#55777),(#55778,#55779),(#55780,#55781),(#55782,
#55783),(#55784,#55785),(#55786,#55787),(#55788,#55789)),.UNSPECIFIED.,
 .F.,.F.,.F.)
B_SPLINE_SURFACE_WITH_KNOTS((6,1,1,1,1,1,1,1,1,1,1,1,1,1,1,1,1,1,1,1,1,
1,1,1,1,1,1,1,1,1,1,1,1,1,1,1,1,1,1,1,1,1,1,1,1,1,1,1,1,1,1,1,1,1,1,1,1,
1,1,1,1,1,1,1,1,6),(2,2),(-1.,-0.984615384615383,-0.969230769230768,-0.953846153846152,
-0.938461538461537,-0.923076923076922,-0.907692307692306,-0.892307692307691,
-0.876923076923076,-0.86153846153846,-0.846153846153845,-0.83076923076923,
-0.815384615384614,-0.799999999999999,-0.784615384615384,-0.769230769230768,
-0.753846153846153,-0.738461538461538,-0.723076923076922,-0.707692307692307,
-0.692307692307692,-0.676923076923076,-0.661538461538461,-0.646153846153846,
-0.63076923076923,-0.615384615384615,-0.6,-0.584615384615384,-0.569230769230769,
-0.553846153846154,-0.538461538461538,-0.523076923076923,-0.507692307692308,
-0.492307692307692,-0.476923076923077,-0.461538461538462,-0.446153846153846,
-0.430769230769231,-0.415384615384615,-0.4,-0.384615384615385,-0.369230769230769,
-0.353846153846154,-0.338461538461538,-0.323076923076923,-0.307692307692308,
-0.292307692307692,-0.276923076923077,-0.261538461538462,-0.246153846153846,
-0.230769230769231,-0.215384615384615,-0.2,-0.184615384615385,-0.169230769230769,
-0.153846153846154,-0.138461538461538,-0.123076923076923,-0.107692307692308,
-0.0923076923076923,-0.0769230769230769,-0.0615384615384615,-0.0461538461538462,
-0.0307692307692308,-0.0153846153846154,0.),(-1.,1.),.UNSPECIFIED.)
GEOMETRIC_REPRESENTATION_ITEM()
RATIONAL_B_SPLINE_SURFACE(((1.,1.),(1.,1.),(1.,1.),(1.,1.),(1.,1.),(1.,
1.),(1.,1.),(1.,1.),(1.,1.),(1.,1.),(1.,1.),(1.,1.),(1.,1.),(1.,1.),(1.,
1.),(1.,1.),(1.,1.),(1.,1.),(1.,1.),(1.,1.),(1.,1.),(1.,1.),(1.,1.),(1.,
1.),(1.,1.),(1.,1.),(1.,1.),(1.,1.),(1.,1.),(1.,1.),(1.,1.),(1.,1.),(1.,
1.),(1.,1.),(1.,1.),(1.,1.),(1.,1.),(1.,1.),(1.,1.),(1.,1.),(1.,1.),(1.,
1.),(1.,1.),(1.,1.),(1.,1.),(1.,1.),(1.,1.),(1.,1.),(1.,1.),(1.,1.),(1.,
1.),(1.,1.),(1.,1.),(1.,1.),(1.,1.),(1.,1.),(1.,1.),(1.,1.),(1.,1.),(1.,
1.),(1.,1.),(1.,1.),(1.,1.),(1.,1.),(1.,1.),(1.,1.),(1.,1.),(1.,1.),(1.,
1.),(1.,1.)))
REPRESENTATION_ITEM('')
SURFACE()
);
#123=(
BOUNDED_SURFACE()
B_SPLINE_SURFACE(5,1,((#55880,#55881),(#55882,#55883),(#55884,#55885),(#55886,
#55887),(#55888,#55889),(#55890,#55891),(#55892,#55893),(#55894,#55895),
(#55896,#55897),(#55898,#55899),(#55900,#55901),(#55902,#55903),(#55904,
#55905),(#55906,#55907),(#55908,#55909),(#55910,#55911),(#55912,#55913),
(#55914,#55915),(#55916,#55917),(#55918,#55919),(#55920,#55921),(#55922,
#55923),(#55924,#55925),(#55926,#55927),(#55928,#55929),(#55930,#55931),
(#55932,#55933),(#55934,#55935),(#55936,#55937),(#55938,#55939),(#55940,
#55941),(#55942,#55943),(#55944,#55945),(#55946,#55947),(#55948,#55949),
(#55950,#55951),(#55952,#55953),(#55954,#55955),(#55956,#55957),(#55958,
#55959),(#55960,#55961),(#55962,#55963),(#55964,#55965),(#55966,#55967),
(#55968,#55969),(#55970,#55971),(#55972,#55973),(#55974,#55975),(#55976,
#55977),(#55978,#55979),(#55980,#55981),(#55982,#55983),(#55984,#55985),
(#55986,#55987),(#55988,#55989),(#55990,#55991),(#55992,#55993),(#55994,
#55995),(#55996,#55997),(#55998,#55999),(#56000,#56001),(#56002,#56003),
(#56004,#56005),(#56006,#56007),(#56008,#56009),(#56010,#56011),(#56012,
#56013),(#56014,#56015),(#56016,#56017),(#56018,#56019)),.UNSPECIFIED.,
 .F.,.F.,.F.)
B_SPLINE_SURFACE_WITH_KNOTS((6,1,1,1,1,1,1,1,1,1,1,1,1,1,1,1,1,1,1,1,1,
1,1,1,1,1,1,1,1,1,1,1,1,1,1,1,1,1,1,1,1,1,1,1,1,1,1,1,1,1,1,1,1,1,1,1,1,
1,1,1,1,1,1,1,1,6),(2,2),(-1.,-0.984615384615383,-0.969230769230768,-0.953846153846152,
-0.938461538461537,-0.923076923076922,-0.907692307692306,-0.892307692307691,
-0.876923076923076,-0.86153846153846,-0.846153846153845,-0.83076923076923,
-0.815384615384614,-0.799999999999999,-0.784615384615384,-0.769230769230768,
-0.753846153846153,-0.738461538461538,-0.723076923076922,-0.707692307692307,
-0.692307692307692,-0.676923076923076,-0.661538461538461,-0.646153846153846,
-0.63076923076923,-0.615384615384615,-0.6,-0.584615384615384,-0.569230769230769,
-0.553846153846154,-0.538461538461538,-0.523076923076923,-0.507692307692308,
-0.492307692307692,-0.476923076923077,-0.461538461538462,-0.446153846153846,
-0.430769230769231,-0.415384615384615,-0.4,-0.384615384615385,-0.369230769230769,
-0.353846153846154,-0.338461538461538,-0.323076923076923,-0.307692307692308,
-0.292307692307692,-0.276923076923077,-0.261538461538462,-0.246153846153846,
-0.230769230769231,-0.215384615384615,-0.2,-0.184615384615385,-0.169230769230769,
-0.153846153846154,-0.138461538461538,-0.123076923076923,-0.107692307692308,
-0.0923076923076923,-0.0769230769230769,-0.0615384615384615,-0.0461538461538462,
-0.0307692307692308,-0.0153846153846154,0.),(-1.,1.),.UNSPECIFIED.)
GEOMETRIC_REPRESENTATION_ITEM()
RATIONAL_B_SPLINE_SURFACE(((1.,1.),(1.,1.),(1.,1.),(1.,1.),(1.,1.),(1.,
1.),(1.,1.),(1.,1.),(1.,1.),(1.,1.),(1.,1.),(1.,1.),(1.,1.),(1.,1.),(1.,
1.),(1.,1.),(1.,1.),(1.,1.),(1.,1.),(1.,1.),(1.,1.),(1.,1.),(1.,1.),(1.,
1.),(1.,1.),(1.,1.),(1.,1.),(1.,1.),(1.,1.),(1.,1.),(1.,1.),(1.,1.),(1.,
1.),(1.,1.),(1.,1.),(1.,1.),(1.,1.),(1.,1.),(1.,1.),(1.,1.),(1.,1.),(1.,
1.),(1.,1.),(1.,1.),(1.,1.),(1.,1.),(1.,1.),(1.,1.),(1.,1.),(1.,1.),(1.,
1.),(1.,1.),(1.,1.),(1.,1.),(1.,1.),(1.,1.),(1.,1.),(1.,1.),(1.,1.),(1.,
1.),(1.,1.),(1.,1.),(1.,1.),(1.,1.),(1.,1.),(1.,1.),(1.,1.),(1.,1.),(1.,
1.),(1.,1.)))
REPRESENTATION_ITEM('')
SURFACE()
);
#124=(
BOUNDED_SURFACE()
B_SPLINE_SURFACE(5,1,((#56092,#56093),(#56094,#56095),(#56096,#56097),(#56098,
#56099),(#56100,#56101),(#56102,#56103),(#56104,#56105),(#56106,#56107),
(#56108,#56109),(#56110,#56111),(#56112,#56113),(#56114,#56115),(#56116,
#56117),(#56118,#56119),(#56120,#56121),(#56122,#56123),(#56124,#56125),
(#56126,#56127),(#56128,#56129),(#56130,#56131),(#56132,#56133),(#56134,
#56135),(#56136,#56137),(#56138,#56139),(#56140,#56141),(#56142,#56143),
(#56144,#56145),(#56146,#56147),(#56148,#56149),(#56150,#56151),(#56152,
#56153),(#56154,#56155),(#56156,#56157),(#56158,#56159),(#56160,#56161),
(#56162,#56163),(#56164,#56165),(#56166,#56167),(#56168,#56169),(#56170,
#56171),(#56172,#56173),(#56174,#56175),(#56176,#56177),(#56178,#56179),
(#56180,#56181),(#56182,#56183),(#56184,#56185),(#56186,#56187),(#56188,
#56189),(#56190,#56191),(#56192,#56193),(#56194,#56195),(#56196,#56197),
(#56198,#56199),(#56200,#56201),(#56202,#56203),(#56204,#56205),(#56206,
#56207),(#56208,#56209),(#56210,#56211),(#56212,#56213),(#56214,#56215),
(#56216,#56217),(#56218,#56219),(#56220,#56221),(#56222,#56223),(#56224,
#56225),(#56226,#56227),(#56228,#56229),(#56230,#56231)),.UNSPECIFIED.,
 .F.,.F.,.F.)
B_SPLINE_SURFACE_WITH_KNOTS((6,1,1,1,1,1,1,1,1,1,1,1,1,1,1,1,1,1,1,1,1,
1,1,1,1,1,1,1,1,1,1,1,1,1,1,1,1,1,1,1,1,1,1,1,1,1,1,1,1,1,1,1,1,1,1,1,1,
1,1,1,1,1,1,1,1,6),(2,2),(-1.,-0.984615384615383,-0.969230769230768,-0.953846153846152,
-0.938461538461537,-0.923076923076922,-0.907692307692306,-0.892307692307691,
-0.876923076923076,-0.86153846153846,-0.846153846153845,-0.83076923076923,
-0.815384615384614,-0.799999999999999,-0.784615384615384,-0.769230769230768,
-0.753846153846153,-0.738461538461538,-0.723076923076922,-0.707692307692307,
-0.692307692307692,-0.676923076923076,-0.661538461538461,-0.646153846153846,
-0.63076923076923,-0.615384615384615,-0.6,-0.584615384615384,-0.569230769230769,
-0.553846153846154,-0.538461538461538,-0.523076923076923,-0.507692307692308,
-0.492307692307692,-0.476923076923077,-0.461538461538462,-0.446153846153846,
-0.430769230769231,-0.415384615384615,-0.4,-0.384615384615385,-0.369230769230769,
-0.353846153846154,-0.338461538461538,-0.323076923076923,-0.307692307692308,
-0.292307692307692,-0.276923076923077,-0.261538461538462,-0.246153846153846,
-0.230769230769231,-0.215384615384615,-0.2,-0.184615384615385,-0.169230769230769,
-0.153846153846154,-0.138461538461538,-0.123076923076923,-0.107692307692308,
-0.0923076923076923,-0.0769230769230769,-0.0615384615384615,-0.0461538461538462,
-0.0307692307692308,-0.0153846153846154,0.),(-1.,1.),.UNSPECIFIED.)
GEOMETRIC_REPRESENTATION_ITEM()
RATIONAL_B_SPLINE_SURFACE(((1.,1.),(1.,1.),(1.,1.),(1.,1.),(1.,1.),(1.,
1.),(1.,1.),(1.,1.),(1.,1.),(1.,1.),(1.,1.),(1.,1.),(1.,1.),(1.,1.),(1.,
1.),(1.,1.),(1.,1.),(1.,1.),(1.,1.),(1.,1.),(1.,1.),(1.,1.),(1.,1.),(1.,
1.),(1.,1.),(1.,1.),(1.,1.),(1.,1.),(1.,1.),(1.,1.),(1.,1.),(1.,1.),(1.,
1.),(1.,1.),(1.,1.),(1.,1.),(1.,1.),(1.,1.),(1.,1.),(1.,1.),(1.,1.),(1.,
1.),(1.,1.),(1.,1.),(1.,1.),(1.,1.),(1.,1.),(1.,1.),(1.,1.),(1.,1.),(1.,
1.),(1.,1.),(1.,1.),(1.,1.),(1.,1.),(1.,1.),(1.,1.),(1.,1.),(1.,1.),(1.,
1.),(1.,1.),(1.,1.),(1.,1.),(1.,1.),(1.,1.),(1.,1.),(1.,1.),(1.,1.),(1.,
1.),(1.,1.)))
REPRESENTATION_ITEM('')
SURFACE()
);
#125=(
BOUNDED_SURFACE()
B_SPLINE_SURFACE(5,1,((#56322,#56323),(#56324,#56325),(#56326,#56327),(#56328,
#56329),(#56330,#56331),(#56332,#56333),(#56334,#56335),(#56336,#56337),
(#56338,#56339),(#56340,#56341),(#56342,#56343),(#56344,#56345),(#56346,
#56347),(#56348,#56349),(#56350,#56351),(#56352,#56353),(#56354,#56355),
(#56356,#56357),(#56358,#56359),(#56360,#56361),(#56362,#56363),(#56364,
#56365),(#56366,#56367),(#56368,#56369),(#56370,#56371),(#56372,#56373),
(#56374,#56375),(#56376,#56377),(#56378,#56379),(#56380,#56381),(#56382,
#56383),(#56384,#56385),(#56386,#56387),(#56388,#56389),(#56390,#56391),
(#56392,#56393),(#56394,#56395),(#56396,#56397),(#56398,#56399),(#56400,
#56401),(#56402,#56403),(#56404,#56405),(#56406,#56407),(#56408,#56409),
(#56410,#56411),(#56412,#56413),(#56414,#56415),(#56416,#56417),(#56418,
#56419),(#56420,#56421),(#56422,#56423),(#56424,#56425),(#56426,#56427),
(#56428,#56429),(#56430,#56431),(#56432,#56433),(#56434,#56435),(#56436,
#56437),(#56438,#56439),(#56440,#56441),(#56442,#56443),(#56444,#56445),
(#56446,#56447),(#56448,#56449),(#56450,#56451),(#56452,#56453),(#56454,
#56455),(#56456,#56457),(#56458,#56459),(#56460,#56461)),.UNSPECIFIED.,
 .F.,.F.,.F.)
B_SPLINE_SURFACE_WITH_KNOTS((6,1,1,1,1,1,1,1,1,1,1,1,1,1,1,1,1,1,1,1,1,
1,1,1,1,1,1,1,1,1,1,1,1,1,1,1,1,1,1,1,1,1,1,1,1,1,1,1,1,1,1,1,1,1,1,1,1,
1,1,1,1,1,1,1,1,6),(2,2),(-1.,-0.984615384615383,-0.969230769230768,-0.953846153846152,
-0.938461538461537,-0.923076923076922,-0.907692307692306,-0.892307692307691,
-0.876923076923076,-0.86153846153846,-0.846153846153845,-0.83076923076923,
-0.815384615384614,-0.799999999999999,-0.784615384615384,-0.769230769230768,
-0.753846153846153,-0.738461538461538,-0.723076923076922,-0.707692307692307,
-0.692307692307692,-0.676923076923076,-0.661538461538461,-0.646153846153846,
-0.63076923076923,-0.615384615384615,-0.6,-0.584615384615384,-0.569230769230769,
-0.553846153846154,-0.538461538461538,-0.523076923076923,-0.507692307692308,
-0.492307692307692,-0.476923076923077,-0.461538461538462,-0.446153846153846,
-0.430769230769231,-0.415384615384615,-0.4,-0.384615384615385,-0.369230769230769,
-0.353846153846154,-0.338461538461538,-0.323076923076923,-0.307692307692308,
-0.292307692307692,-0.276923076923077,-0.261538461538462,-0.246153846153846,
-0.230769230769231,-0.215384615384615,-0.2,-0.184615384615385,-0.169230769230769,
-0.153846153846154,-0.138461538461538,-0.123076923076923,-0.107692307692308,
-0.0923076923076923,-0.0769230769230769,-0.0615384615384615,-0.0461538461538462,
-0.0307692307692308,-0.0153846153846154,0.),(-1.,1.),.UNSPECIFIED.)
GEOMETRIC_REPRESENTATION_ITEM()
RATIONAL_B_SPLINE_SURFACE(((1.,1.),(1.,1.),(1.,1.),(1.,1.),(1.,1.),(1.,
1.),(1.,1.),(1.,1.),(1.,1.),(1.,1.),(1.,1.),(1.,1.),(1.,1.),(1.,1.),(1.,
1.),(1.,1.),(1.,1.),(1.,1.),(1.,1.),(1.,1.),(1.,1.),(1.,1.),(1.,1.),(1.,
1.),(1.,1.),(1.,1.),(1.,1.),(1.,1.),(1.,1.),(1.,1.),(1.,1.),(1.,1.),(1.,
1.),(1.,1.),(1.,1.),(1.,1.),(1.,1.),(1.,1.),(1.,1.),(1.,1.),(1.,1.),(1.,
1.),(1.,1.),(1.,1.),(1.,1.),(1.,1.),(1.,1.),(1.,1.),(1.,1.),(1.,1.),(1.,
1.),(1.,1.),(1.,1.),(1.,1.),(1.,1.),(1.,1.),(1.,1.),(1.,1.),(1.,1.),(1.,
1.),(1.,1.),(1.,1.),(1.,1.),(1.,1.),(1.,1.),(1.,1.),(1.,1.),(1.,1.),(1.,
1.),(1.,1.)))
REPRESENTATION_ITEM('')
SURFACE()
);
#126=(
BOUNDED_SURFACE()
B_SPLINE_SURFACE(5,1,((#56534,#56535),(#56536,#56537),(#56538,#56539),(#56540,
#56541),(#56542,#56543),(#56544,#56545),(#56546,#56547),(#56548,#56549),
(#56550,#56551),(#56552,#56553),(#56554,#56555),(#56556,#56557),(#56558,
#56559),(#56560,#56561),(#56562,#56563),(#56564,#56565),(#56566,#56567),
(#56568,#56569),(#56570,#56571),(#56572,#56573),(#56574,#56575),(#56576,
#56577),(#56578,#56579),(#56580,#56581),(#56582,#56583),(#56584,#56585),
(#56586,#56587),(#56588,#56589),(#56590,#56591),(#56592,#56593),(#56594,
#56595),(#56596,#56597),(#56598,#56599),(#56600,#56601),(#56602,#56603),
(#56604,#56605),(#56606,#56607),(#56608,#56609),(#56610,#56611),(#56612,
#56613),(#56614,#56615),(#56616,#56617),(#56618,#56619),(#56620,#56621),
(#56622,#56623),(#56624,#56625),(#56626,#56627),(#56628,#56629),(#56630,
#56631),(#56632,#56633),(#56634,#56635),(#56636,#56637),(#56638,#56639),
(#56640,#56641),(#56642,#56643),(#56644,#56645),(#56646,#56647),(#56648,
#56649),(#56650,#56651),(#56652,#56653),(#56654,#56655),(#56656,#56657),
(#56658,#56659),(#56660,#56661),(#56662,#56663),(#56664,#56665),(#56666,
#56667),(#56668,#56669),(#56670,#56671),(#56672,#56673)),.UNSPECIFIED.,
 .F.,.F.,.F.)
B_SPLINE_SURFACE_WITH_KNOTS((6,1,1,1,1,1,1,1,1,1,1,1,1,1,1,1,1,1,1,1,1,
1,1,1,1,1,1,1,1,1,1,1,1,1,1,1,1,1,1,1,1,1,1,1,1,1,1,1,1,1,1,1,1,1,1,1,1,
1,1,1,1,1,1,1,1,6),(2,2),(-1.,-0.984615384615383,-0.969230769230768,-0.953846153846152,
-0.938461538461537,-0.923076923076922,-0.907692307692306,-0.892307692307691,
-0.876923076923076,-0.86153846153846,-0.846153846153845,-0.83076923076923,
-0.815384615384614,-0.799999999999999,-0.784615384615384,-0.769230769230768,
-0.753846153846153,-0.738461538461538,-0.723076923076922,-0.707692307692307,
-0.692307692307692,-0.676923076923076,-0.661538461538461,-0.646153846153846,
-0.63076923076923,-0.615384615384615,-0.6,-0.584615384615384,-0.569230769230769,
-0.553846153846154,-0.538461538461538,-0.523076923076923,-0.507692307692308,
-0.492307692307692,-0.476923076923077,-0.461538461538462,-0.446153846153846,
-0.430769230769231,-0.415384615384615,-0.4,-0.384615384615385,-0.369230769230769,
-0.353846153846154,-0.338461538461538,-0.323076923076923,-0.307692307692308,
-0.292307692307692,-0.276923076923077,-0.261538461538462,-0.246153846153846,
-0.230769230769231,-0.215384615384615,-0.2,-0.184615384615385,-0.169230769230769,
-0.153846153846154,-0.138461538461538,-0.123076923076923,-0.107692307692308,
-0.0923076923076923,-0.0769230769230769,-0.0615384615384615,-0.0461538461538462,
-0.0307692307692308,-0.0153846153846154,0.),(-1.,1.),.UNSPECIFIED.)
GEOMETRIC_REPRESENTATION_ITEM()
RATIONAL_B_SPLINE_SURFACE(((1.,1.),(1.,1.),(1.,1.),(1.,1.),(1.,1.),(1.,
1.),(1.,1.),(1.,1.),(1.,1.),(1.,1.),(1.,1.),(1.,1.),(1.,1.),(1.,1.),(1.,
1.),(1.,1.),(1.,1.),(1.,1.),(1.,1.),(1.,1.),(1.,1.),(1.,1.),(1.,1.),(1.,
1.),(1.,1.),(1.,1.),(1.,1.),(1.,1.),(1.,1.),(1.,1.),(1.,1.),(1.,1.),(1.,
1.),(1.,1.),(1.,1.),(1.,1.),(1.,1.),(1.,1.),(1.,1.),(1.,1.),(1.,1.),(1.,
1.),(1.,1.),(1.,1.),(1.,1.),(1.,1.),(1.,1.),(1.,1.),(1.,1.),(1.,1.),(1.,
1.),(1.,1.),(1.,1.),(1.,1.),(1.,1.),(1.,1.),(1.,1.),(1.,1.),(1.,1.),(1.,
1.),(1.,1.),(1.,1.),(1.,1.),(1.,1.),(1.,1.),(1.,1.),(1.,1.),(1.,1.),(1.,
1.),(1.,1.)))
REPRESENTATION_ITEM('')
SURFACE()
);
#127=(
BOUNDED_SURFACE()
B_SPLINE_SURFACE(5,1,((#56764,#56765),(#56766,#56767),(#56768,#56769),(#56770,
#56771),(#56772,#56773),(#56774,#56775),(#56776,#56777),(#56778,#56779),
(#56780,#56781),(#56782,#56783),(#56784,#56785),(#56786,#56787),(#56788,
#56789),(#56790,#56791),(#56792,#56793),(#56794,#56795),(#56796,#56797),
(#56798,#56799),(#56800,#56801),(#56802,#56803),(#56804,#56805),(#56806,
#56807),(#56808,#56809),(#56810,#56811),(#56812,#56813),(#56814,#56815),
(#56816,#56817),(#56818,#56819),(#56820,#56821),(#56822,#56823),(#56824,
#56825),(#56826,#56827),(#56828,#56829),(#56830,#56831),(#56832,#56833),
(#56834,#56835),(#56836,#56837),(#56838,#56839),(#56840,#56841),(#56842,
#56843),(#56844,#56845),(#56846,#56847),(#56848,#56849),(#56850,#56851),
(#56852,#56853),(#56854,#56855),(#56856,#56857),(#56858,#56859),(#56860,
#56861),(#56862,#56863),(#56864,#56865),(#56866,#56867),(#56868,#56869),
(#56870,#56871),(#56872,#56873),(#56874,#56875),(#56876,#56877),(#56878,
#56879),(#56880,#56881),(#56882,#56883),(#56884,#56885),(#56886,#56887),
(#56888,#56889),(#56890,#56891),(#56892,#56893),(#56894,#56895),(#56896,
#56897),(#56898,#56899),(#56900,#56901),(#56902,#56903)),.UNSPECIFIED.,
 .F.,.F.,.F.)
B_SPLINE_SURFACE_WITH_KNOTS((6,1,1,1,1,1,1,1,1,1,1,1,1,1,1,1,1,1,1,1,1,
1,1,1,1,1,1,1,1,1,1,1,1,1,1,1,1,1,1,1,1,1,1,1,1,1,1,1,1,1,1,1,1,1,1,1,1,
1,1,1,1,1,1,1,1,6),(2,2),(-1.,-0.984615384615383,-0.969230769230768,-0.953846153846152,
-0.938461538461537,-0.923076923076922,-0.907692307692306,-0.892307692307691,
-0.876923076923076,-0.86153846153846,-0.846153846153845,-0.83076923076923,
-0.815384615384614,-0.799999999999999,-0.784615384615384,-0.769230769230768,
-0.753846153846153,-0.738461538461538,-0.723076923076922,-0.707692307692307,
-0.692307692307692,-0.676923076923076,-0.661538461538461,-0.646153846153846,
-0.63076923076923,-0.615384615384615,-0.6,-0.584615384615384,-0.569230769230769,
-0.553846153846154,-0.538461538461538,-0.523076923076923,-0.507692307692308,
-0.492307692307692,-0.476923076923077,-0.461538461538462,-0.446153846153846,
-0.430769230769231,-0.415384615384615,-0.4,-0.384615384615385,-0.369230769230769,
-0.353846153846154,-0.338461538461538,-0.323076923076923,-0.307692307692308,
-0.292307692307692,-0.276923076923077,-0.261538461538462,-0.246153846153846,
-0.230769230769231,-0.215384615384615,-0.2,-0.184615384615385,-0.169230769230769,
-0.153846153846154,-0.138461538461538,-0.123076923076923,-0.107692307692308,
-0.0923076923076923,-0.0769230769230769,-0.0615384615384615,-0.0461538461538462,
-0.0307692307692308,-0.0153846153846154,0.),(-1.,1.),.UNSPECIFIED.)
GEOMETRIC_REPRESENTATION_ITEM()
RATIONAL_B_SPLINE_SURFACE(((1.,1.),(1.,1.),(1.,1.),(1.,1.),(1.,1.),(1.,
1.),(1.,1.),(1.,1.),(1.,1.),(1.,1.),(1.,1.),(1.,1.),(1.,1.),(1.,1.),(1.,
1.),(1.,1.),(1.,1.),(1.,1.),(1.,1.),(1.,1.),(1.,1.),(1.,1.),(1.,1.),(1.,
1.),(1.,1.),(1.,1.),(1.,1.),(1.,1.),(1.,1.),(1.,1.),(1.,1.),(1.,1.),(1.,
1.),(1.,1.),(1.,1.),(1.,1.),(1.,1.),(1.,1.),(1.,1.),(1.,1.),(1.,1.),(1.,
1.),(1.,1.),(1.,1.),(1.,1.),(1.,1.),(1.,1.),(1.,1.),(1.,1.),(1.,1.),(1.,
1.),(1.,1.),(1.,1.),(1.,1.),(1.,1.),(1.,1.),(1.,1.),(1.,1.),(1.,1.),(1.,
1.),(1.,1.),(1.,1.),(1.,1.),(1.,1.),(1.,1.),(1.,1.),(1.,1.),(1.,1.),(1.,
1.),(1.,1.)))
REPRESENTATION_ITEM('')
SURFACE()
);
#128=(
BOUNDED_SURFACE()
B_SPLINE_SURFACE(5,1,((#56980,#56981),(#56982,#56983),(#56984,#56985),(#56986,
#56987),(#56988,#56989),(#56990,#56991),(#56992,#56993),(#56994,#56995),
(#56996,#56997),(#56998,#56999),(#57000,#57001),(#57002,#57003),(#57004,
#57005),(#57006,#57007),(#57008,#57009),(#57010,#57011),(#57012,#57013),
(#57014,#57015),(#57016,#57017),(#57018,#57019),(#57020,#57021),(#57022,
#57023),(#57024,#57025),(#57026,#57027),(#57028,#57029),(#57030,#57031),
(#57032,#57033),(#57034,#57035),(#57036,#57037),(#57038,#57039),(#57040,
#57041),(#57042,#57043),(#57044,#57045),(#57046,#57047),(#57048,#57049),
(#57050,#57051),(#57052,#57053),(#57054,#57055),(#57056,#57057),(#57058,
#57059),(#57060,#57061),(#57062,#57063),(#57064,#57065),(#57066,#57067),
(#57068,#57069),(#57070,#57071),(#57072,#57073),(#57074,#57075),(#57076,
#57077),(#57078,#57079),(#57080,#57081),(#57082,#57083),(#57084,#57085),
(#57086,#57087),(#57088,#57089),(#57090,#57091),(#57092,#57093),(#57094,
#57095),(#57096,#57097),(#57098,#57099),(#57100,#57101),(#57102,#57103),
(#57104,#57105),(#57106,#57107),(#57108,#57109),(#57110,#57111),(#57112,
#57113),(#57114,#57115),(#57116,#57117),(#57118,#57119)),.UNSPECIFIED.,
 .F.,.F.,.F.)
B_SPLINE_SURFACE_WITH_KNOTS((6,1,1,1,1,1,1,1,1,1,1,1,1,1,1,1,1,1,1,1,1,
1,1,1,1,1,1,1,1,1,1,1,1,1,1,1,1,1,1,1,1,1,1,1,1,1,1,1,1,1,1,1,1,1,1,1,1,
1,1,1,1,1,1,1,1,6),(2,2),(-1.,-0.984615384615383,-0.969230769230768,-0.953846153846152,
-0.938461538461537,-0.923076923076922,-0.907692307692306,-0.892307692307691,
-0.876923076923076,-0.86153846153846,-0.846153846153845,-0.83076923076923,
-0.815384615384614,-0.799999999999999,-0.784615384615384,-0.769230769230768,
-0.753846153846153,-0.738461538461538,-0.723076923076922,-0.707692307692307,
-0.692307692307692,-0.676923076923076,-0.661538461538461,-0.646153846153846,
-0.63076923076923,-0.615384615384615,-0.6,-0.584615384615384,-0.569230769230769,
-0.553846153846154,-0.538461538461538,-0.523076923076923,-0.507692307692308,
-0.492307692307692,-0.476923076923077,-0.461538461538462,-0.446153846153846,
-0.430769230769231,-0.415384615384615,-0.4,-0.384615384615385,-0.369230769230769,
-0.353846153846154,-0.338461538461538,-0.323076923076923,-0.307692307692308,
-0.292307692307692,-0.276923076923077,-0.261538461538462,-0.246153846153846,
-0.230769230769231,-0.215384615384615,-0.2,-0.184615384615385,-0.169230769230769,
-0.153846153846154,-0.138461538461538,-0.123076923076923,-0.107692307692308,
-0.0923076923076923,-0.0769230769230769,-0.0615384615384615,-0.0461538461538462,
-0.0307692307692308,-0.0153846153846154,0.),(-1.,1.),.UNSPECIFIED.)
GEOMETRIC_REPRESENTATION_ITEM()
RATIONAL_B_SPLINE_SURFACE(((1.,1.),(1.,1.),(1.,1.),(1.,1.),(1.,1.),(1.,
1.),(1.,1.),(1.,1.),(1.,1.),(1.,1.),(1.,1.),(1.,1.),(1.,1.),(1.,1.),(1.,
1.),(1.,1.),(1.,1.),(1.,1.),(1.,1.),(1.,1.),(1.,1.),(1.,1.),(1.,1.),(1.,
1.),(1.,1.),(1.,1.),(1.,1.),(1.,1.),(1.,1.),(1.,1.),(1.,1.),(1.,1.),(1.,
1.),(1.,1.),(1.,1.),(1.,1.),(1.,1.),(1.,1.),(1.,1.),(1.,1.),(1.,1.),(1.,
1.),(1.,1.),(1.,1.),(1.,1.),(1.,1.),(1.,1.),(1.,1.),(1.,1.),(1.,1.),(1.,
1.),(1.,1.),(1.,1.),(1.,1.),(1.,1.),(1.,1.),(1.,1.),(1.,1.),(1.,1.),(1.,
1.),(1.,1.),(1.,1.),(1.,1.),(1.,1.),(1.,1.),(1.,1.),(1.,1.),(1.,1.),(1.,
1.),(1.,1.)))
REPRESENTATION_ITEM('')
SURFACE()
);
#129=(
BOUNDED_SURFACE()
B_SPLINE_SURFACE(5,1,((#57206,#57207),(#57208,#57209),(#57210,#57211),(#57212,
#57213),(#57214,#57215),(#57216,#57217),(#57218,#57219),(#57220,#57221),
(#57222,#57223),(#57224,#57225),(#57226,#57227),(#57228,#57229),(#57230,
#57231),(#57232,#57233),(#57234,#57235),(#57236,#57237),(#57238,#57239),
(#57240,#57241),(#57242,#57243),(#57244,#57245),(#57246,#57247),(#57248,
#57249),(#57250,#57251),(#57252,#57253),(#57254,#57255),(#57256,#57257),
(#57258,#57259),(#57260,#57261),(#57262,#57263),(#57264,#57265),(#57266,
#57267),(#57268,#57269),(#57270,#57271),(#57272,#57273),(#57274,#57275),
(#57276,#57277),(#57278,#57279),(#57280,#57281),(#57282,#57283),(#57284,
#57285),(#57286,#57287),(#57288,#57289),(#57290,#57291),(#57292,#57293),
(#57294,#57295),(#57296,#57297),(#57298,#57299),(#57300,#57301),(#57302,
#57303),(#57304,#57305),(#57306,#57307),(#57308,#57309),(#57310,#57311),
(#57312,#57313),(#57314,#57315),(#57316,#57317),(#57318,#57319),(#57320,
#57321),(#57322,#57323),(#57324,#57325),(#57326,#57327),(#57328,#57329),
(#57330,#57331),(#57332,#57333),(#57334,#57335),(#57336,#57337),(#57338,
#57339),(#57340,#57341),(#57342,#57343),(#57344,#57345)),.UNSPECIFIED.,
 .F.,.F.,.F.)
B_SPLINE_SURFACE_WITH_KNOTS((6,1,1,1,1,1,1,1,1,1,1,1,1,1,1,1,1,1,1,1,1,
1,1,1,1,1,1,1,1,1,1,1,1,1,1,1,1,1,1,1,1,1,1,1,1,1,1,1,1,1,1,1,1,1,1,1,1,
1,1,1,1,1,1,1,1,6),(2,2),(-1.,-0.984615384615383,-0.969230769230768,-0.953846153846152,
-0.938461538461537,-0.923076923076922,-0.907692307692306,-0.892307692307691,
-0.876923076923076,-0.86153846153846,-0.846153846153845,-0.83076923076923,
-0.815384615384614,-0.799999999999999,-0.784615384615384,-0.769230769230768,
-0.753846153846153,-0.738461538461538,-0.723076923076922,-0.707692307692307,
-0.692307692307692,-0.676923076923076,-0.661538461538461,-0.646153846153846,
-0.63076923076923,-0.615384615384615,-0.6,-0.584615384615384,-0.569230769230769,
-0.553846153846154,-0.538461538461538,-0.523076923076923,-0.507692307692308,
-0.492307692307692,-0.476923076923077,-0.461538461538462,-0.446153846153846,
-0.430769230769231,-0.415384615384615,-0.4,-0.384615384615385,-0.369230769230769,
-0.353846153846154,-0.338461538461538,-0.323076923076923,-0.307692307692308,
-0.292307692307692,-0.276923076923077,-0.261538461538462,-0.246153846153846,
-0.230769230769231,-0.215384615384615,-0.2,-0.184615384615385,-0.169230769230769,
-0.153846153846154,-0.138461538461538,-0.123076923076923,-0.107692307692308,
-0.0923076923076923,-0.0769230769230769,-0.0615384615384615,-0.0461538461538462,
-0.0307692307692308,-0.0153846153846154,0.),(-1.,1.),.UNSPECIFIED.)
GEOMETRIC_REPRESENTATION_ITEM()
RATIONAL_B_SPLINE_SURFACE(((1.,1.),(1.,1.),(1.,1.),(1.,1.),(1.,1.),(1.,
1.),(1.,1.),(1.,1.),(1.,1.),(1.,1.),(1.,1.),(1.,1.),(1.,1.),(1.,1.),(1.,
1.),(1.,1.),(1.,1.),(1.,1.),(1.,1.),(1.,1.),(1.,1.),(1.,1.),(1.,1.),(1.,
1.),(1.,1.),(1.,1.),(1.,1.),(1.,1.),(1.,1.),(1.,1.),(1.,1.),(1.,1.),(1.,
1.),(1.,1.),(1.,1.),(1.,1.),(1.,1.),(1.,1.),(1.,1.),(1.,1.),(1.,1.),(1.,
1.),(1.,1.),(1.,1.),(1.,1.),(1.,1.),(1.,1.),(1.,1.),(1.,1.),(1.,1.),(1.,
1.),(1.,1.),(1.,1.),(1.,1.),(1.,1.),(1.,1.),(1.,1.),(1.,1.),(1.,1.),(1.,
1.),(1.,1.),(1.,1.),(1.,1.),(1.,1.),(1.,1.),(1.,1.),(1.,1.),(1.,1.),(1.,
1.),(1.,1.)))
REPRESENTATION_ITEM('')
SURFACE()
);
#130=(
BOUNDED_SURFACE()
B_SPLINE_SURFACE(5,1,((#57425,#57426),(#57427,#57428),(#57429,#57430),(#57431,
#57432),(#57433,#57434),(#57435,#57436),(#57437,#57438),(#57439,#57440),
(#57441,#57442),(#57443,#57444),(#57445,#57446),(#57447,#57448),(#57449,
#57450),(#57451,#57452),(#57453,#57454),(#57455,#57456),(#57457,#57458),
(#57459,#57460),(#57461,#57462),(#57463,#57464),(#57465,#57466),(#57467,
#57468),(#57469,#57470),(#57471,#57472),(#57473,#57474),(#57475,#57476),
(#57477,#57478),(#57479,#57480),(#57481,#57482),(#57483,#57484),(#57485,
#57486),(#57487,#57488),(#57489,#57490),(#57491,#57492),(#57493,#57494),
(#57495,#57496),(#57497,#57498),(#57499,#57500),(#57501,#57502),(#57503,
#57504),(#57505,#57506),(#57507,#57508),(#57509,#57510),(#57511,#57512),
(#57513,#57514),(#57515,#57516),(#57517,#57518),(#57519,#57520),(#57521,
#57522),(#57523,#57524),(#57525,#57526),(#57527,#57528),(#57529,#57530),
(#57531,#57532),(#57533,#57534),(#57535,#57536),(#57537,#57538),(#57539,
#57540),(#57541,#57542),(#57543,#57544),(#57545,#57546),(#57547,#57548),
(#57549,#57550),(#57551,#57552),(#57553,#57554),(#57555,#57556),(#57557,
#57558),(#57559,#57560),(#57561,#57562),(#57563,#57564)),.UNSPECIFIED.,
 .F.,.F.,.F.)
B_SPLINE_SURFACE_WITH_KNOTS((6,1,1,1,1,1,1,1,1,1,1,1,1,1,1,1,1,1,1,1,1,
1,1,1,1,1,1,1,1,1,1,1,1,1,1,1,1,1,1,1,1,1,1,1,1,1,1,1,1,1,1,1,1,1,1,1,1,
1,1,1,1,1,1,1,1,6),(2,2),(-1.,-0.984615384615383,-0.969230769230768,-0.953846153846152,
-0.938461538461537,-0.923076923076922,-0.907692307692306,-0.892307692307691,
-0.876923076923076,-0.86153846153846,-0.846153846153845,-0.83076923076923,
-0.815384615384614,-0.799999999999999,-0.784615384615384,-0.769230769230768,
-0.753846153846153,-0.738461538461538,-0.723076923076922,-0.707692307692307,
-0.692307692307692,-0.676923076923076,-0.661538461538461,-0.646153846153846,
-0.63076923076923,-0.615384615384615,-0.6,-0.584615384615384,-0.569230769230769,
-0.553846153846154,-0.538461538461538,-0.523076923076923,-0.507692307692308,
-0.492307692307692,-0.476923076923077,-0.461538461538462,-0.446153846153846,
-0.430769230769231,-0.415384615384615,-0.4,-0.384615384615385,-0.369230769230769,
-0.353846153846154,-0.338461538461538,-0.323076923076923,-0.307692307692308,
-0.292307692307692,-0.276923076923077,-0.261538461538462,-0.246153846153846,
-0.230769230769231,-0.215384615384615,-0.2,-0.184615384615385,-0.169230769230769,
-0.153846153846154,-0.138461538461538,-0.123076923076923,-0.107692307692308,
-0.0923076923076923,-0.0769230769230769,-0.0615384615384615,-0.0461538461538462,
-0.0307692307692308,-0.0153846153846154,0.),(-1.,1.),.UNSPECIFIED.)
GEOMETRIC_REPRESENTATION_ITEM()
RATIONAL_B_SPLINE_SURFACE(((1.,1.),(1.,1.),(1.,1.),(1.,1.),(1.,1.),(1.,
1.),(1.,1.),(1.,1.),(1.,1.),(1.,1.),(1.,1.),(1.,1.),(1.,1.),(1.,1.),(1.,
1.),(1.,1.),(1.,1.),(1.,1.),(1.,1.),(1.,1.),(1.,1.),(1.,1.),(1.,1.),(1.,
1.),(1.,1.),(1.,1.),(1.,1.),(1.,1.),(1.,1.),(1.,1.),(1.,1.),(1.,1.),(1.,
1.),(1.,1.),(1.,1.),(1.,1.),(1.,1.),(1.,1.),(1.,1.),(1.,1.),(1.,1.),(1.,
1.),(1.,1.),(1.,1.),(1.,1.),(1.,1.),(1.,1.),(1.,1.),(1.,1.),(1.,1.),(1.,
1.),(1.,1.),(1.,1.),(1.,1.),(1.,1.),(1.,1.),(1.,1.),(1.,1.),(1.,1.),(1.,
1.),(1.,1.),(1.,1.),(1.,1.),(1.,1.),(1.,1.),(1.,1.),(1.,1.),(1.,1.),(1.,
1.),(1.,1.)))
REPRESENTATION_ITEM('')
SURFACE()
);
#211=(
BOUNDED_CURVE()
B_SPLINE_CURVE(5,(#34115,#34116,#34117,#34118,#34119,#34120,#34121,#34122,
#34123,#34124,#34125,#34126,#34127,#34128,#34129,#34130,#34131,#34132,#34133,
#34134,#34135,#34136,#34137,#34138,#34139,#34140,#34141,#34142,#34143,#34144,
#34145,#34146,#34147,#34148,#34149,#34150,#34151,#34152,#34153,#34154,#34155,
#34156,#34157,#34158,#34159,#34160,#34161,#34162,#34163,#34164,#34165,#34166,
#34167,#34168,#34169,#34170,#34171,#34172,#34173,#34174,#34175,#34176,#34177,
#34178,#34179,#34180,#34181,#34182,#34183,#34184),.UNSPECIFIED.,.F.,.F.)
B_SPLINE_CURVE_WITH_KNOTS((6,1,1,1,1,1,1,1,1,1,1,1,1,1,1,1,1,1,1,1,1,1,
1,1,1,1,1,1,1,1,1,1,1,1,1,1,1,1,1,1,1,1,1,1,1,1,1,1,1,1,1,1,1,1,1,1,1,1,
1,1,1,1,1,1,1,6),(0.00577184337450058,0.0153846153846154,0.0307692307692308,
0.0461538461538462,0.0615384615384615,0.0769230769230769,0.0923076923076923,
0.107692307692308,0.123076923076923,0.138461538461538,0.153846153846154,
0.169230769230769,0.184615384615385,0.2,0.215384615384615,0.230769230769231,
0.246153846153846,0.261538461538462,0.276923076923077,0.292307692307692,
0.307692307692308,0.323076923076923,0.338461538461538,0.353846153846154,
0.369230769230769,0.384615384615385,0.4,0.415384615384615,0.430769230769231,
0.446153846153846,0.461538461538462,0.476923076923077,0.492307692307692,
0.507692307692308,0.523076923076923,0.538461538461538,0.553846153846154,
0.569230769230769,0.584615384615384,0.6,0.615384615384615,0.63076923076923,
0.646153846153846,0.661538461538461,0.676923076923076,0.692307692307692,
0.707692307692307,0.723076923076922,0.738461538461538,0.753846153846153,
0.769230769230768,0.784615384615384,0.799999999999999,0.815384615384614,
0.83076923076923,0.846153846153845,0.86153846153846,0.876923076923076,0.892307692307691,
0.907692307692306,0.923076923076922,0.938461538461537,0.953846153846152,
0.969230769230768,0.984615384615383,1.),.UNSPECIFIED.)
CURVE()
GEOMETRIC_REPRESENTATION_ITEM()
RATIONAL_B_SPLINE_CURVE((1.,1.,1.,1.,1.,1.,1.,1.,1.,1.,1.,1.,1.,1.,1.,1.,
1.,1.,1.,1.,1.,1.,1.,1.,1.,1.,1.,1.,1.,1.,1.,1.,1.,1.,1.,1.,1.,1.,1.,1.,
1.,1.,1.,1.,1.,1.,1.,1.,1.,1.,1.,1.,1.,1.,1.,1.,1.,1.,1.,1.,1.,1.,1.,1.,
1.,1.,1.,1.,1.,1.))
REPRESENTATION_ITEM('')
);
#212=(
BOUNDED_CURVE()
B_SPLINE_CURVE(5,(#34188,#34189,#34190,#34191,#34192,#34193,#34194,#34195,
#34196,#34197,#34198,#34199,#34200,#34201,#34202,#34203,#34204,#34205,#34206,
#34207,#34208,#34209,#34210,#34211,#34212,#34213,#34214,#34215,#34216,#34217,
#34218,#34219,#34220,#34221,#34222,#34223,#34224,#34225,#34226,#34227,#34228,
#34229,#34230,#34231,#34232,#34233,#34234,#34235,#34236,#34237,#34238,#34239,
#34240,#34241,#34242,#34243,#34244,#34245,#34246,#34247,#34248,#34249,#34250,
#34251,#34252,#34253,#34254,#34255,#34256,#34257),.UNSPECIFIED.,.F.,.F.)
B_SPLINE_CURVE_WITH_KNOTS((6,1,1,1,1,1,1,1,1,1,1,1,1,1,1,1,1,1,1,1,1,1,
1,1,1,1,1,1,1,1,1,1,1,1,1,1,1,1,1,1,1,1,1,1,1,1,1,1,1,1,1,1,1,1,1,1,1,1,
1,1,1,1,1,1,1,6),(0.,0.0153846153846154,0.0307692307692308,0.0461538461538462,
0.0615384615384615,0.0769230769230769,0.0923076923076923,0.107692307692308,
0.123076923076923,0.138461538461538,0.153846153846154,0.169230769230769,
0.184615384615385,0.2,0.215384615384615,0.230769230769231,0.246153846153846,
0.261538461538462,0.276923076923077,0.292307692307692,0.307692307692308,
0.323076923076923,0.338461538461538,0.353846153846154,0.369230769230769,
0.384615384615385,0.4,0.415384615384615,0.430769230769231,0.446153846153846,
0.461538461538462,0.476923076923077,0.492307692307692,0.507692307692308,
0.523076923076923,0.538461538461538,0.553846153846154,0.569230769230769,
0.584615384615384,0.6,0.615384615384615,0.63076923076923,0.646153846153846,
0.661538461538461,0.676923076923076,0.692307692307692,0.707692307692307,
0.723076923076922,0.738461538461538,0.753846153846153,0.769230769230768,
0.784615384615384,0.799999999999999,0.815384615384614,0.83076923076923,
0.846153846153845,0.86153846153846,0.876923076923076,0.892307692307691,
0.907692307692306,0.923076923076922,0.938461538461537,0.953846153846152,
0.969230769230768,0.984615384615383,0.994228156739708),.UNSPECIFIED.)
CURVE()
GEOMETRIC_REPRESENTATION_ITEM()
RATIONAL_B_SPLINE_CURVE((1.,1.,1.,1.,1.,1.,1.,1.,1.,1.,1.,1.,1.,1.,1.,1.,
1.,1.,1.,1.,1.,1.,1.,1.,1.,1.,1.,1.,1.,1.,1.,1.,1.,1.,1.,1.,1.,1.,1.,1.,
1.,1.,1.,1.,1.,1.,1.,1.,1.,1.,1.,1.,1.,1.,1.,1.,1.,1.,1.,1.,1.,1.,1.,1.,
1.,1.,1.,1.,1.,1.))
REPRESENTATION_ITEM('')
);
#213=(
BOUNDED_CURVE()
B_SPLINE_CURVE(5,(#34261,#34262,#34263,#34264,#34265,#34266,#34267,#34268,
#34269,#34270,#34271,#34272,#34273,#34274,#34275,#34276,#34277,#34278,#34279,
#34280,#34281,#34282,#34283,#34284,#34285,#34286,#34287,#34288,#34289,#34290,
#34291,#34292,#34293,#34294,#34295,#34296,#34297,#34298,#34299,#34300,#34301,
#34302,#34303,#34304,#34305,#34306,#34307,#34308,#34309,#34310,#34311,#34312,
#34313,#34314,#34315,#34316,#34317,#34318,#34319,#34320,#34321,#34322,#34323,
#34324,#34325,#34326,#34327,#34328,#34329,#34330),.UNSPECIFIED.,.F.,.F.)
B_SPLINE_CURVE_WITH_KNOTS((6,1,1,1,1,1,1,1,1,1,1,1,1,1,1,1,1,1,1,1,1,1,
1,1,1,1,1,1,1,1,1,1,1,1,1,1,1,1,1,1,1,1,1,1,1,1,1,1,1,1,1,1,1,1,1,1,1,1,
1,1,1,1,1,1,1,6),(0.0057718433745091,0.0153846153846154,0.0307692307692308,
0.0461538461538462,0.0615384615384615,0.0769230769230769,0.0923076923076923,
0.107692307692308,0.123076923076923,0.138461538461538,0.153846153846154,
0.169230769230769,0.184615384615385,0.2,0.215384615384615,0.230769230769231,
0.246153846153846,0.261538461538462,0.276923076923077,0.292307692307692,
0.307692307692308,0.323076923076923,0.338461538461538,0.353846153846154,
0.369230769230769,0.384615384615385,0.4,0.415384615384615,0.430769230769231,
0.446153846153846,0.461538461538462,0.476923076923077,0.492307692307692,
0.507692307692308,0.523076923076923,0.538461538461538,0.553846153846154,
0.569230769230769,0.584615384615384,0.6,0.615384615384615,0.63076923076923,
0.646153846153846,0.661538461538461,0.676923076923076,0.692307692307692,
0.707692307692307,0.723076923076922,0.738461538461538,0.753846153846153,
0.769230769230768,0.784615384615384,0.799999999999999,0.815384615384614,
0.83076923076923,0.846153846153845,0.86153846153846,0.876923076923076,0.892307692307691,
0.907692307692306,0.923076923076922,0.938461538461537,0.953846153846152,
0.969230769230768,0.984615384615383,1.),.UNSPECIFIED.)
CURVE()
GEOMETRIC_REPRESENTATION_ITEM()
RATIONAL_B_SPLINE_CURVE((1.,1.,1.,1.,1.,1.,1.,1.,1.,1.,1.,1.,1.,1.,1.,1.,
1.,1.,1.,1.,1.,1.,1.,1.,1.,1.,1.,1.,1.,1.,1.,1.,1.,1.,1.,1.,1.,1.,1.,1.,
1.,1.,1.,1.,1.,1.,1.,1.,1.,1.,1.,1.,1.,1.,1.,1.,1.,1.,1.,1.,1.,1.,1.,1.,
1.,1.,1.,1.,1.,1.))
REPRESENTATION_ITEM('')
);
#214=(
BOUNDED_CURVE()
B_SPLINE_CURVE(5,(#34334,#34335,#34336,#34337,#34338,#34339,#34340,#34341,
#34342,#34343,#34344,#34345,#34346,#34347,#34348,#34349,#34350,#34351,#34352,
#34353,#34354,#34355,#34356,#34357,#34358,#34359,#34360,#34361,#34362,#34363,
#34364,#34365,#34366,#34367,#34368,#34369,#34370,#34371,#34372,#34373,#34374,
#34375,#34376,#34377,#34378,#34379,#34380,#34381,#34382,#34383,#34384,#34385,
#34386,#34387,#34388,#34389,#34390,#34391,#34392,#34393,#34394,#34395,#34396,
#34397,#34398,#34399,#34400,#34401,#34402,#34403),.UNSPECIFIED.,.F.,.F.)
B_SPLINE_CURVE_WITH_KNOTS((6,1,1,1,1,1,1,1,1,1,1,1,1,1,1,1,1,1,1,1,1,1,
1,1,1,1,1,1,1,1,1,1,1,1,1,1,1,1,1,1,1,1,1,1,1,1,1,1,1,1,1,1,1,1,1,1,1,1,
1,1,1,1,1,1,1,6),(0.,0.0153846153846154,0.0307692307692308,0.0461538461538462,
0.0615384615384615,0.0769230769230769,0.0923076923076923,0.107692307692308,
0.123076923076923,0.138461538461538,0.153846153846154,0.169230769230769,
0.184615384615385,0.2,0.215384615384615,0.230769230769231,0.246153846153846,
0.261538461538462,0.276923076923077,0.292307692307692,0.307692307692308,
0.323076923076923,0.338461538461538,0.353846153846154,0.369230769230769,
0.384615384615385,0.4,0.415384615384615,0.430769230769231,0.446153846153846,
0.461538461538462,0.476923076923077,0.492307692307692,0.507692307692308,
0.523076923076923,0.538461538461538,0.553846153846154,0.569230769230769,
0.584615384615384,0.6,0.615384615384615,0.63076923076923,0.646153846153846,
0.661538461538461,0.676923076923076,0.692307692307692,0.707692307692307,
0.723076923076922,0.738461538461538,0.753846153846153,0.769230769230768,
0.784615384615384,0.799999999999999,0.815384615384614,0.83076923076923,
0.846153846153845,0.86153846153846,0.876923076923076,0.892307692307691,
0.907692307692306,0.923076923076922,0.938461538461537,0.953846153846152,
0.969230769230768,0.984615384615383,0.994228156739689),.UNSPECIFIED.)
CURVE()
GEOMETRIC_REPRESENTATION_ITEM()
RATIONAL_B_SPLINE_CURVE((1.,1.,1.,1.,1.,1.,1.,1.,1.,1.,1.,1.,1.,1.,1.,1.,
1.,1.,1.,1.,1.,1.,1.,1.,1.,1.,1.,1.,1.,1.,1.,1.,1.,1.,1.,1.,1.,1.,1.,1.,
1.,1.,1.,1.,1.,1.,1.,1.,1.,1.,1.,1.,1.,1.,1.,1.,1.,1.,1.,1.,1.,1.,1.,1.,
1.,1.,1.,1.,1.,1.))
REPRESENTATION_ITEM('')
);
#215=(
BOUNDED_CURVE()
B_SPLINE_CURVE(5,(#34407,#34408,#34409,#34410,#34411,#34412,#34413,#34414,
#34415,#34416,#34417,#34418,#34419,#34420,#34421,#34422,#34423,#34424,#34425,
#34426,#34427,#34428,#34429,#34430,#34431,#34432,#34433,#34434,#34435,#34436,
#34437,#34438,#34439,#34440,#34441,#34442,#34443,#34444,#34445,#34446,#34447,
#34448,#34449,#34450,#34451,#34452,#34453,#34454,#34455,#34456,#34457,#34458,
#34459,#34460,#34461,#34462,#34463,#34464,#34465,#34466,#34467,#34468,#34469,
#34470,#34471,#34472,#34473,#34474,#34475,#34476),.UNSPECIFIED.,.F.,.F.)
B_SPLINE_CURVE_WITH_KNOTS((6,1,1,1,1,1,1,1,1,1,1,1,1,1,1,1,1,1,1,1,1,1,
1,1,1,1,1,1,1,1,1,1,1,1,1,1,1,1,1,1,1,1,1,1,1,1,1,1,1,1,1,1,1,1,1,1,1,1,
1,1,1,1,1,1,1,6),(0.00577184337448946,0.0153846153846154,0.0307692307692308,
0.0461538461538462,0.0615384615384615,0.0769230769230769,0.0923076923076923,
0.107692307692308,0.123076923076923,0.138461538461538,0.153846153846154,
0.169230769230769,0.184615384615385,0.2,0.215384615384615,0.230769230769231,
0.246153846153846,0.261538461538462,0.276923076923077,0.292307692307692,
0.307692307692308,0.323076923076923,0.338461538461538,0.353846153846154,
0.369230769230769,0.384615384615385,0.4,0.415384615384615,0.430769230769231,
0.446153846153846,0.461538461538462,0.476923076923077,0.492307692307692,
0.507692307692308,0.523076923076923,0.538461538461538,0.553846153846154,
0.569230769230769,0.584615384615384,0.6,0.615384615384615,0.63076923076923,
0.646153846153846,0.661538461538461,0.676923076923076,0.692307692307692,
0.707692307692307,0.723076923076922,0.738461538461538,0.753846153846153,
0.769230769230768,0.784615384615384,0.799999999999999,0.815384615384614,
0.83076923076923,0.846153846153845,0.86153846153846,0.876923076923076,0.892307692307691,
0.907692307692306,0.923076923076922,0.938461538461537,0.953846153846152,
0.969230769230768,0.984615384615383,1.),.UNSPECIFIED.)
CURVE()
GEOMETRIC_REPRESENTATION_ITEM()
RATIONAL_B_SPLINE_CURVE((1.,1.,1.,1.,1.,1.,1.,1.,1.,1.,1.,1.,1.,1.,1.,1.,
1.,1.,1.,1.,1.,1.,1.,1.,1.,1.,1.,1.,1.,1.,1.,1.,1.,1.,1.,1.,1.,1.,1.,1.,
1.,1.,1.,1.,1.,1.,1.,1.,1.,1.,1.,1.,1.,1.,1.,1.,1.,1.,1.,1.,1.,1.,1.,1.,
1.,1.,1.,1.,1.,1.))
REPRESENTATION_ITEM('')
);
#216=(
BOUNDED_CURVE()
B_SPLINE_CURVE(5,(#34480,#34481,#34482,#34483,#34484,#34485,#34486,#34487,
#34488,#34489,#34490,#34491,#34492,#34493,#34494,#34495,#34496,#34497,#34498,
#34499,#34500,#34501,#34502,#34503,#34504,#34505,#34506,#34507,#34508,#34509,
#34510,#34511,#34512,#34513,#34514,#34515,#34516,#34517,#34518,#34519,#34520,
#34521,#34522,#34523,#34524,#34525,#34526,#34527,#34528,#34529,#34530,#34531,
#34532,#34533,#34534,#34535,#34536,#34537,#34538,#34539,#34540,#34541,#34542,
#34543,#34544,#34545,#34546,#34547,#34548,#34549),.UNSPECIFIED.,.F.,.F.)
B_SPLINE_CURVE_WITH_KNOTS((6,1,1,1,1,1,1,1,1,1,1,1,1,1,1,1,1,1,1,1,1,1,
1,1,1,1,1,1,1,1,1,1,1,1,1,1,1,1,1,1,1,1,1,1,1,1,1,1,1,1,1,1,1,1,1,1,1,1,
1,1,1,1,1,1,1,6),(0.,0.0153846153846154,0.0307692307692308,0.0461538461538462,
0.0615384615384615,0.0769230769230769,0.0923076923076923,0.107692307692308,
0.123076923076923,0.138461538461538,0.153846153846154,0.169230769230769,
0.184615384615385,0.2,0.215384615384615,0.230769230769231,0.246153846153846,
0.261538461538462,0.276923076923077,0.292307692307692,0.307692307692308,
0.323076923076923,0.338461538461538,0.353846153846154,0.369230769230769,
0.384615384615385,0.4,0.415384615384615,0.430769230769231,0.446153846153846,
0.461538461538462,0.476923076923077,0.492307692307692,0.507692307692308,
0.523076923076923,0.538461538461538,0.553846153846154,0.569230769230769,
0.584615384615384,0.6,0.615384615384615,0.63076923076923,0.646153846153846,
0.661538461538461,0.676923076923076,0.692307692307692,0.707692307692307,
0.723076923076922,0.738461538461538,0.753846153846153,0.769230769230768,
0.784615384615384,0.799999999999999,0.815384615384614,0.83076923076923,
0.846153846153845,0.86153846153846,0.876923076923076,0.892307692307691,
0.907692307692306,0.923076923076922,0.938461538461537,0.953846153846152,
0.969230769230768,0.984615384615383,0.994228156739718),.UNSPECIFIED.)
CURVE()
GEOMETRIC_REPRESENTATION_ITEM()
RATIONAL_B_SPLINE_CURVE((1.,1.,1.,1.,1.,1.,1.,1.,1.,1.,1.,1.,1.,1.,1.,1.,
1.,1.,1.,1.,1.,1.,1.,1.,1.,1.,1.,1.,1.,1.,1.,1.,1.,1.,1.,1.,1.,1.,1.,1.,
1.,1.,1.,1.,1.,1.,1.,1.,1.,1.,1.,1.,1.,1.,1.,1.,1.,1.,1.,1.,1.,1.,1.,1.,
1.,1.,1.,1.,1.,1.))
REPRESENTATION_ITEM('')
);
#217=(
BOUNDED_CURVE()
B_SPLINE_CURVE(5,(#34553,#34554,#34555,#34556,#34557,#34558,#34559,#34560,
#34561,#34562,#34563,#34564,#34565,#34566,#34567,#34568,#34569,#34570,#34571,
#34572,#34573,#34574,#34575,#34576,#34577,#34578,#34579,#34580,#34581,#34582,
#34583,#34584,#34585,#34586,#34587,#34588,#34589,#34590,#34591,#34592,#34593,
#34594,#34595,#34596,#34597,#34598,#34599,#34600,#34601,#34602,#34603,#34604,
#34605,#34606,#34607,#34608,#34609,#34610,#34611,#34612,#34613,#34614,#34615,
#34616,#34617,#34618,#34619,#34620,#34621,#34622),.UNSPECIFIED.,.F.,.F.)
B_SPLINE_CURVE_WITH_KNOTS((6,1,1,1,1,1,1,1,1,1,1,1,1,1,1,1,1,1,1,1,1,1,
1,1,1,1,1,1,1,1,1,1,1,1,1,1,1,1,1,1,1,1,1,1,1,1,1,1,1,1,1,1,1,1,1,1,1,1,
1,1,1,1,1,1,1,6),(0.00577184337450897,0.0153846153846154,0.0307692307692308,
0.0461538461538462,0.0615384615384615,0.0769230769230769,0.0923076923076923,
0.107692307692308,0.123076923076923,0.138461538461538,0.153846153846154,
0.169230769230769,0.184615384615385,0.2,0.215384615384615,0.230769230769231,
0.246153846153846,0.261538461538462,0.276923076923077,0.292307692307692,
0.307692307692308,0.323076923076923,0.338461538461538,0.353846153846154,
0.369230769230769,0.384615384615385,0.4,0.415384615384615,0.430769230769231,
0.446153846153846,0.461538461538462,0.476923076923077,0.492307692307692,
0.507692307692308,0.523076923076923,0.538461538461538,0.553846153846154,
0.569230769230769,0.584615384615384,0.6,0.615384615384615,0.63076923076923,
0.646153846153846,0.661538461538461,0.676923076923076,0.692307692307692,
0.707692307692307,0.723076923076922,0.738461538461538,0.753846153846153,
0.769230769230768,0.784615384615384,0.799999999999999,0.815384615384614,
0.83076923076923,0.846153846153845,0.86153846153846,0.876923076923076,0.892307692307691,
0.907692307692306,0.923076923076922,0.938461538461537,0.953846153846152,
0.969230769230768,0.984615384615383,1.),.UNSPECIFIED.)
CURVE()
GEOMETRIC_REPRESENTATION_ITEM()
RATIONAL_B_SPLINE_CURVE((1.,1.,1.,1.,1.,1.,1.,1.,1.,1.,1.,1.,1.,1.,1.,1.,
1.,1.,1.,1.,1.,1.,1.,1.,1.,1.,1.,1.,1.,1.,1.,1.,1.,1.,1.,1.,1.,1.,1.,1.,
1.,1.,1.,1.,1.,1.,1.,1.,1.,1.,1.,1.,1.,1.,1.,1.,1.,1.,1.,1.,1.,1.,1.,1.,
1.,1.,1.,1.,1.,1.))
REPRESENTATION_ITEM('')
);
#218=(
BOUNDED_CURVE()
B_SPLINE_CURVE(5,(#34626,#34627,#34628,#34629,#34630,#34631,#34632,#34633,
#34634,#34635,#34636,#34637,#34638,#34639,#34640,#34641,#34642,#34643,#34644,
#34645,#34646,#34647,#34648,#34649,#34650,#34651,#34652,#34653,#34654,#34655,
#34656,#34657,#34658,#34659,#34660,#34661,#34662,#34663,#34664,#34665,#34666,
#34667,#34668,#34669,#34670,#34671,#34672,#34673,#34674,#34675,#34676,#34677,
#34678,#34679,#34680,#34681,#34682,#34683,#34684,#34685,#34686,#34687,#34688,
#34689,#34690,#34691,#34692,#34693,#34694,#34695),.UNSPECIFIED.,.F.,.F.)
B_SPLINE_CURVE_WITH_KNOTS((6,1,1,1,1,1,1,1,1,1,1,1,1,1,1,1,1,1,1,1,1,1,
1,1,1,1,1,1,1,1,1,1,1,1,1,1,1,1,1,1,1,1,1,1,1,1,1,1,1,1,1,1,1,1,1,1,1,1,
1,1,1,1,1,1,1,6),(0.,0.0153846153846154,0.0307692307692308,0.0461538461538462,
0.0615384615384615,0.0769230769230769,0.0923076923076923,0.107692307692308,
0.123076923076923,0.138461538461538,0.153846153846154,0.169230769230769,
0.184615384615385,0.2,0.215384615384615,0.230769230769231,0.246153846153846,
0.261538461538462,0.276923076923077,0.292307692307692,0.307692307692308,
0.323076923076923,0.338461538461538,0.353846153846154,0.369230769230769,
0.384615384615385,0.4,0.415384615384615,0.430769230769231,0.446153846153846,
0.461538461538462,0.476923076923077,0.492307692307692,0.507692307692308,
0.523076923076923,0.538461538461538,0.553846153846154,0.569230769230769,
0.584615384615384,0.6,0.615384615384615,0.63076923076923,0.646153846153846,
0.661538461538461,0.676923076923076,0.692307692307692,0.707692307692307,
0.723076923076922,0.738461538461538,0.753846153846153,0.769230769230768,
0.784615384615384,0.799999999999999,0.815384615384614,0.83076923076923,
0.846153846153845,0.86153846153846,0.876923076923076,0.892307692307691,
0.907692307692306,0.923076923076922,0.938461538461537,0.953846153846152,
0.969230769230768,0.984615384615383,0.994228156739701),.UNSPECIFIED.)
CURVE()
GEOMETRIC_REPRESENTATION_ITEM()
RATIONAL_B_SPLINE_CURVE((1.,1.,1.,1.,1.,1.,1.,1.,1.,1.,1.,1.,1.,1.,1.,1.,
1.,1.,1.,1.,1.,1.,1.,1.,1.,1.,1.,1.,1.,1.,1.,1.,1.,1.,1.,1.,1.,1.,1.,1.,
1.,1.,1.,1.,1.,1.,1.,1.,1.,1.,1.,1.,1.,1.,1.,1.,1.,1.,1.,1.,1.,1.,1.,1.,
1.,1.,1.,1.,1.,1.))
REPRESENTATION_ITEM('')
);
#219=(
BOUNDED_CURVE()
B_SPLINE_CURVE(5,(#34699,#34700,#34701,#34702,#34703,#34704,#34705,#34706,
#34707,#34708,#34709,#34710,#34711,#34712,#34713,#34714,#34715,#34716,#34717,
#34718,#34719,#34720,#34721,#34722,#34723,#34724,#34725,#34726,#34727,#34728,
#34729,#34730,#34731,#34732,#34733,#34734,#34735,#34736,#34737,#34738,#34739,
#34740,#34741,#34742,#34743,#34744,#34745,#34746,#34747,#34748,#34749,#34750,
#34751,#34752,#34753,#34754,#34755,#34756,#34757,#34758,#34759,#34760,#34761,
#34762,#34763,#34764,#34765,#34766,#34767,#34768),.UNSPECIFIED.,.F.,.F.)
B_SPLINE_CURVE_WITH_KNOTS((6,1,1,1,1,1,1,1,1,1,1,1,1,1,1,1,1,1,1,1,1,1,
1,1,1,1,1,1,1,1,1,1,1,1,1,1,1,1,1,1,1,1,1,1,1,1,1,1,1,1,1,1,1,1,1,1,1,1,
1,1,1,1,1,1,1,6),(0.00577184337451001,0.0153846153846154,0.0307692307692308,
0.0461538461538462,0.0615384615384615,0.0769230769230769,0.0923076923076923,
0.107692307692308,0.123076923076923,0.138461538461538,0.153846153846154,
0.169230769230769,0.184615384615385,0.2,0.215384615384615,0.230769230769231,
0.246153846153846,0.261538461538462,0.276923076923077,0.292307692307692,
0.307692307692308,0.323076923076923,0.338461538461538,0.353846153846154,
0.369230769230769,0.384615384615385,0.4,0.415384615384615,0.430769230769231,
0.446153846153846,0.461538461538462,0.476923076923077,0.492307692307692,
0.507692307692308,0.523076923076923,0.538461538461538,0.553846153846154,
0.569230769230769,0.584615384615384,0.6,0.615384615384615,0.63076923076923,
0.646153846153846,0.661538461538461,0.676923076923076,0.692307692307692,
0.707692307692307,0.723076923076922,0.738461538461538,0.753846153846153,
0.769230769230768,0.784615384615384,0.799999999999999,0.815384615384614,
0.83076923076923,0.846153846153845,0.86153846153846,0.876923076923076,0.892307692307691,
0.907692307692306,0.923076923076922,0.938461538461537,0.953846153846152,
0.969230769230768,0.984615384615383,1.),.UNSPECIFIED.)
CURVE()
GEOMETRIC_REPRESENTATION_ITEM()
RATIONAL_B_SPLINE_CURVE((1.,1.,1.,1.,1.,1.,1.,1.,1.,1.,1.,1.,1.,1.,1.,1.,
1.,1.,1.,1.,1.,1.,1.,1.,1.,1.,1.,1.,1.,1.,1.,1.,1.,1.,1.,1.,1.,1.,1.,1.,
1.,1.,1.,1.,1.,1.,1.,1.,1.,1.,1.,1.,1.,1.,1.,1.,1.,1.,1.,1.,1.,1.,1.,1.,
1.,1.,1.,1.,1.,1.))
REPRESENTATION_ITEM('')
);
#220=(
BOUNDED_CURVE()
B_SPLINE_CURVE(5,(#34772,#34773,#34774,#34775,#34776,#34777,#34778,#34779,
#34780,#34781,#34782,#34783,#34784,#34785,#34786,#34787,#34788,#34789,#34790,
#34791,#34792,#34793,#34794,#34795,#34796,#34797,#34798,#34799,#34800,#34801,
#34802,#34803,#34804,#34805,#34806,#34807,#34808,#34809,#34810,#34811,#34812,
#34813,#34814,#34815,#34816,#34817,#34818,#34819,#34820,#34821,#34822,#34823,
#34824,#34825,#34826,#34827,#34828,#34829,#34830,#34831,#34832,#34833,#34834,
#34835,#34836,#34837,#34838,#34839,#34840,#34841),.UNSPECIFIED.,.F.,.F.)
B_SPLINE_CURVE_WITH_KNOTS((6,1,1,1,1,1,1,1,1,1,1,1,1,1,1,1,1,1,1,1,1,1,
1,1,1,1,1,1,1,1,1,1,1,1,1,1,1,1,1,1,1,1,1,1,1,1,1,1,1,1,1,1,1,1,1,1,1,1,
1,1,1,1,1,1,1,6),(0.,0.0153846153846154,0.0307692307692308,0.0461538461538462,
0.0615384615384615,0.0769230769230769,0.0923076923076923,0.107692307692308,
0.123076923076923,0.138461538461538,0.153846153846154,0.169230769230769,
0.184615384615385,0.2,0.215384615384615,0.230769230769231,0.246153846153846,
0.261538461538462,0.276923076923077,0.292307692307692,0.307692307692308,
0.323076923076923,0.338461538461538,0.353846153846154,0.369230769230769,
0.384615384615385,0.4,0.415384615384615,0.430769230769231,0.446153846153846,
0.461538461538462,0.476923076923077,0.492307692307692,0.507692307692308,
0.523076923076923,0.538461538461538,0.553846153846154,0.569230769230769,
0.584615384615384,0.6,0.615384615384615,0.63076923076923,0.646153846153846,
0.661538461538461,0.676923076923076,0.692307692307692,0.707692307692307,
0.723076923076922,0.738461538461538,0.753846153846153,0.769230769230768,
0.784615384615384,0.799999999999999,0.815384615384614,0.83076923076923,
0.846153846153845,0.86153846153846,0.876923076923076,0.892307692307691,
0.907692307692306,0.923076923076922,0.938461538461537,0.953846153846152,
0.969230769230768,0.984615384615383,0.994228156739697),.UNSPECIFIED.)
CURVE()
GEOMETRIC_REPRESENTATION_ITEM()
RATIONAL_B_SPLINE_CURVE((1.,1.,1.,1.,1.,1.,1.,1.,1.,1.,1.,1.,1.,1.,1.,1.,
1.,1.,1.,1.,1.,1.,1.,1.,1.,1.,1.,1.,1.,1.,1.,1.,1.,1.,1.,1.,1.,1.,1.,1.,
1.,1.,1.,1.,1.,1.,1.,1.,1.,1.,1.,1.,1.,1.,1.,1.,1.,1.,1.,1.,1.,1.,1.,1.,
1.,1.,1.,1.,1.,1.))
REPRESENTATION_ITEM('')
);
#221=(
BOUNDED_CURVE()
B_SPLINE_CURVE(5,(#34845,#34846,#34847,#34848,#34849,#34850,#34851,#34852,
#34853,#34854,#34855,#34856,#34857,#34858,#34859,#34860,#34861,#34862,#34863,
#34864,#34865,#34866,#34867,#34868,#34869,#34870,#34871,#34872,#34873,#34874,
#34875,#34876,#34877,#34878,#34879,#34880,#34881,#34882,#34883,#34884,#34885,
#34886,#34887,#34888,#34889,#34890,#34891,#34892,#34893,#34894,#34895,#34896,
#34897,#34898,#34899,#34900,#34901,#34902,#34903,#34904,#34905,#34906,#34907,
#34908,#34909,#34910,#34911,#34912,#34913,#34914),.UNSPECIFIED.,.F.,.F.)
B_SPLINE_CURVE_WITH_KNOTS((6,1,1,1,1,1,1,1,1,1,1,1,1,1,1,1,1,1,1,1,1,1,
1,1,1,1,1,1,1,1,1,1,1,1,1,1,1,1,1,1,1,1,1,1,1,1,1,1,1,1,1,1,1,1,1,1,1,1,
1,1,1,1,1,1,1,6),(0.00577184337452306,0.0153846153846154,0.0307692307692308,
0.0461538461538462,0.0615384615384615,0.0769230769230769,0.0923076923076923,
0.107692307692308,0.123076923076923,0.138461538461538,0.153846153846154,
0.169230769230769,0.184615384615385,0.2,0.215384615384615,0.230769230769231,
0.246153846153846,0.261538461538462,0.276923076923077,0.292307692307692,
0.307692307692308,0.323076923076923,0.338461538461538,0.353846153846154,
0.369230769230769,0.384615384615385,0.4,0.415384615384615,0.430769230769231,
0.446153846153846,0.461538461538462,0.476923076923077,0.492307692307692,
0.507692307692308,0.523076923076923,0.538461538461538,0.553846153846154,
0.569230769230769,0.584615384615384,0.6,0.615384615384615,0.63076923076923,
0.646153846153846,0.661538461538461,0.676923076923076,0.692307692307692,
0.707692307692307,0.723076923076922,0.738461538461538,0.753846153846153,
0.769230769230768,0.784615384615384,0.799999999999999,0.815384615384614,
0.83076923076923,0.846153846153845,0.86153846153846,0.876923076923076,0.892307692307691,
0.907692307692306,0.923076923076922,0.938461538461537,0.953846153846152,
0.969230769230768,0.984615384615383,1.),.UNSPECIFIED.)
CURVE()
GEOMETRIC_REPRESENTATION_ITEM()
RATIONAL_B_SPLINE_CURVE((1.,1.,1.,1.,1.,1.,1.,1.,1.,1.,1.,1.,1.,1.,1.,1.,
1.,1.,1.,1.,1.,1.,1.,1.,1.,1.,1.,1.,1.,1.,1.,1.,1.,1.,1.,1.,1.,1.,1.,1.,
1.,1.,1.,1.,1.,1.,1.,1.,1.,1.,1.,1.,1.,1.,1.,1.,1.,1.,1.,1.,1.,1.,1.,1.,
1.,1.,1.,1.,1.,1.))
REPRESENTATION_ITEM('')
);
#222=(
BOUNDED_CURVE()
B_SPLINE_CURVE(5,(#34918,#34919,#34920,#34921,#34922,#34923,#34924,#34925,
#34926,#34927,#34928,#34929,#34930,#34931,#34932,#34933,#34934,#34935,#34936,
#34937,#34938,#34939,#34940,#34941,#34942,#34943,#34944,#34945,#34946,#34947,
#34948,#34949,#34950,#34951,#34952,#34953,#34954,#34955,#34956,#34957,#34958,
#34959,#34960,#34961,#34962,#34963,#34964,#34965,#34966,#34967,#34968,#34969,
#34970,#34971,#34972,#34973,#34974,#34975,#34976,#34977,#34978,#34979,#34980,
#34981,#34982,#34983,#34984,#34985,#34986,#34987),.UNSPECIFIED.,.F.,.F.)
B_SPLINE_CURVE_WITH_KNOTS((6,1,1,1,1,1,1,1,1,1,1,1,1,1,1,1,1,1,1,1,1,1,
1,1,1,1,1,1,1,1,1,1,1,1,1,1,1,1,1,1,1,1,1,1,1,1,1,1,1,1,1,1,1,1,1,1,1,1,
1,1,1,1,1,1,1,6),(0.,0.0153846153846154,0.0307692307692308,0.0461538461538462,
0.0615384615384615,0.0769230769230769,0.0923076923076923,0.107692307692308,
0.123076923076923,0.138461538461538,0.153846153846154,0.169230769230769,
0.184615384615385,0.2,0.215384615384615,0.230769230769231,0.246153846153846,
0.261538461538462,0.276923076923077,0.292307692307692,0.307692307692308,
0.323076923076923,0.338461538461538,0.353846153846154,0.369230769230769,
0.384615384615385,0.4,0.415384615384615,0.430769230769231,0.446153846153846,
0.461538461538462,0.476923076923077,0.492307692307692,0.507692307692308,
0.523076923076923,0.538461538461538,0.553846153846154,0.569230769230769,
0.584615384615384,0.6,0.615384615384615,0.63076923076923,0.646153846153846,
0.661538461538461,0.676923076923076,0.692307692307692,0.707692307692307,
0.723076923076922,0.738461538461538,0.753846153846153,0.769230769230768,
0.784615384615384,0.799999999999999,0.815384615384614,0.83076923076923,
0.846153846153845,0.86153846153846,0.876923076923076,0.892307692307691,
0.907692307692306,0.923076923076922,0.938461538461537,0.953846153846152,
0.969230769230768,0.984615384615383,0.994228156739688),.UNSPECIFIED.)
CURVE()
GEOMETRIC_REPRESENTATION_ITEM()
RATIONAL_B_SPLINE_CURVE((1.,1.,1.,1.,1.,1.,1.,1.,1.,1.,1.,1.,1.,1.,1.,1.,
1.,1.,1.,1.,1.,1.,1.,1.,1.,1.,1.,1.,1.,1.,1.,1.,1.,1.,1.,1.,1.,1.,1.,1.,
1.,1.,1.,1.,1.,1.,1.,1.,1.,1.,1.,1.,1.,1.,1.,1.,1.,1.,1.,1.,1.,1.,1.,1.,
1.,1.,1.,1.,1.,1.))
REPRESENTATION_ITEM('')
);
#223=(
BOUNDED_CURVE()
B_SPLINE_CURVE(5,(#34991,#34992,#34993,#34994,#34995,#34996,#34997,#34998,
#34999,#35000,#35001,#35002,#35003,#35004,#35005,#35006,#35007,#35008,#35009,
#35010,#35011,#35012,#35013,#35014,#35015,#35016,#35017,#35018,#35019,#35020,
#35021,#35022,#35023,#35024,#35025,#35026,#35027,#35028,#35029,#35030,#35031,
#35032,#35033,#35034,#35035,#35036,#35037,#35038,#35039,#35040,#35041,#35042,
#35043,#35044,#35045,#35046,#35047,#35048,#35049,#35050,#35051,#35052,#35053,
#35054,#35055,#35056,#35057,#35058,#35059,#35060),.UNSPECIFIED.,.F.,.F.)
B_SPLINE_CURVE_WITH_KNOTS((6,1,1,1,1,1,1,1,1,1,1,1,1,1,1,1,1,1,1,1,1,1,
1,1,1,1,1,1,1,1,1,1,1,1,1,1,1,1,1,1,1,1,1,1,1,1,1,1,1,1,1,1,1,1,1,1,1,1,
1,1,1,1,1,1,1,6),(0.00577184337449862,0.0153846153846154,0.0307692307692308,
0.0461538461538462,0.0615384615384615,0.0769230769230769,0.0923076923076923,
0.107692307692308,0.123076923076923,0.138461538461538,0.153846153846154,
0.169230769230769,0.184615384615385,0.2,0.215384615384615,0.230769230769231,
0.246153846153846,0.261538461538462,0.276923076923077,0.292307692307692,
0.307692307692308,0.323076923076923,0.338461538461538,0.353846153846154,
0.369230769230769,0.384615384615385,0.4,0.415384615384615,0.430769230769231,
0.446153846153846,0.461538461538462,0.476923076923077,0.492307692307692,
0.507692307692308,0.523076923076923,0.538461538461538,0.553846153846154,
0.569230769230769,0.584615384615384,0.6,0.615384615384615,0.63076923076923,
0.646153846153846,0.661538461538461,0.676923076923076,0.692307692307692,
0.707692307692307,0.723076923076922,0.738461538461538,0.753846153846153,
0.769230769230768,0.784615384615384,0.799999999999999,0.815384615384614,
0.83076923076923,0.846153846153845,0.86153846153846,0.876923076923076,0.892307692307691,
0.907692307692306,0.923076923076922,0.938461538461537,0.953846153846152,
0.969230769230768,0.984615384615383,1.),.UNSPECIFIED.)
CURVE()
GEOMETRIC_REPRESENTATION_ITEM()
RATIONAL_B_SPLINE_CURVE((1.,1.,1.,1.,1.,1.,1.,1.,1.,1.,1.,1.,1.,1.,1.,1.,
1.,1.,1.,1.,1.,1.,1.,1.,1.,1.,1.,1.,1.,1.,1.,1.,1.,1.,1.,1.,1.,1.,1.,1.,
1.,1.,1.,1.,1.,1.,1.,1.,1.,1.,1.,1.,1.,1.,1.,1.,1.,1.,1.,1.,1.,1.,1.,1.,
1.,1.,1.,1.,1.,1.))
REPRESENTATION_ITEM('')
);
#224=(
BOUNDED_CURVE()
B_SPLINE_CURVE(5,(#35064,#35065,#35066,#35067,#35068,#35069,#35070,#35071,
#35072,#35073,#35074,#35075,#35076,#35077,#35078,#35079,#35080,#35081,#35082,
#35083,#35084,#35085,#35086,#35087,#35088,#35089,#35090,#35091,#35092,#35093,
#35094,#35095,#35096,#35097,#35098,#35099,#35100,#35101,#35102,#35103,#35104,
#35105,#35106,#35107,#35108,#35109,#35110,#35111,#35112,#35113,#35114,#35115,
#35116,#35117,#35118,#35119,#35120,#35121,#35122,#35123,#35124,#35125,#35126,
#35127,#35128,#35129,#35130,#35131,#35132,#35133),.UNSPECIFIED.,.F.,.F.)
B_SPLINE_CURVE_WITH_KNOTS((6,1,1,1,1,1,1,1,1,1,1,1,1,1,1,1,1,1,1,1,1,1,
1,1,1,1,1,1,1,1,1,1,1,1,1,1,1,1,1,1,1,1,1,1,1,1,1,1,1,1,1,1,1,1,1,1,1,1,
1,1,1,1,1,1,1,6),(0.,0.0153846153846154,0.0307692307692308,0.0461538461538462,
0.0615384615384615,0.0769230769230769,0.0923076923076923,0.107692307692308,
0.123076923076923,0.138461538461538,0.153846153846154,0.169230769230769,
0.184615384615385,0.2,0.215384615384615,0.230769230769231,0.246153846153846,
0.261538461538462,0.276923076923077,0.292307692307692,0.307692307692308,
0.323076923076923,0.338461538461538,0.353846153846154,0.369230769230769,
0.384615384615385,0.4,0.415384615384615,0.430769230769231,0.446153846153846,
0.461538461538462,0.476923076923077,0.492307692307692,0.507692307692308,
0.523076923076923,0.538461538461538,0.553846153846154,0.569230769230769,
0.584615384615384,0.6,0.615384615384615,0.63076923076923,0.646153846153846,
0.661538461538461,0.676923076923076,0.692307692307692,0.707692307692307,
0.723076923076922,0.738461538461538,0.753846153846153,0.769230769230768,
0.784615384615384,0.799999999999999,0.815384615384614,0.83076923076923,
0.846153846153845,0.86153846153846,0.876923076923076,0.892307692307691,
0.907692307692306,0.923076923076922,0.938461538461537,0.953846153846152,
0.969230769230768,0.984615384615383,0.994228156739696),.UNSPECIFIED.)
CURVE()
GEOMETRIC_REPRESENTATION_ITEM()
RATIONAL_B_SPLINE_CURVE((1.,1.,1.,1.,1.,1.,1.,1.,1.,1.,1.,1.,1.,1.,1.,1.,
1.,1.,1.,1.,1.,1.,1.,1.,1.,1.,1.,1.,1.,1.,1.,1.,1.,1.,1.,1.,1.,1.,1.,1.,
1.,1.,1.,1.,1.,1.,1.,1.,1.,1.,1.,1.,1.,1.,1.,1.,1.,1.,1.,1.,1.,1.,1.,1.,
1.,1.,1.,1.,1.,1.))
REPRESENTATION_ITEM('')
);
#225=(
BOUNDED_CURVE()
B_SPLINE_CURVE(5,(#35137,#35138,#35139,#35140,#35141,#35142,#35143,#35144,
#35145,#35146,#35147,#35148,#35149,#35150,#35151,#35152,#35153,#35154,#35155,
#35156,#35157,#35158,#35159,#35160,#35161,#35162,#35163,#35164,#35165,#35166,
#35167,#35168,#35169,#35170,#35171,#35172,#35173,#35174,#35175,#35176,#35177,
#35178,#35179,#35180,#35181,#35182,#35183,#35184,#35185,#35186,#35187,#35188,
#35189,#35190,#35191,#35192,#35193,#35194,#35195,#35196,#35197,#35198,#35199,
#35200,#35201,#35202,#35203,#35204,#35205,#35206),.UNSPECIFIED.,.F.,.F.)
B_SPLINE_CURVE_WITH_KNOTS((6,1,1,1,1,1,1,1,1,1,1,1,1,1,1,1,1,1,1,1,1,1,
1,1,1,1,1,1,1,1,1,1,1,1,1,1,1,1,1,1,1,1,1,1,1,1,1,1,1,1,1,1,1,1,1,1,1,1,
1,1,1,1,1,1,1,6),(0.00577184337452068,0.0153846153846154,0.0307692307692308,
0.0461538461538462,0.0615384615384615,0.0769230769230769,0.0923076923076923,
0.107692307692308,0.123076923076923,0.138461538461538,0.153846153846154,
0.169230769230769,0.184615384615385,0.2,0.215384615384615,0.230769230769231,
0.246153846153846,0.261538461538462,0.276923076923077,0.292307692307692,
0.307692307692308,0.323076923076923,0.338461538461538,0.353846153846154,
0.369230769230769,0.384615384615385,0.4,0.415384615384615,0.430769230769231,
0.446153846153846,0.461538461538462,0.476923076923077,0.492307692307692,
0.507692307692308,0.523076923076923,0.538461538461538,0.553846153846154,
0.569230769230769,0.584615384615384,0.6,0.615384615384615,0.63076923076923,
0.646153846153846,0.661538461538461,0.676923076923076,0.692307692307692,
0.707692307692307,0.723076923076922,0.738461538461538,0.753846153846153,
0.769230769230768,0.784615384615384,0.799999999999999,0.815384615384614,
0.83076923076923,0.846153846153845,0.86153846153846,0.876923076923076,0.892307692307691,
0.907692307692306,0.923076923076922,0.938461538461537,0.953846153846152,
0.969230769230768,0.984615384615383,1.),.UNSPECIFIED.)
CURVE()
GEOMETRIC_REPRESENTATION_ITEM()
RATIONAL_B_SPLINE_CURVE((1.,1.,1.,1.,1.,1.,1.,1.,1.,1.,1.,1.,1.,1.,1.,1.,
1.,1.,1.,1.,1.,1.,1.,1.,1.,1.,1.,1.,1.,1.,1.,1.,1.,1.,1.,1.,1.,1.,1.,1.,
1.,1.,1.,1.,1.,1.,1.,1.,1.,1.,1.,1.,1.,1.,1.,1.,1.,1.,1.,1.,1.,1.,1.,1.,
1.,1.,1.,1.,1.,1.))
REPRESENTATION_ITEM('')
);
#226=(
BOUNDED_CURVE()
B_SPLINE_CURVE(5,(#35210,#35211,#35212,#35213,#35214,#35215,#35216,#35217,
#35218,#35219,#35220,#35221,#35222,#35223,#35224,#35225,#35226,#35227,#35228,
#35229,#35230,#35231,#35232,#35233,#35234,#35235,#35236,#35237,#35238,#35239,
#35240,#35241,#35242,#35243,#35244,#35245,#35246,#35247,#35248,#35249,#35250,
#35251,#35252,#35253,#35254,#35255,#35256,#35257,#35258,#35259,#35260,#35261,
#35262,#35263,#35264,#35265,#35266,#35267,#35268,#35269,#35270,#35271,#35272,
#35273,#35274,#35275,#35276,#35277,#35278,#35279),.UNSPECIFIED.,.F.,.F.)
B_SPLINE_CURVE_WITH_KNOTS((6,1,1,1,1,1,1,1,1,1,1,1,1,1,1,1,1,1,1,1,1,1,
1,1,1,1,1,1,1,1,1,1,1,1,1,1,1,1,1,1,1,1,1,1,1,1,1,1,1,1,1,1,1,1,1,1,1,1,
1,1,1,1,1,1,1,6),(0.,0.0153846153846154,0.0307692307692308,0.0461538461538462,
0.0615384615384615,0.0769230769230769,0.0923076923076923,0.107692307692308,
0.123076923076923,0.138461538461538,0.153846153846154,0.169230769230769,
0.184615384615385,0.2,0.215384615384615,0.230769230769231,0.246153846153846,
0.261538461538462,0.276923076923077,0.292307692307692,0.307692307692308,
0.323076923076923,0.338461538461538,0.353846153846154,0.369230769230769,
0.384615384615385,0.4,0.415384615384615,0.430769230769231,0.446153846153846,
0.461538461538462,0.476923076923077,0.492307692307692,0.507692307692308,
0.523076923076923,0.538461538461538,0.553846153846154,0.569230769230769,
0.584615384615384,0.6,0.615384615384615,0.63076923076923,0.646153846153846,
0.661538461538461,0.676923076923076,0.692307692307692,0.707692307692307,
0.723076923076922,0.738461538461538,0.753846153846153,0.769230769230768,
0.784615384615384,0.799999999999999,0.815384615384614,0.83076923076923,
0.846153846153845,0.86153846153846,0.876923076923076,0.892307692307691,
0.907692307692306,0.923076923076922,0.938461538461537,0.953846153846152,
0.969230769230768,0.984615384615383,0.994228156739698),.UNSPECIFIED.)
CURVE()
GEOMETRIC_REPRESENTATION_ITEM()
RATIONAL_B_SPLINE_CURVE((1.,1.,1.,1.,1.,1.,1.,1.,1.,1.,1.,1.,1.,1.,1.,1.,
1.,1.,1.,1.,1.,1.,1.,1.,1.,1.,1.,1.,1.,1.,1.,1.,1.,1.,1.,1.,1.,1.,1.,1.,
1.,1.,1.,1.,1.,1.,1.,1.,1.,1.,1.,1.,1.,1.,1.,1.,1.,1.,1.,1.,1.,1.,1.,1.,
1.,1.,1.,1.,1.,1.))
REPRESENTATION_ITEM('')
);
#227=(
BOUNDED_CURVE()
B_SPLINE_CURVE(5,(#35283,#35284,#35285,#35286,#35287,#35288,#35289,#35290,
#35291,#35292,#35293,#35294,#35295,#35296,#35297,#35298,#35299,#35300,#35301,
#35302,#35303,#35304,#35305,#35306,#35307,#35308,#35309,#35310,#35311,#35312,
#35313,#35314,#35315,#35316,#35317,#35318,#35319,#35320,#35321,#35322,#35323,
#35324,#35325,#35326,#35327,#35328,#35329,#35330,#35331,#35332,#35333,#35334,
#35335,#35336,#35337,#35338,#35339,#35340,#35341,#35342,#35343,#35344,#35345,
#35346,#35347,#35348,#35349,#35350,#35351,#35352),.UNSPECIFIED.,.F.,.F.)
B_SPLINE_CURVE_WITH_KNOTS((6,1,1,1,1,1,1,1,1,1,1,1,1,1,1,1,1,1,1,1,1,1,
1,1,1,1,1,1,1,1,1,1,1,1,1,1,1,1,1,1,1,1,1,1,1,1,1,1,1,1,1,1,1,1,1,1,1,1,
1,1,1,1,1,1,1,6),(0.00577184337451607,0.0153846153846154,0.0307692307692308,
0.0461538461538462,0.0615384615384615,0.0769230769230769,0.0923076923076923,
0.107692307692308,0.123076923076923,0.138461538461538,0.153846153846154,
0.169230769230769,0.184615384615385,0.2,0.215384615384615,0.230769230769231,
0.246153846153846,0.261538461538462,0.276923076923077,0.292307692307692,
0.307692307692308,0.323076923076923,0.338461538461538,0.353846153846154,
0.369230769230769,0.384615384615385,0.4,0.415384615384615,0.430769230769231,
0.446153846153846,0.461538461538462,0.476923076923077,0.492307692307692,
0.507692307692308,0.523076923076923,0.538461538461538,0.553846153846154,
0.569230769230769,0.584615384615384,0.6,0.615384615384615,0.63076923076923,
0.646153846153846,0.661538461538461,0.676923076923076,0.692307692307692,
0.707692307692307,0.723076923076922,0.738461538461538,0.753846153846153,
0.769230769230768,0.784615384615384,0.799999999999999,0.815384615384614,
0.83076923076923,0.846153846153845,0.86153846153846,0.876923076923076,0.892307692307691,
0.907692307692306,0.923076923076922,0.938461538461537,0.953846153846152,
0.969230769230768,0.984615384615383,1.),.UNSPECIFIED.)
CURVE()
GEOMETRIC_REPRESENTATION_ITEM()
RATIONAL_B_SPLINE_CURVE((1.,1.,1.,1.,1.,1.,1.,1.,1.,1.,1.,1.,1.,1.,1.,1.,
1.,1.,1.,1.,1.,1.,1.,1.,1.,1.,1.,1.,1.,1.,1.,1.,1.,1.,1.,1.,1.,1.,1.,1.,
1.,1.,1.,1.,1.,1.,1.,1.,1.,1.,1.,1.,1.,1.,1.,1.,1.,1.,1.,1.,1.,1.,1.,1.,
1.,1.,1.,1.,1.,1.))
REPRESENTATION_ITEM('')
);
#228=(
BOUNDED_CURVE()
B_SPLINE_CURVE(5,(#35356,#35357,#35358,#35359,#35360,#35361,#35362,#35363,
#35364,#35365,#35366,#35367,#35368,#35369,#35370,#35371,#35372,#35373,#35374,
#35375,#35376,#35377,#35378,#35379,#35380,#35381,#35382,#35383,#35384,#35385,
#35386,#35387,#35388,#35389,#35390,#35391,#35392,#35393,#35394,#35395,#35396,
#35397,#35398,#35399,#35400,#35401,#35402,#35403,#35404,#35405,#35406,#35407,
#35408,#35409,#35410,#35411,#35412,#35413,#35414,#35415,#35416,#35417,#35418,
#35419,#35420,#35421,#35422,#35423,#35424,#35425),.UNSPECIFIED.,.F.,.F.)
B_SPLINE_CURVE_WITH_KNOTS((6,1,1,1,1,1,1,1,1,1,1,1,1,1,1,1,1,1,1,1,1,1,
1,1,1,1,1,1,1,1,1,1,1,1,1,1,1,1,1,1,1,1,1,1,1,1,1,1,1,1,1,1,1,1,1,1,1,1,
1,1,1,1,1,1,1,6),(0.,0.0153846153846154,0.0307692307692308,0.0461538461538462,
0.0615384615384615,0.0769230769230769,0.0923076923076923,0.107692307692308,
0.123076923076923,0.138461538461538,0.153846153846154,0.169230769230769,
0.184615384615385,0.2,0.215384615384615,0.230769230769231,0.246153846153846,
0.261538461538462,0.276923076923077,0.292307692307692,0.307692307692308,
0.323076923076923,0.338461538461538,0.353846153846154,0.369230769230769,
0.384615384615385,0.4,0.415384615384615,0.430769230769231,0.446153846153846,
0.461538461538462,0.476923076923077,0.492307692307692,0.507692307692308,
0.523076923076923,0.538461538461538,0.553846153846154,0.569230769230769,
0.584615384615384,0.6,0.615384615384615,0.63076923076923,0.646153846153846,
0.661538461538461,0.676923076923076,0.692307692307692,0.707692307692307,
0.723076923076922,0.738461538461538,0.753846153846153,0.769230769230768,
0.784615384615384,0.799999999999999,0.815384615384614,0.83076923076923,
0.846153846153845,0.86153846153846,0.876923076923076,0.892307692307691,
0.907692307692306,0.923076923076922,0.938461538461537,0.953846153846152,
0.969230769230768,0.984615384615383,0.994228156739704),.UNSPECIFIED.)
CURVE()
GEOMETRIC_REPRESENTATION_ITEM()
RATIONAL_B_SPLINE_CURVE((1.,1.,1.,1.,1.,1.,1.,1.,1.,1.,1.,1.,1.,1.,1.,1.,
1.,1.,1.,1.,1.,1.,1.,1.,1.,1.,1.,1.,1.,1.,1.,1.,1.,1.,1.,1.,1.,1.,1.,1.,
1.,1.,1.,1.,1.,1.,1.,1.,1.,1.,1.,1.,1.,1.,1.,1.,1.,1.,1.,1.,1.,1.,1.,1.,
1.,1.,1.,1.,1.,1.))
REPRESENTATION_ITEM('')
);
#229=(
BOUNDED_CURVE()
B_SPLINE_CURVE(5,(#35429,#35430,#35431,#35432,#35433,#35434,#35435,#35436,
#35437,#35438,#35439,#35440,#35441,#35442,#35443,#35444,#35445,#35446,#35447,
#35448,#35449,#35450,#35451,#35452,#35453,#35454,#35455,#35456,#35457,#35458,
#35459,#35460,#35461,#35462,#35463,#35464,#35465,#35466,#35467,#35468,#35469,
#35470,#35471,#35472,#35473,#35474,#35475,#35476,#35477,#35478,#35479,#35480,
#35481,#35482,#35483,#35484,#35485,#35486,#35487,#35488,#35489,#35490,#35491,
#35492,#35493,#35494,#35495,#35496,#35497,#35498),.UNSPECIFIED.,.F.,.F.)
B_SPLINE_CURVE_WITH_KNOTS((6,1,1,1,1,1,1,1,1,1,1,1,1,1,1,1,1,1,1,1,1,1,
1,1,1,1,1,1,1,1,1,1,1,1,1,1,1,1,1,1,1,1,1,1,1,1,1,1,1,1,1,1,1,1,1,1,1,1,
1,1,1,1,1,1,1,6),(0.00577184337449692,0.0153846153846154,0.0307692307692308,
0.0461538461538462,0.0615384615384615,0.0769230769230769,0.0923076923076923,
0.107692307692308,0.123076923076923,0.138461538461538,0.153846153846154,
0.169230769230769,0.184615384615385,0.2,0.215384615384615,0.230769230769231,
0.246153846153846,0.261538461538462,0.276923076923077,0.292307692307692,
0.307692307692308,0.323076923076923,0.338461538461538,0.353846153846154,
0.369230769230769,0.384615384615385,0.4,0.415384615384615,0.430769230769231,
0.446153846153846,0.461538461538462,0.476923076923077,0.492307692307692,
0.507692307692308,0.523076923076923,0.538461538461538,0.553846153846154,
0.569230769230769,0.584615384615384,0.6,0.615384615384615,0.63076923076923,
0.646153846153846,0.661538461538461,0.676923076923076,0.692307692307692,
0.707692307692307,0.723076923076922,0.738461538461538,0.753846153846153,
0.769230769230768,0.784615384615384,0.799999999999999,0.815384615384614,
0.83076923076923,0.846153846153845,0.86153846153846,0.876923076923076,0.892307692307691,
0.907692307692306,0.923076923076922,0.938461538461537,0.953846153846152,
0.969230769230768,0.984615384615383,1.),.UNSPECIFIED.)
CURVE()
GEOMETRIC_REPRESENTATION_ITEM()
RATIONAL_B_SPLINE_CURVE((1.,1.,1.,1.,1.,1.,1.,1.,1.,1.,1.,1.,1.,1.,1.,1.,
1.,1.,1.,1.,1.,1.,1.,1.,1.,1.,1.,1.,1.,1.,1.,1.,1.,1.,1.,1.,1.,1.,1.,1.,
1.,1.,1.,1.,1.,1.,1.,1.,1.,1.,1.,1.,1.,1.,1.,1.,1.,1.,1.,1.,1.,1.,1.,1.,
1.,1.,1.,1.,1.,1.))
REPRESENTATION_ITEM('')
);
#230=(
BOUNDED_CURVE()
B_SPLINE_CURVE(5,(#35502,#35503,#35504,#35505,#35506,#35507,#35508,#35509,
#35510,#35511,#35512,#35513,#35514,#35515,#35516,#35517,#35518,#35519,#35520,
#35521,#35522,#35523,#35524,#35525,#35526,#35527,#35528,#35529,#35530,#35531,
#35532,#35533,#35534,#35535,#35536,#35537,#35538,#35539,#35540,#35541,#35542,
#35543,#35544,#35545,#35546,#35547,#35548,#35549,#35550,#35551,#35552,#35553,
#35554,#35555,#35556,#35557,#35558,#35559,#35560,#35561,#35562,#35563,#35564,
#35565,#35566,#35567,#35568,#35569,#35570,#35571),.UNSPECIFIED.,.F.,.F.)
B_SPLINE_CURVE_WITH_KNOTS((6,1,1,1,1,1,1,1,1,1,1,1,1,1,1,1,1,1,1,1,1,1,
1,1,1,1,1,1,1,1,1,1,1,1,1,1,1,1,1,1,1,1,1,1,1,1,1,1,1,1,1,1,1,1,1,1,1,1,
1,1,1,1,1,1,1,6),(0.,0.0153846153846154,0.0307692307692308,0.0461538461538462,
0.0615384615384615,0.0769230769230769,0.0923076923076923,0.107692307692308,
0.123076923076923,0.138461538461538,0.153846153846154,0.169230769230769,
0.184615384615385,0.2,0.215384615384615,0.230769230769231,0.246153846153846,
0.261538461538462,0.276923076923077,0.292307692307692,0.307692307692308,
0.323076923076923,0.338461538461538,0.353846153846154,0.369230769230769,
0.384615384615385,0.4,0.415384615384615,0.430769230769231,0.446153846153846,
0.461538461538462,0.476923076923077,0.492307692307692,0.507692307692308,
0.523076923076923,0.538461538461538,0.553846153846154,0.569230769230769,
0.584615384615384,0.6,0.615384615384615,0.63076923076923,0.646153846153846,
0.661538461538461,0.676923076923076,0.692307692307692,0.707692307692307,
0.723076923076922,0.738461538461538,0.753846153846153,0.769230769230768,
0.784615384615384,0.799999999999999,0.815384615384614,0.83076923076923,
0.846153846153845,0.86153846153846,0.876923076923076,0.892307692307691,
0.907692307692306,0.923076923076922,0.938461538461537,0.953846153846152,
0.969230769230768,0.984615384615383,0.994228156739711),.UNSPECIFIED.)
CURVE()
GEOMETRIC_REPRESENTATION_ITEM()
RATIONAL_B_SPLINE_CURVE((1.,1.,1.,1.,1.,1.,1.,1.,1.,1.,1.,1.,1.,1.,1.,1.,
1.,1.,1.,1.,1.,1.,1.,1.,1.,1.,1.,1.,1.,1.,1.,1.,1.,1.,1.,1.,1.,1.,1.,1.,
1.,1.,1.,1.,1.,1.,1.,1.,1.,1.,1.,1.,1.,1.,1.,1.,1.,1.,1.,1.,1.,1.,1.,1.,
1.,1.,1.,1.,1.,1.))
REPRESENTATION_ITEM('')
);
#231=(
BOUNDED_CURVE()
B_SPLINE_CURVE(5,(#35575,#35576,#35577,#35578,#35579,#35580,#35581,#35582,
#35583,#35584,#35585,#35586,#35587,#35588,#35589,#35590,#35591,#35592,#35593,
#35594,#35595,#35596,#35597,#35598,#35599,#35600,#35601,#35602,#35603,#35604,
#35605,#35606,#35607,#35608,#35609,#35610,#35611,#35612,#35613,#35614,#35615,
#35616,#35617,#35618,#35619,#35620,#35621,#35622,#35623,#35624,#35625,#35626,
#35627,#35628,#35629,#35630,#35631,#35632,#35633,#35634,#35635,#35636,#35637,
#35638,#35639,#35640,#35641,#35642,#35643,#35644),.UNSPECIFIED.,.F.,.F.)
B_SPLINE_CURVE_WITH_KNOTS((6,1,1,1,1,1,1,1,1,1,1,1,1,1,1,1,1,1,1,1,1,1,
1,1,1,1,1,1,1,1,1,1,1,1,1,1,1,1,1,1,1,1,1,1,1,1,1,1,1,1,1,1,1,1,1,1,1,1,
1,1,1,1,1,1,1,6),(0.00577184337450058,0.0153846153846154,0.0307692307692308,
0.0461538461538462,0.0615384615384615,0.0769230769230769,0.0923076923076923,
0.107692307692308,0.123076923076923,0.138461538461538,0.153846153846154,
0.169230769230769,0.184615384615385,0.2,0.215384615384615,0.230769230769231,
0.246153846153846,0.261538461538462,0.276923076923077,0.292307692307692,
0.307692307692308,0.323076923076923,0.338461538461538,0.353846153846154,
0.369230769230769,0.384615384615385,0.4,0.415384615384615,0.430769230769231,
0.446153846153846,0.461538461538462,0.476923076923077,0.492307692307692,
0.507692307692308,0.523076923076923,0.538461538461538,0.553846153846154,
0.569230769230769,0.584615384615384,0.6,0.615384615384615,0.63076923076923,
0.646153846153846,0.661538461538461,0.676923076923076,0.692307692307692,
0.707692307692307,0.723076923076922,0.738461538461538,0.753846153846153,
0.769230769230768,0.784615384615384,0.799999999999999,0.815384615384614,
0.83076923076923,0.846153846153845,0.86153846153846,0.876923076923076,0.892307692307691,
0.907692307692306,0.923076923076922,0.938461538461537,0.953846153846152,
0.969230769230768,0.984615384615383,1.),.UNSPECIFIED.)
CURVE()
GEOMETRIC_REPRESENTATION_ITEM()
RATIONAL_B_SPLINE_CURVE((1.,1.,1.,1.,1.,1.,1.,1.,1.,1.,1.,1.,1.,1.,1.,1.,
1.,1.,1.,1.,1.,1.,1.,1.,1.,1.,1.,1.,1.,1.,1.,1.,1.,1.,1.,1.,1.,1.,1.,1.,
1.,1.,1.,1.,1.,1.,1.,1.,1.,1.,1.,1.,1.,1.,1.,1.,1.,1.,1.,1.,1.,1.,1.,1.,
1.,1.,1.,1.,1.,1.))
REPRESENTATION_ITEM('')
);
#232=(
BOUNDED_CURVE()
B_SPLINE_CURVE(5,(#35648,#35649,#35650,#35651,#35652,#35653,#35654,#35655,
#35656,#35657,#35658,#35659,#35660,#35661,#35662,#35663,#35664,#35665,#35666,
#35667,#35668,#35669,#35670,#35671,#35672,#35673,#35674,#35675,#35676,#35677,
#35678,#35679,#35680,#35681,#35682,#35683,#35684,#35685,#35686,#35687,#35688,
#35689,#35690,#35691,#35692,#35693,#35694,#35695,#35696,#35697,#35698,#35699,
#35700,#35701,#35702,#35703,#35704,#35705,#35706,#35707,#35708,#35709,#35710,
#35711,#35712,#35713,#35714,#35715,#35716,#35717),.UNSPECIFIED.,.F.,.F.)
B_SPLINE_CURVE_WITH_KNOTS((6,1,1,1,1,1,1,1,1,1,1,1,1,1,1,1,1,1,1,1,1,1,
1,1,1,1,1,1,1,1,1,1,1,1,1,1,1,1,1,1,1,1,1,1,1,1,1,1,1,1,1,1,1,1,1,1,1,1,
1,1,1,1,1,1,1,6),(0.,0.0153846153846154,0.0307692307692308,0.0461538461538462,
0.0615384615384615,0.0769230769230769,0.0923076923076923,0.107692307692308,
0.123076923076923,0.138461538461538,0.153846153846154,0.169230769230769,
0.184615384615385,0.2,0.215384615384615,0.230769230769231,0.246153846153846,
0.261538461538462,0.276923076923077,0.292307692307692,0.307692307692308,
0.323076923076923,0.338461538461538,0.353846153846154,0.369230769230769,
0.384615384615385,0.4,0.415384615384615,0.430769230769231,0.446153846153846,
0.461538461538462,0.476923076923077,0.492307692307692,0.507692307692308,
0.523076923076923,0.538461538461538,0.553846153846154,0.569230769230769,
0.584615384615384,0.6,0.615384615384615,0.63076923076923,0.646153846153846,
0.661538461538461,0.676923076923076,0.692307692307692,0.707692307692307,
0.723076923076922,0.738461538461538,0.753846153846153,0.769230769230768,
0.784615384615384,0.799999999999999,0.815384615384614,0.83076923076923,
0.846153846153845,0.86153846153846,0.876923076923076,0.892307692307691,
0.907692307692306,0.923076923076922,0.938461538461537,0.953846153846152,
0.969230769230768,0.984615384615383,0.994228156739701),.UNSPECIFIED.)
CURVE()
GEOMETRIC_REPRESENTATION_ITEM()
RATIONAL_B_SPLINE_CURVE((1.,1.,1.,1.,1.,1.,1.,1.,1.,1.,1.,1.,1.,1.,1.,1.,
1.,1.,1.,1.,1.,1.,1.,1.,1.,1.,1.,1.,1.,1.,1.,1.,1.,1.,1.,1.,1.,1.,1.,1.,
1.,1.,1.,1.,1.,1.,1.,1.,1.,1.,1.,1.,1.,1.,1.,1.,1.,1.,1.,1.,1.,1.,1.,1.,
1.,1.,1.,1.,1.,1.))
REPRESENTATION_ITEM('')
);
#233=(
BOUNDED_CURVE()
B_SPLINE_CURVE(5,(#35721,#35722,#35723,#35724,#35725,#35726,#35727,#35728,
#35729,#35730,#35731,#35732,#35733,#35734,#35735,#35736,#35737,#35738,#35739,
#35740,#35741,#35742,#35743,#35744,#35745,#35746,#35747,#35748,#35749,#35750,
#35751,#35752,#35753,#35754,#35755,#35756,#35757,#35758,#35759,#35760,#35761,
#35762,#35763,#35764,#35765,#35766,#35767,#35768,#35769,#35770,#35771,#35772,
#35773,#35774,#35775,#35776,#35777,#35778,#35779,#35780,#35781,#35782,#35783,
#35784,#35785,#35786,#35787,#35788,#35789,#35790),.UNSPECIFIED.,.F.,.F.)
B_SPLINE_CURVE_WITH_KNOTS((6,1,1,1,1,1,1,1,1,1,1,1,1,1,1,1,1,1,1,1,1,1,
1,1,1,1,1,1,1,1,1,1,1,1,1,1,1,1,1,1,1,1,1,1,1,1,1,1,1,1,1,1,1,1,1,1,1,1,
1,1,1,1,1,1,1,6),(0.0057718433745091,0.0153846153846154,0.0307692307692308,
0.0461538461538462,0.0615384615384615,0.0769230769230769,0.0923076923076923,
0.107692307692308,0.123076923076923,0.138461538461538,0.153846153846154,
0.169230769230769,0.184615384615385,0.2,0.215384615384615,0.230769230769231,
0.246153846153846,0.261538461538462,0.276923076923077,0.292307692307692,
0.307692307692308,0.323076923076923,0.338461538461538,0.353846153846154,
0.369230769230769,0.384615384615385,0.4,0.415384615384615,0.430769230769231,
0.446153846153846,0.461538461538462,0.476923076923077,0.492307692307692,
0.507692307692308,0.523076923076923,0.538461538461538,0.553846153846154,
0.569230769230769,0.584615384615384,0.6,0.615384615384615,0.63076923076923,
0.646153846153846,0.661538461538461,0.676923076923076,0.692307692307692,
0.707692307692307,0.723076923076922,0.738461538461538,0.753846153846153,
0.769230769230768,0.784615384615384,0.799999999999999,0.815384615384614,
0.83076923076923,0.846153846153845,0.86153846153846,0.876923076923076,0.892307692307691,
0.907692307692306,0.923076923076922,0.938461538461537,0.953846153846152,
0.969230769230768,0.984615384615383,1.),.UNSPECIFIED.)
CURVE()
GEOMETRIC_REPRESENTATION_ITEM()
RATIONAL_B_SPLINE_CURVE((1.,1.,1.,1.,1.,1.,1.,1.,1.,1.,1.,1.,1.,1.,1.,1.,
1.,1.,1.,1.,1.,1.,1.,1.,1.,1.,1.,1.,1.,1.,1.,1.,1.,1.,1.,1.,1.,1.,1.,1.,
1.,1.,1.,1.,1.,1.,1.,1.,1.,1.,1.,1.,1.,1.,1.,1.,1.,1.,1.,1.,1.,1.,1.,1.,
1.,1.,1.,1.,1.,1.))
REPRESENTATION_ITEM('')
);
#234=(
BOUNDED_CURVE()
B_SPLINE_CURVE(5,(#35794,#35795,#35796,#35797,#35798,#35799,#35800,#35801,
#35802,#35803,#35804,#35805,#35806,#35807,#35808,#35809,#35810,#35811,#35812,
#35813,#35814,#35815,#35816,#35817,#35818,#35819,#35820,#35821,#35822,#35823,
#35824,#35825,#35826,#35827,#35828,#35829,#35830,#35831,#35832,#35833,#35834,
#35835,#35836,#35837,#35838,#35839,#35840,#35841,#35842,#35843,#35844,#35845,
#35846,#35847,#35848,#35849,#35850,#35851,#35852,#35853,#35854,#35855,#35856,
#35857,#35858,#35859,#35860,#35861,#35862,#35863),.UNSPECIFIED.,.F.,.F.)
B_SPLINE_CURVE_WITH_KNOTS((6,1,1,1,1,1,1,1,1,1,1,1,1,1,1,1,1,1,1,1,1,1,
1,1,1,1,1,1,1,1,1,1,1,1,1,1,1,1,1,1,1,1,1,1,1,1,1,1,1,1,1,1,1,1,1,1,1,1,
1,1,1,1,1,1,1,6),(0.,0.0153846153846154,0.0307692307692308,0.0461538461538462,
0.0615384615384615,0.0769230769230769,0.0923076923076923,0.107692307692308,
0.123076923076923,0.138461538461538,0.153846153846154,0.169230769230769,
0.184615384615385,0.2,0.215384615384615,0.230769230769231,0.246153846153846,
0.261538461538462,0.276923076923077,0.292307692307692,0.307692307692308,
0.323076923076923,0.338461538461538,0.353846153846154,0.369230769230769,
0.384615384615385,0.4,0.415384615384615,0.430769230769231,0.446153846153846,
0.461538461538462,0.476923076923077,0.492307692307692,0.507692307692308,
0.523076923076923,0.538461538461538,0.553846153846154,0.569230769230769,
0.584615384615384,0.6,0.615384615384615,0.63076923076923,0.646153846153846,
0.661538461538461,0.676923076923076,0.692307692307692,0.707692307692307,
0.723076923076922,0.738461538461538,0.753846153846153,0.769230769230768,
0.784615384615384,0.799999999999999,0.815384615384614,0.83076923076923,
0.846153846153845,0.86153846153846,0.876923076923076,0.892307692307691,
0.907692307692306,0.923076923076922,0.938461538461537,0.953846153846152,
0.969230769230768,0.984615384615383,0.994228156739689),.UNSPECIFIED.)
CURVE()
GEOMETRIC_REPRESENTATION_ITEM()
RATIONAL_B_SPLINE_CURVE((1.,1.,1.,1.,1.,1.,1.,1.,1.,1.,1.,1.,1.,1.,1.,1.,
1.,1.,1.,1.,1.,1.,1.,1.,1.,1.,1.,1.,1.,1.,1.,1.,1.,1.,1.,1.,1.,1.,1.,1.,
1.,1.,1.,1.,1.,1.,1.,1.,1.,1.,1.,1.,1.,1.,1.,1.,1.,1.,1.,1.,1.,1.,1.,1.,
1.,1.,1.,1.,1.,1.))
REPRESENTATION_ITEM('')
);
#235=(
BOUNDED_CURVE()
B_SPLINE_CURVE(5,(#35867,#35868,#35869,#35870,#35871,#35872,#35873,#35874,
#35875,#35876,#35877,#35878,#35879,#35880,#35881,#35882,#35883,#35884,#35885,
#35886,#35887,#35888,#35889,#35890,#35891,#35892,#35893,#35894,#35895,#35896,
#35897,#35898,#35899,#35900,#35901,#35902,#35903,#35904,#35905,#35906,#35907,
#35908,#35909,#35910,#35911,#35912,#35913,#35914,#35915,#35916,#35917,#35918,
#35919,#35920,#35921,#35922,#35923,#35924,#35925,#35926,#35927,#35928,#35929,
#35930,#35931,#35932,#35933,#35934,#35935,#35936),.UNSPECIFIED.,.F.,.F.)
B_SPLINE_CURVE_WITH_KNOTS((6,1,1,1,1,1,1,1,1,1,1,1,1,1,1,1,1,1,1,1,1,1,
1,1,1,1,1,1,1,1,1,1,1,1,1,1,1,1,1,1,1,1,1,1,1,1,1,1,1,1,1,1,1,1,1,1,1,1,
1,1,1,1,1,1,1,6),(0.00577184337450777,0.0153846153846154,0.0307692307692308,
0.0461538461538462,0.0615384615384615,0.0769230769230769,0.0923076923076923,
0.107692307692308,0.123076923076923,0.138461538461538,0.153846153846154,
0.169230769230769,0.184615384615385,0.2,0.215384615384615,0.230769230769231,
0.246153846153846,0.261538461538462,0.276923076923077,0.292307692307692,
0.307692307692308,0.323076923076923,0.338461538461538,0.353846153846154,
0.369230769230769,0.384615384615385,0.4,0.415384615384615,0.430769230769231,
0.446153846153846,0.461538461538462,0.476923076923077,0.492307692307692,
0.507692307692308,0.523076923076923,0.538461538461538,0.553846153846154,
0.569230769230769,0.584615384615384,0.6,0.615384615384615,0.63076923076923,
0.646153846153846,0.661538461538461,0.676923076923076,0.692307692307692,
0.707692307692307,0.723076923076922,0.738461538461538,0.753846153846153,
0.769230769230768,0.784615384615384,0.799999999999999,0.815384615384614,
0.83076923076923,0.846153846153845,0.86153846153846,0.876923076923076,0.892307692307691,
0.907692307692306,0.923076923076922,0.938461538461537,0.953846153846152,
0.969230769230768,0.984615384615383,1.),.UNSPECIFIED.)
CURVE()
GEOMETRIC_REPRESENTATION_ITEM()
RATIONAL_B_SPLINE_CURVE((1.,1.,1.,1.,1.,1.,1.,1.,1.,1.,1.,1.,1.,1.,1.,1.,
1.,1.,1.,1.,1.,1.,1.,1.,1.,1.,1.,1.,1.,1.,1.,1.,1.,1.,1.,1.,1.,1.,1.,1.,
1.,1.,1.,1.,1.,1.,1.,1.,1.,1.,1.,1.,1.,1.,1.,1.,1.,1.,1.,1.,1.,1.,1.,1.,
1.,1.,1.,1.,1.,1.))
REPRESENTATION_ITEM('')
);
#236=(
BOUNDED_CURVE()
B_SPLINE_CURVE(5,(#35940,#35941,#35942,#35943,#35944,#35945,#35946,#35947,
#35948,#35949,#35950,#35951,#35952,#35953,#35954,#35955,#35956,#35957,#35958,
#35959,#35960,#35961,#35962,#35963,#35964,#35965,#35966,#35967,#35968,#35969,
#35970,#35971,#35972,#35973,#35974,#35975,#35976,#35977,#35978,#35979,#35980,
#35981,#35982,#35983,#35984,#35985,#35986,#35987,#35988,#35989,#35990,#35991,
#35992,#35993,#35994,#35995,#35996,#35997,#35998,#35999,#36000,#36001,#36002,
#36003,#36004,#36005,#36006,#36007,#36008,#36009),.UNSPECIFIED.,.F.,.F.)
B_SPLINE_CURVE_WITH_KNOTS((6,1,1,1,1,1,1,1,1,1,1,1,1,1,1,1,1,1,1,1,1,1,
1,1,1,1,1,1,1,1,1,1,1,1,1,1,1,1,1,1,1,1,1,1,1,1,1,1,1,1,1,1,1,1,1,1,1,1,
1,1,1,1,1,1,1,6),(0.,0.0153846153846154,0.0307692307692308,0.0461538461538462,
0.0615384615384615,0.0769230769230769,0.0923076923076923,0.107692307692308,
0.123076923076923,0.138461538461538,0.153846153846154,0.169230769230769,
0.184615384615385,0.2,0.215384615384615,0.230769230769231,0.246153846153846,
0.261538461538462,0.276923076923077,0.292307692307692,0.307692307692308,
0.323076923076923,0.338461538461538,0.353846153846154,0.369230769230769,
0.384615384615385,0.4,0.415384615384615,0.430769230769231,0.446153846153846,
0.461538461538462,0.476923076923077,0.492307692307692,0.507692307692308,
0.523076923076923,0.538461538461538,0.553846153846154,0.569230769230769,
0.584615384615384,0.6,0.615384615384615,0.63076923076923,0.646153846153846,
0.661538461538461,0.676923076923076,0.692307692307692,0.707692307692307,
0.723076923076922,0.738461538461538,0.753846153846153,0.769230769230768,
0.784615384615384,0.799999999999999,0.815384615384614,0.83076923076923,
0.846153846153845,0.86153846153846,0.876923076923076,0.892307692307691,
0.907692307692306,0.923076923076922,0.938461538461537,0.953846153846152,
0.969230769230768,0.984615384615383,0.994228156739701),.UNSPECIFIED.)
CURVE()
GEOMETRIC_REPRESENTATION_ITEM()
RATIONAL_B_SPLINE_CURVE((1.,1.,1.,1.,1.,1.,1.,1.,1.,1.,1.,1.,1.,1.,1.,1.,
1.,1.,1.,1.,1.,1.,1.,1.,1.,1.,1.,1.,1.,1.,1.,1.,1.,1.,1.,1.,1.,1.,1.,1.,
1.,1.,1.,1.,1.,1.,1.,1.,1.,1.,1.,1.,1.,1.,1.,1.,1.,1.,1.,1.,1.,1.,1.,1.,
1.,1.,1.,1.,1.,1.))
REPRESENTATION_ITEM('')
);
#237=(
BOUNDED_CURVE()
B_SPLINE_CURVE(5,(#36013,#36014,#36015,#36016,#36017,#36018,#36019,#36020,
#36021,#36022,#36023,#36024,#36025,#36026,#36027,#36028,#36029,#36030,#36031,
#36032,#36033,#36034,#36035,#36036,#36037,#36038,#36039,#36040,#36041,#36042,
#36043,#36044,#36045,#36046,#36047,#36048,#36049,#36050,#36051,#36052,#36053,
#36054,#36055,#36056,#36057,#36058,#36059,#36060,#36061,#36062,#36063,#36064,
#36065,#36066,#36067,#36068,#36069,#36070,#36071,#36072,#36073,#36074,#36075,
#36076,#36077,#36078,#36079,#36080,#36081,#36082),.UNSPECIFIED.,.F.,.F.)
B_SPLINE_CURVE_WITH_KNOTS((6,1,1,1,1,1,1,1,1,1,1,1,1,1,1,1,1,1,1,1,1,1,
1,1,1,1,1,1,1,1,1,1,1,1,1,1,1,1,1,1,1,1,1,1,1,1,1,1,1,1,1,1,1,1,1,1,1,1,
1,1,1,1,1,1,1,6),(0.00577184337450172,0.0153846153846154,0.0307692307692308,
0.0461538461538462,0.0615384615384615,0.0769230769230769,0.0923076923076923,
0.107692307692308,0.123076923076923,0.138461538461538,0.153846153846154,
0.169230769230769,0.184615384615385,0.2,0.215384615384615,0.230769230769231,
0.246153846153846,0.261538461538462,0.276923076923077,0.292307692307692,
0.307692307692308,0.323076923076923,0.338461538461538,0.353846153846154,
0.369230769230769,0.384615384615385,0.4,0.415384615384615,0.430769230769231,
0.446153846153846,0.461538461538462,0.476923076923077,0.492307692307692,
0.507692307692308,0.523076923076923,0.538461538461538,0.553846153846154,
0.569230769230769,0.584615384615384,0.6,0.615384615384615,0.63076923076923,
0.646153846153846,0.661538461538461,0.676923076923076,0.692307692307692,
0.707692307692307,0.723076923076922,0.738461538461538,0.753846153846153,
0.769230769230768,0.784615384615384,0.799999999999999,0.815384615384614,
0.83076923076923,0.846153846153845,0.86153846153846,0.876923076923076,0.892307692307691,
0.907692307692306,0.923076923076922,0.938461538461537,0.953846153846152,
0.969230769230768,0.984615384615383,1.),.UNSPECIFIED.)
CURVE()
GEOMETRIC_REPRESENTATION_ITEM()
RATIONAL_B_SPLINE_CURVE((1.,1.,1.,1.,1.,1.,1.,1.,1.,1.,1.,1.,1.,1.,1.,1.,
1.,1.,1.,1.,1.,1.,1.,1.,1.,1.,1.,1.,1.,1.,1.,1.,1.,1.,1.,1.,1.,1.,1.,1.,
1.,1.,1.,1.,1.,1.,1.,1.,1.,1.,1.,1.,1.,1.,1.,1.,1.,1.,1.,1.,1.,1.,1.,1.,
1.,1.,1.,1.,1.,1.))
REPRESENTATION_ITEM('')
);
#238=(
BOUNDED_CURVE()
B_SPLINE_CURVE(5,(#36086,#36087,#36088,#36089,#36090,#36091,#36092,#36093,
#36094,#36095,#36096,#36097,#36098,#36099,#36100,#36101,#36102,#36103,#36104,
#36105,#36106,#36107,#36108,#36109,#36110,#36111,#36112,#36113,#36114,#36115,
#36116,#36117,#36118,#36119,#36120,#36121,#36122,#36123,#36124,#36125,#36126,
#36127,#36128,#36129,#36130,#36131,#36132,#36133,#36134,#36135,#36136,#36137,
#36138,#36139,#36140,#36141,#36142,#36143,#36144,#36145,#36146,#36147,#36148,
#36149,#36150,#36151,#36152,#36153,#36154,#36155),.UNSPECIFIED.,.F.,.F.)
B_SPLINE_CURVE_WITH_KNOTS((6,1,1,1,1,1,1,1,1,1,1,1,1,1,1,1,1,1,1,1,1,1,
1,1,1,1,1,1,1,1,1,1,1,1,1,1,1,1,1,1,1,1,1,1,1,1,1,1,1,1,1,1,1,1,1,1,1,1,
1,1,1,1,1,1,1,6),(0.,0.0153846153846154,0.0307692307692308,0.0461538461538462,
0.0615384615384615,0.0769230769230769,0.0923076923076923,0.107692307692308,
0.123076923076923,0.138461538461538,0.153846153846154,0.169230769230769,
0.184615384615385,0.2,0.215384615384615,0.230769230769231,0.246153846153846,
0.261538461538462,0.276923076923077,0.292307692307692,0.307692307692308,
0.323076923076923,0.338461538461538,0.353846153846154,0.369230769230769,
0.384615384615385,0.4,0.415384615384615,0.430769230769231,0.446153846153846,
0.461538461538462,0.476923076923077,0.492307692307692,0.507692307692308,
0.523076923076923,0.538461538461538,0.553846153846154,0.569230769230769,
0.584615384615384,0.6,0.615384615384615,0.63076923076923,0.646153846153846,
0.661538461538461,0.676923076923076,0.692307692307692,0.707692307692307,
0.723076923076922,0.738461538461538,0.753846153846153,0.769230769230768,
0.784615384615384,0.799999999999999,0.815384615384614,0.83076923076923,
0.846153846153845,0.86153846153846,0.876923076923076,0.892307692307691,
0.907692307692306,0.923076923076922,0.938461538461537,0.953846153846152,
0.969230769230768,0.984615384615383,0.99422815673971),.UNSPECIFIED.)
CURVE()
GEOMETRIC_REPRESENTATION_ITEM()
RATIONAL_B_SPLINE_CURVE((1.,1.,1.,1.,1.,1.,1.,1.,1.,1.,1.,1.,1.,1.,1.,1.,
1.,1.,1.,1.,1.,1.,1.,1.,1.,1.,1.,1.,1.,1.,1.,1.,1.,1.,1.,1.,1.,1.,1.,1.,
1.,1.,1.,1.,1.,1.,1.,1.,1.,1.,1.,1.,1.,1.,1.,1.,1.,1.,1.,1.,1.,1.,1.,1.,
1.,1.,1.,1.,1.,1.))
REPRESENTATION_ITEM('')
);
#239=(
BOUNDED_CURVE()
B_SPLINE_CURVE(5,(#36159,#36160,#36161,#36162,#36163,#36164,#36165,#36166,
#36167,#36168,#36169,#36170,#36171,#36172,#36173,#36174,#36175,#36176,#36177,
#36178,#36179,#36180,#36181,#36182,#36183,#36184,#36185,#36186,#36187,#36188,
#36189,#36190,#36191,#36192,#36193,#36194,#36195,#36196,#36197,#36198,#36199,
#36200,#36201,#36202,#36203,#36204,#36205,#36206,#36207,#36208,#36209,#36210,
#36211,#36212,#36213,#36214,#36215,#36216,#36217,#36218,#36219,#36220,#36221,
#36222,#36223,#36224,#36225,#36226,#36227,#36228),.UNSPECIFIED.,.F.,.F.)
B_SPLINE_CURVE_WITH_KNOTS((6,1,1,1,1,1,1,1,1,1,1,1,1,1,1,1,1,1,1,1,1,1,
1,1,1,1,1,1,1,1,1,1,1,1,1,1,1,1,1,1,1,1,1,1,1,1,1,1,1,1,1,1,1,1,1,1,1,1,
1,1,1,1,1,1,1,6),(0.00577184337448657,0.0153846153846154,0.0307692307692308,
0.0461538461538462,0.0615384615384615,0.0769230769230769,0.0923076923076923,
0.107692307692308,0.123076923076923,0.138461538461538,0.153846153846154,
0.169230769230769,0.184615384615385,0.2,0.215384615384615,0.230769230769231,
0.246153846153846,0.261538461538462,0.276923076923077,0.292307692307692,
0.307692307692308,0.323076923076923,0.338461538461538,0.353846153846154,
0.369230769230769,0.384615384615385,0.4,0.415384615384615,0.430769230769231,
0.446153846153846,0.461538461538462,0.476923076923077,0.492307692307692,
0.507692307692308,0.523076923076923,0.538461538461538,0.553846153846154,
0.569230769230769,0.584615384615384,0.6,0.615384615384615,0.63076923076923,
0.646153846153846,0.661538461538461,0.676923076923076,0.692307692307692,
0.707692307692307,0.723076923076922,0.738461538461538,0.753846153846153,
0.769230769230768,0.784615384615384,0.799999999999999,0.815384615384614,
0.83076923076923,0.846153846153845,0.86153846153846,0.876923076923076,0.892307692307691,
0.907692307692306,0.923076923076922,0.938461538461537,0.953846153846152,
0.969230769230768,0.984615384615383,1.),.UNSPECIFIED.)
CURVE()
GEOMETRIC_REPRESENTATION_ITEM()
RATIONAL_B_SPLINE_CURVE((1.,1.,1.,1.,1.,1.,1.,1.,1.,1.,1.,1.,1.,1.,1.,1.,
1.,1.,1.,1.,1.,1.,1.,1.,1.,1.,1.,1.,1.,1.,1.,1.,1.,1.,1.,1.,1.,1.,1.,1.,
1.,1.,1.,1.,1.,1.,1.,1.,1.,1.,1.,1.,1.,1.,1.,1.,1.,1.,1.,1.,1.,1.,1.,1.,
1.,1.,1.,1.,1.,1.))
REPRESENTATION_ITEM('')
);
#240=(
BOUNDED_CURVE()
B_SPLINE_CURVE(5,(#36232,#36233,#36234,#36235,#36236,#36237,#36238,#36239,
#36240,#36241,#36242,#36243,#36244,#36245,#36246,#36247,#36248,#36249,#36250,
#36251,#36252,#36253,#36254,#36255,#36256,#36257,#36258,#36259,#36260,#36261,
#36262,#36263,#36264,#36265,#36266,#36267,#36268,#36269,#36270,#36271,#36272,
#36273,#36274,#36275,#36276,#36277,#36278,#36279,#36280,#36281,#36282,#36283,
#36284,#36285,#36286,#36287,#36288,#36289,#36290,#36291,#36292,#36293,#36294,
#36295,#36296,#36297,#36298,#36299,#36300,#36301),.UNSPECIFIED.,.F.,.F.)
B_SPLINE_CURVE_WITH_KNOTS((6,1,1,1,1,1,1,1,1,1,1,1,1,1,1,1,1,1,1,1,1,1,
1,1,1,1,1,1,1,1,1,1,1,1,1,1,1,1,1,1,1,1,1,1,1,1,1,1,1,1,1,1,1,1,1,1,1,1,
1,1,1,1,1,1,1,6),(0.,0.0153846153846154,0.0307692307692308,0.0461538461538462,
0.0615384615384615,0.0769230769230769,0.0923076923076923,0.107692307692308,
0.123076923076923,0.138461538461538,0.153846153846154,0.169230769230769,
0.184615384615385,0.2,0.215384615384615,0.230769230769231,0.246153846153846,
0.261538461538462,0.276923076923077,0.292307692307692,0.307692307692308,
0.323076923076923,0.338461538461538,0.353846153846154,0.369230769230769,
0.384615384615385,0.4,0.415384615384615,0.430769230769231,0.446153846153846,
0.461538461538462,0.476923076923077,0.492307692307692,0.507692307692308,
0.523076923076923,0.538461538461538,0.553846153846154,0.569230769230769,
0.584615384615384,0.6,0.615384615384615,0.63076923076923,0.646153846153846,
0.661538461538461,0.676923076923076,0.692307692307692,0.707692307692307,
0.723076923076922,0.738461538461538,0.753846153846153,0.769230769230768,
0.784615384615384,0.799999999999999,0.815384615384614,0.83076923076923,
0.846153846153845,0.86153846153846,0.876923076923076,0.892307692307691,
0.907692307692306,0.923076923076922,0.938461538461537,0.953846153846152,
0.969230769230768,0.984615384615383,0.994228156739709),.UNSPECIFIED.)
CURVE()
GEOMETRIC_REPRESENTATION_ITEM()
RATIONAL_B_SPLINE_CURVE((1.,1.,1.,1.,1.,1.,1.,1.,1.,1.,1.,1.,1.,1.,1.,1.,
1.,1.,1.,1.,1.,1.,1.,1.,1.,1.,1.,1.,1.,1.,1.,1.,1.,1.,1.,1.,1.,1.,1.,1.,
1.,1.,1.,1.,1.,1.,1.,1.,1.,1.,1.,1.,1.,1.,1.,1.,1.,1.,1.,1.,1.,1.,1.,1.,
1.,1.,1.,1.,1.,1.))
REPRESENTATION_ITEM('')
);
#241=(
BOUNDED_CURVE()
B_SPLINE_CURVE(5,(#36305,#36306,#36307,#36308,#36309,#36310,#36311,#36312,
#36313,#36314,#36315,#36316,#36317,#36318,#36319,#36320,#36321,#36322,#36323,
#36324,#36325,#36326,#36327,#36328,#36329,#36330,#36331,#36332,#36333,#36334,
#36335,#36336,#36337,#36338,#36339,#36340,#36341,#36342,#36343,#36344,#36345,
#36346,#36347,#36348,#36349,#36350,#36351,#36352,#36353,#36354,#36355,#36356,
#36357,#36358,#36359,#36360,#36361,#36362,#36363,#36364,#36365,#36366,#36367,
#36368,#36369,#36370,#36371,#36372,#36373,#36374),.UNSPECIFIED.,.F.,.F.)
B_SPLINE_CURVE_WITH_KNOTS((6,1,1,1,1,1,1,1,1,1,1,1,1,1,1,1,1,1,1,1,1,1,
1,1,1,1,1,1,1,1,1,1,1,1,1,1,1,1,1,1,1,1,1,1,1,1,1,1,1,1,1,1,1,1,1,1,1,1,
1,1,1,1,1,1,1,6),(0.00577184337451094,0.0153846153846154,0.0307692307692308,
0.0461538461538462,0.0615384615384615,0.0769230769230769,0.0923076923076923,
0.107692307692308,0.123076923076923,0.138461538461538,0.153846153846154,
0.169230769230769,0.184615384615385,0.2,0.215384615384615,0.230769230769231,
0.246153846153846,0.261538461538462,0.276923076923077,0.292307692307692,
0.307692307692308,0.323076923076923,0.338461538461538,0.353846153846154,
0.369230769230769,0.384615384615385,0.4,0.415384615384615,0.430769230769231,
0.446153846153846,0.461538461538462,0.476923076923077,0.492307692307692,
0.507692307692308,0.523076923076923,0.538461538461538,0.553846153846154,
0.569230769230769,0.584615384615384,0.6,0.615384615384615,0.63076923076923,
0.646153846153846,0.661538461538461,0.676923076923076,0.692307692307692,
0.707692307692307,0.723076923076922,0.738461538461538,0.753846153846153,
0.769230769230768,0.784615384615384,0.799999999999999,0.815384615384614,
0.83076923076923,0.846153846153845,0.86153846153846,0.876923076923076,0.892307692307691,
0.907692307692306,0.923076923076922,0.938461538461537,0.953846153846152,
0.969230769230768,0.984615384615383,1.),.UNSPECIFIED.)
CURVE()
GEOMETRIC_REPRESENTATION_ITEM()
RATIONAL_B_SPLINE_CURVE((1.,1.,1.,1.,1.,1.,1.,1.,1.,1.,1.,1.,1.,1.,1.,1.,
1.,1.,1.,1.,1.,1.,1.,1.,1.,1.,1.,1.,1.,1.,1.,1.,1.,1.,1.,1.,1.,1.,1.,1.,
1.,1.,1.,1.,1.,1.,1.,1.,1.,1.,1.,1.,1.,1.,1.,1.,1.,1.,1.,1.,1.,1.,1.,1.,
1.,1.,1.,1.,1.,1.))
REPRESENTATION_ITEM('')
);
#242=(
BOUNDED_CURVE()
B_SPLINE_CURVE(5,(#36378,#36379,#36380,#36381,#36382,#36383,#36384,#36385,
#36386,#36387,#36388,#36389,#36390,#36391,#36392,#36393,#36394,#36395,#36396,
#36397,#36398,#36399,#36400,#36401,#36402,#36403,#36404,#36405,#36406,#36407,
#36408,#36409,#36410,#36411,#36412,#36413,#36414,#36415,#36416,#36417,#36418,
#36419,#36420,#36421,#36422,#36423,#36424,#36425,#36426,#36427,#36428,#36429,
#36430,#36431,#36432,#36433,#36434,#36435,#36436,#36437,#36438,#36439,#36440,
#36441,#36442,#36443,#36444,#36445,#36446,#36447),.UNSPECIFIED.,.F.,.F.)
B_SPLINE_CURVE_WITH_KNOTS((6,1,1,1,1,1,1,1,1,1,1,1,1,1,1,1,1,1,1,1,1,1,
1,1,1,1,1,1,1,1,1,1,1,1,1,1,1,1,1,1,1,1,1,1,1,1,1,1,1,1,1,1,1,1,1,1,1,1,
1,1,1,1,1,1,1,6),(0.,0.0153846153846154,0.0307692307692308,0.0461538461538462,
0.0615384615384615,0.0769230769230769,0.0923076923076923,0.107692307692308,
0.123076923076923,0.138461538461538,0.153846153846154,0.169230769230769,
0.184615384615385,0.2,0.215384615384615,0.230769230769231,0.246153846153846,
0.261538461538462,0.276923076923077,0.292307692307692,0.307692307692308,
0.323076923076923,0.338461538461538,0.353846153846154,0.369230769230769,
0.384615384615385,0.4,0.415384615384615,0.430769230769231,0.446153846153846,
0.461538461538462,0.476923076923077,0.492307692307692,0.507692307692308,
0.523076923076923,0.538461538461538,0.553846153846154,0.569230769230769,
0.584615384615384,0.6,0.615384615384615,0.63076923076923,0.646153846153846,
0.661538461538461,0.676923076923076,0.692307692307692,0.707692307692307,
0.723076923076922,0.738461538461538,0.753846153846153,0.769230769230768,
0.784615384615384,0.799999999999999,0.815384615384614,0.83076923076923,
0.846153846153845,0.86153846153846,0.876923076923076,0.892307692307691,
0.907692307692306,0.923076923076922,0.938461538461537,0.953846153846152,
0.969230769230768,0.984615384615383,0.994228156739701),.UNSPECIFIED.)
CURVE()
GEOMETRIC_REPRESENTATION_ITEM()
RATIONAL_B_SPLINE_CURVE((1.,1.,1.,1.,1.,1.,1.,1.,1.,1.,1.,1.,1.,1.,1.,1.,
1.,1.,1.,1.,1.,1.,1.,1.,1.,1.,1.,1.,1.,1.,1.,1.,1.,1.,1.,1.,1.,1.,1.,1.,
1.,1.,1.,1.,1.,1.,1.,1.,1.,1.,1.,1.,1.,1.,1.,1.,1.,1.,1.,1.,1.,1.,1.,1.,
1.,1.,1.,1.,1.,1.))
REPRESENTATION_ITEM('')
);
#243=(
BOUNDED_CURVE()
B_SPLINE_CURVE(5,(#36451,#36452,#36453,#36454,#36455,#36456,#36457,#36458,
#36459,#36460,#36461,#36462,#36463,#36464,#36465,#36466,#36467,#36468,#36469,
#36470,#36471,#36472,#36473,#36474,#36475,#36476,#36477,#36478,#36479,#36480,
#36481,#36482,#36483,#36484,#36485,#36486,#36487,#36488,#36489,#36490,#36491,
#36492,#36493,#36494,#36495,#36496,#36497,#36498,#36499,#36500,#36501,#36502,
#36503,#36504,#36505,#36506,#36507,#36508,#36509,#36510,#36511,#36512,#36513,
#36514,#36515,#36516,#36517,#36518,#36519,#36520),.UNSPECIFIED.,.F.,.F.)
B_SPLINE_CURVE_WITH_KNOTS((6,1,1,1,1,1,1,1,1,1,1,1,1,1,1,1,1,1,1,1,1,1,
1,1,1,1,1,1,1,1,1,1,1,1,1,1,1,1,1,1,1,1,1,1,1,1,1,1,1,1,1,1,1,1,1,1,1,1,
1,1,1,1,1,1,1,6),(0.0057718433745102,0.0153846153846154,0.0307692307692308,
0.0461538461538462,0.0615384615384615,0.0769230769230769,0.0923076923076923,
0.107692307692308,0.123076923076923,0.138461538461538,0.153846153846154,
0.169230769230769,0.184615384615385,0.2,0.215384615384615,0.230769230769231,
0.246153846153846,0.261538461538462,0.276923076923077,0.292307692307692,
0.307692307692308,0.323076923076923,0.338461538461538,0.353846153846154,
0.369230769230769,0.384615384615385,0.4,0.415384615384615,0.430769230769231,
0.446153846153846,0.461538461538462,0.476923076923077,0.492307692307692,
0.507692307692308,0.523076923076923,0.538461538461538,0.553846153846154,
0.569230769230769,0.584615384615384,0.6,0.615384615384615,0.63076923076923,
0.646153846153846,0.661538461538461,0.676923076923076,0.692307692307692,
0.707692307692307,0.723076923076922,0.738461538461538,0.753846153846153,
0.769230769230768,0.784615384615384,0.799999999999999,0.815384615384614,
0.83076923076923,0.846153846153845,0.86153846153846,0.876923076923076,0.892307692307691,
0.907692307692306,0.923076923076922,0.938461538461537,0.953846153846152,
0.969230769230768,0.984615384615383,1.),.UNSPECIFIED.)
CURVE()
GEOMETRIC_REPRESENTATION_ITEM()
RATIONAL_B_SPLINE_CURVE((1.,1.,1.,1.,1.,1.,1.,1.,1.,1.,1.,1.,1.,1.,1.,1.,
1.,1.,1.,1.,1.,1.,1.,1.,1.,1.,1.,1.,1.,1.,1.,1.,1.,1.,1.,1.,1.,1.,1.,1.,
1.,1.,1.,1.,1.,1.,1.,1.,1.,1.,1.,1.,1.,1.,1.,1.,1.,1.,1.,1.,1.,1.,1.,1.,
1.,1.,1.,1.,1.,1.))
REPRESENTATION_ITEM('')
);
#244=(
BOUNDED_CURVE()
B_SPLINE_CURVE(5,(#36524,#36525,#36526,#36527,#36528,#36529,#36530,#36531,
#36532,#36533,#36534,#36535,#36536,#36537,#36538,#36539,#36540,#36541,#36542,
#36543,#36544,#36545,#36546,#36547,#36548,#36549,#36550,#36551,#36552,#36553,
#36554,#36555,#36556,#36557,#36558,#36559,#36560,#36561,#36562,#36563,#36564,
#36565,#36566,#36567,#36568,#36569,#36570,#36571,#36572,#36573,#36574,#36575,
#36576,#36577,#36578,#36579,#36580,#36581,#36582,#36583,#36584,#36585,#36586,
#36587,#36588,#36589,#36590,#36591,#36592,#36593),.UNSPECIFIED.,.F.,.F.)
B_SPLINE_CURVE_WITH_KNOTS((6,1,1,1,1,1,1,1,1,1,1,1,1,1,1,1,1,1,1,1,1,1,
1,1,1,1,1,1,1,1,1,1,1,1,1,1,1,1,1,1,1,1,1,1,1,1,1,1,1,1,1,1,1,1,1,1,1,1,
1,1,1,1,1,1,1,6),(0.,0.0153846153846154,0.0307692307692308,0.0461538461538462,
0.0615384615384615,0.0769230769230769,0.0923076923076923,0.107692307692308,
0.123076923076923,0.138461538461538,0.153846153846154,0.169230769230769,
0.184615384615385,0.2,0.215384615384615,0.230769230769231,0.246153846153846,
0.261538461538462,0.276923076923077,0.292307692307692,0.307692307692308,
0.323076923076923,0.338461538461538,0.353846153846154,0.369230769230769,
0.384615384615385,0.4,0.415384615384615,0.430769230769231,0.446153846153846,
0.461538461538462,0.476923076923077,0.492307692307692,0.507692307692308,
0.523076923076923,0.538461538461538,0.553846153846154,0.569230769230769,
0.584615384615384,0.6,0.615384615384615,0.63076923076923,0.646153846153846,
0.661538461538461,0.676923076923076,0.692307692307692,0.707692307692307,
0.723076923076922,0.738461538461538,0.753846153846153,0.769230769230768,
0.784615384615384,0.799999999999999,0.815384615384614,0.83076923076923,
0.846153846153845,0.86153846153846,0.876923076923076,0.892307692307691,
0.907692307692306,0.923076923076922,0.938461538461537,0.953846153846152,
0.969230769230768,0.984615384615383,0.994228156739694),.UNSPECIFIED.)
CURVE()
GEOMETRIC_REPRESENTATION_ITEM()
RATIONAL_B_SPLINE_CURVE((1.,1.,1.,1.,1.,1.,1.,1.,1.,1.,1.,1.,1.,1.,1.,1.,
1.,1.,1.,1.,1.,1.,1.,1.,1.,1.,1.,1.,1.,1.,1.,1.,1.,1.,1.,1.,1.,1.,1.,1.,
1.,1.,1.,1.,1.,1.,1.,1.,1.,1.,1.,1.,1.,1.,1.,1.,1.,1.,1.,1.,1.,1.,1.,1.,
1.,1.,1.,1.,1.,1.))
REPRESENTATION_ITEM('')
);
#245=(
BOUNDED_CURVE()
B_SPLINE_CURVE(5,(#36597,#36598,#36599,#36600,#36601,#36602,#36603,#36604,
#36605,#36606,#36607,#36608,#36609,#36610,#36611,#36612,#36613,#36614,#36615,
#36616,#36617,#36618,#36619,#36620,#36621,#36622,#36623,#36624,#36625,#36626,
#36627,#36628,#36629,#36630,#36631,#36632,#36633,#36634,#36635,#36636,#36637,
#36638,#36639,#36640,#36641,#36642,#36643,#36644,#36645,#36646,#36647,#36648,
#36649,#36650,#36651,#36652,#36653,#36654,#36655,#36656,#36657,#36658,#36659,
#36660,#36661,#36662,#36663,#36664,#36665,#36666),.UNSPECIFIED.,.F.,.F.)
B_SPLINE_CURVE_WITH_KNOTS((6,1,1,1,1,1,1,1,1,1,1,1,1,1,1,1,1,1,1,1,1,1,
1,1,1,1,1,1,1,1,1,1,1,1,1,1,1,1,1,1,1,1,1,1,1,1,1,1,1,1,1,1,1,1,1,1,1,1,
1,1,1,1,1,1,1,6),(0.00577184337452044,0.0153846153846154,0.0307692307692308,
0.0461538461538462,0.0615384615384615,0.0769230769230769,0.0923076923076923,
0.107692307692308,0.123076923076923,0.138461538461538,0.153846153846154,
0.169230769230769,0.184615384615385,0.2,0.215384615384615,0.230769230769231,
0.246153846153846,0.261538461538462,0.276923076923077,0.292307692307692,
0.307692307692308,0.323076923076923,0.338461538461538,0.353846153846154,
0.369230769230769,0.384615384615385,0.4,0.415384615384615,0.430769230769231,
0.446153846153846,0.461538461538462,0.476923076923077,0.492307692307692,
0.507692307692308,0.523076923076923,0.538461538461538,0.553846153846154,
0.569230769230769,0.584615384615384,0.6,0.615384615384615,0.63076923076923,
0.646153846153846,0.661538461538461,0.676923076923076,0.692307692307692,
0.707692307692307,0.723076923076922,0.738461538461538,0.753846153846153,
0.769230769230768,0.784615384615384,0.799999999999999,0.815384615384614,
0.83076923076923,0.846153846153845,0.86153846153846,0.876923076923076,0.892307692307691,
0.907692307692306,0.923076923076922,0.938461538461537,0.953846153846152,
0.969230769230768,0.984615384615383,1.),.UNSPECIFIED.)
CURVE()
GEOMETRIC_REPRESENTATION_ITEM()
RATIONAL_B_SPLINE_CURVE((1.,1.,1.,1.,1.,1.,1.,1.,1.,1.,1.,1.,1.,1.,1.,1.,
1.,1.,1.,1.,1.,1.,1.,1.,1.,1.,1.,1.,1.,1.,1.,1.,1.,1.,1.,1.,1.,1.,1.,1.,
1.,1.,1.,1.,1.,1.,1.,1.,1.,1.,1.,1.,1.,1.,1.,1.,1.,1.,1.,1.,1.,1.,1.,1.,
1.,1.,1.,1.,1.,1.))
REPRESENTATION_ITEM('')
);
#246=(
BOUNDED_CURVE()
B_SPLINE_CURVE(5,(#36670,#36671,#36672,#36673,#36674,#36675,#36676,#36677,
#36678,#36679,#36680,#36681,#36682,#36683,#36684,#36685,#36686,#36687,#36688,
#36689,#36690,#36691,#36692,#36693,#36694,#36695,#36696,#36697,#36698,#36699,
#36700,#36701,#36702,#36703,#36704,#36705,#36706,#36707,#36708,#36709,#36710,
#36711,#36712,#36713,#36714,#36715,#36716,#36717,#36718,#36719,#36720,#36721,
#36722,#36723,#36724,#36725,#36726,#36727,#36728,#36729,#36730,#36731,#36732,
#36733,#36734,#36735,#36736,#36737,#36738,#36739),.UNSPECIFIED.,.F.,.F.)
B_SPLINE_CURVE_WITH_KNOTS((6,1,1,1,1,1,1,1,1,1,1,1,1,1,1,1,1,1,1,1,1,1,
1,1,1,1,1,1,1,1,1,1,1,1,1,1,1,1,1,1,1,1,1,1,1,1,1,1,1,1,1,1,1,1,1,1,1,1,
1,1,1,1,1,1,1,6),(0.,0.0153846153846154,0.0307692307692308,0.0461538461538462,
0.0615384615384615,0.0769230769230769,0.0923076923076923,0.107692307692308,
0.123076923076923,0.138461538461538,0.153846153846154,0.169230769230769,
0.184615384615385,0.2,0.215384615384615,0.230769230769231,0.246153846153846,
0.261538461538462,0.276923076923077,0.292307692307692,0.307692307692308,
0.323076923076923,0.338461538461538,0.353846153846154,0.369230769230769,
0.384615384615385,0.4,0.415384615384615,0.430769230769231,0.446153846153846,
0.461538461538462,0.476923076923077,0.492307692307692,0.507692307692308,
0.523076923076923,0.538461538461538,0.553846153846154,0.569230769230769,
0.584615384615384,0.6,0.615384615384615,0.63076923076923,0.646153846153846,
0.661538461538461,0.676923076923076,0.692307692307692,0.707692307692307,
0.723076923076922,0.738461538461538,0.753846153846153,0.769230769230768,
0.784615384615384,0.799999999999999,0.815384615384614,0.83076923076923,
0.846153846153845,0.86153846153846,0.876923076923076,0.892307692307691,
0.907692307692306,0.923076923076922,0.938461538461537,0.953846153846152,
0.969230769230768,0.984615384615383,0.994228156739698),.UNSPECIFIED.)
CURVE()
GEOMETRIC_REPRESENTATION_ITEM()
RATIONAL_B_SPLINE_CURVE((1.,1.,1.,1.,1.,1.,1.,1.,1.,1.,1.,1.,1.,1.,1.,1.,
1.,1.,1.,1.,1.,1.,1.,1.,1.,1.,1.,1.,1.,1.,1.,1.,1.,1.,1.,1.,1.,1.,1.,1.,
1.,1.,1.,1.,1.,1.,1.,1.,1.,1.,1.,1.,1.,1.,1.,1.,1.,1.,1.,1.,1.,1.,1.,1.,
1.,1.,1.,1.,1.,1.))
REPRESENTATION_ITEM('')
);
#247=(
BOUNDED_CURVE()
B_SPLINE_CURVE(5,(#36743,#36744,#36745,#36746,#36747,#36748,#36749,#36750,
#36751,#36752,#36753,#36754,#36755,#36756,#36757,#36758,#36759,#36760,#36761,
#36762,#36763,#36764,#36765,#36766,#36767,#36768,#36769,#36770,#36771,#36772,
#36773,#36774,#36775,#36776,#36777,#36778,#36779,#36780,#36781,#36782,#36783,
#36784,#36785,#36786,#36787,#36788,#36789,#36790,#36791,#36792,#36793,#36794,
#36795,#36796,#36797,#36798,#36799,#36800,#36801,#36802,#36803,#36804,#36805,
#36806,#36807,#36808,#36809,#36810,#36811,#36812),.UNSPECIFIED.,.F.,.F.)
B_SPLINE_CURVE_WITH_KNOTS((6,1,1,1,1,1,1,1,1,1,1,1,1,1,1,1,1,1,1,1,1,1,
1,1,1,1,1,1,1,1,1,1,1,1,1,1,1,1,1,1,1,1,1,1,1,1,1,1,1,1,1,1,1,1,1,1,1,1,
1,1,1,1,1,1,1,6),(0.00577184337451607,0.0153846153846154,0.0307692307692308,
0.0461538461538462,0.0615384615384615,0.0769230769230769,0.0923076923076923,
0.107692307692308,0.123076923076923,0.138461538461538,0.153846153846154,
0.169230769230769,0.184615384615385,0.2,0.215384615384615,0.230769230769231,
0.246153846153846,0.261538461538462,0.276923076923077,0.292307692307692,
0.307692307692308,0.323076923076923,0.338461538461538,0.353846153846154,
0.369230769230769,0.384615384615385,0.4,0.415384615384615,0.430769230769231,
0.446153846153846,0.461538461538462,0.476923076923077,0.492307692307692,
0.507692307692308,0.523076923076923,0.538461538461538,0.553846153846154,
0.569230769230769,0.584615384615384,0.6,0.615384615384615,0.63076923076923,
0.646153846153846,0.661538461538461,0.676923076923076,0.692307692307692,
0.707692307692307,0.723076923076922,0.738461538461538,0.753846153846153,
0.769230769230768,0.784615384615384,0.799999999999999,0.815384615384614,
0.83076923076923,0.846153846153845,0.86153846153846,0.876923076923076,0.892307692307691,
0.907692307692306,0.923076923076922,0.938461538461537,0.953846153846152,
0.969230769230768,0.984615384615383,1.),.UNSPECIFIED.)
CURVE()
GEOMETRIC_REPRESENTATION_ITEM()
RATIONAL_B_SPLINE_CURVE((1.,1.,1.,1.,1.,1.,1.,1.,1.,1.,1.,1.,1.,1.,1.,1.,
1.,1.,1.,1.,1.,1.,1.,1.,1.,1.,1.,1.,1.,1.,1.,1.,1.,1.,1.,1.,1.,1.,1.,1.,
1.,1.,1.,1.,1.,1.,1.,1.,1.,1.,1.,1.,1.,1.,1.,1.,1.,1.,1.,1.,1.,1.,1.,1.,
1.,1.,1.,1.,1.,1.))
REPRESENTATION_ITEM('')
);
#248=(
BOUNDED_CURVE()
B_SPLINE_CURVE(5,(#36816,#36817,#36818,#36819,#36820,#36821,#36822,#36823,
#36824,#36825,#36826,#36827,#36828,#36829,#36830,#36831,#36832,#36833,#36834,
#36835,#36836,#36837,#36838,#36839,#36840,#36841,#36842,#36843,#36844,#36845,
#36846,#36847,#36848,#36849,#36850,#36851,#36852,#36853,#36854,#36855,#36856,
#36857,#36858,#36859,#36860,#36861,#36862,#36863,#36864,#36865,#36866,#36867,
#36868,#36869,#36870,#36871,#36872,#36873,#36874,#36875,#36876,#36877,#36878,
#36879,#36880,#36881,#36882,#36883,#36884,#36885),.UNSPECIFIED.,.F.,.F.)
B_SPLINE_CURVE_WITH_KNOTS((6,1,1,1,1,1,1,1,1,1,1,1,1,1,1,1,1,1,1,1,1,1,
1,1,1,1,1,1,1,1,1,1,1,1,1,1,1,1,1,1,1,1,1,1,1,1,1,1,1,1,1,1,1,1,1,1,1,1,
1,1,1,1,1,1,1,6),(0.,0.0153846153846154,0.0307692307692308,0.0461538461538462,
0.0615384615384615,0.0769230769230769,0.0923076923076923,0.107692307692308,
0.123076923076923,0.138461538461538,0.153846153846154,0.169230769230769,
0.184615384615385,0.2,0.215384615384615,0.230769230769231,0.246153846153846,
0.261538461538462,0.276923076923077,0.292307692307692,0.307692307692308,
0.323076923076923,0.338461538461538,0.353846153846154,0.369230769230769,
0.384615384615385,0.4,0.415384615384615,0.430769230769231,0.446153846153846,
0.461538461538462,0.476923076923077,0.492307692307692,0.507692307692308,
0.523076923076923,0.538461538461538,0.553846153846154,0.569230769230769,
0.584615384615384,0.6,0.615384615384615,0.63076923076923,0.646153846153846,
0.661538461538461,0.676923076923076,0.692307692307692,0.707692307692307,
0.723076923076922,0.738461538461538,0.753846153846153,0.769230769230768,
0.784615384615384,0.799999999999999,0.815384615384614,0.83076923076923,
0.846153846153845,0.86153846153846,0.876923076923076,0.892307692307691,
0.907692307692306,0.923076923076922,0.938461538461537,0.953846153846152,
0.969230769230768,0.984615384615383,0.994228156739704),.UNSPECIFIED.)
CURVE()
GEOMETRIC_REPRESENTATION_ITEM()
RATIONAL_B_SPLINE_CURVE((1.,1.,1.,1.,1.,1.,1.,1.,1.,1.,1.,1.,1.,1.,1.,1.,
1.,1.,1.,1.,1.,1.,1.,1.,1.,1.,1.,1.,1.,1.,1.,1.,1.,1.,1.,1.,1.,1.,1.,1.,
1.,1.,1.,1.,1.,1.,1.,1.,1.,1.,1.,1.,1.,1.,1.,1.,1.,1.,1.,1.,1.,1.,1.,1.,
1.,1.,1.,1.,1.,1.))
REPRESENTATION_ITEM('')
);
#249=(
BOUNDED_CURVE()
B_SPLINE_CURVE(5,(#36889,#36890,#36891,#36892,#36893,#36894,#36895,#36896,
#36897,#36898,#36899,#36900,#36901,#36902,#36903,#36904,#36905,#36906,#36907,
#36908,#36909,#36910,#36911,#36912,#36913,#36914,#36915,#36916,#36917,#36918,
#36919,#36920,#36921,#36922,#36923,#36924,#36925,#36926,#36927,#36928,#36929,
#36930,#36931,#36932,#36933,#36934,#36935,#36936,#36937,#36938,#36939,#36940,
#36941,#36942,#36943,#36944,#36945,#36946,#36947,#36948,#36949,#36950,#36951,
#36952,#36953,#36954,#36955,#36956,#36957,#36958),.UNSPECIFIED.,.F.,.F.)
B_SPLINE_CURVE_WITH_KNOTS((6,1,1,1,1,1,1,1,1,1,1,1,1,1,1,1,1,1,1,1,1,1,
1,1,1,1,1,1,1,1,1,1,1,1,1,1,1,1,1,1,1,1,1,1,1,1,1,1,1,1,1,1,1,1,1,1,1,1,
1,1,1,1,1,1,1,6),(0.00577184337449682,0.0153846153846154,0.0307692307692308,
0.0461538461538462,0.0615384615384615,0.0769230769230769,0.0923076923076923,
0.107692307692308,0.123076923076923,0.138461538461538,0.153846153846154,
0.169230769230769,0.184615384615385,0.2,0.215384615384615,0.230769230769231,
0.246153846153846,0.261538461538462,0.276923076923077,0.292307692307692,
0.307692307692308,0.323076923076923,0.338461538461538,0.353846153846154,
0.369230769230769,0.384615384615385,0.4,0.415384615384615,0.430769230769231,
0.446153846153846,0.461538461538462,0.476923076923077,0.492307692307692,
0.507692307692308,0.523076923076923,0.538461538461538,0.553846153846154,
0.569230769230769,0.584615384615384,0.6,0.615384615384615,0.63076923076923,
0.646153846153846,0.661538461538461,0.676923076923076,0.692307692307692,
0.707692307692307,0.723076923076922,0.738461538461538,0.753846153846153,
0.769230769230768,0.784615384615384,0.799999999999999,0.815384615384614,
0.83076923076923,0.846153846153845,0.86153846153846,0.876923076923076,0.892307692307691,
0.907692307692306,0.923076923076922,0.938461538461537,0.953846153846152,
0.969230769230768,0.984615384615383,1.),.UNSPECIFIED.)
CURVE()
GEOMETRIC_REPRESENTATION_ITEM()
RATIONAL_B_SPLINE_CURVE((1.,1.,1.,1.,1.,1.,1.,1.,1.,1.,1.,1.,1.,1.,1.,1.,
1.,1.,1.,1.,1.,1.,1.,1.,1.,1.,1.,1.,1.,1.,1.,1.,1.,1.,1.,1.,1.,1.,1.,1.,
1.,1.,1.,1.,1.,1.,1.,1.,1.,1.,1.,1.,1.,1.,1.,1.,1.,1.,1.,1.,1.,1.,1.,1.,
1.,1.,1.,1.,1.,1.))
REPRESENTATION_ITEM('')
);
#250=(
BOUNDED_CURVE()
B_SPLINE_CURVE(5,(#36962,#36963,#36964,#36965,#36966,#36967,#36968,#36969,
#36970,#36971,#36972,#36973,#36974,#36975,#36976,#36977,#36978,#36979,#36980,
#36981,#36982,#36983,#36984,#36985,#36986,#36987,#36988,#36989,#36990,#36991,
#36992,#36993,#36994,#36995,#36996,#36997,#36998,#36999,#37000,#37001,#37002,
#37003,#37004,#37005,#37006,#37007,#37008,#37009,#37010,#37011,#37012,#37013,
#37014,#37015,#37016,#37017,#37018,#37019,#37020,#37021,#37022,#37023,#37024,
#37025,#37026,#37027,#37028,#37029,#37030,#37031),.UNSPECIFIED.,.F.,.F.)
B_SPLINE_CURVE_WITH_KNOTS((6,1,1,1,1,1,1,1,1,1,1,1,1,1,1,1,1,1,1,1,1,1,
1,1,1,1,1,1,1,1,1,1,1,1,1,1,1,1,1,1,1,1,1,1,1,1,1,1,1,1,1,1,1,1,1,1,1,1,
1,1,1,1,1,1,1,6),(0.,0.0153846153846154,0.0307692307692308,0.0461538461538462,
0.0615384615384615,0.0769230769230769,0.0923076923076923,0.107692307692308,
0.123076923076923,0.138461538461538,0.153846153846154,0.169230769230769,
0.184615384615385,0.2,0.215384615384615,0.230769230769231,0.246153846153846,
0.261538461538462,0.276923076923077,0.292307692307692,0.307692307692308,
0.323076923076923,0.338461538461538,0.353846153846154,0.369230769230769,
0.384615384615385,0.4,0.415384615384615,0.430769230769231,0.446153846153846,
0.461538461538462,0.476923076923077,0.492307692307692,0.507692307692308,
0.523076923076923,0.538461538461538,0.553846153846154,0.569230769230769,
0.584615384615384,0.6,0.615384615384615,0.63076923076923,0.646153846153846,
0.661538461538461,0.676923076923076,0.692307692307692,0.707692307692307,
0.723076923076922,0.738461538461538,0.753846153846153,0.769230769230768,
0.784615384615384,0.799999999999999,0.815384615384614,0.83076923076923,
0.846153846153845,0.86153846153846,0.876923076923076,0.892307692307691,
0.907692307692306,0.923076923076922,0.938461538461537,0.953846153846152,
0.969230769230768,0.984615384615383,0.994228156739711),.UNSPECIFIED.)
CURVE()
GEOMETRIC_REPRESENTATION_ITEM()
RATIONAL_B_SPLINE_CURVE((1.,1.,1.,1.,1.,1.,1.,1.,1.,1.,1.,1.,1.,1.,1.,1.,
1.,1.,1.,1.,1.,1.,1.,1.,1.,1.,1.,1.,1.,1.,1.,1.,1.,1.,1.,1.,1.,1.,1.,1.,
1.,1.,1.,1.,1.,1.,1.,1.,1.,1.,1.,1.,1.,1.,1.,1.,1.,1.,1.,1.,1.,1.,1.,1.,
1.,1.,1.,1.,1.,1.))
REPRESENTATION_ITEM('')
);
#251=(
BOUNDED_CURVE()
B_SPLINE_CURVE(5,(#37035,#37036,#37037,#37038,#37039,#37040,#37041,#37042,
#37043,#37044,#37045,#37046,#37047,#37048,#37049,#37050,#37051,#37052,#37053,
#37054,#37055,#37056,#37057,#37058,#37059,#37060,#37061,#37062,#37063,#37064,
#37065,#37066,#37067,#37068,#37069,#37070,#37071,#37072,#37073,#37074,#37075,
#37076,#37077,#37078,#37079,#37080,#37081,#37082,#37083,#37084,#37085,#37086,
#37087,#37088,#37089,#37090,#37091,#37092,#37093,#37094,#37095,#37096,#37097,
#37098,#37099,#37100,#37101,#37102,#37103,#37104),.UNSPECIFIED.,.F.,.F.)
B_SPLINE_CURVE_WITH_KNOTS((6,1,1,1,1,1,1,1,1,1,1,1,1,1,1,1,1,1,1,1,1,1,
1,1,1,1,1,1,1,1,1,1,1,1,1,1,1,1,1,1,1,1,1,1,1,1,1,1,1,1,1,1,1,1,1,1,1,1,
1,1,1,1,1,1,1,6),(0.00577184337450313,0.0153846153846154,0.0307692307692308,
0.0461538461538462,0.0615384615384615,0.0769230769230769,0.0923076923076923,
0.107692307692308,0.123076923076923,0.138461538461538,0.153846153846154,
0.169230769230769,0.184615384615385,0.2,0.215384615384615,0.230769230769231,
0.246153846153846,0.261538461538462,0.276923076923077,0.292307692307692,
0.307692307692308,0.323076923076923,0.338461538461538,0.353846153846154,
0.369230769230769,0.384615384615385,0.4,0.415384615384615,0.430769230769231,
0.446153846153846,0.461538461538462,0.476923076923077,0.492307692307692,
0.507692307692308,0.523076923076923,0.538461538461538,0.553846153846154,
0.569230769230769,0.584615384615384,0.6,0.615384615384615,0.63076923076923,
0.646153846153846,0.661538461538461,0.676923076923076,0.692307692307692,
0.707692307692307,0.723076923076922,0.738461538461538,0.753846153846153,
0.769230769230768,0.784615384615384,0.799999999999999,0.815384615384614,
0.83076923076923,0.846153846153845,0.86153846153846,0.876923076923076,0.892307692307691,
0.907692307692306,0.923076923076922,0.938461538461537,0.953846153846152,
0.969230769230768,0.984615384615383,1.),.UNSPECIFIED.)
CURVE()
GEOMETRIC_REPRESENTATION_ITEM()
RATIONAL_B_SPLINE_CURVE((1.,1.,1.,1.,1.,1.,1.,1.,1.,1.,1.,1.,1.,1.,1.,1.,
1.,1.,1.,1.,1.,1.,1.,1.,1.,1.,1.,1.,1.,1.,1.,1.,1.,1.,1.,1.,1.,1.,1.,1.,
1.,1.,1.,1.,1.,1.,1.,1.,1.,1.,1.,1.,1.,1.,1.,1.,1.,1.,1.,1.,1.,1.,1.,1.,
1.,1.,1.,1.,1.,1.))
REPRESENTATION_ITEM('')
);
#252=(
BOUNDED_CURVE()
B_SPLINE_CURVE(5,(#37108,#37109,#37110,#37111,#37112,#37113,#37114,#37115,
#37116,#37117,#37118,#37119,#37120,#37121,#37122,#37123,#37124,#37125,#37126,
#37127,#37128,#37129,#37130,#37131,#37132,#37133,#37134,#37135,#37136,#37137,
#37138,#37139,#37140,#37141,#37142,#37143,#37144,#37145,#37146,#37147,#37148,
#37149,#37150,#37151,#37152,#37153,#37154,#37155,#37156,#37157,#37158,#37159,
#37160,#37161,#37162,#37163,#37164,#37165,#37166,#37167,#37168,#37169,#37170,
#37171,#37172,#37173,#37174,#37175,#37176,#37177),.UNSPECIFIED.,.F.,.F.)
B_SPLINE_CURVE_WITH_KNOTS((6,1,1,1,1,1,1,1,1,1,1,1,1,1,1,1,1,1,1,1,1,1,
1,1,1,1,1,1,1,1,1,1,1,1,1,1,1,1,1,1,1,1,1,1,1,1,1,1,1,1,1,1,1,1,1,1,1,1,
1,1,1,1,1,1,1,6),(0.,0.0153846153846154,0.0307692307692308,0.0461538461538462,
0.0615384615384615,0.0769230769230769,0.0923076923076923,0.107692307692308,
0.123076923076923,0.138461538461538,0.153846153846154,0.169230769230769,
0.184615384615385,0.2,0.215384615384615,0.230769230769231,0.246153846153846,
0.261538461538462,0.276923076923077,0.292307692307692,0.307692307692308,
0.323076923076923,0.338461538461538,0.353846153846154,0.369230769230769,
0.384615384615385,0.4,0.415384615384615,0.430769230769231,0.446153846153846,
0.461538461538462,0.476923076923077,0.492307692307692,0.507692307692308,
0.523076923076923,0.538461538461538,0.553846153846154,0.569230769230769,
0.584615384615384,0.6,0.615384615384615,0.63076923076923,0.646153846153846,
0.661538461538461,0.676923076923076,0.692307692307692,0.707692307692307,
0.723076923076922,0.738461538461538,0.753846153846153,0.769230769230768,
0.784615384615384,0.799999999999999,0.815384615384614,0.83076923076923,
0.846153846153845,0.86153846153846,0.876923076923076,0.892307692307691,
0.907692307692306,0.923076923076922,0.938461538461537,0.953846153846152,
0.969230769230768,0.984615384615383,0.9942281567397),.UNSPECIFIED.)
CURVE()
GEOMETRIC_REPRESENTATION_ITEM()
RATIONAL_B_SPLINE_CURVE((1.,1.,1.,1.,1.,1.,1.,1.,1.,1.,1.,1.,1.,1.,1.,1.,
1.,1.,1.,1.,1.,1.,1.,1.,1.,1.,1.,1.,1.,1.,1.,1.,1.,1.,1.,1.,1.,1.,1.,1.,
1.,1.,1.,1.,1.,1.,1.,1.,1.,1.,1.,1.,1.,1.,1.,1.,1.,1.,1.,1.,1.,1.,1.,1.,
1.,1.,1.,1.,1.,1.))
REPRESENTATION_ITEM('')
);
#253=(
BOUNDED_CURVE()
B_SPLINE_CURVE(5,(#37181,#37182,#37183,#37184,#37185,#37186,#37187,#37188,
#37189,#37190,#37191,#37192,#37193,#37194,#37195,#37196,#37197,#37198,#37199,
#37200,#37201,#37202,#37203,#37204,#37205,#37206,#37207,#37208,#37209,#37210,
#37211,#37212,#37213,#37214,#37215,#37216,#37217,#37218,#37219,#37220,#37221,
#37222,#37223,#37224,#37225,#37226,#37227,#37228,#37229,#37230,#37231,#37232,
#37233,#37234,#37235,#37236,#37237,#37238,#37239,#37240,#37241,#37242,#37243,
#37244,#37245,#37246,#37247,#37248,#37249,#37250),.UNSPECIFIED.,.F.,.F.)
B_SPLINE_CURVE_WITH_KNOTS((6,1,1,1,1,1,1,1,1,1,1,1,1,1,1,1,1,1,1,1,1,1,
1,1,1,1,1,1,1,1,1,1,1,1,1,1,1,1,1,1,1,1,1,1,1,1,1,1,1,1,1,1,1,1,1,1,1,1,
1,1,1,1,1,1,1,6),(0.00577184337452087,0.0153846153846154,0.0307692307692308,
0.0461538461538462,0.0615384615384615,0.0769230769230769,0.0923076923076923,
0.107692307692308,0.123076923076923,0.138461538461538,0.153846153846154,
0.169230769230769,0.184615384615385,0.2,0.215384615384615,0.230769230769231,
0.246153846153846,0.261538461538462,0.276923076923077,0.292307692307692,
0.307692307692308,0.323076923076923,0.338461538461538,0.353846153846154,
0.369230769230769,0.384615384615385,0.4,0.415384615384615,0.430769230769231,
0.446153846153846,0.461538461538462,0.476923076923077,0.492307692307692,
0.507692307692308,0.523076923076923,0.538461538461538,0.553846153846154,
0.569230769230769,0.584615384615384,0.6,0.615384615384615,0.63076923076923,
0.646153846153846,0.661538461538461,0.676923076923076,0.692307692307692,
0.707692307692307,0.723076923076922,0.738461538461538,0.753846153846153,
0.769230769230768,0.784615384615384,0.799999999999999,0.815384615384614,
0.83076923076923,0.846153846153845,0.86153846153846,0.876923076923076,0.892307692307691,
0.907692307692306,0.923076923076922,0.938461538461537,0.953846153846152,
0.969230769230768,0.984615384615383,1.),.UNSPECIFIED.)
CURVE()
GEOMETRIC_REPRESENTATION_ITEM()
RATIONAL_B_SPLINE_CURVE((1.,1.,1.,1.,1.,1.,1.,1.,1.,1.,1.,1.,1.,1.,1.,1.,
1.,1.,1.,1.,1.,1.,1.,1.,1.,1.,1.,1.,1.,1.,1.,1.,1.,1.,1.,1.,1.,1.,1.,1.,
1.,1.,1.,1.,1.,1.,1.,1.,1.,1.,1.,1.,1.,1.,1.,1.,1.,1.,1.,1.,1.,1.,1.,1.,
1.,1.,1.,1.,1.,1.))
REPRESENTATION_ITEM('')
);
#254=(
BOUNDED_CURVE()
B_SPLINE_CURVE(5,(#37254,#37255,#37256,#37257,#37258,#37259,#37260,#37261,
#37262,#37263,#37264,#37265,#37266,#37267,#37268,#37269,#37270,#37271,#37272,
#37273,#37274,#37275,#37276,#37277,#37278,#37279,#37280,#37281,#37282,#37283,
#37284,#37285,#37286,#37287,#37288,#37289,#37290,#37291,#37292,#37293,#37294,
#37295,#37296,#37297,#37298,#37299,#37300,#37301,#37302,#37303,#37304,#37305,
#37306,#37307,#37308,#37309,#37310,#37311,#37312,#37313,#37314,#37315,#37316,
#37317,#37318,#37319,#37320,#37321,#37322,#37323),.UNSPECIFIED.,.F.,.F.)
B_SPLINE_CURVE_WITH_KNOTS((6,1,1,1,1,1,1,1,1,1,1,1,1,1,1,1,1,1,1,1,1,1,
1,1,1,1,1,1,1,1,1,1,1,1,1,1,1,1,1,1,1,1,1,1,1,1,1,1,1,1,1,1,1,1,1,1,1,1,
1,1,1,1,1,1,1,6),(0.,0.0153846153846154,0.0307692307692308,0.0461538461538462,
0.0615384615384615,0.0769230769230769,0.0923076923076923,0.107692307692308,
0.123076923076923,0.138461538461538,0.153846153846154,0.169230769230769,
0.184615384615385,0.2,0.215384615384615,0.230769230769231,0.246153846153846,
0.261538461538462,0.276923076923077,0.292307692307692,0.307692307692308,
0.323076923076923,0.338461538461538,0.353846153846154,0.369230769230769,
0.384615384615385,0.4,0.415384615384615,0.430769230769231,0.446153846153846,
0.461538461538462,0.476923076923077,0.492307692307692,0.507692307692308,
0.523076923076923,0.538461538461538,0.553846153846154,0.569230769230769,
0.584615384615384,0.6,0.615384615384615,0.63076923076923,0.646153846153846,
0.661538461538461,0.676923076923076,0.692307692307692,0.707692307692307,
0.723076923076922,0.738461538461538,0.753846153846153,0.769230769230768,
0.784615384615384,0.799999999999999,0.815384615384614,0.83076923076923,
0.846153846153845,0.86153846153846,0.876923076923076,0.892307692307691,
0.907692307692306,0.923076923076922,0.938461538461537,0.953846153846152,
0.969230769230768,0.984615384615383,0.994228156739692),.UNSPECIFIED.)
CURVE()
GEOMETRIC_REPRESENTATION_ITEM()
RATIONAL_B_SPLINE_CURVE((1.,1.,1.,1.,1.,1.,1.,1.,1.,1.,1.,1.,1.,1.,1.,1.,
1.,1.,1.,1.,1.,1.,1.,1.,1.,1.,1.,1.,1.,1.,1.,1.,1.,1.,1.,1.,1.,1.,1.,1.,
1.,1.,1.,1.,1.,1.,1.,1.,1.,1.,1.,1.,1.,1.,1.,1.,1.,1.,1.,1.,1.,1.,1.,1.,
1.,1.,1.,1.,1.,1.))
REPRESENTATION_ITEM('')
);
#255=(
BOUNDED_CURVE()
B_SPLINE_CURVE(5,(#37327,#37328,#37329,#37330,#37331,#37332,#37333,#37334,
#37335,#37336,#37337,#37338,#37339,#37340,#37341,#37342,#37343,#37344,#37345,
#37346,#37347,#37348,#37349,#37350,#37351,#37352,#37353,#37354,#37355,#37356,
#37357,#37358,#37359,#37360,#37361,#37362,#37363,#37364,#37365,#37366,#37367,
#37368,#37369,#37370,#37371,#37372,#37373,#37374,#37375,#37376,#37377,#37378,
#37379,#37380,#37381,#37382,#37383,#37384,#37385,#37386,#37387,#37388,#37389,
#37390,#37391,#37392,#37393,#37394,#37395,#37396),.UNSPECIFIED.,.F.,.F.)
B_SPLINE_CURVE_WITH_KNOTS((6,1,1,1,1,1,1,1,1,1,1,1,1,1,1,1,1,1,1,1,1,1,
1,1,1,1,1,1,1,1,1,1,1,1,1,1,1,1,1,1,1,1,1,1,1,1,1,1,1,1,1,1,1,1,1,1,1,1,
1,1,1,1,1,1,1,6),(0.00577184337450777,0.0153846153846154,0.0307692307692308,
0.0461538461538462,0.0615384615384615,0.0769230769230769,0.0923076923076923,
0.107692307692308,0.123076923076923,0.138461538461538,0.153846153846154,
0.169230769230769,0.184615384615385,0.2,0.215384615384615,0.230769230769231,
0.246153846153846,0.261538461538462,0.276923076923077,0.292307692307692,
0.307692307692308,0.323076923076923,0.338461538461538,0.353846153846154,
0.369230769230769,0.384615384615385,0.4,0.415384615384615,0.430769230769231,
0.446153846153846,0.461538461538462,0.476923076923077,0.492307692307692,
0.507692307692308,0.523076923076923,0.538461538461538,0.553846153846154,
0.569230769230769,0.584615384615384,0.6,0.615384615384615,0.63076923076923,
0.646153846153846,0.661538461538461,0.676923076923076,0.692307692307692,
0.707692307692307,0.723076923076922,0.738461538461538,0.753846153846153,
0.769230769230768,0.784615384615384,0.799999999999999,0.815384615384614,
0.83076923076923,0.846153846153845,0.86153846153846,0.876923076923076,0.892307692307691,
0.907692307692306,0.923076923076922,0.938461538461537,0.953846153846152,
0.969230769230768,0.984615384615383,1.),.UNSPECIFIED.)
CURVE()
GEOMETRIC_REPRESENTATION_ITEM()
RATIONAL_B_SPLINE_CURVE((1.,1.,1.,1.,1.,1.,1.,1.,1.,1.,1.,1.,1.,1.,1.,1.,
1.,1.,1.,1.,1.,1.,1.,1.,1.,1.,1.,1.,1.,1.,1.,1.,1.,1.,1.,1.,1.,1.,1.,1.,
1.,1.,1.,1.,1.,1.,1.,1.,1.,1.,1.,1.,1.,1.,1.,1.,1.,1.,1.,1.,1.,1.,1.,1.,
1.,1.,1.,1.,1.,1.))
REPRESENTATION_ITEM('')
);
#256=(
BOUNDED_CURVE()
B_SPLINE_CURVE(5,(#37400,#37401,#37402,#37403,#37404,#37405,#37406,#37407,
#37408,#37409,#37410,#37411,#37412,#37413,#37414,#37415,#37416,#37417,#37418,
#37419,#37420,#37421,#37422,#37423,#37424,#37425,#37426,#37427,#37428,#37429,
#37430,#37431,#37432,#37433,#37434,#37435,#37436,#37437,#37438,#37439,#37440,
#37441,#37442,#37443,#37444,#37445,#37446,#37447,#37448,#37449,#37450,#37451,
#37452,#37453,#37454,#37455,#37456,#37457,#37458,#37459,#37460,#37461,#37462,
#37463,#37464,#37465,#37466,#37467,#37468,#37469),.UNSPECIFIED.,.F.,.F.)
B_SPLINE_CURVE_WITH_KNOTS((6,1,1,1,1,1,1,1,1,1,1,1,1,1,1,1,1,1,1,1,1,1,
1,1,1,1,1,1,1,1,1,1,1,1,1,1,1,1,1,1,1,1,1,1,1,1,1,1,1,1,1,1,1,1,1,1,1,1,
1,1,1,1,1,1,1,6),(0.,0.0153846153846154,0.0307692307692308,0.0461538461538462,
0.0615384615384615,0.0769230769230769,0.0923076923076923,0.107692307692308,
0.123076923076923,0.138461538461538,0.153846153846154,0.169230769230769,
0.184615384615385,0.2,0.215384615384615,0.230769230769231,0.246153846153846,
0.261538461538462,0.276923076923077,0.292307692307692,0.307692307692308,
0.323076923076923,0.338461538461538,0.353846153846154,0.369230769230769,
0.384615384615385,0.4,0.415384615384615,0.430769230769231,0.446153846153846,
0.461538461538462,0.476923076923077,0.492307692307692,0.507692307692308,
0.523076923076923,0.538461538461538,0.553846153846154,0.569230769230769,
0.584615384615384,0.6,0.615384615384615,0.63076923076923,0.646153846153846,
0.661538461538461,0.676923076923076,0.692307692307692,0.707692307692307,
0.723076923076922,0.738461538461538,0.753846153846153,0.769230769230768,
0.784615384615384,0.799999999999999,0.815384615384614,0.83076923076923,
0.846153846153845,0.86153846153846,0.876923076923076,0.892307692307691,
0.907692307692306,0.923076923076922,0.938461538461537,0.953846153846152,
0.969230769230768,0.984615384615383,0.994228156739701),.UNSPECIFIED.)
CURVE()
GEOMETRIC_REPRESENTATION_ITEM()
RATIONAL_B_SPLINE_CURVE((1.,1.,1.,1.,1.,1.,1.,1.,1.,1.,1.,1.,1.,1.,1.,1.,
1.,1.,1.,1.,1.,1.,1.,1.,1.,1.,1.,1.,1.,1.,1.,1.,1.,1.,1.,1.,1.,1.,1.,1.,
1.,1.,1.,1.,1.,1.,1.,1.,1.,1.,1.,1.,1.,1.,1.,1.,1.,1.,1.,1.,1.,1.,1.,1.,
1.,1.,1.,1.,1.,1.))
REPRESENTATION_ITEM('')
);
#257=(
BOUNDED_CURVE()
B_SPLINE_CURVE(5,(#37473,#37474,#37475,#37476,#37477,#37478,#37479,#37480,
#37481,#37482,#37483,#37484,#37485,#37486,#37487,#37488,#37489,#37490,#37491,
#37492,#37493,#37494,#37495,#37496,#37497,#37498,#37499,#37500,#37501,#37502,
#37503,#37504,#37505,#37506,#37507,#37508,#37509,#37510,#37511,#37512,#37513,
#37514,#37515,#37516,#37517,#37518,#37519,#37520,#37521,#37522,#37523,#37524,
#37525,#37526,#37527,#37528,#37529,#37530,#37531,#37532,#37533,#37534,#37535,
#37536,#37537,#37538,#37539,#37540,#37541,#37542),.UNSPECIFIED.,.F.,.F.)
B_SPLINE_CURVE_WITH_KNOTS((6,1,1,1,1,1,1,1,1,1,1,1,1,1,1,1,1,1,1,1,1,1,
1,1,1,1,1,1,1,1,1,1,1,1,1,1,1,1,1,1,1,1,1,1,1,1,1,1,1,1,1,1,1,1,1,1,1,1,
1,1,1,1,1,1,1,6),(0.00577184337450943,0.0153846153846154,0.0307692307692308,
0.0461538461538462,0.0615384615384615,0.0769230769230769,0.0923076923076923,
0.107692307692308,0.123076923076923,0.138461538461538,0.153846153846154,
0.169230769230769,0.184615384615385,0.2,0.215384615384615,0.230769230769231,
0.246153846153846,0.261538461538462,0.276923076923077,0.292307692307692,
0.307692307692308,0.323076923076923,0.338461538461538,0.353846153846154,
0.369230769230769,0.384615384615385,0.4,0.415384615384615,0.430769230769231,
0.446153846153846,0.461538461538462,0.476923076923077,0.492307692307692,
0.507692307692308,0.523076923076923,0.538461538461538,0.553846153846154,
0.569230769230769,0.584615384615384,0.6,0.615384615384615,0.63076923076923,
0.646153846153846,0.661538461538461,0.676923076923076,0.692307692307692,
0.707692307692307,0.723076923076922,0.738461538461538,0.753846153846153,
0.769230769230768,0.784615384615384,0.799999999999999,0.815384615384614,
0.83076923076923,0.846153846153845,0.86153846153846,0.876923076923076,0.892307692307691,
0.907692307692306,0.923076923076922,0.938461538461537,0.953846153846152,
0.969230769230768,0.984615384615383,1.),.UNSPECIFIED.)
CURVE()
GEOMETRIC_REPRESENTATION_ITEM()
RATIONAL_B_SPLINE_CURVE((1.,1.,1.,1.,1.,1.,1.,1.,1.,1.,1.,1.,1.,1.,1.,1.,
1.,1.,1.,1.,1.,1.,1.,1.,1.,1.,1.,1.,1.,1.,1.,1.,1.,1.,1.,1.,1.,1.,1.,1.,
1.,1.,1.,1.,1.,1.,1.,1.,1.,1.,1.,1.,1.,1.,1.,1.,1.,1.,1.,1.,1.,1.,1.,1.,
1.,1.,1.,1.,1.,1.))
REPRESENTATION_ITEM('')
);
#258=(
BOUNDED_CURVE()
B_SPLINE_CURVE(5,(#37546,#37547,#37548,#37549,#37550,#37551,#37552,#37553,
#37554,#37555,#37556,#37557,#37558,#37559,#37560,#37561,#37562,#37563,#37564,
#37565,#37566,#37567,#37568,#37569,#37570,#37571,#37572,#37573,#37574,#37575,
#37576,#37577,#37578,#37579,#37580,#37581,#37582,#37583,#37584,#37585,#37586,
#37587,#37588,#37589,#37590,#37591,#37592,#37593,#37594,#37595,#37596,#37597,
#37598,#37599,#37600,#37601,#37602,#37603,#37604,#37605,#37606,#37607,#37608,
#37609,#37610,#37611,#37612,#37613,#37614,#37615),.UNSPECIFIED.,.F.,.F.)
B_SPLINE_CURVE_WITH_KNOTS((6,1,1,1,1,1,1,1,1,1,1,1,1,1,1,1,1,1,1,1,1,1,
1,1,1,1,1,1,1,1,1,1,1,1,1,1,1,1,1,1,1,1,1,1,1,1,1,1,1,1,1,1,1,1,1,1,1,1,
1,1,1,1,1,1,1,6),(0.,0.0153846153846154,0.0307692307692308,0.0461538461538462,
0.0615384615384615,0.0769230769230769,0.0923076923076923,0.107692307692308,
0.123076923076923,0.138461538461538,0.153846153846154,0.169230769230769,
0.184615384615385,0.2,0.215384615384615,0.230769230769231,0.246153846153846,
0.261538461538462,0.276923076923077,0.292307692307692,0.307692307692308,
0.323076923076923,0.338461538461538,0.353846153846154,0.369230769230769,
0.384615384615385,0.4,0.415384615384615,0.430769230769231,0.446153846153846,
0.461538461538462,0.476923076923077,0.492307692307692,0.507692307692308,
0.523076923076923,0.538461538461538,0.553846153846154,0.569230769230769,
0.584615384615384,0.6,0.615384615384615,0.63076923076923,0.646153846153846,
0.661538461538461,0.676923076923076,0.692307692307692,0.707692307692307,
0.723076923076922,0.738461538461538,0.753846153846153,0.769230769230768,
0.784615384615384,0.799999999999999,0.815384615384614,0.83076923076923,
0.846153846153845,0.86153846153846,0.876923076923076,0.892307692307691,
0.907692307692306,0.923076923076922,0.938461538461537,0.953846153846152,
0.969230769230768,0.984615384615383,0.994228156739699),.UNSPECIFIED.)
CURVE()
GEOMETRIC_REPRESENTATION_ITEM()
RATIONAL_B_SPLINE_CURVE((1.,1.,1.,1.,1.,1.,1.,1.,1.,1.,1.,1.,1.,1.,1.,1.,
1.,1.,1.,1.,1.,1.,1.,1.,1.,1.,1.,1.,1.,1.,1.,1.,1.,1.,1.,1.,1.,1.,1.,1.,
1.,1.,1.,1.,1.,1.,1.,1.,1.,1.,1.,1.,1.,1.,1.,1.,1.,1.,1.,1.,1.,1.,1.,1.,
1.,1.,1.,1.,1.,1.))
REPRESENTATION_ITEM('')
);
#259=(
BOUNDED_CURVE()
B_SPLINE_CURVE(5,(#37619,#37620,#37621,#37622,#37623,#37624,#37625,#37626,
#37627,#37628,#37629,#37630,#37631,#37632,#37633,#37634,#37635,#37636,#37637,
#37638,#37639,#37640,#37641,#37642,#37643,#37644,#37645,#37646,#37647,#37648,
#37649,#37650,#37651,#37652,#37653,#37654,#37655,#37656,#37657,#37658,#37659,
#37660,#37661,#37662,#37663,#37664,#37665,#37666,#37667,#37668,#37669,#37670,
#37671,#37672,#37673,#37674,#37675,#37676,#37677,#37678,#37679,#37680,#37681,
#37682,#37683,#37684,#37685,#37686,#37687,#37688),.UNSPECIFIED.,.F.,.F.)
B_SPLINE_CURVE_WITH_KNOTS((6,1,1,1,1,1,1,1,1,1,1,1,1,1,1,1,1,1,1,1,1,1,
1,1,1,1,1,1,1,1,1,1,1,1,1,1,1,1,1,1,1,1,1,1,1,1,1,1,1,1,1,1,1,1,1,1,1,1,
1,1,1,1,1,1,1,6),(0.00577184337448657,0.0153846153846154,0.0307692307692308,
0.0461538461538462,0.0615384615384615,0.0769230769230769,0.0923076923076923,
0.107692307692308,0.123076923076923,0.138461538461538,0.153846153846154,
0.169230769230769,0.184615384615385,0.2,0.215384615384615,0.230769230769231,
0.246153846153846,0.261538461538462,0.276923076923077,0.292307692307692,
0.307692307692308,0.323076923076923,0.338461538461538,0.353846153846154,
0.369230769230769,0.384615384615385,0.4,0.415384615384615,0.430769230769231,
0.446153846153846,0.461538461538462,0.476923076923077,0.492307692307692,
0.507692307692308,0.523076923076923,0.538461538461538,0.553846153846154,
0.569230769230769,0.584615384615384,0.6,0.615384615384615,0.63076923076923,
0.646153846153846,0.661538461538461,0.676923076923076,0.692307692307692,
0.707692307692307,0.723076923076922,0.738461538461538,0.753846153846153,
0.769230769230768,0.784615384615384,0.799999999999999,0.815384615384614,
0.83076923076923,0.846153846153845,0.86153846153846,0.876923076923076,0.892307692307691,
0.907692307692306,0.923076923076922,0.938461538461537,0.953846153846152,
0.969230769230768,0.984615384615383,1.),.UNSPECIFIED.)
CURVE()
GEOMETRIC_REPRESENTATION_ITEM()
RATIONAL_B_SPLINE_CURVE((1.,1.,1.,1.,1.,1.,1.,1.,1.,1.,1.,1.,1.,1.,1.,1.,
1.,1.,1.,1.,1.,1.,1.,1.,1.,1.,1.,1.,1.,1.,1.,1.,1.,1.,1.,1.,1.,1.,1.,1.,
1.,1.,1.,1.,1.,1.,1.,1.,1.,1.,1.,1.,1.,1.,1.,1.,1.,1.,1.,1.,1.,1.,1.,1.,
1.,1.,1.,1.,1.,1.))
REPRESENTATION_ITEM('')
);
#260=(
BOUNDED_CURVE()
B_SPLINE_CURVE(5,(#37692,#37693,#37694,#37695,#37696,#37697,#37698,#37699,
#37700,#37701,#37702,#37703,#37704,#37705,#37706,#37707,#37708,#37709,#37710,
#37711,#37712,#37713,#37714,#37715,#37716,#37717,#37718,#37719,#37720,#37721,
#37722,#37723,#37724,#37725,#37726,#37727,#37728,#37729,#37730,#37731,#37732,
#37733,#37734,#37735,#37736,#37737,#37738,#37739,#37740,#37741,#37742,#37743,
#37744,#37745,#37746,#37747,#37748,#37749,#37750,#37751,#37752,#37753,#37754,
#37755,#37756,#37757,#37758,#37759,#37760,#37761),.UNSPECIFIED.,.F.,.F.)
B_SPLINE_CURVE_WITH_KNOTS((6,1,1,1,1,1,1,1,1,1,1,1,1,1,1,1,1,1,1,1,1,1,
1,1,1,1,1,1,1,1,1,1,1,1,1,1,1,1,1,1,1,1,1,1,1,1,1,1,1,1,1,1,1,1,1,1,1,1,
1,1,1,1,1,1,1,6),(0.,0.0153846153846154,0.0307692307692308,0.0461538461538462,
0.0615384615384615,0.0769230769230769,0.0923076923076923,0.107692307692308,
0.123076923076923,0.138461538461538,0.153846153846154,0.169230769230769,
0.184615384615385,0.2,0.215384615384615,0.230769230769231,0.246153846153846,
0.261538461538462,0.276923076923077,0.292307692307692,0.307692307692308,
0.323076923076923,0.338461538461538,0.353846153846154,0.369230769230769,
0.384615384615385,0.4,0.415384615384615,0.430769230769231,0.446153846153846,
0.461538461538462,0.476923076923077,0.492307692307692,0.507692307692308,
0.523076923076923,0.538461538461538,0.553846153846154,0.569230769230769,
0.584615384615384,0.6,0.615384615384615,0.63076923076923,0.646153846153846,
0.661538461538461,0.676923076923076,0.692307692307692,0.707692307692307,
0.723076923076922,0.738461538461538,0.753846153846153,0.769230769230768,
0.784615384615384,0.799999999999999,0.815384615384614,0.83076923076923,
0.846153846153845,0.86153846153846,0.876923076923076,0.892307692307691,
0.907692307692306,0.923076923076922,0.938461538461537,0.953846153846152,
0.969230769230768,0.984615384615383,0.994228156739709),.UNSPECIFIED.)
CURVE()
GEOMETRIC_REPRESENTATION_ITEM()
RATIONAL_B_SPLINE_CURVE((1.,1.,1.,1.,1.,1.,1.,1.,1.,1.,1.,1.,1.,1.,1.,1.,
1.,1.,1.,1.,1.,1.,1.,1.,1.,1.,1.,1.,1.,1.,1.,1.,1.,1.,1.,1.,1.,1.,1.,1.,
1.,1.,1.,1.,1.,1.,1.,1.,1.,1.,1.,1.,1.,1.,1.,1.,1.,1.,1.,1.,1.,1.,1.,1.,
1.,1.,1.,1.,1.,1.))
REPRESENTATION_ITEM('')
);
#261=(
BOUNDED_CURVE()
B_SPLINE_CURVE(5,(#37765,#37766,#37767,#37768,#37769,#37770,#37771,#37772,
#37773,#37774,#37775,#37776,#37777,#37778,#37779,#37780,#37781,#37782,#37783,
#37784,#37785,#37786,#37787,#37788,#37789,#37790,#37791,#37792,#37793,#37794,
#37795,#37796,#37797,#37798,#37799,#37800,#37801,#37802,#37803,#37804,#37805,
#37806,#37807,#37808,#37809,#37810,#37811,#37812,#37813,#37814,#37815,#37816,
#37817,#37818,#37819,#37820,#37821,#37822,#37823,#37824,#37825,#37826,#37827,
#37828,#37829,#37830,#37831,#37832,#37833,#37834),.UNSPECIFIED.,.F.,.F.)
B_SPLINE_CURVE_WITH_KNOTS((6,1,1,1,1,1,1,1,1,1,1,1,1,1,1,1,1,1,1,1,1,1,
1,1,1,1,1,1,1,1,1,1,1,1,1,1,1,1,1,1,1,1,1,1,1,1,1,1,1,1,1,1,1,1,1,1,1,1,
1,1,1,1,1,1,1,6),(0.00577184337451132,0.0153846153846154,0.0307692307692308,
0.0461538461538462,0.0615384615384615,0.0769230769230769,0.0923076923076923,
0.107692307692308,0.123076923076923,0.138461538461538,0.153846153846154,
0.169230769230769,0.184615384615385,0.2,0.215384615384615,0.230769230769231,
0.246153846153846,0.261538461538462,0.276923076923077,0.292307692307692,
0.307692307692308,0.323076923076923,0.338461538461538,0.353846153846154,
0.369230769230769,0.384615384615385,0.4,0.415384615384615,0.430769230769231,
0.446153846153846,0.461538461538462,0.476923076923077,0.492307692307692,
0.507692307692308,0.523076923076923,0.538461538461538,0.553846153846154,
0.569230769230769,0.584615384615384,0.6,0.615384615384615,0.63076923076923,
0.646153846153846,0.661538461538461,0.676923076923076,0.692307692307692,
0.707692307692307,0.723076923076922,0.738461538461538,0.753846153846153,
0.769230769230768,0.784615384615384,0.799999999999999,0.815384615384614,
0.83076923076923,0.846153846153845,0.86153846153846,0.876923076923076,0.892307692307691,
0.907692307692306,0.923076923076922,0.938461538461537,0.953846153846152,
0.969230769230768,0.984615384615383,1.),.UNSPECIFIED.)
CURVE()
GEOMETRIC_REPRESENTATION_ITEM()
RATIONAL_B_SPLINE_CURVE((1.,1.,1.,1.,1.,1.,1.,1.,1.,1.,1.,1.,1.,1.,1.,1.,
1.,1.,1.,1.,1.,1.,1.,1.,1.,1.,1.,1.,1.,1.,1.,1.,1.,1.,1.,1.,1.,1.,1.,1.,
1.,1.,1.,1.,1.,1.,1.,1.,1.,1.,1.,1.,1.,1.,1.,1.,1.,1.,1.,1.,1.,1.,1.,1.,
1.,1.,1.,1.,1.,1.))
REPRESENTATION_ITEM('')
);
#262=(
BOUNDED_CURVE()
B_SPLINE_CURVE(5,(#37838,#37839,#37840,#37841,#37842,#37843,#37844,#37845,
#37846,#37847,#37848,#37849,#37850,#37851,#37852,#37853,#37854,#37855,#37856,
#37857,#37858,#37859,#37860,#37861,#37862,#37863,#37864,#37865,#37866,#37867,
#37868,#37869,#37870,#37871,#37872,#37873,#37874,#37875,#37876,#37877,#37878,
#37879,#37880,#37881,#37882,#37883,#37884,#37885,#37886,#37887,#37888,#37889,
#37890,#37891,#37892,#37893,#37894,#37895,#37896,#37897,#37898,#37899,#37900,
#37901,#37902,#37903,#37904,#37905,#37906,#37907),.UNSPECIFIED.,.F.,.F.)
B_SPLINE_CURVE_WITH_KNOTS((6,1,1,1,1,1,1,1,1,1,1,1,1,1,1,1,1,1,1,1,1,1,
1,1,1,1,1,1,1,1,1,1,1,1,1,1,1,1,1,1,1,1,1,1,1,1,1,1,1,1,1,1,1,1,1,1,1,1,
1,1,1,1,1,1,1,6),(0.,0.0153846153846154,0.0307692307692308,0.0461538461538462,
0.0615384615384615,0.0769230769230769,0.0923076923076923,0.107692307692308,
0.123076923076923,0.138461538461538,0.153846153846154,0.169230769230769,
0.184615384615385,0.2,0.215384615384615,0.230769230769231,0.246153846153846,
0.261538461538462,0.276923076923077,0.292307692307692,0.307692307692308,
0.323076923076923,0.338461538461538,0.353846153846154,0.369230769230769,
0.384615384615385,0.4,0.415384615384615,0.430769230769231,0.446153846153846,
0.461538461538462,0.476923076923077,0.492307692307692,0.507692307692308,
0.523076923076923,0.538461538461538,0.553846153846154,0.569230769230769,
0.584615384615384,0.6,0.615384615384615,0.63076923076923,0.646153846153846,
0.661538461538461,0.676923076923076,0.692307692307692,0.707692307692307,
0.723076923076922,0.738461538461538,0.753846153846153,0.769230769230768,
0.784615384615384,0.799999999999999,0.815384615384614,0.83076923076923,
0.846153846153845,0.86153846153846,0.876923076923076,0.892307692307691,
0.907692307692306,0.923076923076922,0.938461538461537,0.953846153846152,
0.969230769230768,0.984615384615383,0.994228156739705),.UNSPECIFIED.)
CURVE()
GEOMETRIC_REPRESENTATION_ITEM()
RATIONAL_B_SPLINE_CURVE((1.,1.,1.,1.,1.,1.,1.,1.,1.,1.,1.,1.,1.,1.,1.,1.,
1.,1.,1.,1.,1.,1.,1.,1.,1.,1.,1.,1.,1.,1.,1.,1.,1.,1.,1.,1.,1.,1.,1.,1.,
1.,1.,1.,1.,1.,1.,1.,1.,1.,1.,1.,1.,1.,1.,1.,1.,1.,1.,1.,1.,1.,1.,1.,1.,
1.,1.,1.,1.,1.,1.))
REPRESENTATION_ITEM('')
);
#263=(
BOUNDED_CURVE()
B_SPLINE_CURVE(5,(#37911,#37912,#37913,#37914,#37915,#37916,#37917,#37918,
#37919,#37920,#37921,#37922,#37923,#37924,#37925,#37926,#37927,#37928,#37929,
#37930,#37931,#37932,#37933,#37934,#37935,#37936,#37937,#37938,#37939,#37940,
#37941,#37942,#37943,#37944,#37945,#37946,#37947,#37948,#37949,#37950,#37951,
#37952,#37953,#37954,#37955,#37956,#37957,#37958,#37959,#37960,#37961,#37962,
#37963,#37964,#37965,#37966,#37967,#37968,#37969,#37970,#37971,#37972,#37973,
#37974,#37975,#37976,#37977,#37978,#37979,#37980),.UNSPECIFIED.,.F.,.F.)
B_SPLINE_CURVE_WITH_KNOTS((6,1,1,1,1,1,1,1,1,1,1,1,1,1,1,1,1,1,1,1,1,1,
1,1,1,1,1,1,1,1,1,1,1,1,1,1,1,1,1,1,1,1,1,1,1,1,1,1,1,1,1,1,1,1,1,1,1,1,
1,1,1,1,1,1,1,6),(0.00577184337450072,0.0153846153846154,0.0307692307692308,
0.0461538461538462,0.0615384615384615,0.0769230769230769,0.0923076923076923,
0.107692307692308,0.123076923076923,0.138461538461538,0.153846153846154,
0.169230769230769,0.184615384615385,0.2,0.215384615384615,0.230769230769231,
0.246153846153846,0.261538461538462,0.276923076923077,0.292307692307692,
0.307692307692308,0.323076923076923,0.338461538461538,0.353846153846154,
0.369230769230769,0.384615384615385,0.4,0.415384615384615,0.430769230769231,
0.446153846153846,0.461538461538462,0.476923076923077,0.492307692307692,
0.507692307692308,0.523076923076923,0.538461538461538,0.553846153846154,
0.569230769230769,0.584615384615384,0.6,0.615384615384615,0.63076923076923,
0.646153846153846,0.661538461538461,0.676923076923076,0.692307692307692,
0.707692307692307,0.723076923076922,0.738461538461538,0.753846153846153,
0.769230769230768,0.784615384615384,0.799999999999999,0.815384615384614,
0.83076923076923,0.846153846153845,0.86153846153846,0.876923076923076,0.892307692307691,
0.907692307692306,0.923076923076922,0.938461538461537,0.953846153846152,
0.969230769230768,0.984615384615383,1.),.UNSPECIFIED.)
CURVE()
GEOMETRIC_REPRESENTATION_ITEM()
RATIONAL_B_SPLINE_CURVE((1.,1.,1.,1.,1.,1.,1.,1.,1.,1.,1.,1.,1.,1.,1.,1.,
1.,1.,1.,1.,1.,1.,1.,1.,1.,1.,1.,1.,1.,1.,1.,1.,1.,1.,1.,1.,1.,1.,1.,1.,
1.,1.,1.,1.,1.,1.,1.,1.,1.,1.,1.,1.,1.,1.,1.,1.,1.,1.,1.,1.,1.,1.,1.,1.,
1.,1.,1.,1.,1.,1.))
REPRESENTATION_ITEM('')
);
#264=(
BOUNDED_CURVE()
B_SPLINE_CURVE(5,(#37984,#37985,#37986,#37987,#37988,#37989,#37990,#37991,
#37992,#37993,#37994,#37995,#37996,#37997,#37998,#37999,#38000,#38001,#38002,
#38003,#38004,#38005,#38006,#38007,#38008,#38009,#38010,#38011,#38012,#38013,
#38014,#38015,#38016,#38017,#38018,#38019,#38020,#38021,#38022,#38023,#38024,
#38025,#38026,#38027,#38028,#38029,#38030,#38031,#38032,#38033,#38034,#38035,
#38036,#38037,#38038,#38039,#38040,#38041,#38042,#38043,#38044,#38045,#38046,
#38047,#38048,#38049,#38050,#38051,#38052,#38053),.UNSPECIFIED.,.F.,.F.)
B_SPLINE_CURVE_WITH_KNOTS((6,1,1,1,1,1,1,1,1,1,1,1,1,1,1,1,1,1,1,1,1,1,
1,1,1,1,1,1,1,1,1,1,1,1,1,1,1,1,1,1,1,1,1,1,1,1,1,1,1,1,1,1,1,1,1,1,1,1,
1,1,1,1,1,1,1,6),(0.,0.0153846153846154,0.0307692307692308,0.0461538461538462,
0.0615384615384615,0.0769230769230769,0.0923076923076923,0.107692307692308,
0.123076923076923,0.138461538461538,0.153846153846154,0.169230769230769,
0.184615384615385,0.2,0.215384615384615,0.230769230769231,0.246153846153846,
0.261538461538462,0.276923076923077,0.292307692307692,0.307692307692308,
0.323076923076923,0.338461538461538,0.353846153846154,0.369230769230769,
0.384615384615385,0.4,0.415384615384615,0.430769230769231,0.446153846153846,
0.461538461538462,0.476923076923077,0.492307692307692,0.507692307692308,
0.523076923076923,0.538461538461538,0.553846153846154,0.569230769230769,
0.584615384615384,0.6,0.615384615384615,0.63076923076923,0.646153846153846,
0.661538461538461,0.676923076923076,0.692307692307692,0.707692307692307,
0.723076923076922,0.738461538461538,0.753846153846153,0.769230769230768,
0.784615384615384,0.799999999999999,0.815384615384614,0.83076923076923,
0.846153846153845,0.86153846153846,0.876923076923076,0.892307692307691,
0.907692307692306,0.923076923076922,0.938461538461537,0.953846153846152,
0.969230769230768,0.984615384615383,0.994228156739706),.UNSPECIFIED.)
CURVE()
GEOMETRIC_REPRESENTATION_ITEM()
RATIONAL_B_SPLINE_CURVE((1.,1.,1.,1.,1.,1.,1.,1.,1.,1.,1.,1.,1.,1.,1.,1.,
1.,1.,1.,1.,1.,1.,1.,1.,1.,1.,1.,1.,1.,1.,1.,1.,1.,1.,1.,1.,1.,1.,1.,1.,
1.,1.,1.,1.,1.,1.,1.,1.,1.,1.,1.,1.,1.,1.,1.,1.,1.,1.,1.,1.,1.,1.,1.,1.,
1.,1.,1.,1.,1.,1.))
REPRESENTATION_ITEM('')
);
#265=(
BOUNDED_CURVE()
B_SPLINE_CURVE(5,(#38057,#38058,#38059,#38060,#38061,#38062,#38063,#38064,
#38065,#38066,#38067,#38068,#38069,#38070,#38071,#38072,#38073,#38074,#38075,
#38076,#38077,#38078,#38079,#38080,#38081,#38082,#38083,#38084,#38085,#38086,
#38087,#38088,#38089,#38090,#38091,#38092,#38093,#38094,#38095,#38096,#38097,
#38098,#38099,#38100,#38101,#38102,#38103,#38104,#38105,#38106,#38107,#38108,
#38109,#38110,#38111,#38112,#38113,#38114,#38115,#38116,#38117,#38118,#38119,
#38120,#38121,#38122,#38123,#38124,#38125,#38126),.UNSPECIFIED.,.F.,.F.)
B_SPLINE_CURVE_WITH_KNOTS((6,1,1,1,1,1,1,1,1,1,1,1,1,1,1,1,1,1,1,1,1,1,
1,1,1,1,1,1,1,1,1,1,1,1,1,1,1,1,1,1,1,1,1,1,1,1,1,1,1,1,1,1,1,1,1,1,1,1,
1,1,1,1,1,1,1,6),(0.00577184337450902,0.0153846153846154,0.0307692307692308,
0.0461538461538462,0.0615384615384615,0.0769230769230769,0.0923076923076923,
0.107692307692308,0.123076923076923,0.138461538461538,0.153846153846154,
0.169230769230769,0.184615384615385,0.2,0.215384615384615,0.230769230769231,
0.246153846153846,0.261538461538462,0.276923076923077,0.292307692307692,
0.307692307692308,0.323076923076923,0.338461538461538,0.353846153846154,
0.369230769230769,0.384615384615385,0.4,0.415384615384615,0.430769230769231,
0.446153846153846,0.461538461538462,0.476923076923077,0.492307692307692,
0.507692307692308,0.523076923076923,0.538461538461538,0.553846153846154,
0.569230769230769,0.584615384615384,0.6,0.615384615384615,0.63076923076923,
0.646153846153846,0.661538461538461,0.676923076923076,0.692307692307692,
0.707692307692307,0.723076923076922,0.738461538461538,0.753846153846153,
0.769230769230768,0.784615384615384,0.799999999999999,0.815384615384614,
0.83076923076923,0.846153846153845,0.86153846153846,0.876923076923076,0.892307692307691,
0.907692307692306,0.923076923076922,0.938461538461537,0.953846153846152,
0.969230769230768,0.984615384615383,1.),.UNSPECIFIED.)
CURVE()
GEOMETRIC_REPRESENTATION_ITEM()
RATIONAL_B_SPLINE_CURVE((1.,1.,1.,1.,1.,1.,1.,1.,1.,1.,1.,1.,1.,1.,1.,1.,
1.,1.,1.,1.,1.,1.,1.,1.,1.,1.,1.,1.,1.,1.,1.,1.,1.,1.,1.,1.,1.,1.,1.,1.,
1.,1.,1.,1.,1.,1.,1.,1.,1.,1.,1.,1.,1.,1.,1.,1.,1.,1.,1.,1.,1.,1.,1.,1.,
1.,1.,1.,1.,1.,1.))
REPRESENTATION_ITEM('')
);
#266=(
BOUNDED_CURVE()
B_SPLINE_CURVE(5,(#38130,#38131,#38132,#38133,#38134,#38135,#38136,#38137,
#38138,#38139,#38140,#38141,#38142,#38143,#38144,#38145,#38146,#38147,#38148,
#38149,#38150,#38151,#38152,#38153,#38154,#38155,#38156,#38157,#38158,#38159,
#38160,#38161,#38162,#38163,#38164,#38165,#38166,#38167,#38168,#38169,#38170,
#38171,#38172,#38173,#38174,#38175,#38176,#38177,#38178,#38179,#38180,#38181,
#38182,#38183,#38184,#38185,#38186,#38187,#38188,#38189,#38190,#38191,#38192,
#38193,#38194,#38195,#38196,#38197,#38198,#38199),.UNSPECIFIED.,.F.,.F.)
B_SPLINE_CURVE_WITH_KNOTS((6,1,1,1,1,1,1,1,1,1,1,1,1,1,1,1,1,1,1,1,1,1,
1,1,1,1,1,1,1,1,1,1,1,1,1,1,1,1,1,1,1,1,1,1,1,1,1,1,1,1,1,1,1,1,1,1,1,1,
1,1,1,1,1,1,1,6),(0.,0.0153846153846154,0.0307692307692308,0.0461538461538462,
0.0615384615384615,0.0769230769230769,0.0923076923076923,0.107692307692308,
0.123076923076923,0.138461538461538,0.153846153846154,0.169230769230769,
0.184615384615385,0.2,0.215384615384615,0.230769230769231,0.246153846153846,
0.261538461538462,0.276923076923077,0.292307692307692,0.307692307692308,
0.323076923076923,0.338461538461538,0.353846153846154,0.369230769230769,
0.384615384615385,0.4,0.415384615384615,0.430769230769231,0.446153846153846,
0.461538461538462,0.476923076923077,0.492307692307692,0.507692307692308,
0.523076923076923,0.538461538461538,0.553846153846154,0.569230769230769,
0.584615384615384,0.6,0.615384615384615,0.63076923076923,0.646153846153846,
0.661538461538461,0.676923076923076,0.692307692307692,0.707692307692307,
0.723076923076922,0.738461538461538,0.753846153846153,0.769230769230768,
0.784615384615384,0.799999999999999,0.815384615384614,0.83076923076923,
0.846153846153845,0.86153846153846,0.876923076923076,0.892307692307691,
0.907692307692306,0.923076923076922,0.938461538461537,0.953846153846152,
0.969230769230768,0.984615384615383,0.994228156739698),.UNSPECIFIED.)
CURVE()
GEOMETRIC_REPRESENTATION_ITEM()
RATIONAL_B_SPLINE_CURVE((1.,1.,1.,1.,1.,1.,1.,1.,1.,1.,1.,1.,1.,1.,1.,1.,
1.,1.,1.,1.,1.,1.,1.,1.,1.,1.,1.,1.,1.,1.,1.,1.,1.,1.,1.,1.,1.,1.,1.,1.,
1.,1.,1.,1.,1.,1.,1.,1.,1.,1.,1.,1.,1.,1.,1.,1.,1.,1.,1.,1.,1.,1.,1.,1.,
1.,1.,1.,1.,1.,1.))
REPRESENTATION_ITEM('')
);
#267=(
BOUNDED_CURVE()
B_SPLINE_CURVE(5,(#38203,#38204,#38205,#38206,#38207,#38208,#38209,#38210,
#38211,#38212,#38213,#38214,#38215,#38216,#38217,#38218,#38219,#38220,#38221,
#38222,#38223,#38224,#38225,#38226,#38227,#38228,#38229,#38230,#38231,#38232,
#38233,#38234,#38235,#38236,#38237,#38238,#38239,#38240,#38241,#38242,#38243,
#38244,#38245,#38246,#38247,#38248,#38249,#38250,#38251,#38252,#38253,#38254,
#38255,#38256,#38257,#38258,#38259,#38260,#38261,#38262,#38263,#38264,#38265,
#38266,#38267,#38268,#38269,#38270,#38271,#38272),.UNSPECIFIED.,.F.,.F.)
B_SPLINE_CURVE_WITH_KNOTS((6,1,1,1,1,1,1,1,1,1,1,1,1,1,1,1,1,1,1,1,1,1,
1,1,1,1,1,1,1,1,1,1,1,1,1,1,1,1,1,1,1,1,1,1,1,1,1,1,1,1,1,1,1,1,1,1,1,1,
1,1,1,1,1,1,1,6),(0.00577184337451611,0.0153846153846154,0.0307692307692308,
0.0461538461538462,0.0615384615384615,0.0769230769230769,0.0923076923076923,
0.107692307692308,0.123076923076923,0.138461538461538,0.153846153846154,
0.169230769230769,0.184615384615385,0.2,0.215384615384615,0.230769230769231,
0.246153846153846,0.261538461538462,0.276923076923077,0.292307692307692,
0.307692307692308,0.323076923076923,0.338461538461538,0.353846153846154,
0.369230769230769,0.384615384615385,0.4,0.415384615384615,0.430769230769231,
0.446153846153846,0.461538461538462,0.476923076923077,0.492307692307692,
0.507692307692308,0.523076923076923,0.538461538461538,0.553846153846154,
0.569230769230769,0.584615384615384,0.6,0.615384615384615,0.63076923076923,
0.646153846153846,0.661538461538461,0.676923076923076,0.692307692307692,
0.707692307692307,0.723076923076922,0.738461538461538,0.753846153846153,
0.769230769230768,0.784615384615384,0.799999999999999,0.815384615384614,
0.83076923076923,0.846153846153845,0.86153846153846,0.876923076923076,0.892307692307691,
0.907692307692306,0.923076923076922,0.938461538461537,0.953846153846152,
0.969230769230768,0.984615384615383,1.),.UNSPECIFIED.)
CURVE()
GEOMETRIC_REPRESENTATION_ITEM()
RATIONAL_B_SPLINE_CURVE((1.,1.,1.,1.,1.,1.,1.,1.,1.,1.,1.,1.,1.,1.,1.,1.,
1.,1.,1.,1.,1.,1.,1.,1.,1.,1.,1.,1.,1.,1.,1.,1.,1.,1.,1.,1.,1.,1.,1.,1.,
1.,1.,1.,1.,1.,1.,1.,1.,1.,1.,1.,1.,1.,1.,1.,1.,1.,1.,1.,1.,1.,1.,1.,1.,
1.,1.,1.,1.,1.,1.))
REPRESENTATION_ITEM('')
);
#268=(
BOUNDED_CURVE()
B_SPLINE_CURVE(5,(#38276,#38277,#38278,#38279,#38280,#38281,#38282,#38283,
#38284,#38285,#38286,#38287,#38288,#38289,#38290,#38291,#38292,#38293,#38294,
#38295,#38296,#38297,#38298,#38299,#38300,#38301,#38302,#38303,#38304,#38305,
#38306,#38307,#38308,#38309,#38310,#38311,#38312,#38313,#38314,#38315,#38316,
#38317,#38318,#38319,#38320,#38321,#38322,#38323,#38324,#38325,#38326,#38327,
#38328,#38329,#38330,#38331,#38332,#38333,#38334,#38335,#38336,#38337,#38338,
#38339,#38340,#38341,#38342,#38343,#38344,#38345),.UNSPECIFIED.,.F.,.F.)
B_SPLINE_CURVE_WITH_KNOTS((6,1,1,1,1,1,1,1,1,1,1,1,1,1,1,1,1,1,1,1,1,1,
1,1,1,1,1,1,1,1,1,1,1,1,1,1,1,1,1,1,1,1,1,1,1,1,1,1,1,1,1,1,1,1,1,1,1,1,
1,1,1,1,1,1,1,6),(0.,0.0153846153846154,0.0307692307692308,0.0461538461538462,
0.0615384615384615,0.0769230769230769,0.0923076923076923,0.107692307692308,
0.123076923076923,0.138461538461538,0.153846153846154,0.169230769230769,
0.184615384615385,0.2,0.215384615384615,0.230769230769231,0.246153846153846,
0.261538461538462,0.276923076923077,0.292307692307692,0.307692307692308,
0.323076923076923,0.338461538461538,0.353846153846154,0.369230769230769,
0.384615384615385,0.4,0.415384615384615,0.430769230769231,0.446153846153846,
0.461538461538462,0.476923076923077,0.492307692307692,0.507692307692308,
0.523076923076923,0.538461538461538,0.553846153846154,0.569230769230769,
0.584615384615384,0.6,0.615384615384615,0.63076923076923,0.646153846153846,
0.661538461538461,0.676923076923076,0.692307692307692,0.707692307692307,
0.723076923076922,0.738461538461538,0.753846153846153,0.769230769230768,
0.784615384615384,0.799999999999999,0.815384615384614,0.83076923076923,
0.846153846153845,0.86153846153846,0.876923076923076,0.892307692307691,
0.907692307692306,0.923076923076922,0.938461538461537,0.953846153846152,
0.969230769230768,0.984615384615383,0.994228156739704),.UNSPECIFIED.)
CURVE()
GEOMETRIC_REPRESENTATION_ITEM()
RATIONAL_B_SPLINE_CURVE((1.,1.,1.,1.,1.,1.,1.,1.,1.,1.,1.,1.,1.,1.,1.,1.,
1.,1.,1.,1.,1.,1.,1.,1.,1.,1.,1.,1.,1.,1.,1.,1.,1.,1.,1.,1.,1.,1.,1.,1.,
1.,1.,1.,1.,1.,1.,1.,1.,1.,1.,1.,1.,1.,1.,1.,1.,1.,1.,1.,1.,1.,1.,1.,1.,
1.,1.,1.,1.,1.,1.))
REPRESENTATION_ITEM('')
);
#269=(
BOUNDED_CURVE()
B_SPLINE_CURVE(5,(#38349,#38350,#38351,#38352,#38353,#38354,#38355,#38356,
#38357,#38358,#38359,#38360,#38361,#38362,#38363,#38364,#38365,#38366,#38367,
#38368,#38369,#38370,#38371,#38372,#38373,#38374,#38375,#38376,#38377,#38378,
#38379,#38380,#38381,#38382,#38383,#38384,#38385,#38386,#38387,#38388,#38389,
#38390,#38391,#38392,#38393,#38394,#38395,#38396,#38397,#38398,#38399,#38400,
#38401,#38402,#38403,#38404,#38405,#38406,#38407,#38408,#38409,#38410,#38411,
#38412,#38413,#38414,#38415,#38416,#38417,#38418),.UNSPECIFIED.,.F.,.F.)
B_SPLINE_CURVE_WITH_KNOTS((6,1,1,1,1,1,1,1,1,1,1,1,1,1,1,1,1,1,1,1,1,1,
1,1,1,1,1,1,1,1,1,1,1,1,1,1,1,1,1,1,1,1,1,1,1,1,1,1,1,1,1,1,1,1,1,1,1,1,
1,1,1,1,1,1,1,6),(0.00577184337449682,0.0153846153846154,0.0307692307692308,
0.0461538461538462,0.0615384615384615,0.0769230769230769,0.0923076923076923,
0.107692307692308,0.123076923076923,0.138461538461538,0.153846153846154,
0.169230769230769,0.184615384615385,0.2,0.215384615384615,0.230769230769231,
0.246153846153846,0.261538461538462,0.276923076923077,0.292307692307692,
0.307692307692308,0.323076923076923,0.338461538461538,0.353846153846154,
0.369230769230769,0.384615384615385,0.4,0.415384615384615,0.430769230769231,
0.446153846153846,0.461538461538462,0.476923076923077,0.492307692307692,
0.507692307692308,0.523076923076923,0.538461538461538,0.553846153846154,
0.569230769230769,0.584615384615384,0.6,0.615384615384615,0.63076923076923,
0.646153846153846,0.661538461538461,0.676923076923076,0.692307692307692,
0.707692307692307,0.723076923076922,0.738461538461538,0.753846153846153,
0.769230769230768,0.784615384615384,0.799999999999999,0.815384615384614,
0.83076923076923,0.846153846153845,0.86153846153846,0.876923076923076,0.892307692307691,
0.907692307692306,0.923076923076922,0.938461538461537,0.953846153846152,
0.969230769230768,0.984615384615383,1.),.UNSPECIFIED.)
CURVE()
GEOMETRIC_REPRESENTATION_ITEM()
RATIONAL_B_SPLINE_CURVE((1.,1.,1.,1.,1.,1.,1.,1.,1.,1.,1.,1.,1.,1.,1.,1.,
1.,1.,1.,1.,1.,1.,1.,1.,1.,1.,1.,1.,1.,1.,1.,1.,1.,1.,1.,1.,1.,1.,1.,1.,
1.,1.,1.,1.,1.,1.,1.,1.,1.,1.,1.,1.,1.,1.,1.,1.,1.,1.,1.,1.,1.,1.,1.,1.,
1.,1.,1.,1.,1.,1.))
REPRESENTATION_ITEM('')
);
#270=(
BOUNDED_CURVE()
B_SPLINE_CURVE(5,(#38422,#38423,#38424,#38425,#38426,#38427,#38428,#38429,
#38430,#38431,#38432,#38433,#38434,#38435,#38436,#38437,#38438,#38439,#38440,
#38441,#38442,#38443,#38444,#38445,#38446,#38447,#38448,#38449,#38450,#38451,
#38452,#38453,#38454,#38455,#38456,#38457,#38458,#38459,#38460,#38461,#38462,
#38463,#38464,#38465,#38466,#38467,#38468,#38469,#38470,#38471,#38472,#38473,
#38474,#38475,#38476,#38477,#38478,#38479,#38480,#38481,#38482,#38483,#38484,
#38485,#38486,#38487,#38488,#38489,#38490,#38491),.UNSPECIFIED.,.F.,.F.)
B_SPLINE_CURVE_WITH_KNOTS((6,1,1,1,1,1,1,1,1,1,1,1,1,1,1,1,1,1,1,1,1,1,
1,1,1,1,1,1,1,1,1,1,1,1,1,1,1,1,1,1,1,1,1,1,1,1,1,1,1,1,1,1,1,1,1,1,1,1,
1,1,1,1,1,1,1,6),(0.,0.0153846153846154,0.0307692307692308,0.0461538461538462,
0.0615384615384615,0.0769230769230769,0.0923076923076923,0.107692307692308,
0.123076923076923,0.138461538461538,0.153846153846154,0.169230769230769,
0.184615384615385,0.2,0.215384615384615,0.230769230769231,0.246153846153846,
0.261538461538462,0.276923076923077,0.292307692307692,0.307692307692308,
0.323076923076923,0.338461538461538,0.353846153846154,0.369230769230769,
0.384615384615385,0.4,0.415384615384615,0.430769230769231,0.446153846153846,
0.461538461538462,0.476923076923077,0.492307692307692,0.507692307692308,
0.523076923076923,0.538461538461538,0.553846153846154,0.569230769230769,
0.584615384615384,0.6,0.615384615384615,0.63076923076923,0.646153846153846,
0.661538461538461,0.676923076923076,0.692307692307692,0.707692307692307,
0.723076923076922,0.738461538461538,0.753846153846153,0.769230769230768,
0.784615384615384,0.799999999999999,0.815384615384614,0.83076923076923,
0.846153846153845,0.86153846153846,0.876923076923076,0.892307692307691,
0.907692307692306,0.923076923076922,0.938461538461537,0.953846153846152,
0.969230769230768,0.984615384615383,0.994228156739711),.UNSPECIFIED.)
CURVE()
GEOMETRIC_REPRESENTATION_ITEM()
RATIONAL_B_SPLINE_CURVE((1.,1.,1.,1.,1.,1.,1.,1.,1.,1.,1.,1.,1.,1.,1.,1.,
1.,1.,1.,1.,1.,1.,1.,1.,1.,1.,1.,1.,1.,1.,1.,1.,1.,1.,1.,1.,1.,1.,1.,1.,
1.,1.,1.,1.,1.,1.,1.,1.,1.,1.,1.,1.,1.,1.,1.,1.,1.,1.,1.,1.,1.,1.,1.,1.,
1.,1.,1.,1.,1.,1.))
REPRESENTATION_ITEM('')
);
#271=(
BOUNDED_CURVE()
B_SPLINE_CURVE(5,(#38495,#38496,#38497,#38498,#38499,#38500,#38501,#38502,
#38503,#38504,#38505,#38506,#38507,#38508,#38509,#38510,#38511,#38512,#38513,
#38514,#38515,#38516,#38517,#38518,#38519,#38520,#38521,#38522,#38523,#38524,
#38525,#38526,#38527,#38528,#38529,#38530,#38531,#38532,#38533,#38534,#38535,
#38536,#38537,#38538,#38539,#38540,#38541,#38542,#38543,#38544,#38545,#38546,
#38547,#38548,#38549,#38550,#38551,#38552,#38553,#38554,#38555,#38556,#38557,
#38558,#38559,#38560,#38561,#38562,#38563,#38564),.UNSPECIFIED.,.F.,.F.)
B_SPLINE_CURVE_WITH_KNOTS((6,1,1,1,1,1,1,1,1,1,1,1,1,1,1,1,1,1,1,1,1,1,
1,1,1,1,1,1,1,1,1,1,1,1,1,1,1,1,1,1,1,1,1,1,1,1,1,1,1,1,1,1,1,1,1,1,1,1,
1,1,1,1,1,1,1,6),(0.00577184337449159,0.0153846153846154,0.0307692307692308,
0.0461538461538462,0.0615384615384615,0.0769230769230769,0.0923076923076923,
0.107692307692308,0.123076923076923,0.138461538461538,0.153846153846154,
0.169230769230769,0.184615384615385,0.2,0.215384615384615,0.230769230769231,
0.246153846153846,0.261538461538462,0.276923076923077,0.292307692307692,
0.307692307692308,0.323076923076923,0.338461538461538,0.353846153846154,
0.369230769230769,0.384615384615385,0.4,0.415384615384615,0.430769230769231,
0.446153846153846,0.461538461538462,0.476923076923077,0.492307692307692,
0.507692307692308,0.523076923076923,0.538461538461538,0.553846153846154,
0.569230769230769,0.584615384615384,0.6,0.615384615384615,0.63076923076923,
0.646153846153846,0.661538461538461,0.676923076923076,0.692307692307692,
0.707692307692307,0.723076923076922,0.738461538461538,0.753846153846153,
0.769230769230768,0.784615384615384,0.799999999999999,0.815384615384614,
0.83076923076923,0.846153846153845,0.86153846153846,0.876923076923076,0.892307692307691,
0.907692307692306,0.923076923076922,0.938461538461537,0.953846153846152,
0.969230769230768,0.984615384615383,1.),.UNSPECIFIED.)
CURVE()
GEOMETRIC_REPRESENTATION_ITEM()
RATIONAL_B_SPLINE_CURVE((1.,1.,1.,1.,1.,1.,1.,1.,1.,1.,1.,1.,1.,1.,1.,1.,
1.,1.,1.,1.,1.,1.,1.,1.,1.,1.,1.,1.,1.,1.,1.,1.,1.,1.,1.,1.,1.,1.,1.,1.,
1.,1.,1.,1.,1.,1.,1.,1.,1.,1.,1.,1.,1.,1.,1.,1.,1.,1.,1.,1.,1.,1.,1.,1.,
1.,1.,1.,1.,1.,1.))
REPRESENTATION_ITEM('')
);
#272=(
BOUNDED_CURVE()
B_SPLINE_CURVE(5,(#38568,#38569,#38570,#38571,#38572,#38573,#38574,#38575,
#38576,#38577,#38578,#38579,#38580,#38581,#38582,#38583,#38584,#38585,#38586,
#38587,#38588,#38589,#38590,#38591,#38592,#38593,#38594,#38595,#38596,#38597,
#38598,#38599,#38600,#38601,#38602,#38603,#38604,#38605,#38606,#38607,#38608,
#38609,#38610,#38611,#38612,#38613,#38614,#38615,#38616,#38617,#38618,#38619,
#38620,#38621,#38622,#38623,#38624,#38625,#38626,#38627,#38628,#38629,#38630,
#38631,#38632,#38633,#38634,#38635,#38636,#38637),.UNSPECIFIED.,.F.,.F.)
B_SPLINE_CURVE_WITH_KNOTS((6,1,1,1,1,1,1,1,1,1,1,1,1,1,1,1,1,1,1,1,1,1,
1,1,1,1,1,1,1,1,1,1,1,1,1,1,1,1,1,1,1,1,1,1,1,1,1,1,1,1,1,1,1,1,1,1,1,1,
1,1,1,1,1,1,1,6),(0.,0.0153846153846154,0.0307692307692308,0.0461538461538462,
0.0615384615384615,0.0769230769230769,0.0923076923076923,0.107692307692308,
0.123076923076923,0.138461538461538,0.153846153846154,0.169230769230769,
0.184615384615385,0.2,0.215384615384615,0.230769230769231,0.246153846153846,
0.261538461538462,0.276923076923077,0.292307692307692,0.307692307692308,
0.323076923076923,0.338461538461538,0.353846153846154,0.369230769230769,
0.384615384615385,0.4,0.415384615384615,0.430769230769231,0.446153846153846,
0.461538461538462,0.476923076923077,0.492307692307692,0.507692307692308,
0.523076923076923,0.538461538461538,0.553846153846154,0.569230769230769,
0.584615384615384,0.6,0.615384615384615,0.63076923076923,0.646153846153846,
0.661538461538461,0.676923076923076,0.692307692307692,0.707692307692307,
0.723076923076922,0.738461538461538,0.753846153846153,0.769230769230768,
0.784615384615384,0.799999999999999,0.815384615384614,0.83076923076923,
0.846153846153845,0.86153846153846,0.876923076923076,0.892307692307691,
0.907692307692306,0.923076923076922,0.938461538461537,0.953846153846152,
0.969230769230768,0.984615384615383,0.994228156739723),.UNSPECIFIED.)
CURVE()
GEOMETRIC_REPRESENTATION_ITEM()
RATIONAL_B_SPLINE_CURVE((1.,1.,1.,1.,1.,1.,1.,1.,1.,1.,1.,1.,1.,1.,1.,1.,
1.,1.,1.,1.,1.,1.,1.,1.,1.,1.,1.,1.,1.,1.,1.,1.,1.,1.,1.,1.,1.,1.,1.,1.,
1.,1.,1.,1.,1.,1.,1.,1.,1.,1.,1.,1.,1.,1.,1.,1.,1.,1.,1.,1.,1.,1.,1.,1.,
1.,1.,1.,1.,1.,1.))
REPRESENTATION_ITEM('')
);
#273=(
BOUNDED_CURVE()
B_SPLINE_CURVE(5,(#38641,#38642,#38643,#38644,#38645,#38646,#38647,#38648,
#38649,#38650,#38651,#38652,#38653,#38654,#38655,#38656,#38657,#38658,#38659,
#38660,#38661,#38662,#38663,#38664,#38665,#38666,#38667,#38668,#38669,#38670,
#38671,#38672,#38673,#38674,#38675,#38676,#38677,#38678,#38679,#38680,#38681,
#38682,#38683,#38684,#38685,#38686,#38687,#38688,#38689,#38690,#38691,#38692,
#38693,#38694,#38695,#38696,#38697,#38698,#38699,#38700,#38701,#38702,#38703,
#38704,#38705,#38706,#38707,#38708,#38709,#38710),.UNSPECIFIED.,.F.,.F.)
B_SPLINE_CURVE_WITH_KNOTS((6,1,1,1,1,1,1,1,1,1,1,1,1,1,1,1,1,1,1,1,1,1,
1,1,1,1,1,1,1,1,1,1,1,1,1,1,1,1,1,1,1,1,1,1,1,1,1,1,1,1,1,1,1,1,1,1,1,1,
1,1,1,1,1,1,1,6),(0.00577184337450718,0.0153846153846154,0.0307692307692308,
0.0461538461538462,0.0615384615384615,0.0769230769230769,0.0923076923076923,
0.107692307692308,0.123076923076923,0.138461538461538,0.153846153846154,
0.169230769230769,0.184615384615385,0.2,0.215384615384615,0.230769230769231,
0.246153846153846,0.261538461538462,0.276923076923077,0.292307692307692,
0.307692307692308,0.323076923076923,0.338461538461538,0.353846153846154,
0.369230769230769,0.384615384615385,0.4,0.415384615384615,0.430769230769231,
0.446153846153846,0.461538461538462,0.476923076923077,0.492307692307692,
0.507692307692308,0.523076923076923,0.538461538461538,0.553846153846154,
0.569230769230769,0.584615384615384,0.6,0.615384615384615,0.63076923076923,
0.646153846153846,0.661538461538461,0.676923076923076,0.692307692307692,
0.707692307692307,0.723076923076922,0.738461538461538,0.753846153846153,
0.769230769230768,0.784615384615384,0.799999999999999,0.815384615384614,
0.83076923076923,0.846153846153845,0.86153846153846,0.876923076923076,0.892307692307691,
0.907692307692306,0.923076923076922,0.938461538461537,0.953846153846152,
0.969230769230768,0.984615384615383,1.),.UNSPECIFIED.)
CURVE()
GEOMETRIC_REPRESENTATION_ITEM()
RATIONAL_B_SPLINE_CURVE((1.,1.,1.,1.,1.,1.,1.,1.,1.,1.,1.,1.,1.,1.,1.,1.,
1.,1.,1.,1.,1.,1.,1.,1.,1.,1.,1.,1.,1.,1.,1.,1.,1.,1.,1.,1.,1.,1.,1.,1.,
1.,1.,1.,1.,1.,1.,1.,1.,1.,1.,1.,1.,1.,1.,1.,1.,1.,1.,1.,1.,1.,1.,1.,1.,
1.,1.,1.,1.,1.,1.))
REPRESENTATION_ITEM('')
);
#274=(
BOUNDED_CURVE()
B_SPLINE_CURVE(5,(#38714,#38715,#38716,#38717,#38718,#38719,#38720,#38721,
#38722,#38723,#38724,#38725,#38726,#38727,#38728,#38729,#38730,#38731,#38732,
#38733,#38734,#38735,#38736,#38737,#38738,#38739,#38740,#38741,#38742,#38743,
#38744,#38745,#38746,#38747,#38748,#38749,#38750,#38751,#38752,#38753,#38754,
#38755,#38756,#38757,#38758,#38759,#38760,#38761,#38762,#38763,#38764,#38765,
#38766,#38767,#38768,#38769,#38770,#38771,#38772,#38773,#38774,#38775,#38776,
#38777,#38778,#38779,#38780,#38781,#38782,#38783),.UNSPECIFIED.,.F.,.F.)
B_SPLINE_CURVE_WITH_KNOTS((6,1,1,1,1,1,1,1,1,1,1,1,1,1,1,1,1,1,1,1,1,1,
1,1,1,1,1,1,1,1,1,1,1,1,1,1,1,1,1,1,1,1,1,1,1,1,1,1,1,1,1,1,1,1,1,1,1,1,
1,1,1,1,1,1,1,6),(0.,0.0153846153846154,0.0307692307692308,0.0461538461538462,
0.0615384615384615,0.0769230769230769,0.0923076923076923,0.107692307692308,
0.123076923076923,0.138461538461538,0.153846153846154,0.169230769230769,
0.184615384615385,0.2,0.215384615384615,0.230769230769231,0.246153846153846,
0.261538461538462,0.276923076923077,0.292307692307692,0.307692307692308,
0.323076923076923,0.338461538461538,0.353846153846154,0.369230769230769,
0.384615384615385,0.4,0.415384615384615,0.430769230769231,0.446153846153846,
0.461538461538462,0.476923076923077,0.492307692307692,0.507692307692308,
0.523076923076923,0.538461538461538,0.553846153846154,0.569230769230769,
0.584615384615384,0.6,0.615384615384615,0.63076923076923,0.646153846153846,
0.661538461538461,0.676923076923076,0.692307692307692,0.707692307692307,
0.723076923076922,0.738461538461538,0.753846153846153,0.769230769230768,
0.784615384615384,0.799999999999999,0.815384615384614,0.83076923076923,
0.846153846153845,0.86153846153846,0.876923076923076,0.892307692307691,
0.907692307692306,0.923076923076922,0.938461538461537,0.953846153846152,
0.969230769230768,0.984615384615383,0.994228156739716),.UNSPECIFIED.)
CURVE()
GEOMETRIC_REPRESENTATION_ITEM()
RATIONAL_B_SPLINE_CURVE((1.,1.,1.,1.,1.,1.,1.,1.,1.,1.,1.,1.,1.,1.,1.,1.,
1.,1.,1.,1.,1.,1.,1.,1.,1.,1.,1.,1.,1.,1.,1.,1.,1.,1.,1.,1.,1.,1.,1.,1.,
1.,1.,1.,1.,1.,1.,1.,1.,1.,1.,1.,1.,1.,1.,1.,1.,1.,1.,1.,1.,1.,1.,1.,1.,
1.,1.,1.,1.,1.,1.))
REPRESENTATION_ITEM('')
);
#275=(
BOUNDED_CURVE()
B_SPLINE_CURVE(5,(#38787,#38788,#38789,#38790,#38791,#38792,#38793,#38794,
#38795,#38796,#38797,#38798,#38799,#38800,#38801,#38802,#38803,#38804,#38805,
#38806,#38807,#38808,#38809,#38810,#38811,#38812,#38813,#38814,#38815,#38816,
#38817,#38818,#38819,#38820,#38821,#38822,#38823,#38824,#38825,#38826,#38827,
#38828,#38829,#38830,#38831,#38832,#38833,#38834,#38835,#38836,#38837,#38838,
#38839,#38840,#38841,#38842,#38843,#38844,#38845,#38846,#38847,#38848,#38849,
#38850,#38851,#38852,#38853,#38854,#38855,#38856),.UNSPECIFIED.,.F.,.F.)
B_SPLINE_CURVE_WITH_KNOTS((6,1,1,1,1,1,1,1,1,1,1,1,1,1,1,1,1,1,1,1,1,1,
1,1,1,1,1,1,1,1,1,1,1,1,1,1,1,1,1,1,1,1,1,1,1,1,1,1,1,1,1,1,1,1,1,1,1,1,
1,1,1,1,1,1,1,6),(0.00577184337450174,0.0153846153846154,0.0307692307692308,
0.0461538461538462,0.0615384615384615,0.0769230769230769,0.0923076923076923,
0.107692307692308,0.123076923076923,0.138461538461538,0.153846153846154,
0.169230769230769,0.184615384615385,0.2,0.215384615384615,0.230769230769231,
0.246153846153846,0.261538461538462,0.276923076923077,0.292307692307692,
0.307692307692308,0.323076923076923,0.338461538461538,0.353846153846154,
0.369230769230769,0.384615384615385,0.4,0.415384615384615,0.430769230769231,
0.446153846153846,0.461538461538462,0.476923076923077,0.492307692307692,
0.507692307692308,0.523076923076923,0.538461538461538,0.553846153846154,
0.569230769230769,0.584615384615384,0.6,0.615384615384615,0.63076923076923,
0.646153846153846,0.661538461538461,0.676923076923076,0.692307692307692,
0.707692307692307,0.723076923076922,0.738461538461538,0.753846153846153,
0.769230769230768,0.784615384615384,0.799999999999999,0.815384615384614,
0.83076923076923,0.846153846153845,0.86153846153846,0.876923076923076,0.892307692307691,
0.907692307692306,0.923076923076922,0.938461538461537,0.953846153846152,
0.969230769230768,0.984615384615383,1.),.UNSPECIFIED.)
CURVE()
GEOMETRIC_REPRESENTATION_ITEM()
RATIONAL_B_SPLINE_CURVE((1.,1.,1.,1.,1.,1.,1.,1.,1.,1.,1.,1.,1.,1.,1.,1.,
1.,1.,1.,1.,1.,1.,1.,1.,1.,1.,1.,1.,1.,1.,1.,1.,1.,1.,1.,1.,1.,1.,1.,1.,
1.,1.,1.,1.,1.,1.,1.,1.,1.,1.,1.,1.,1.,1.,1.,1.,1.,1.,1.,1.,1.,1.,1.,1.,
1.,1.,1.,1.,1.,1.))
REPRESENTATION_ITEM('')
);
#276=(
BOUNDED_CURVE()
B_SPLINE_CURVE(5,(#38860,#38861,#38862,#38863,#38864,#38865,#38866,#38867,
#38868,#38869,#38870,#38871,#38872,#38873,#38874,#38875,#38876,#38877,#38878,
#38879,#38880,#38881,#38882,#38883,#38884,#38885,#38886,#38887,#38888,#38889,
#38890,#38891,#38892,#38893,#38894,#38895,#38896,#38897,#38898,#38899,#38900,
#38901,#38902,#38903,#38904,#38905,#38906,#38907,#38908,#38909,#38910,#38911,
#38912,#38913,#38914,#38915,#38916,#38917,#38918,#38919,#38920,#38921,#38922,
#38923,#38924,#38925,#38926,#38927,#38928,#38929),.UNSPECIFIED.,.F.,.F.)
B_SPLINE_CURVE_WITH_KNOTS((6,1,1,1,1,1,1,1,1,1,1,1,1,1,1,1,1,1,1,1,1,1,
1,1,1,1,1,1,1,1,1,1,1,1,1,1,1,1,1,1,1,1,1,1,1,1,1,1,1,1,1,1,1,1,1,1,1,1,
1,1,1,1,1,1,1,6),(0.,0.0153846153846154,0.0307692307692308,0.0461538461538462,
0.0615384615384615,0.0769230769230769,0.0923076923076923,0.107692307692308,
0.123076923076923,0.138461538461538,0.153846153846154,0.169230769230769,
0.184615384615385,0.2,0.215384615384615,0.230769230769231,0.246153846153846,
0.261538461538462,0.276923076923077,0.292307692307692,0.307692307692308,
0.323076923076923,0.338461538461538,0.353846153846154,0.369230769230769,
0.384615384615385,0.4,0.415384615384615,0.430769230769231,0.446153846153846,
0.461538461538462,0.476923076923077,0.492307692307692,0.507692307692308,
0.523076923076923,0.538461538461538,0.553846153846154,0.569230769230769,
0.584615384615384,0.6,0.615384615384615,0.63076923076923,0.646153846153846,
0.661538461538461,0.676923076923076,0.692307692307692,0.707692307692307,
0.723076923076922,0.738461538461538,0.753846153846153,0.769230769230768,
0.784615384615384,0.799999999999999,0.815384615384614,0.83076923076923,
0.846153846153845,0.86153846153846,0.876923076923076,0.892307692307691,
0.907692307692306,0.923076923076922,0.938461538461537,0.953846153846152,
0.969230769230768,0.984615384615383,0.994228156739722),.UNSPECIFIED.)
CURVE()
GEOMETRIC_REPRESENTATION_ITEM()
RATIONAL_B_SPLINE_CURVE((1.,1.,1.,1.,1.,1.,1.,1.,1.,1.,1.,1.,1.,1.,1.,1.,
1.,1.,1.,1.,1.,1.,1.,1.,1.,1.,1.,1.,1.,1.,1.,1.,1.,1.,1.,1.,1.,1.,1.,1.,
1.,1.,1.,1.,1.,1.,1.,1.,1.,1.,1.,1.,1.,1.,1.,1.,1.,1.,1.,1.,1.,1.,1.,1.,
1.,1.,1.,1.,1.,1.))
REPRESENTATION_ITEM('')
);
#277=(
BOUNDED_CURVE()
B_SPLINE_CURVE(5,(#38933,#38934,#38935,#38936,#38937,#38938,#38939,#38940,
#38941,#38942,#38943,#38944,#38945,#38946,#38947,#38948,#38949,#38950,#38951,
#38952,#38953,#38954,#38955,#38956,#38957,#38958,#38959,#38960,#38961,#38962,
#38963,#38964,#38965,#38966,#38967,#38968,#38969,#38970,#38971,#38972,#38973,
#38974,#38975,#38976,#38977,#38978,#38979,#38980,#38981,#38982,#38983,#38984,
#38985,#38986,#38987,#38988,#38989,#38990,#38991,#38992,#38993,#38994,#38995,
#38996,#38997,#38998,#38999,#39000,#39001,#39002),.UNSPECIFIED.,.F.,.F.)
B_SPLINE_CURVE_WITH_KNOTS((6,1,1,1,1,1,1,1,1,1,1,1,1,1,1,1,1,1,1,1,1,1,
1,1,1,1,1,1,1,1,1,1,1,1,1,1,1,1,1,1,1,1,1,1,1,1,1,1,1,1,1,1,1,1,1,1,1,1,
1,1,1,1,1,1,1,6),(0.00577184337450943,0.0153846153846154,0.0307692307692308,
0.0461538461538462,0.0615384615384615,0.0769230769230769,0.0923076923076923,
0.107692307692308,0.123076923076923,0.138461538461538,0.153846153846154,
0.169230769230769,0.184615384615385,0.2,0.215384615384615,0.230769230769231,
0.246153846153846,0.261538461538462,0.276923076923077,0.292307692307692,
0.307692307692308,0.323076923076923,0.338461538461538,0.353846153846154,
0.369230769230769,0.384615384615385,0.4,0.415384615384615,0.430769230769231,
0.446153846153846,0.461538461538462,0.476923076923077,0.492307692307692,
0.507692307692308,0.523076923076923,0.538461538461538,0.553846153846154,
0.569230769230769,0.584615384615384,0.6,0.615384615384615,0.63076923076923,
0.646153846153846,0.661538461538461,0.676923076923076,0.692307692307692,
0.707692307692307,0.723076923076922,0.738461538461538,0.753846153846153,
0.769230769230768,0.784615384615384,0.799999999999999,0.815384615384614,
0.83076923076923,0.846153846153845,0.86153846153846,0.876923076923076,0.892307692307691,
0.907692307692306,0.923076923076922,0.938461538461537,0.953846153846152,
0.969230769230768,0.984615384615383,1.),.UNSPECIFIED.)
CURVE()
GEOMETRIC_REPRESENTATION_ITEM()
RATIONAL_B_SPLINE_CURVE((1.,1.,1.,1.,1.,1.,1.,1.,1.,1.,1.,1.,1.,1.,1.,1.,
1.,1.,1.,1.,1.,1.,1.,1.,1.,1.,1.,1.,1.,1.,1.,1.,1.,1.,1.,1.,1.,1.,1.,1.,
1.,1.,1.,1.,1.,1.,1.,1.,1.,1.,1.,1.,1.,1.,1.,1.,1.,1.,1.,1.,1.,1.,1.,1.,
1.,1.,1.,1.,1.,1.))
REPRESENTATION_ITEM('')
);
#278=(
BOUNDED_CURVE()
B_SPLINE_CURVE(5,(#39006,#39007,#39008,#39009,#39010,#39011,#39012,#39013,
#39014,#39015,#39016,#39017,#39018,#39019,#39020,#39021,#39022,#39023,#39024,
#39025,#39026,#39027,#39028,#39029,#39030,#39031,#39032,#39033,#39034,#39035,
#39036,#39037,#39038,#39039,#39040,#39041,#39042,#39043,#39044,#39045,#39046,
#39047,#39048,#39049,#39050,#39051,#39052,#39053,#39054,#39055,#39056,#39057,
#39058,#39059,#39060,#39061,#39062,#39063,#39064,#39065,#39066,#39067,#39068,
#39069,#39070,#39071,#39072,#39073,#39074,#39075),.UNSPECIFIED.,.F.,.F.)
B_SPLINE_CURVE_WITH_KNOTS((6,1,1,1,1,1,1,1,1,1,1,1,1,1,1,1,1,1,1,1,1,1,
1,1,1,1,1,1,1,1,1,1,1,1,1,1,1,1,1,1,1,1,1,1,1,1,1,1,1,1,1,1,1,1,1,1,1,1,
1,1,1,1,1,1,1,6),(0.,0.0153846153846154,0.0307692307692308,0.0461538461538462,
0.0615384615384615,0.0769230769230769,0.0923076923076923,0.107692307692308,
0.123076923076923,0.138461538461538,0.153846153846154,0.169230769230769,
0.184615384615385,0.2,0.215384615384615,0.230769230769231,0.246153846153846,
0.261538461538462,0.276923076923077,0.292307692307692,0.307692307692308,
0.323076923076923,0.338461538461538,0.353846153846154,0.369230769230769,
0.384615384615385,0.4,0.415384615384615,0.430769230769231,0.446153846153846,
0.461538461538462,0.476923076923077,0.492307692307692,0.507692307692308,
0.523076923076923,0.538461538461538,0.553846153846154,0.569230769230769,
0.584615384615384,0.6,0.615384615384615,0.63076923076923,0.646153846153846,
0.661538461538461,0.676923076923076,0.692307692307692,0.707692307692307,
0.723076923076922,0.738461538461538,0.753846153846153,0.769230769230768,
0.784615384615384,0.799999999999999,0.815384615384614,0.83076923076923,
0.846153846153845,0.86153846153846,0.876923076923076,0.892307692307691,
0.907692307692306,0.923076923076922,0.938461538461537,0.953846153846152,
0.969230769230768,0.984615384615383,0.994228156739699),.UNSPECIFIED.)
CURVE()
GEOMETRIC_REPRESENTATION_ITEM()
RATIONAL_B_SPLINE_CURVE((1.,1.,1.,1.,1.,1.,1.,1.,1.,1.,1.,1.,1.,1.,1.,1.,
1.,1.,1.,1.,1.,1.,1.,1.,1.,1.,1.,1.,1.,1.,1.,1.,1.,1.,1.,1.,1.,1.,1.,1.,
1.,1.,1.,1.,1.,1.,1.,1.,1.,1.,1.,1.,1.,1.,1.,1.,1.,1.,1.,1.,1.,1.,1.,1.,
1.,1.,1.,1.,1.,1.))
REPRESENTATION_ITEM('')
);
#279=(
BOUNDED_CURVE()
B_SPLINE_CURVE(5,(#39079,#39080,#39081,#39082,#39083,#39084,#39085,#39086,
#39087,#39088,#39089,#39090,#39091,#39092,#39093,#39094,#39095,#39096,#39097,
#39098,#39099,#39100,#39101,#39102,#39103,#39104,#39105,#39106,#39107,#39108,
#39109,#39110,#39111,#39112,#39113,#39114,#39115,#39116,#39117,#39118,#39119,
#39120,#39121,#39122,#39123,#39124,#39125,#39126,#39127,#39128,#39129,#39130,
#39131,#39132,#39133,#39134,#39135,#39136,#39137,#39138,#39139,#39140,#39141,
#39142,#39143,#39144,#39145,#39146,#39147,#39148),.UNSPECIFIED.,.F.,.F.)
B_SPLINE_CURVE_WITH_KNOTS((6,1,1,1,1,1,1,1,1,1,1,1,1,1,1,1,1,1,1,1,1,1,
1,1,1,1,1,1,1,1,1,1,1,1,1,1,1,1,1,1,1,1,1,1,1,1,1,1,1,1,1,1,1,1,1,1,1,1,
1,1,1,1,1,1,1,6),(0.00577184337450665,0.0153846153846154,0.0307692307692308,
0.0461538461538462,0.0615384615384615,0.0769230769230769,0.0923076923076923,
0.107692307692308,0.123076923076923,0.138461538461538,0.153846153846154,
0.169230769230769,0.184615384615385,0.2,0.215384615384615,0.230769230769231,
0.246153846153846,0.261538461538462,0.276923076923077,0.292307692307692,
0.307692307692308,0.323076923076923,0.338461538461538,0.353846153846154,
0.369230769230769,0.384615384615385,0.4,0.415384615384615,0.430769230769231,
0.446153846153846,0.461538461538462,0.476923076923077,0.492307692307692,
0.507692307692308,0.523076923076923,0.538461538461538,0.553846153846154,
0.569230769230769,0.584615384615384,0.6,0.615384615384615,0.63076923076923,
0.646153846153846,0.661538461538461,0.676923076923076,0.692307692307692,
0.707692307692307,0.723076923076922,0.738461538461538,0.753846153846153,
0.769230769230768,0.784615384615384,0.799999999999999,0.815384615384614,
0.83076923076923,0.846153846153845,0.86153846153846,0.876923076923076,0.892307692307691,
0.907692307692306,0.923076923076922,0.938461538461537,0.953846153846152,
0.969230769230768,0.984615384615383,1.),.UNSPECIFIED.)
CURVE()
GEOMETRIC_REPRESENTATION_ITEM()
RATIONAL_B_SPLINE_CURVE((1.,1.,1.,1.,1.,1.,1.,1.,1.,1.,1.,1.,1.,1.,1.,1.,
1.,1.,1.,1.,1.,1.,1.,1.,1.,1.,1.,1.,1.,1.,1.,1.,1.,1.,1.,1.,1.,1.,1.,1.,
1.,1.,1.,1.,1.,1.,1.,1.,1.,1.,1.,1.,1.,1.,1.,1.,1.,1.,1.,1.,1.,1.,1.,1.,
1.,1.,1.,1.,1.,1.))
REPRESENTATION_ITEM('')
);
#280=(
BOUNDED_CURVE()
B_SPLINE_CURVE(5,(#39152,#39153,#39154,#39155,#39156,#39157,#39158,#39159,
#39160,#39161,#39162,#39163,#39164,#39165,#39166,#39167,#39168,#39169,#39170,
#39171,#39172,#39173,#39174,#39175,#39176,#39177,#39178,#39179,#39180,#39181,
#39182,#39183,#39184,#39185,#39186,#39187,#39188,#39189,#39190,#39191,#39192,
#39193,#39194,#39195,#39196,#39197,#39198,#39199,#39200,#39201,#39202,#39203,
#39204,#39205,#39206,#39207,#39208,#39209,#39210,#39211,#39212,#39213,#39214,
#39215,#39216,#39217,#39218,#39219,#39220,#39221),.UNSPECIFIED.,.F.,.F.)
B_SPLINE_CURVE_WITH_KNOTS((6,1,1,1,1,1,1,1,1,1,1,1,1,1,1,1,1,1,1,1,1,1,
1,1,1,1,1,1,1,1,1,1,1,1,1,1,1,1,1,1,1,1,1,1,1,1,1,1,1,1,1,1,1,1,1,1,1,1,
1,1,1,1,1,1,1,6),(0.,0.0153846153846154,0.0307692307692308,0.0461538461538462,
0.0615384615384615,0.0769230769230769,0.0923076923076923,0.107692307692308,
0.123076923076923,0.138461538461538,0.153846153846154,0.169230769230769,
0.184615384615385,0.2,0.215384615384615,0.230769230769231,0.246153846153846,
0.261538461538462,0.276923076923077,0.292307692307692,0.307692307692308,
0.323076923076923,0.338461538461538,0.353846153846154,0.369230769230769,
0.384615384615385,0.4,0.415384615384615,0.430769230769231,0.446153846153846,
0.461538461538462,0.476923076923077,0.492307692307692,0.507692307692308,
0.523076923076923,0.538461538461538,0.553846153846154,0.569230769230769,
0.584615384615384,0.6,0.615384615384615,0.63076923076923,0.646153846153846,
0.661538461538461,0.676923076923076,0.692307692307692,0.707692307692307,
0.723076923076922,0.738461538461538,0.753846153846153,0.769230769230768,
0.784615384615384,0.799999999999999,0.815384615384614,0.83076923076923,
0.846153846153845,0.86153846153846,0.876923076923076,0.892307692307691,
0.907692307692306,0.923076923076922,0.938461538461537,0.953846153846152,
0.969230769230768,0.984615384615383,0.994228156739691),.UNSPECIFIED.)
CURVE()
GEOMETRIC_REPRESENTATION_ITEM()
RATIONAL_B_SPLINE_CURVE((1.,1.,1.,1.,1.,1.,1.,1.,1.,1.,1.,1.,1.,1.,1.,1.,
1.,1.,1.,1.,1.,1.,1.,1.,1.,1.,1.,1.,1.,1.,1.,1.,1.,1.,1.,1.,1.,1.,1.,1.,
1.,1.,1.,1.,1.,1.,1.,1.,1.,1.,1.,1.,1.,1.,1.,1.,1.,1.,1.,1.,1.,1.,1.,1.,
1.,1.,1.,1.,1.,1.))
REPRESENTATION_ITEM('')
);
#281=(
BOUNDED_CURVE()
B_SPLINE_CURVE(5,(#39225,#39226,#39227,#39228,#39229,#39230,#39231,#39232,
#39233,#39234,#39235,#39236,#39237,#39238,#39239,#39240,#39241,#39242,#39243,
#39244,#39245,#39246,#39247,#39248,#39249,#39250,#39251,#39252,#39253,#39254,
#39255,#39256,#39257,#39258,#39259,#39260,#39261,#39262,#39263,#39264,#39265,
#39266,#39267,#39268,#39269,#39270,#39271,#39272,#39273,#39274,#39275,#39276,
#39277,#39278,#39279,#39280,#39281,#39282,#39283,#39284,#39285,#39286,#39287,
#39288,#39289,#39290,#39291,#39292,#39293,#39294),.UNSPECIFIED.,.F.,.F.)
B_SPLINE_CURVE_WITH_KNOTS((6,1,1,1,1,1,1,1,1,1,1,1,1,1,1,1,1,1,1,1,1,1,
1,1,1,1,1,1,1,1,1,1,1,1,1,1,1,1,1,1,1,1,1,1,1,1,1,1,1,1,1,1,1,1,1,1,1,1,
1,1,1,1,1,1,1,6),(0.00577184337450785,0.0153846153846154,0.0307692307692308,
0.0461538461538462,0.0615384615384615,0.0769230769230769,0.0923076923076923,
0.107692307692308,0.123076923076923,0.138461538461538,0.153846153846154,
0.169230769230769,0.184615384615385,0.2,0.215384615384615,0.230769230769231,
0.246153846153846,0.261538461538462,0.276923076923077,0.292307692307692,
0.307692307692308,0.323076923076923,0.338461538461538,0.353846153846154,
0.369230769230769,0.384615384615385,0.4,0.415384615384615,0.430769230769231,
0.446153846153846,0.461538461538462,0.476923076923077,0.492307692307692,
0.507692307692308,0.523076923076923,0.538461538461538,0.553846153846154,
0.569230769230769,0.584615384615384,0.6,0.615384615384615,0.63076923076923,
0.646153846153846,0.661538461538461,0.676923076923076,0.692307692307692,
0.707692307692307,0.723076923076922,0.738461538461538,0.753846153846153,
0.769230769230768,0.784615384615384,0.799999999999999,0.815384615384614,
0.83076923076923,0.846153846153845,0.86153846153846,0.876923076923076,0.892307692307691,
0.907692307692306,0.923076923076922,0.938461538461537,0.953846153846152,
0.969230769230768,0.984615384615383,1.),.UNSPECIFIED.)
CURVE()
GEOMETRIC_REPRESENTATION_ITEM()
RATIONAL_B_SPLINE_CURVE((1.,1.,1.,1.,1.,1.,1.,1.,1.,1.,1.,1.,1.,1.,1.,1.,
1.,1.,1.,1.,1.,1.,1.,1.,1.,1.,1.,1.,1.,1.,1.,1.,1.,1.,1.,1.,1.,1.,1.,1.,
1.,1.,1.,1.,1.,1.,1.,1.,1.,1.,1.,1.,1.,1.,1.,1.,1.,1.,1.,1.,1.,1.,1.,1.,
1.,1.,1.,1.,1.,1.))
REPRESENTATION_ITEM('')
);
#282=(
BOUNDED_CURVE()
B_SPLINE_CURVE(5,(#39298,#39299,#39300,#39301,#39302,#39303,#39304,#39305,
#39306,#39307,#39308,#39309,#39310,#39311,#39312,#39313,#39314,#39315,#39316,
#39317,#39318,#39319,#39320,#39321,#39322,#39323,#39324,#39325,#39326,#39327,
#39328,#39329,#39330,#39331,#39332,#39333,#39334,#39335,#39336,#39337,#39338,
#39339,#39340,#39341,#39342,#39343,#39344,#39345,#39346,#39347,#39348,#39349,
#39350,#39351,#39352,#39353,#39354,#39355,#39356,#39357,#39358,#39359,#39360,
#39361,#39362,#39363,#39364,#39365,#39366,#39367),.UNSPECIFIED.,.F.,.F.)
B_SPLINE_CURVE_WITH_KNOTS((6,1,1,1,1,1,1,1,1,1,1,1,1,1,1,1,1,1,1,1,1,1,
1,1,1,1,1,1,1,1,1,1,1,1,1,1,1,1,1,1,1,1,1,1,1,1,1,1,1,1,1,1,1,1,1,1,1,1,
1,1,1,1,1,1,1,6),(0.,0.0153846153846154,0.0307692307692308,0.0461538461538462,
0.0615384615384615,0.0769230769230769,0.0923076923076923,0.107692307692308,
0.123076923076923,0.138461538461538,0.153846153846154,0.169230769230769,
0.184615384615385,0.2,0.215384615384615,0.230769230769231,0.246153846153846,
0.261538461538462,0.276923076923077,0.292307692307692,0.307692307692308,
0.323076923076923,0.338461538461538,0.353846153846154,0.369230769230769,
0.384615384615385,0.4,0.415384615384615,0.430769230769231,0.446153846153846,
0.461538461538462,0.476923076923077,0.492307692307692,0.507692307692308,
0.523076923076923,0.538461538461538,0.553846153846154,0.569230769230769,
0.584615384615384,0.6,0.615384615384615,0.63076923076923,0.646153846153846,
0.661538461538461,0.676923076923076,0.692307692307692,0.707692307692307,
0.723076923076922,0.738461538461538,0.753846153846153,0.769230769230768,
0.784615384615384,0.799999999999999,0.815384615384614,0.83076923076923,
0.846153846153845,0.86153846153846,0.876923076923076,0.892307692307691,
0.907692307692306,0.923076923076922,0.938461538461537,0.953846153846152,
0.969230769230768,0.984615384615383,0.994228156739708),.UNSPECIFIED.)
CURVE()
GEOMETRIC_REPRESENTATION_ITEM()
RATIONAL_B_SPLINE_CURVE((1.,1.,1.,1.,1.,1.,1.,1.,1.,1.,1.,1.,1.,1.,1.,1.,
1.,1.,1.,1.,1.,1.,1.,1.,1.,1.,1.,1.,1.,1.,1.,1.,1.,1.,1.,1.,1.,1.,1.,1.,
1.,1.,1.,1.,1.,1.,1.,1.,1.,1.,1.,1.,1.,1.,1.,1.,1.,1.,1.,1.,1.,1.,1.,1.,
1.,1.,1.,1.,1.,1.))
REPRESENTATION_ITEM('')
);
#283=(
BOUNDED_CURVE()
B_SPLINE_CURVE(5,(#39371,#39372,#39373,#39374,#39375,#39376,#39377,#39378,
#39379,#39380,#39381,#39382,#39383,#39384,#39385,#39386,#39387,#39388,#39389,
#39390,#39391,#39392,#39393,#39394,#39395,#39396,#39397,#39398,#39399,#39400,
#39401,#39402,#39403,#39404,#39405,#39406,#39407,#39408,#39409,#39410,#39411,
#39412,#39413,#39414,#39415,#39416,#39417,#39418,#39419,#39420,#39421,#39422,
#39423,#39424,#39425,#39426,#39427,#39428,#39429,#39430,#39431,#39432,#39433,
#39434,#39435,#39436,#39437,#39438,#39439,#39440),.UNSPECIFIED.,.F.,.F.)
B_SPLINE_CURVE_WITH_KNOTS((6,1,1,1,1,1,1,1,1,1,1,1,1,1,1,1,1,1,1,1,1,1,
1,1,1,1,1,1,1,1,1,1,1,1,1,1,1,1,1,1,1,1,1,1,1,1,1,1,1,1,1,1,1,1,1,1,1,1,
1,1,1,1,1,1,1,6),(0.00577184337450072,0.0153846153846154,0.0307692307692308,
0.0461538461538462,0.0615384615384615,0.0769230769230769,0.0923076923076923,
0.107692307692308,0.123076923076923,0.138461538461538,0.153846153846154,
0.169230769230769,0.184615384615385,0.2,0.215384615384615,0.230769230769231,
0.246153846153846,0.261538461538462,0.276923076923077,0.292307692307692,
0.307692307692308,0.323076923076923,0.338461538461538,0.353846153846154,
0.369230769230769,0.384615384615385,0.4,0.415384615384615,0.430769230769231,
0.446153846153846,0.461538461538462,0.476923076923077,0.492307692307692,
0.507692307692308,0.523076923076923,0.538461538461538,0.553846153846154,
0.569230769230769,0.584615384615384,0.6,0.615384615384615,0.63076923076923,
0.646153846153846,0.661538461538461,0.676923076923076,0.692307692307692,
0.707692307692307,0.723076923076922,0.738461538461538,0.753846153846153,
0.769230769230768,0.784615384615384,0.799999999999999,0.815384615384614,
0.83076923076923,0.846153846153845,0.86153846153846,0.876923076923076,0.892307692307691,
0.907692307692306,0.923076923076922,0.938461538461537,0.953846153846152,
0.969230769230768,0.984615384615383,1.),.UNSPECIFIED.)
CURVE()
GEOMETRIC_REPRESENTATION_ITEM()
RATIONAL_B_SPLINE_CURVE((1.,1.,1.,1.,1.,1.,1.,1.,1.,1.,1.,1.,1.,1.,1.,1.,
1.,1.,1.,1.,1.,1.,1.,1.,1.,1.,1.,1.,1.,1.,1.,1.,1.,1.,1.,1.,1.,1.,1.,1.,
1.,1.,1.,1.,1.,1.,1.,1.,1.,1.,1.,1.,1.,1.,1.,1.,1.,1.,1.,1.,1.,1.,1.,1.,
1.,1.,1.,1.,1.,1.))
REPRESENTATION_ITEM('')
);
#284=(
BOUNDED_CURVE()
B_SPLINE_CURVE(5,(#39444,#39445,#39446,#39447,#39448,#39449,#39450,#39451,
#39452,#39453,#39454,#39455,#39456,#39457,#39458,#39459,#39460,#39461,#39462,
#39463,#39464,#39465,#39466,#39467,#39468,#39469,#39470,#39471,#39472,#39473,
#39474,#39475,#39476,#39477,#39478,#39479,#39480,#39481,#39482,#39483,#39484,
#39485,#39486,#39487,#39488,#39489,#39490,#39491,#39492,#39493,#39494,#39495,
#39496,#39497,#39498,#39499,#39500,#39501,#39502,#39503,#39504,#39505,#39506,
#39507,#39508,#39509,#39510,#39511,#39512,#39513),.UNSPECIFIED.,.F.,.F.)
B_SPLINE_CURVE_WITH_KNOTS((6,1,1,1,1,1,1,1,1,1,1,1,1,1,1,1,1,1,1,1,1,1,
1,1,1,1,1,1,1,1,1,1,1,1,1,1,1,1,1,1,1,1,1,1,1,1,1,1,1,1,1,1,1,1,1,1,1,1,
1,1,1,1,1,1,1,6),(0.,0.0153846153846154,0.0307692307692308,0.0461538461538462,
0.0615384615384615,0.0769230769230769,0.0923076923076923,0.107692307692308,
0.123076923076923,0.138461538461538,0.153846153846154,0.169230769230769,
0.184615384615385,0.2,0.215384615384615,0.230769230769231,0.246153846153846,
0.261538461538462,0.276923076923077,0.292307692307692,0.307692307692308,
0.323076923076923,0.338461538461538,0.353846153846154,0.369230769230769,
0.384615384615385,0.4,0.415384615384615,0.430769230769231,0.446153846153846,
0.461538461538462,0.476923076923077,0.492307692307692,0.507692307692308,
0.523076923076923,0.538461538461538,0.553846153846154,0.569230769230769,
0.584615384615384,0.6,0.615384615384615,0.63076923076923,0.646153846153846,
0.661538461538461,0.676923076923076,0.692307692307692,0.707692307692307,
0.723076923076922,0.738461538461538,0.753846153846153,0.769230769230768,
0.784615384615384,0.799999999999999,0.815384615384614,0.83076923076923,
0.846153846153845,0.86153846153846,0.876923076923076,0.892307692307691,
0.907692307692306,0.923076923076922,0.938461538461537,0.953846153846152,
0.969230769230768,0.984615384615383,0.994228156739706),.UNSPECIFIED.)
CURVE()
GEOMETRIC_REPRESENTATION_ITEM()
RATIONAL_B_SPLINE_CURVE((1.,1.,1.,1.,1.,1.,1.,1.,1.,1.,1.,1.,1.,1.,1.,1.,
1.,1.,1.,1.,1.,1.,1.,1.,1.,1.,1.,1.,1.,1.,1.,1.,1.,1.,1.,1.,1.,1.,1.,1.,
1.,1.,1.,1.,1.,1.,1.,1.,1.,1.,1.,1.,1.,1.,1.,1.,1.,1.,1.,1.,1.,1.,1.,1.,
1.,1.,1.,1.,1.,1.))
REPRESENTATION_ITEM('')
);
#285=(
BOUNDED_CURVE()
B_SPLINE_CURVE(5,(#39517,#39518,#39519,#39520,#39521,#39522,#39523,#39524,
#39525,#39526,#39527,#39528,#39529,#39530,#39531,#39532,#39533,#39534,#39535,
#39536,#39537,#39538,#39539,#39540,#39541,#39542,#39543,#39544,#39545,#39546,
#39547,#39548,#39549,#39550,#39551,#39552,#39553,#39554,#39555,#39556,#39557,
#39558,#39559,#39560,#39561,#39562,#39563,#39564,#39565,#39566,#39567,#39568,
#39569,#39570,#39571,#39572,#39573,#39574,#39575,#39576,#39577,#39578,#39579,
#39580,#39581,#39582,#39583,#39584,#39585,#39586),.UNSPECIFIED.,.F.,.F.)
B_SPLINE_CURVE_WITH_KNOTS((6,1,1,1,1,1,1,1,1,1,1,1,1,1,1,1,1,1,1,1,1,1,
1,1,1,1,1,1,1,1,1,1,1,1,1,1,1,1,1,1,1,1,1,1,1,1,1,1,1,1,1,1,1,1,1,1,1,1,
1,1,1,1,1,1,1,6),(0.00577184337450902,0.0153846153846154,0.0307692307692308,
0.0461538461538462,0.0615384615384615,0.0769230769230769,0.0923076923076923,
0.107692307692308,0.123076923076923,0.138461538461538,0.153846153846154,
0.169230769230769,0.184615384615385,0.2,0.215384615384615,0.230769230769231,
0.246153846153846,0.261538461538462,0.276923076923077,0.292307692307692,
0.307692307692308,0.323076923076923,0.338461538461538,0.353846153846154,
0.369230769230769,0.384615384615385,0.4,0.415384615384615,0.430769230769231,
0.446153846153846,0.461538461538462,0.476923076923077,0.492307692307692,
0.507692307692308,0.523076923076923,0.538461538461538,0.553846153846154,
0.569230769230769,0.584615384615384,0.6,0.615384615384615,0.63076923076923,
0.646153846153846,0.661538461538461,0.676923076923076,0.692307692307692,
0.707692307692307,0.723076923076922,0.738461538461538,0.753846153846153,
0.769230769230768,0.784615384615384,0.799999999999999,0.815384615384614,
0.83076923076923,0.846153846153845,0.86153846153846,0.876923076923076,0.892307692307691,
0.907692307692306,0.923076923076922,0.938461538461537,0.953846153846152,
0.969230769230768,0.984615384615383,1.),.UNSPECIFIED.)
CURVE()
GEOMETRIC_REPRESENTATION_ITEM()
RATIONAL_B_SPLINE_CURVE((1.,1.,1.,1.,1.,1.,1.,1.,1.,1.,1.,1.,1.,1.,1.,1.,
1.,1.,1.,1.,1.,1.,1.,1.,1.,1.,1.,1.,1.,1.,1.,1.,1.,1.,1.,1.,1.,1.,1.,1.,
1.,1.,1.,1.,1.,1.,1.,1.,1.,1.,1.,1.,1.,1.,1.,1.,1.,1.,1.,1.,1.,1.,1.,1.,
1.,1.,1.,1.,1.,1.))
REPRESENTATION_ITEM('')
);
#286=(
BOUNDED_CURVE()
B_SPLINE_CURVE(5,(#39590,#39591,#39592,#39593,#39594,#39595,#39596,#39597,
#39598,#39599,#39600,#39601,#39602,#39603,#39604,#39605,#39606,#39607,#39608,
#39609,#39610,#39611,#39612,#39613,#39614,#39615,#39616,#39617,#39618,#39619,
#39620,#39621,#39622,#39623,#39624,#39625,#39626,#39627,#39628,#39629,#39630,
#39631,#39632,#39633,#39634,#39635,#39636,#39637,#39638,#39639,#39640,#39641,
#39642,#39643,#39644,#39645,#39646,#39647,#39648,#39649,#39650,#39651,#39652,
#39653,#39654,#39655,#39656,#39657,#39658,#39659),.UNSPECIFIED.,.F.,.F.)
B_SPLINE_CURVE_WITH_KNOTS((6,1,1,1,1,1,1,1,1,1,1,1,1,1,1,1,1,1,1,1,1,1,
1,1,1,1,1,1,1,1,1,1,1,1,1,1,1,1,1,1,1,1,1,1,1,1,1,1,1,1,1,1,1,1,1,1,1,1,
1,1,1,1,1,1,1,6),(0.,0.0153846153846154,0.0307692307692308,0.0461538461538462,
0.0615384615384615,0.0769230769230769,0.0923076923076923,0.107692307692308,
0.123076923076923,0.138461538461538,0.153846153846154,0.169230769230769,
0.184615384615385,0.2,0.215384615384615,0.230769230769231,0.246153846153846,
0.261538461538462,0.276923076923077,0.292307692307692,0.307692307692308,
0.323076923076923,0.338461538461538,0.353846153846154,0.369230769230769,
0.384615384615385,0.4,0.415384615384615,0.430769230769231,0.446153846153846,
0.461538461538462,0.476923076923077,0.492307692307692,0.507692307692308,
0.523076923076923,0.538461538461538,0.553846153846154,0.569230769230769,
0.584615384615384,0.6,0.615384615384615,0.63076923076923,0.646153846153846,
0.661538461538461,0.676923076923076,0.692307692307692,0.707692307692307,
0.723076923076922,0.738461538461538,0.753846153846153,0.769230769230768,
0.784615384615384,0.799999999999999,0.815384615384614,0.83076923076923,
0.846153846153845,0.86153846153846,0.876923076923076,0.892307692307691,
0.907692307692306,0.923076923076922,0.938461538461537,0.953846153846152,
0.969230769230768,0.984615384615383,0.994228156739698),.UNSPECIFIED.)
CURVE()
GEOMETRIC_REPRESENTATION_ITEM()
RATIONAL_B_SPLINE_CURVE((1.,1.,1.,1.,1.,1.,1.,1.,1.,1.,1.,1.,1.,1.,1.,1.,
1.,1.,1.,1.,1.,1.,1.,1.,1.,1.,1.,1.,1.,1.,1.,1.,1.,1.,1.,1.,1.,1.,1.,1.,
1.,1.,1.,1.,1.,1.,1.,1.,1.,1.,1.,1.,1.,1.,1.,1.,1.,1.,1.,1.,1.,1.,1.,1.,
1.,1.,1.,1.,1.,1.))
REPRESENTATION_ITEM('')
);
#287=(
BOUNDED_CURVE()
B_SPLINE_CURVE(5,(#39663,#39664,#39665,#39666,#39667,#39668,#39669,#39670,
#39671,#39672,#39673,#39674,#39675,#39676,#39677,#39678,#39679,#39680,#39681,
#39682,#39683,#39684,#39685,#39686,#39687,#39688,#39689,#39690,#39691,#39692,
#39693,#39694,#39695,#39696,#39697,#39698,#39699,#39700,#39701,#39702,#39703,
#39704,#39705,#39706,#39707,#39708,#39709,#39710,#39711,#39712,#39713,#39714,
#39715,#39716,#39717,#39718,#39719,#39720,#39721,#39722,#39723,#39724,#39725,
#39726,#39727,#39728,#39729,#39730,#39731,#39732),.UNSPECIFIED.,.F.,.F.)
B_SPLINE_CURVE_WITH_KNOTS((6,1,1,1,1,1,1,1,1,1,1,1,1,1,1,1,1,1,1,1,1,1,
1,1,1,1,1,1,1,1,1,1,1,1,1,1,1,1,1,1,1,1,1,1,1,1,1,1,1,1,1,1,1,1,1,1,1,1,
1,1,1,1,1,1,1,6),(0.00577184337451611,0.0153846153846154,0.0307692307692308,
0.0461538461538462,0.0615384615384615,0.0769230769230769,0.0923076923076923,
0.107692307692308,0.123076923076923,0.138461538461538,0.153846153846154,
0.169230769230769,0.184615384615385,0.2,0.215384615384615,0.230769230769231,
0.246153846153846,0.261538461538462,0.276923076923077,0.292307692307692,
0.307692307692308,0.323076923076923,0.338461538461538,0.353846153846154,
0.369230769230769,0.384615384615385,0.4,0.415384615384615,0.430769230769231,
0.446153846153846,0.461538461538462,0.476923076923077,0.492307692307692,
0.507692307692308,0.523076923076923,0.538461538461538,0.553846153846154,
0.569230769230769,0.584615384615384,0.6,0.615384615384615,0.63076923076923,
0.646153846153846,0.661538461538461,0.676923076923076,0.692307692307692,
0.707692307692307,0.723076923076922,0.738461538461538,0.753846153846153,
0.769230769230768,0.784615384615384,0.799999999999999,0.815384615384614,
0.83076923076923,0.846153846153845,0.86153846153846,0.876923076923076,0.892307692307691,
0.907692307692306,0.923076923076922,0.938461538461537,0.953846153846152,
0.969230769230768,0.984615384615383,1.),.UNSPECIFIED.)
CURVE()
GEOMETRIC_REPRESENTATION_ITEM()
RATIONAL_B_SPLINE_CURVE((1.,1.,1.,1.,1.,1.,1.,1.,1.,1.,1.,1.,1.,1.,1.,1.,
1.,1.,1.,1.,1.,1.,1.,1.,1.,1.,1.,1.,1.,1.,1.,1.,1.,1.,1.,1.,1.,1.,1.,1.,
1.,1.,1.,1.,1.,1.,1.,1.,1.,1.,1.,1.,1.,1.,1.,1.,1.,1.,1.,1.,1.,1.,1.,1.,
1.,1.,1.,1.,1.,1.))
REPRESENTATION_ITEM('')
);
#288=(
BOUNDED_CURVE()
B_SPLINE_CURVE(5,(#39736,#39737,#39738,#39739,#39740,#39741,#39742,#39743,
#39744,#39745,#39746,#39747,#39748,#39749,#39750,#39751,#39752,#39753,#39754,
#39755,#39756,#39757,#39758,#39759,#39760,#39761,#39762,#39763,#39764,#39765,
#39766,#39767,#39768,#39769,#39770,#39771,#39772,#39773,#39774,#39775,#39776,
#39777,#39778,#39779,#39780,#39781,#39782,#39783,#39784,#39785,#39786,#39787,
#39788,#39789,#39790,#39791,#39792,#39793,#39794,#39795,#39796,#39797,#39798,
#39799,#39800,#39801,#39802,#39803,#39804,#39805),.UNSPECIFIED.,.F.,.F.)
B_SPLINE_CURVE_WITH_KNOTS((6,1,1,1,1,1,1,1,1,1,1,1,1,1,1,1,1,1,1,1,1,1,
1,1,1,1,1,1,1,1,1,1,1,1,1,1,1,1,1,1,1,1,1,1,1,1,1,1,1,1,1,1,1,1,1,1,1,1,
1,1,1,1,1,1,1,6),(0.,0.0153846153846154,0.0307692307692308,0.0461538461538462,
0.0615384615384615,0.0769230769230769,0.0923076923076923,0.107692307692308,
0.123076923076923,0.138461538461538,0.153846153846154,0.169230769230769,
0.184615384615385,0.2,0.215384615384615,0.230769230769231,0.246153846153846,
0.261538461538462,0.276923076923077,0.292307692307692,0.307692307692308,
0.323076923076923,0.338461538461538,0.353846153846154,0.369230769230769,
0.384615384615385,0.4,0.415384615384615,0.430769230769231,0.446153846153846,
0.461538461538462,0.476923076923077,0.492307692307692,0.507692307692308,
0.523076923076923,0.538461538461538,0.553846153846154,0.569230769230769,
0.584615384615384,0.6,0.615384615384615,0.63076923076923,0.646153846153846,
0.661538461538461,0.676923076923076,0.692307692307692,0.707692307692307,
0.723076923076922,0.738461538461538,0.753846153846153,0.769230769230768,
0.784615384615384,0.799999999999999,0.815384615384614,0.83076923076923,
0.846153846153845,0.86153846153846,0.876923076923076,0.892307692307691,
0.907692307692306,0.923076923076922,0.938461538461537,0.953846153846152,
0.969230769230768,0.984615384615383,0.994228156739704),.UNSPECIFIED.)
CURVE()
GEOMETRIC_REPRESENTATION_ITEM()
RATIONAL_B_SPLINE_CURVE((1.,1.,1.,1.,1.,1.,1.,1.,1.,1.,1.,1.,1.,1.,1.,1.,
1.,1.,1.,1.,1.,1.,1.,1.,1.,1.,1.,1.,1.,1.,1.,1.,1.,1.,1.,1.,1.,1.,1.,1.,
1.,1.,1.,1.,1.,1.,1.,1.,1.,1.,1.,1.,1.,1.,1.,1.,1.,1.,1.,1.,1.,1.,1.,1.,
1.,1.,1.,1.,1.,1.))
REPRESENTATION_ITEM('')
);
#289=(
BOUNDED_CURVE()
B_SPLINE_CURVE(5,(#39809,#39810,#39811,#39812,#39813,#39814,#39815,#39816,
#39817,#39818,#39819,#39820,#39821,#39822,#39823,#39824,#39825,#39826,#39827,
#39828,#39829,#39830,#39831,#39832,#39833,#39834,#39835,#39836,#39837,#39838,
#39839,#39840,#39841,#39842,#39843,#39844,#39845,#39846,#39847,#39848,#39849,
#39850,#39851,#39852,#39853,#39854,#39855,#39856,#39857,#39858,#39859,#39860,
#39861,#39862,#39863,#39864,#39865,#39866,#39867,#39868,#39869,#39870,#39871,
#39872,#39873,#39874,#39875,#39876,#39877,#39878),.UNSPECIFIED.,.F.,.F.)
B_SPLINE_CURVE_WITH_KNOTS((6,1,1,1,1,1,1,1,1,1,1,1,1,1,1,1,1,1,1,1,1,1,
1,1,1,1,1,1,1,1,1,1,1,1,1,1,1,1,1,1,1,1,1,1,1,1,1,1,1,1,1,1,1,1,1,1,1,1,
1,1,1,1,1,1,1,6),(0.00577184337449692,0.0153846153846154,0.0307692307692308,
0.0461538461538462,0.0615384615384615,0.0769230769230769,0.0923076923076923,
0.107692307692308,0.123076923076923,0.138461538461538,0.153846153846154,
0.169230769230769,0.184615384615385,0.2,0.215384615384615,0.230769230769231,
0.246153846153846,0.261538461538462,0.276923076923077,0.292307692307692,
0.307692307692308,0.323076923076923,0.338461538461538,0.353846153846154,
0.369230769230769,0.384615384615385,0.4,0.415384615384615,0.430769230769231,
0.446153846153846,0.461538461538462,0.476923076923077,0.492307692307692,
0.507692307692308,0.523076923076923,0.538461538461538,0.553846153846154,
0.569230769230769,0.584615384615384,0.6,0.615384615384615,0.63076923076923,
0.646153846153846,0.661538461538461,0.676923076923076,0.692307692307692,
0.707692307692307,0.723076923076922,0.738461538461538,0.753846153846153,
0.769230769230768,0.784615384615384,0.799999999999999,0.815384615384614,
0.83076923076923,0.846153846153845,0.86153846153846,0.876923076923076,0.892307692307691,
0.907692307692306,0.923076923076922,0.938461538461537,0.953846153846152,
0.969230769230768,0.984615384615383,1.),.UNSPECIFIED.)
CURVE()
GEOMETRIC_REPRESENTATION_ITEM()
RATIONAL_B_SPLINE_CURVE((1.,1.,1.,1.,1.,1.,1.,1.,1.,1.,1.,1.,1.,1.,1.,1.,
1.,1.,1.,1.,1.,1.,1.,1.,1.,1.,1.,1.,1.,1.,1.,1.,1.,1.,1.,1.,1.,1.,1.,1.,
1.,1.,1.,1.,1.,1.,1.,1.,1.,1.,1.,1.,1.,1.,1.,1.,1.,1.,1.,1.,1.,1.,1.,1.,
1.,1.,1.,1.,1.,1.))
REPRESENTATION_ITEM('')
);
#290=(
BOUNDED_CURVE()
B_SPLINE_CURVE(5,(#39881,#39882,#39883,#39884,#39885,#39886,#39887,#39888,
#39889,#39890,#39891,#39892,#39893,#39894,#39895,#39896,#39897,#39898,#39899,
#39900,#39901,#39902,#39903,#39904,#39905,#39906,#39907,#39908,#39909,#39910,
#39911,#39912,#39913,#39914,#39915,#39916,#39917,#39918,#39919,#39920,#39921,
#39922,#39923,#39924,#39925,#39926,#39927,#39928,#39929,#39930,#39931,#39932,
#39933,#39934,#39935,#39936,#39937,#39938,#39939,#39940,#39941,#39942,#39943,
#39944,#39945,#39946,#39947,#39948,#39949,#39950),.UNSPECIFIED.,.F.,.F.)
B_SPLINE_CURVE_WITH_KNOTS((6,1,1,1,1,1,1,1,1,1,1,1,1,1,1,1,1,1,1,1,1,1,
1,1,1,1,1,1,1,1,1,1,1,1,1,1,1,1,1,1,1,1,1,1,1,1,1,1,1,1,1,1,1,1,1,1,1,1,
1,1,1,1,1,1,1,6),(0.,0.0153846153846154,0.0307692307692308,0.0461538461538462,
0.0615384615384615,0.0769230769230769,0.0923076923076923,0.107692307692308,
0.123076923076923,0.138461538461538,0.153846153846154,0.169230769230769,
0.184615384615385,0.2,0.215384615384615,0.230769230769231,0.246153846153846,
0.261538461538462,0.276923076923077,0.292307692307692,0.307692307692308,
0.323076923076923,0.338461538461538,0.353846153846154,0.369230769230769,
0.384615384615385,0.4,0.415384615384615,0.430769230769231,0.446153846153846,
0.461538461538462,0.476923076923077,0.492307692307692,0.507692307692308,
0.523076923076923,0.538461538461538,0.553846153846154,0.569230769230769,
0.584615384615384,0.6,0.615384615384615,0.63076923076923,0.646153846153846,
0.661538461538461,0.676923076923076,0.692307692307692,0.707692307692307,
0.723076923076922,0.738461538461538,0.753846153846153,0.769230769230768,
0.784615384615384,0.799999999999999,0.815384615384614,0.83076923076923,
0.846153846153845,0.86153846153846,0.876923076923076,0.892307692307691,
0.907692307692306,0.923076923076922,0.938461538461537,0.953846153846152,
0.969230769230768,0.984615384615383,0.994228156739723),.UNSPECIFIED.)
CURVE()
GEOMETRIC_REPRESENTATION_ITEM()
RATIONAL_B_SPLINE_CURVE((1.,1.,1.,1.,1.,1.,1.,1.,1.,1.,1.,1.,1.,1.,1.,1.,
1.,1.,1.,1.,1.,1.,1.,1.,1.,1.,1.,1.,1.,1.,1.,1.,1.,1.,1.,1.,1.,1.,1.,1.,
1.,1.,1.,1.,1.,1.,1.,1.,1.,1.,1.,1.,1.,1.,1.,1.,1.,1.,1.,1.,1.,1.,1.,1.,
1.,1.,1.,1.,1.,1.))
REPRESENTATION_ITEM('')
);
#291=(
BOUNDED_CURVE()
B_SPLINE_CURVE(5,(#40109,#40110,#40111,#40112,#40113,#40114,#40115,#40116,
#40117,#40118,#40119,#40120,#40121,#40122,#40123,#40124,#40125,#40126,#40127,
#40128,#40129,#40130,#40131,#40132,#40133,#40134,#40135,#40136,#40137,#40138,
#40139,#40140,#40141,#40142,#40143,#40144,#40145,#40146,#40147,#40148,#40149,
#40150,#40151,#40152,#40153,#40154,#40155,#40156,#40157,#40158,#40159,#40160,
#40161,#40162,#40163,#40164,#40165,#40166,#40167,#40168,#40169,#40170,#40171,
#40172,#40173,#40174,#40175,#40176,#40177,#40178),.UNSPECIFIED.,.F.,.F.)
B_SPLINE_CURVE_WITH_KNOTS((6,1,1,1,1,1,1,1,1,1,1,1,1,1,1,1,1,1,1,1,1,1,
1,1,1,1,1,1,1,1,1,1,1,1,1,1,1,1,1,1,1,1,1,1,1,1,1,1,1,1,1,1,1,1,1,1,1,1,
1,1,1,1,1,1,1,6),(-1.,-0.984615384615383,-0.969230769230768,-0.953846153846152,
-0.938461538461537,-0.923076923076922,-0.907692307692306,-0.892307692307691,
-0.876923076923076,-0.86153846153846,-0.846153846153845,-0.83076923076923,
-0.815384615384614,-0.799999999999999,-0.784615384615384,-0.769230769230768,
-0.753846153846153,-0.738461538461538,-0.723076923076922,-0.707692307692307,
-0.692307692307692,-0.676923076923076,-0.661538461538461,-0.646153846153846,
-0.63076923076923,-0.615384615384615,-0.6,-0.584615384615384,-0.569230769230769,
-0.553846153846154,-0.538461538461538,-0.523076923076923,-0.507692307692308,
-0.492307692307692,-0.476923076923077,-0.461538461538462,-0.446153846153846,
-0.430769230769231,-0.415384615384615,-0.4,-0.384615384615385,-0.369230769230769,
-0.353846153846154,-0.338461538461538,-0.323076923076923,-0.307692307692308,
-0.292307692307692,-0.276923076923077,-0.261538461538462,-0.246153846153846,
-0.230769230769231,-0.215384615384615,-0.2,-0.184615384615385,-0.169230769230769,
-0.153846153846154,-0.138461538461538,-0.123076923076923,-0.107692307692308,
-0.0923076923076923,-0.0769230769230769,-0.0615384615384615,-0.0461538461538462,
-0.0307692307692308,-0.0153846153846154,-0.00577184337448906),
 .UNSPECIFIED.)
CURVE()
GEOMETRIC_REPRESENTATION_ITEM()
RATIONAL_B_SPLINE_CURVE((1.,1.,1.,1.,1.,1.,1.,1.,1.,1.,1.,1.,1.,1.,1.,1.,
1.,1.,1.,1.,1.,1.,1.,1.,1.,1.,1.,1.,1.,1.,1.,1.,1.,1.,1.,1.,1.,1.,1.,1.,
1.,1.,1.,1.,1.,1.,1.,1.,1.,1.,1.,1.,1.,1.,1.,1.,1.,1.,1.,1.,1.,1.,1.,1.,
1.,1.,1.,1.,1.,1.))
REPRESENTATION_ITEM('')
);
#292=(
BOUNDED_CURVE()
B_SPLINE_CURVE(5,(#40329,#40330,#40331,#40332,#40333,#40334,#40335,#40336,
#40337,#40338,#40339,#40340,#40341,#40342,#40343,#40344,#40345,#40346,#40347,
#40348,#40349,#40350,#40351,#40352,#40353,#40354,#40355,#40356,#40357,#40358,
#40359,#40360,#40361,#40362,#40363,#40364,#40365,#40366,#40367,#40368,#40369,
#40370,#40371,#40372,#40373,#40374,#40375,#40376,#40377,#40378,#40379,#40380,
#40381,#40382,#40383,#40384,#40385,#40386,#40387,#40388,#40389,#40390,#40391,
#40392,#40393,#40394,#40395,#40396,#40397,#40398),.UNSPECIFIED.,.F.,.F.)
B_SPLINE_CURVE_WITH_KNOTS((6,1,1,1,1,1,1,1,1,1,1,1,1,1,1,1,1,1,1,1,1,1,
1,1,1,1,1,1,1,1,1,1,1,1,1,1,1,1,1,1,1,1,1,1,1,1,1,1,1,1,1,1,1,1,1,1,1,1,
1,1,1,1,1,1,1,6),(-0.994228156739728,-0.984615384615383,-0.969230769230768,
-0.953846153846152,-0.938461538461537,-0.923076923076922,-0.907692307692306,
-0.892307692307691,-0.876923076923076,-0.86153846153846,-0.846153846153845,
-0.83076923076923,-0.815384615384614,-0.799999999999999,-0.784615384615384,
-0.769230769230768,-0.753846153846153,-0.738461538461538,-0.723076923076922,
-0.707692307692307,-0.692307692307692,-0.676923076923076,-0.661538461538461,
-0.646153846153846,-0.63076923076923,-0.615384615384615,-0.6,-0.584615384615384,
-0.569230769230769,-0.553846153846154,-0.538461538461538,-0.523076923076923,
-0.507692307692308,-0.492307692307692,-0.476923076923077,-0.461538461538462,
-0.446153846153846,-0.430769230769231,-0.415384615384615,-0.4,-0.384615384615385,
-0.369230769230769,-0.353846153846154,-0.338461538461538,-0.323076923076923,
-0.307692307692308,-0.292307692307692,-0.276923076923077,-0.261538461538462,
-0.246153846153846,-0.230769230769231,-0.215384615384615,-0.2,-0.184615384615385,
-0.169230769230769,-0.153846153846154,-0.138461538461538,-0.123076923076923,
-0.107692307692308,-0.0923076923076923,-0.0769230769230769,-0.0615384615384615,
-0.0461538461538462,-0.0307692307692308,-0.0153846153846154,0.),
 .UNSPECIFIED.)
CURVE()
GEOMETRIC_REPRESENTATION_ITEM()
RATIONAL_B_SPLINE_CURVE((1.,1.,1.,1.,1.,1.,1.,1.,1.,1.,1.,1.,1.,1.,1.,1.,
1.,1.,1.,1.,1.,1.,1.,1.,1.,1.,1.,1.,1.,1.,1.,1.,1.,1.,1.,1.,1.,1.,1.,1.,
1.,1.,1.,1.,1.,1.,1.,1.,1.,1.,1.,1.,1.,1.,1.,1.,1.,1.,1.,1.,1.,1.,1.,1.,
1.,1.,1.,1.,1.,1.))
REPRESENTATION_ITEM('')
);
#293=(
BOUNDED_CURVE()
B_SPLINE_CURVE(5,(#40551,#40552,#40553,#40554,#40555,#40556,#40557,#40558,
#40559,#40560,#40561,#40562,#40563,#40564,#40565,#40566,#40567,#40568,#40569,
#40570,#40571,#40572,#40573,#40574,#40575,#40576,#40577,#40578,#40579,#40580,
#40581,#40582,#40583,#40584,#40585,#40586,#40587,#40588,#40589,#40590,#40591,
#40592,#40593,#40594,#40595,#40596,#40597,#40598,#40599,#40600,#40601,#40602,
#40603,#40604,#40605,#40606,#40607,#40608,#40609,#40610,#40611,#40612,#40613,
#40614,#40615,#40616,#40617,#40618,#40619,#40620),.UNSPECIFIED.,.F.,.F.)
B_SPLINE_CURVE_WITH_KNOTS((6,1,1,1,1,1,1,1,1,1,1,1,1,1,1,1,1,1,1,1,1,1,
1,1,1,1,1,1,1,1,1,1,1,1,1,1,1,1,1,1,1,1,1,1,1,1,1,1,1,1,1,1,1,1,1,1,1,1,
1,1,1,1,1,1,1,6),(-1.,-0.984615384615383,-0.969230769230768,-0.953846153846152,
-0.938461538461537,-0.923076923076922,-0.907692307692306,-0.892307692307691,
-0.876923076923076,-0.86153846153846,-0.846153846153845,-0.83076923076923,
-0.815384615384614,-0.799999999999999,-0.784615384615384,-0.769230769230768,
-0.753846153846153,-0.738461538461538,-0.723076923076922,-0.707692307692307,
-0.692307692307692,-0.676923076923076,-0.661538461538461,-0.646153846153846,
-0.63076923076923,-0.615384615384615,-0.6,-0.584615384615384,-0.569230769230769,
-0.553846153846154,-0.538461538461538,-0.523076923076923,-0.507692307692308,
-0.492307692307692,-0.476923076923077,-0.461538461538462,-0.446153846153846,
-0.430769230769231,-0.415384615384615,-0.4,-0.384615384615385,-0.369230769230769,
-0.353846153846154,-0.338461538461538,-0.323076923076923,-0.307692307692308,
-0.292307692307692,-0.276923076923077,-0.261538461538462,-0.246153846153846,
-0.230769230769231,-0.215384615384615,-0.2,-0.184615384615385,-0.169230769230769,
-0.153846153846154,-0.138461538461538,-0.123076923076923,-0.107692307692308,
-0.0923076923076923,-0.0769230769230769,-0.0615384615384615,-0.0461538461538462,
-0.0307692307692308,-0.0153846153846154,-0.0057718433744926),
 .UNSPECIFIED.)
CURVE()
GEOMETRIC_REPRESENTATION_ITEM()
RATIONAL_B_SPLINE_CURVE((1.,1.,1.,1.,1.,1.,1.,1.,1.,1.,1.,1.,1.,1.,1.,1.,
1.,1.,1.,1.,1.,1.,1.,1.,1.,1.,1.,1.,1.,1.,1.,1.,1.,1.,1.,1.,1.,1.,1.,1.,
1.,1.,1.,1.,1.,1.,1.,1.,1.,1.,1.,1.,1.,1.,1.,1.,1.,1.,1.,1.,1.,1.,1.,1.,
1.,1.,1.,1.,1.,1.))
REPRESENTATION_ITEM('')
);
#294=(
BOUNDED_CURVE()
B_SPLINE_CURVE(5,(#40771,#40772,#40773,#40774,#40775,#40776,#40777,#40778,
#40779,#40780,#40781,#40782,#40783,#40784,#40785,#40786,#40787,#40788,#40789,
#40790,#40791,#40792,#40793,#40794,#40795,#40796,#40797,#40798,#40799,#40800,
#40801,#40802,#40803,#40804,#40805,#40806,#40807,#40808,#40809,#40810,#40811,
#40812,#40813,#40814,#40815,#40816,#40817,#40818,#40819,#40820,#40821,#40822,
#40823,#40824,#40825,#40826,#40827,#40828,#40829,#40830,#40831,#40832,#40833,
#40834,#40835,#40836,#40837,#40838,#40839,#40840),.UNSPECIFIED.,.F.,.F.)
B_SPLINE_CURVE_WITH_KNOTS((6,1,1,1,1,1,1,1,1,1,1,1,1,1,1,1,1,1,1,1,1,1,
1,1,1,1,1,1,1,1,1,1,1,1,1,1,1,1,1,1,1,1,1,1,1,1,1,1,1,1,1,1,1,1,1,1,1,1,
1,1,1,1,1,1,1,6),(-0.994228156739718,-0.984615384615383,-0.969230769230768,
-0.953846153846152,-0.938461538461537,-0.923076923076922,-0.907692307692306,
-0.892307692307691,-0.876923076923076,-0.86153846153846,-0.846153846153845,
-0.83076923076923,-0.815384615384614,-0.799999999999999,-0.784615384615384,
-0.769230769230768,-0.753846153846153,-0.738461538461538,-0.723076923076922,
-0.707692307692307,-0.692307692307692,-0.676923076923076,-0.661538461538461,
-0.646153846153846,-0.63076923076923,-0.615384615384615,-0.6,-0.584615384615384,
-0.569230769230769,-0.553846153846154,-0.538461538461538,-0.523076923076923,
-0.507692307692308,-0.492307692307692,-0.476923076923077,-0.461538461538462,
-0.446153846153846,-0.430769230769231,-0.415384615384615,-0.4,-0.384615384615385,
-0.369230769230769,-0.353846153846154,-0.338461538461538,-0.323076923076923,
-0.307692307692308,-0.292307692307692,-0.276923076923077,-0.261538461538462,
-0.246153846153846,-0.230769230769231,-0.215384615384615,-0.2,-0.184615384615385,
-0.169230769230769,-0.153846153846154,-0.138461538461538,-0.123076923076923,
-0.107692307692308,-0.0923076923076923,-0.0769230769230769,-0.0615384615384615,
-0.0461538461538462,-0.0307692307692308,-0.0153846153846154,0.),
 .UNSPECIFIED.)
CURVE()
GEOMETRIC_REPRESENTATION_ITEM()
RATIONAL_B_SPLINE_CURVE((1.,1.,1.,1.,1.,1.,1.,1.,1.,1.,1.,1.,1.,1.,1.,1.,
1.,1.,1.,1.,1.,1.,1.,1.,1.,1.,1.,1.,1.,1.,1.,1.,1.,1.,1.,1.,1.,1.,1.,1.,
1.,1.,1.,1.,1.,1.,1.,1.,1.,1.,1.,1.,1.,1.,1.,1.,1.,1.,1.,1.,1.,1.,1.,1.,
1.,1.,1.,1.,1.,1.))
REPRESENTATION_ITEM('')
);
#295=(
BOUNDED_CURVE()
B_SPLINE_CURVE(5,(#40993,#40994,#40995,#40996,#40997,#40998,#40999,#41000,
#41001,#41002,#41003,#41004,#41005,#41006,#41007,#41008,#41009,#41010,#41011,
#41012,#41013,#41014,#41015,#41016,#41017,#41018,#41019,#41020,#41021,#41022,
#41023,#41024,#41025,#41026,#41027,#41028,#41029,#41030,#41031,#41032,#41033,
#41034,#41035,#41036,#41037,#41038,#41039,#41040,#41041,#41042,#41043,#41044,
#41045,#41046,#41047,#41048,#41049,#41050,#41051,#41052,#41053,#41054,#41055,
#41056,#41057,#41058,#41059,#41060,#41061,#41062),.UNSPECIFIED.,.F.,.F.)
B_SPLINE_CURVE_WITH_KNOTS((6,1,1,1,1,1,1,1,1,1,1,1,1,1,1,1,1,1,1,1,1,1,
1,1,1,1,1,1,1,1,1,1,1,1,1,1,1,1,1,1,1,1,1,1,1,1,1,1,1,1,1,1,1,1,1,1,1,1,
1,1,1,1,1,1,1,6),(-1.,-0.984615384615383,-0.969230769230768,-0.953846153846152,
-0.938461538461537,-0.923076923076922,-0.907692307692306,-0.892307692307691,
-0.876923076923076,-0.86153846153846,-0.846153846153845,-0.83076923076923,
-0.815384615384614,-0.799999999999999,-0.784615384615384,-0.769230769230768,
-0.753846153846153,-0.738461538461538,-0.723076923076922,-0.707692307692307,
-0.692307692307692,-0.676923076923076,-0.661538461538461,-0.646153846153846,
-0.63076923076923,-0.615384615384615,-0.6,-0.584615384615384,-0.569230769230769,
-0.553846153846154,-0.538461538461538,-0.523076923076923,-0.507692307692308,
-0.492307692307692,-0.476923076923077,-0.461538461538462,-0.446153846153846,
-0.430769230769231,-0.415384615384615,-0.4,-0.384615384615385,-0.369230769230769,
-0.353846153846154,-0.338461538461538,-0.323076923076923,-0.307692307692308,
-0.292307692307692,-0.276923076923077,-0.261538461538462,-0.246153846153846,
-0.230769230769231,-0.215384615384615,-0.2,-0.184615384615385,-0.169230769230769,
-0.153846153846154,-0.138461538461538,-0.123076923076923,-0.107692307692308,
-0.0923076923076923,-0.0769230769230769,-0.0615384615384615,-0.0461538461538462,
-0.0307692307692308,-0.0153846153846154,-0.00577184337449396),
 .UNSPECIFIED.)
CURVE()
GEOMETRIC_REPRESENTATION_ITEM()
RATIONAL_B_SPLINE_CURVE((1.,1.,1.,1.,1.,1.,1.,1.,1.,1.,1.,1.,1.,1.,1.,1.,
1.,1.,1.,1.,1.,1.,1.,1.,1.,1.,1.,1.,1.,1.,1.,1.,1.,1.,1.,1.,1.,1.,1.,1.,
1.,1.,1.,1.,1.,1.,1.,1.,1.,1.,1.,1.,1.,1.,1.,1.,1.,1.,1.,1.,1.,1.,1.,1.,
1.,1.,1.,1.,1.,1.))
REPRESENTATION_ITEM('')
);
#296=(
BOUNDED_CURVE()
B_SPLINE_CURVE(5,(#41213,#41214,#41215,#41216,#41217,#41218,#41219,#41220,
#41221,#41222,#41223,#41224,#41225,#41226,#41227,#41228,#41229,#41230,#41231,
#41232,#41233,#41234,#41235,#41236,#41237,#41238,#41239,#41240,#41241,#41242,
#41243,#41244,#41245,#41246,#41247,#41248,#41249,#41250,#41251,#41252,#41253,
#41254,#41255,#41256,#41257,#41258,#41259,#41260,#41261,#41262,#41263,#41264,
#41265,#41266,#41267,#41268,#41269,#41270,#41271,#41272,#41273,#41274,#41275,
#41276,#41277,#41278,#41279,#41280,#41281,#41282),.UNSPECIFIED.,.F.,.F.)
B_SPLINE_CURVE_WITH_KNOTS((6,1,1,1,1,1,1,1,1,1,1,1,1,1,1,1,1,1,1,1,1,1,
1,1,1,1,1,1,1,1,1,1,1,1,1,1,1,1,1,1,1,1,1,1,1,1,1,1,1,1,1,1,1,1,1,1,1,1,
1,1,1,1,1,1,1,6),(-0.994228156739702,-0.984615384615383,-0.969230769230768,
-0.953846153846152,-0.938461538461537,-0.923076923076922,-0.907692307692306,
-0.892307692307691,-0.876923076923076,-0.86153846153846,-0.846153846153845,
-0.83076923076923,-0.815384615384614,-0.799999999999999,-0.784615384615384,
-0.769230769230768,-0.753846153846153,-0.738461538461538,-0.723076923076922,
-0.707692307692307,-0.692307692307692,-0.676923076923076,-0.661538461538461,
-0.646153846153846,-0.63076923076923,-0.615384615384615,-0.6,-0.584615384615384,
-0.569230769230769,-0.553846153846154,-0.538461538461538,-0.523076923076923,
-0.507692307692308,-0.492307692307692,-0.476923076923077,-0.461538461538462,
-0.446153846153846,-0.430769230769231,-0.415384615384615,-0.4,-0.384615384615385,
-0.369230769230769,-0.353846153846154,-0.338461538461538,-0.323076923076923,
-0.307692307692308,-0.292307692307692,-0.276923076923077,-0.261538461538462,
-0.246153846153846,-0.230769230769231,-0.215384615384615,-0.2,-0.184615384615385,
-0.169230769230769,-0.153846153846154,-0.138461538461538,-0.123076923076923,
-0.107692307692308,-0.0923076923076923,-0.0769230769230769,-0.0615384615384615,
-0.0461538461538462,-0.0307692307692308,-0.0153846153846154,0.),
 .UNSPECIFIED.)
CURVE()
GEOMETRIC_REPRESENTATION_ITEM()
RATIONAL_B_SPLINE_CURVE((1.,1.,1.,1.,1.,1.,1.,1.,1.,1.,1.,1.,1.,1.,1.,1.,
1.,1.,1.,1.,1.,1.,1.,1.,1.,1.,1.,1.,1.,1.,1.,1.,1.,1.,1.,1.,1.,1.,1.,1.,
1.,1.,1.,1.,1.,1.,1.,1.,1.,1.,1.,1.,1.,1.,1.,1.,1.,1.,1.,1.,1.,1.,1.,1.,
1.,1.,1.,1.,1.,1.))
REPRESENTATION_ITEM('')
);
#297=(
BOUNDED_CURVE()
B_SPLINE_CURVE(5,(#41435,#41436,#41437,#41438,#41439,#41440,#41441,#41442,
#41443,#41444,#41445,#41446,#41447,#41448,#41449,#41450,#41451,#41452,#41453,
#41454,#41455,#41456,#41457,#41458,#41459,#41460,#41461,#41462,#41463,#41464,
#41465,#41466,#41467,#41468,#41469,#41470,#41471,#41472,#41473,#41474,#41475,
#41476,#41477,#41478,#41479,#41480,#41481,#41482,#41483,#41484,#41485,#41486,
#41487,#41488,#41489,#41490,#41491,#41492,#41493,#41494,#41495,#41496,#41497,
#41498,#41499,#41500,#41501,#41502,#41503,#41504),.UNSPECIFIED.,.F.,.F.)
B_SPLINE_CURVE_WITH_KNOTS((6,1,1,1,1,1,1,1,1,1,1,1,1,1,1,1,1,1,1,1,1,1,
1,1,1,1,1,1,1,1,1,1,1,1,1,1,1,1,1,1,1,1,1,1,1,1,1,1,1,1,1,1,1,1,1,1,1,1,
1,1,1,1,1,1,1,6),(-1.,-0.984615384615383,-0.969230769230768,-0.953846153846152,
-0.938461538461537,-0.923076923076922,-0.907692307692306,-0.892307692307691,
-0.876923076923076,-0.86153846153846,-0.846153846153845,-0.83076923076923,
-0.815384615384614,-0.799999999999999,-0.784615384615384,-0.769230769230768,
-0.753846153846153,-0.738461538461538,-0.723076923076922,-0.707692307692307,
-0.692307692307692,-0.676923076923076,-0.661538461538461,-0.646153846153846,
-0.63076923076923,-0.615384615384615,-0.6,-0.584615384615384,-0.569230769230769,
-0.553846153846154,-0.538461538461538,-0.523076923076923,-0.507692307692308,
-0.492307692307692,-0.476923076923077,-0.461538461538462,-0.446153846153846,
-0.430769230769231,-0.415384615384615,-0.4,-0.384615384615385,-0.369230769230769,
-0.353846153846154,-0.338461538461538,-0.323076923076923,-0.307692307692308,
-0.292307692307692,-0.276923076923077,-0.261538461538462,-0.246153846153846,
-0.230769230769231,-0.215384615384615,-0.2,-0.184615384615385,-0.169230769230769,
-0.153846153846154,-0.138461538461538,-0.123076923076923,-0.107692307692308,
-0.0923076923076923,-0.0769230769230769,-0.0615384615384615,-0.0461538461538462,
-0.0307692307692308,-0.0153846153846154,-0.00577184337450989),
 .UNSPECIFIED.)
CURVE()
GEOMETRIC_REPRESENTATION_ITEM()
RATIONAL_B_SPLINE_CURVE((1.,1.,1.,1.,1.,1.,1.,1.,1.,1.,1.,1.,1.,1.,1.,1.,
1.,1.,1.,1.,1.,1.,1.,1.,1.,1.,1.,1.,1.,1.,1.,1.,1.,1.,1.,1.,1.,1.,1.,1.,
1.,1.,1.,1.,1.,1.,1.,1.,1.,1.,1.,1.,1.,1.,1.,1.,1.,1.,1.,1.,1.,1.,1.,1.,
1.,1.,1.,1.,1.,1.))
REPRESENTATION_ITEM('')
);
#298=(
BOUNDED_CURVE()
B_SPLINE_CURVE(5,(#41655,#41656,#41657,#41658,#41659,#41660,#41661,#41662,
#41663,#41664,#41665,#41666,#41667,#41668,#41669,#41670,#41671,#41672,#41673,
#41674,#41675,#41676,#41677,#41678,#41679,#41680,#41681,#41682,#41683,#41684,
#41685,#41686,#41687,#41688,#41689,#41690,#41691,#41692,#41693,#41694,#41695,
#41696,#41697,#41698,#41699,#41700,#41701,#41702,#41703,#41704,#41705,#41706,
#41707,#41708,#41709,#41710,#41711,#41712,#41713,#41714,#41715,#41716,#41717,
#41718,#41719,#41720,#41721,#41722,#41723,#41724),.UNSPECIFIED.,.F.,.F.)
B_SPLINE_CURVE_WITH_KNOTS((6,1,1,1,1,1,1,1,1,1,1,1,1,1,1,1,1,1,1,1,1,1,
1,1,1,1,1,1,1,1,1,1,1,1,1,1,1,1,1,1,1,1,1,1,1,1,1,1,1,1,1,1,1,1,1,1,1,1,
1,1,1,1,1,1,1,6),(-0.994228156739736,-0.984615384615383,-0.969230769230768,
-0.953846153846152,-0.938461538461537,-0.923076923076922,-0.907692307692306,
-0.892307692307691,-0.876923076923076,-0.86153846153846,-0.846153846153845,
-0.83076923076923,-0.815384615384614,-0.799999999999999,-0.784615384615384,
-0.769230769230768,-0.753846153846153,-0.738461538461538,-0.723076923076922,
-0.707692307692307,-0.692307692307692,-0.676923076923076,-0.661538461538461,
-0.646153846153846,-0.63076923076923,-0.615384615384615,-0.6,-0.584615384615384,
-0.569230769230769,-0.553846153846154,-0.538461538461538,-0.523076923076923,
-0.507692307692308,-0.492307692307692,-0.476923076923077,-0.461538461538462,
-0.446153846153846,-0.430769230769231,-0.415384615384615,-0.4,-0.384615384615385,
-0.369230769230769,-0.353846153846154,-0.338461538461538,-0.323076923076923,
-0.307692307692308,-0.292307692307692,-0.276923076923077,-0.261538461538462,
-0.246153846153846,-0.230769230769231,-0.215384615384615,-0.2,-0.184615384615385,
-0.169230769230769,-0.153846153846154,-0.138461538461538,-0.123076923076923,
-0.107692307692308,-0.0923076923076923,-0.0769230769230769,-0.0615384615384615,
-0.0461538461538462,-0.0307692307692308,-0.0153846153846154,0.),
 .UNSPECIFIED.)
CURVE()
GEOMETRIC_REPRESENTATION_ITEM()
RATIONAL_B_SPLINE_CURVE((1.,1.,1.,1.,1.,1.,1.,1.,1.,1.,1.,1.,1.,1.,1.,1.,
1.,1.,1.,1.,1.,1.,1.,1.,1.,1.,1.,1.,1.,1.,1.,1.,1.,1.,1.,1.,1.,1.,1.,1.,
1.,1.,1.,1.,1.,1.,1.,1.,1.,1.,1.,1.,1.,1.,1.,1.,1.,1.,1.,1.,1.,1.,1.,1.,
1.,1.,1.,1.,1.,1.))
REPRESENTATION_ITEM('')
);
#299=(
BOUNDED_CURVE()
B_SPLINE_CURVE(5,(#41877,#41878,#41879,#41880,#41881,#41882,#41883,#41884,
#41885,#41886,#41887,#41888,#41889,#41890,#41891,#41892,#41893,#41894,#41895,
#41896,#41897,#41898,#41899,#41900,#41901,#41902,#41903,#41904,#41905,#41906,
#41907,#41908,#41909,#41910,#41911,#41912,#41913,#41914,#41915,#41916,#41917,
#41918,#41919,#41920,#41921,#41922,#41923,#41924,#41925,#41926,#41927,#41928,
#41929,#41930,#41931,#41932,#41933,#41934,#41935,#41936,#41937,#41938,#41939,
#41940,#41941,#41942,#41943,#41944,#41945,#41946),.UNSPECIFIED.,.F.,.F.)
B_SPLINE_CURVE_WITH_KNOTS((6,1,1,1,1,1,1,1,1,1,1,1,1,1,1,1,1,1,1,1,1,1,
1,1,1,1,1,1,1,1,1,1,1,1,1,1,1,1,1,1,1,1,1,1,1,1,1,1,1,1,1,1,1,1,1,1,1,1,
1,1,1,1,1,1,1,6),(-1.,-0.984615384615383,-0.969230769230768,-0.953846153846152,
-0.938461538461537,-0.923076923076922,-0.907692307692306,-0.892307692307691,
-0.876923076923076,-0.86153846153846,-0.846153846153845,-0.83076923076923,
-0.815384615384614,-0.799999999999999,-0.784615384615384,-0.769230769230768,
-0.753846153846153,-0.738461538461538,-0.723076923076922,-0.707692307692307,
-0.692307692307692,-0.676923076923076,-0.661538461538461,-0.646153846153846,
-0.63076923076923,-0.615384615384615,-0.6,-0.584615384615384,-0.569230769230769,
-0.553846153846154,-0.538461538461538,-0.523076923076923,-0.507692307692308,
-0.492307692307692,-0.476923076923077,-0.461538461538462,-0.446153846153846,
-0.430769230769231,-0.415384615384615,-0.4,-0.384615384615385,-0.369230769230769,
-0.353846153846154,-0.338461538461538,-0.323076923076923,-0.307692307692308,
-0.292307692307692,-0.276923076923077,-0.261538461538462,-0.246153846153846,
-0.230769230769231,-0.215384615384615,-0.2,-0.184615384615385,-0.169230769230769,
-0.153846153846154,-0.138461538461538,-0.123076923076923,-0.107692307692308,
-0.0923076923076923,-0.0769230769230769,-0.0615384615384615,-0.0461538461538462,
-0.0307692307692308,-0.0153846153846154,-0.00577184337452469),
 .UNSPECIFIED.)
CURVE()
GEOMETRIC_REPRESENTATION_ITEM()
RATIONAL_B_SPLINE_CURVE((1.,1.,1.,1.,1.,1.,1.,1.,1.,1.,1.,1.,1.,1.,1.,1.,
1.,1.,1.,1.,1.,1.,1.,1.,1.,1.,1.,1.,1.,1.,1.,1.,1.,1.,1.,1.,1.,1.,1.,1.,
1.,1.,1.,1.,1.,1.,1.,1.,1.,1.,1.,1.,1.,1.,1.,1.,1.,1.,1.,1.,1.,1.,1.,1.,
1.,1.,1.,1.,1.,1.))
REPRESENTATION_ITEM('')
);
#300=(
BOUNDED_CURVE()
B_SPLINE_CURVE(5,(#42097,#42098,#42099,#42100,#42101,#42102,#42103,#42104,
#42105,#42106,#42107,#42108,#42109,#42110,#42111,#42112,#42113,#42114,#42115,
#42116,#42117,#42118,#42119,#42120,#42121,#42122,#42123,#42124,#42125,#42126,
#42127,#42128,#42129,#42130,#42131,#42132,#42133,#42134,#42135,#42136,#42137,
#42138,#42139,#42140,#42141,#42142,#42143,#42144,#42145,#42146,#42147,#42148,
#42149,#42150,#42151,#42152,#42153,#42154,#42155,#42156,#42157,#42158,#42159,
#42160,#42161,#42162,#42163,#42164,#42165,#42166),.UNSPECIFIED.,.F.,.F.)
B_SPLINE_CURVE_WITH_KNOTS((6,1,1,1,1,1,1,1,1,1,1,1,1,1,1,1,1,1,1,1,1,1,
1,1,1,1,1,1,1,1,1,1,1,1,1,1,1,1,1,1,1,1,1,1,1,1,1,1,1,1,1,1,1,1,1,1,1,1,
1,1,1,1,1,1,1,6),(-0.994228156739717,-0.984615384615383,-0.969230769230768,
-0.953846153846152,-0.938461538461537,-0.923076923076922,-0.907692307692306,
-0.892307692307691,-0.876923076923076,-0.86153846153846,-0.846153846153845,
-0.83076923076923,-0.815384615384614,-0.799999999999999,-0.784615384615384,
-0.769230769230768,-0.753846153846153,-0.738461538461538,-0.723076923076922,
-0.707692307692307,-0.692307692307692,-0.676923076923076,-0.661538461538461,
-0.646153846153846,-0.63076923076923,-0.615384615384615,-0.6,-0.584615384615384,
-0.569230769230769,-0.553846153846154,-0.538461538461538,-0.523076923076923,
-0.507692307692308,-0.492307692307692,-0.476923076923077,-0.461538461538462,
-0.446153846153846,-0.430769230769231,-0.415384615384615,-0.4,-0.384615384615385,
-0.369230769230769,-0.353846153846154,-0.338461538461538,-0.323076923076923,
-0.307692307692308,-0.292307692307692,-0.276923076923077,-0.261538461538462,
-0.246153846153846,-0.230769230769231,-0.215384615384615,-0.2,-0.184615384615385,
-0.169230769230769,-0.153846153846154,-0.138461538461538,-0.123076923076923,
-0.107692307692308,-0.0923076923076923,-0.0769230769230769,-0.0615384615384615,
-0.0461538461538462,-0.0307692307692308,-0.0153846153846154,0.),
 .UNSPECIFIED.)
CURVE()
GEOMETRIC_REPRESENTATION_ITEM()
RATIONAL_B_SPLINE_CURVE((1.,1.,1.,1.,1.,1.,1.,1.,1.,1.,1.,1.,1.,1.,1.,1.,
1.,1.,1.,1.,1.,1.,1.,1.,1.,1.,1.,1.,1.,1.,1.,1.,1.,1.,1.,1.,1.,1.,1.,1.,
1.,1.,1.,1.,1.,1.,1.,1.,1.,1.,1.,1.,1.,1.,1.,1.,1.,1.,1.,1.,1.,1.,1.,1.,
1.,1.,1.,1.,1.,1.))
REPRESENTATION_ITEM('')
);
#301=(
BOUNDED_CURVE()
B_SPLINE_CURVE(5,(#42319,#42320,#42321,#42322,#42323,#42324,#42325,#42326,
#42327,#42328,#42329,#42330,#42331,#42332,#42333,#42334,#42335,#42336,#42337,
#42338,#42339,#42340,#42341,#42342,#42343,#42344,#42345,#42346,#42347,#42348,
#42349,#42350,#42351,#42352,#42353,#42354,#42355,#42356,#42357,#42358,#42359,
#42360,#42361,#42362,#42363,#42364,#42365,#42366,#42367,#42368,#42369,#42370,
#42371,#42372,#42373,#42374,#42375,#42376,#42377,#42378,#42379,#42380,#42381,
#42382,#42383,#42384,#42385,#42386,#42387,#42388),.UNSPECIFIED.,.F.,.F.)
B_SPLINE_CURVE_WITH_KNOTS((6,1,1,1,1,1,1,1,1,1,1,1,1,1,1,1,1,1,1,1,1,1,
1,1,1,1,1,1,1,1,1,1,1,1,1,1,1,1,1,1,1,1,1,1,1,1,1,1,1,1,1,1,1,1,1,1,1,1,
1,1,1,1,1,1,1,6),(-1.,-0.984615384615383,-0.969230769230768,-0.953846153846152,
-0.938461538461537,-0.923076923076922,-0.907692307692306,-0.892307692307691,
-0.876923076923076,-0.86153846153846,-0.846153846153845,-0.83076923076923,
-0.815384615384614,-0.799999999999999,-0.784615384615384,-0.769230769230768,
-0.753846153846153,-0.738461538461538,-0.723076923076922,-0.707692307692307,
-0.692307692307692,-0.676923076923076,-0.661538461538461,-0.646153846153846,
-0.63076923076923,-0.615384615384615,-0.6,-0.584615384615384,-0.569230769230769,
-0.553846153846154,-0.538461538461538,-0.523076923076923,-0.507692307692308,
-0.492307692307692,-0.476923076923077,-0.461538461538462,-0.446153846153846,
-0.430769230769231,-0.415384615384615,-0.4,-0.384615384615385,-0.369230769230769,
-0.353846153846154,-0.338461538461538,-0.323076923076923,-0.307692307692308,
-0.292307692307692,-0.276923076923077,-0.261538461538462,-0.246153846153846,
-0.230769230769231,-0.215384615384615,-0.2,-0.184615384615385,-0.169230769230769,
-0.153846153846154,-0.138461538461538,-0.123076923076923,-0.107692307692308,
-0.0923076923076923,-0.0769230769230769,-0.0615384615384615,-0.0461538461538462,
-0.0307692307692308,-0.0153846153846154,-0.00577184337453472),
 .UNSPECIFIED.)
CURVE()
GEOMETRIC_REPRESENTATION_ITEM()
RATIONAL_B_SPLINE_CURVE((1.,1.,1.,1.,1.,1.,1.,1.,1.,1.,1.,1.,1.,1.,1.,1.,
1.,1.,1.,1.,1.,1.,1.,1.,1.,1.,1.,1.,1.,1.,1.,1.,1.,1.,1.,1.,1.,1.,1.,1.,
1.,1.,1.,1.,1.,1.,1.,1.,1.,1.,1.,1.,1.,1.,1.,1.,1.,1.,1.,1.,1.,1.,1.,1.,
1.,1.,1.,1.,1.,1.))
REPRESENTATION_ITEM('')
);
#302=(
BOUNDED_CURVE()
B_SPLINE_CURVE(5,(#42539,#42540,#42541,#42542,#42543,#42544,#42545,#42546,
#42547,#42548,#42549,#42550,#42551,#42552,#42553,#42554,#42555,#42556,#42557,
#42558,#42559,#42560,#42561,#42562,#42563,#42564,#42565,#42566,#42567,#42568,
#42569,#42570,#42571,#42572,#42573,#42574,#42575,#42576,#42577,#42578,#42579,
#42580,#42581,#42582,#42583,#42584,#42585,#42586,#42587,#42588,#42589,#42590,
#42591,#42592,#42593,#42594,#42595,#42596,#42597,#42598,#42599,#42600,#42601,
#42602,#42603,#42604,#42605,#42606,#42607,#42608),.UNSPECIFIED.,.F.,.F.)
B_SPLINE_CURVE_WITH_KNOTS((6,1,1,1,1,1,1,1,1,1,1,1,1,1,1,1,1,1,1,1,1,1,
1,1,1,1,1,1,1,1,1,1,1,1,1,1,1,1,1,1,1,1,1,1,1,1,1,1,1,1,1,1,1,1,1,1,1,1,
1,1,1,1,1,1,1,6),(-0.994228156739652,-0.984615384615383,-0.969230769230768,
-0.953846153846152,-0.938461538461537,-0.923076923076922,-0.907692307692306,
-0.892307692307691,-0.876923076923076,-0.86153846153846,-0.846153846153845,
-0.83076923076923,-0.815384615384614,-0.799999999999999,-0.784615384615384,
-0.769230769230768,-0.753846153846153,-0.738461538461538,-0.723076923076922,
-0.707692307692307,-0.692307692307692,-0.676923076923076,-0.661538461538461,
-0.646153846153846,-0.63076923076923,-0.615384615384615,-0.6,-0.584615384615384,
-0.569230769230769,-0.553846153846154,-0.538461538461538,-0.523076923076923,
-0.507692307692308,-0.492307692307692,-0.476923076923077,-0.461538461538462,
-0.446153846153846,-0.430769230769231,-0.415384615384615,-0.4,-0.384615384615385,
-0.369230769230769,-0.353846153846154,-0.338461538461538,-0.323076923076923,
-0.307692307692308,-0.292307692307692,-0.276923076923077,-0.261538461538462,
-0.246153846153846,-0.230769230769231,-0.215384615384615,-0.2,-0.184615384615385,
-0.169230769230769,-0.153846153846154,-0.138461538461538,-0.123076923076923,
-0.107692307692308,-0.0923076923076923,-0.0769230769230769,-0.0615384615384615,
-0.0461538461538462,-0.0307692307692308,-0.0153846153846154,0.),
 .UNSPECIFIED.)
CURVE()
GEOMETRIC_REPRESENTATION_ITEM()
RATIONAL_B_SPLINE_CURVE((1.,1.,1.,1.,1.,1.,1.,1.,1.,1.,1.,1.,1.,1.,1.,1.,
1.,1.,1.,1.,1.,1.,1.,1.,1.,1.,1.,1.,1.,1.,1.,1.,1.,1.,1.,1.,1.,1.,1.,1.,
1.,1.,1.,1.,1.,1.,1.,1.,1.,1.,1.,1.,1.,1.,1.,1.,1.,1.,1.,1.,1.,1.,1.,1.,
1.,1.,1.,1.,1.,1.))
REPRESENTATION_ITEM('')
);
#303=(
BOUNDED_CURVE()
B_SPLINE_CURVE(5,(#42761,#42762,#42763,#42764,#42765,#42766,#42767,#42768,
#42769,#42770,#42771,#42772,#42773,#42774,#42775,#42776,#42777,#42778,#42779,
#42780,#42781,#42782,#42783,#42784,#42785,#42786,#42787,#42788,#42789,#42790,
#42791,#42792,#42793,#42794,#42795,#42796,#42797,#42798,#42799,#42800,#42801,
#42802,#42803,#42804,#42805,#42806,#42807,#42808,#42809,#42810,#42811,#42812,
#42813,#42814,#42815,#42816,#42817,#42818,#42819,#42820,#42821,#42822,#42823,
#42824,#42825,#42826,#42827,#42828,#42829,#42830),.UNSPECIFIED.,.F.,.F.)
B_SPLINE_CURVE_WITH_KNOTS((6,1,1,1,1,1,1,1,1,1,1,1,1,1,1,1,1,1,1,1,1,1,
1,1,1,1,1,1,1,1,1,1,1,1,1,1,1,1,1,1,1,1,1,1,1,1,1,1,1,1,1,1,1,1,1,1,1,1,
1,1,1,1,1,1,1,6),(-1.,-0.984615384615383,-0.969230769230768,-0.953846153846152,
-0.938461538461537,-0.923076923076922,-0.907692307692306,-0.892307692307691,
-0.876923076923076,-0.86153846153846,-0.846153846153845,-0.83076923076923,
-0.815384615384614,-0.799999999999999,-0.784615384615384,-0.769230769230768,
-0.753846153846153,-0.738461538461538,-0.723076923076922,-0.707692307692307,
-0.692307692307692,-0.676923076923076,-0.661538461538461,-0.646153846153846,
-0.63076923076923,-0.615384615384615,-0.6,-0.584615384615384,-0.569230769230769,
-0.553846153846154,-0.538461538461538,-0.523076923076923,-0.507692307692308,
-0.492307692307692,-0.476923076923077,-0.461538461538462,-0.446153846153846,
-0.430769230769231,-0.415384615384615,-0.4,-0.384615384615385,-0.369230769230769,
-0.353846153846154,-0.338461538461538,-0.323076923076923,-0.307692307692308,
-0.292307692307692,-0.276923076923077,-0.261538461538462,-0.246153846153846,
-0.230769230769231,-0.215384615384615,-0.2,-0.184615384615385,-0.169230769230769,
-0.153846153846154,-0.138461538461538,-0.123076923076923,-0.107692307692308,
-0.0923076923076923,-0.0769230769230769,-0.0615384615384615,-0.0461538461538462,
-0.0307692307692308,-0.0153846153846154,-0.00577184337450876),
 .UNSPECIFIED.)
CURVE()
GEOMETRIC_REPRESENTATION_ITEM()
RATIONAL_B_SPLINE_CURVE((1.,1.,1.,1.,1.,1.,1.,1.,1.,1.,1.,1.,1.,1.,1.,1.,
1.,1.,1.,1.,1.,1.,1.,1.,1.,1.,1.,1.,1.,1.,1.,1.,1.,1.,1.,1.,1.,1.,1.,1.,
1.,1.,1.,1.,1.,1.,1.,1.,1.,1.,1.,1.,1.,1.,1.,1.,1.,1.,1.,1.,1.,1.,1.,1.,
1.,1.,1.,1.,1.,1.))
REPRESENTATION_ITEM('')
);
#304=(
BOUNDED_CURVE()
B_SPLINE_CURVE(5,(#42981,#42982,#42983,#42984,#42985,#42986,#42987,#42988,
#42989,#42990,#42991,#42992,#42993,#42994,#42995,#42996,#42997,#42998,#42999,
#43000,#43001,#43002,#43003,#43004,#43005,#43006,#43007,#43008,#43009,#43010,
#43011,#43012,#43013,#43014,#43015,#43016,#43017,#43018,#43019,#43020,#43021,
#43022,#43023,#43024,#43025,#43026,#43027,#43028,#43029,#43030,#43031,#43032,
#43033,#43034,#43035,#43036,#43037,#43038,#43039,#43040,#43041,#43042,#43043,
#43044,#43045,#43046,#43047,#43048,#43049,#43050),.UNSPECIFIED.,.F.,.F.)
B_SPLINE_CURVE_WITH_KNOTS((6,1,1,1,1,1,1,1,1,1,1,1,1,1,1,1,1,1,1,1,1,1,
1,1,1,1,1,1,1,1,1,1,1,1,1,1,1,1,1,1,1,1,1,1,1,1,1,1,1,1,1,1,1,1,1,1,1,1,
1,1,1,1,1,1,1,6),(-0.994228156739683,-0.984615384615383,-0.969230769230768,
-0.953846153846152,-0.938461538461537,-0.923076923076922,-0.907692307692306,
-0.892307692307691,-0.876923076923076,-0.86153846153846,-0.846153846153845,
-0.83076923076923,-0.815384615384614,-0.799999999999999,-0.784615384615384,
-0.769230769230768,-0.753846153846153,-0.738461538461538,-0.723076923076922,
-0.707692307692307,-0.692307692307692,-0.676923076923076,-0.661538461538461,
-0.646153846153846,-0.63076923076923,-0.615384615384615,-0.6,-0.584615384615384,
-0.569230769230769,-0.553846153846154,-0.538461538461538,-0.523076923076923,
-0.507692307692308,-0.492307692307692,-0.476923076923077,-0.461538461538462,
-0.446153846153846,-0.430769230769231,-0.415384615384615,-0.4,-0.384615384615385,
-0.369230769230769,-0.353846153846154,-0.338461538461538,-0.323076923076923,
-0.307692307692308,-0.292307692307692,-0.276923076923077,-0.261538461538462,
-0.246153846153846,-0.230769230769231,-0.215384615384615,-0.2,-0.184615384615385,
-0.169230769230769,-0.153846153846154,-0.138461538461538,-0.123076923076923,
-0.107692307692308,-0.0923076923076923,-0.0769230769230769,-0.0615384615384615,
-0.0461538461538462,-0.0307692307692308,-0.0153846153846154,0.),
 .UNSPECIFIED.)
CURVE()
GEOMETRIC_REPRESENTATION_ITEM()
RATIONAL_B_SPLINE_CURVE((1.,1.,1.,1.,1.,1.,1.,1.,1.,1.,1.,1.,1.,1.,1.,1.,
1.,1.,1.,1.,1.,1.,1.,1.,1.,1.,1.,1.,1.,1.,1.,1.,1.,1.,1.,1.,1.,1.,1.,1.,
1.,1.,1.,1.,1.,1.,1.,1.,1.,1.,1.,1.,1.,1.,1.,1.,1.,1.,1.,1.,1.,1.,1.,1.,
1.,1.,1.,1.,1.,1.))
REPRESENTATION_ITEM('')
);
#305=(
BOUNDED_CURVE()
B_SPLINE_CURVE(5,(#43203,#43204,#43205,#43206,#43207,#43208,#43209,#43210,
#43211,#43212,#43213,#43214,#43215,#43216,#43217,#43218,#43219,#43220,#43221,
#43222,#43223,#43224,#43225,#43226,#43227,#43228,#43229,#43230,#43231,#43232,
#43233,#43234,#43235,#43236,#43237,#43238,#43239,#43240,#43241,#43242,#43243,
#43244,#43245,#43246,#43247,#43248,#43249,#43250,#43251,#43252,#43253,#43254,
#43255,#43256,#43257,#43258,#43259,#43260,#43261,#43262,#43263,#43264,#43265,
#43266,#43267,#43268,#43269,#43270,#43271,#43272),.UNSPECIFIED.,.F.,.F.)
B_SPLINE_CURVE_WITH_KNOTS((6,1,1,1,1,1,1,1,1,1,1,1,1,1,1,1,1,1,1,1,1,1,
1,1,1,1,1,1,1,1,1,1,1,1,1,1,1,1,1,1,1,1,1,1,1,1,1,1,1,1,1,1,1,1,1,1,1,1,
1,1,1,1,1,1,1,6),(-1.,-0.984615384615383,-0.969230769230768,-0.953846153846152,
-0.938461538461537,-0.923076923076922,-0.907692307692306,-0.892307692307691,
-0.876923076923076,-0.86153846153846,-0.846153846153845,-0.83076923076923,
-0.815384615384614,-0.799999999999999,-0.784615384615384,-0.769230769230768,
-0.753846153846153,-0.738461538461538,-0.723076923076922,-0.707692307692307,
-0.692307692307692,-0.676923076923076,-0.661538461538461,-0.646153846153846,
-0.63076923076923,-0.615384615384615,-0.6,-0.584615384615384,-0.569230769230769,
-0.553846153846154,-0.538461538461538,-0.523076923076923,-0.507692307692308,
-0.492307692307692,-0.476923076923077,-0.461538461538462,-0.446153846153846,
-0.430769230769231,-0.415384615384615,-0.4,-0.384615384615385,-0.369230769230769,
-0.353846153846154,-0.338461538461538,-0.323076923076923,-0.307692307692308,
-0.292307692307692,-0.276923076923077,-0.261538461538462,-0.246153846153846,
-0.230769230769231,-0.215384615384615,-0.2,-0.184615384615385,-0.169230769230769,
-0.153846153846154,-0.138461538461538,-0.123076923076923,-0.107692307692308,
-0.0923076923076923,-0.0769230769230769,-0.0615384615384615,-0.0461538461538462,
-0.0307692307692308,-0.0153846153846154,-0.00577184337450277),
 .UNSPECIFIED.)
CURVE()
GEOMETRIC_REPRESENTATION_ITEM()
RATIONAL_B_SPLINE_CURVE((1.,1.,1.,1.,1.,1.,1.,1.,1.,1.,1.,1.,1.,1.,1.,1.,
1.,1.,1.,1.,1.,1.,1.,1.,1.,1.,1.,1.,1.,1.,1.,1.,1.,1.,1.,1.,1.,1.,1.,1.,
1.,1.,1.,1.,1.,1.,1.,1.,1.,1.,1.,1.,1.,1.,1.,1.,1.,1.,1.,1.,1.,1.,1.,1.,
1.,1.,1.,1.,1.,1.))
REPRESENTATION_ITEM('')
);
#306=(
BOUNDED_CURVE()
B_SPLINE_CURVE(5,(#43423,#43424,#43425,#43426,#43427,#43428,#43429,#43430,
#43431,#43432,#43433,#43434,#43435,#43436,#43437,#43438,#43439,#43440,#43441,
#43442,#43443,#43444,#43445,#43446,#43447,#43448,#43449,#43450,#43451,#43452,
#43453,#43454,#43455,#43456,#43457,#43458,#43459,#43460,#43461,#43462,#43463,
#43464,#43465,#43466,#43467,#43468,#43469,#43470,#43471,#43472,#43473,#43474,
#43475,#43476,#43477,#43478,#43479,#43480,#43481,#43482,#43483,#43484,#43485,
#43486,#43487,#43488,#43489,#43490,#43491,#43492),.UNSPECIFIED.,.F.,.F.)
B_SPLINE_CURVE_WITH_KNOTS((6,1,1,1,1,1,1,1,1,1,1,1,1,1,1,1,1,1,1,1,1,1,
1,1,1,1,1,1,1,1,1,1,1,1,1,1,1,1,1,1,1,1,1,1,1,1,1,1,1,1,1,1,1,1,1,1,1,1,
1,1,1,1,1,1,1,6),(-0.994228156739689,-0.984615384615383,-0.969230769230768,
-0.953846153846152,-0.938461538461537,-0.923076923076922,-0.907692307692306,
-0.892307692307691,-0.876923076923076,-0.86153846153846,-0.846153846153845,
-0.83076923076923,-0.815384615384614,-0.799999999999999,-0.784615384615384,
-0.769230769230768,-0.753846153846153,-0.738461538461538,-0.723076923076922,
-0.707692307692307,-0.692307692307692,-0.676923076923076,-0.661538461538461,
-0.646153846153846,-0.63076923076923,-0.615384615384615,-0.6,-0.584615384615384,
-0.569230769230769,-0.553846153846154,-0.538461538461538,-0.523076923076923,
-0.507692307692308,-0.492307692307692,-0.476923076923077,-0.461538461538462,
-0.446153846153846,-0.430769230769231,-0.415384615384615,-0.4,-0.384615384615385,
-0.369230769230769,-0.353846153846154,-0.338461538461538,-0.323076923076923,
-0.307692307692308,-0.292307692307692,-0.276923076923077,-0.261538461538462,
-0.246153846153846,-0.230769230769231,-0.215384615384615,-0.2,-0.184615384615385,
-0.169230769230769,-0.153846153846154,-0.138461538461538,-0.123076923076923,
-0.107692307692308,-0.0923076923076923,-0.0769230769230769,-0.0615384615384615,
-0.0461538461538462,-0.0307692307692308,-0.0153846153846154,0.),
 .UNSPECIFIED.)
CURVE()
GEOMETRIC_REPRESENTATION_ITEM()
RATIONAL_B_SPLINE_CURVE((1.,1.,1.,1.,1.,1.,1.,1.,1.,1.,1.,1.,1.,1.,1.,1.,
1.,1.,1.,1.,1.,1.,1.,1.,1.,1.,1.,1.,1.,1.,1.,1.,1.,1.,1.,1.,1.,1.,1.,1.,
1.,1.,1.,1.,1.,1.,1.,1.,1.,1.,1.,1.,1.,1.,1.,1.,1.,1.,1.,1.,1.,1.,1.,1.,
1.,1.,1.,1.,1.,1.))
REPRESENTATION_ITEM('')
);
#307=(
BOUNDED_CURVE()
B_SPLINE_CURVE(5,(#43645,#43646,#43647,#43648,#43649,#43650,#43651,#43652,
#43653,#43654,#43655,#43656,#43657,#43658,#43659,#43660,#43661,#43662,#43663,
#43664,#43665,#43666,#43667,#43668,#43669,#43670,#43671,#43672,#43673,#43674,
#43675,#43676,#43677,#43678,#43679,#43680,#43681,#43682,#43683,#43684,#43685,
#43686,#43687,#43688,#43689,#43690,#43691,#43692,#43693,#43694,#43695,#43696,
#43697,#43698,#43699,#43700,#43701,#43702,#43703,#43704,#43705,#43706,#43707,
#43708,#43709,#43710,#43711,#43712,#43713,#43714),.UNSPECIFIED.,.F.,.F.)
B_SPLINE_CURVE_WITH_KNOTS((6,1,1,1,1,1,1,1,1,1,1,1,1,1,1,1,1,1,1,1,1,1,
1,1,1,1,1,1,1,1,1,1,1,1,1,1,1,1,1,1,1,1,1,1,1,1,1,1,1,1,1,1,1,1,1,1,1,1,
1,1,1,1,1,1,1,6),(-1.,-0.984615384615383,-0.969230769230768,-0.953846153846152,
-0.938461538461537,-0.923076923076922,-0.907692307692306,-0.892307692307691,
-0.876923076923076,-0.86153846153846,-0.846153846153845,-0.83076923076923,
-0.815384615384614,-0.799999999999999,-0.784615384615384,-0.769230769230768,
-0.753846153846153,-0.738461538461538,-0.723076923076922,-0.707692307692307,
-0.692307692307692,-0.676923076923076,-0.661538461538461,-0.646153846153846,
-0.63076923076923,-0.615384615384615,-0.6,-0.584615384615384,-0.569230769230769,
-0.553846153846154,-0.538461538461538,-0.523076923076923,-0.507692307692308,
-0.492307692307692,-0.476923076923077,-0.461538461538462,-0.446153846153846,
-0.430769230769231,-0.415384615384615,-0.4,-0.384615384615385,-0.369230769230769,
-0.353846153846154,-0.338461538461538,-0.323076923076923,-0.307692307692308,
-0.292307692307692,-0.276923076923077,-0.261538461538462,-0.246153846153846,
-0.230769230769231,-0.215384615384615,-0.2,-0.184615384615385,-0.169230769230769,
-0.153846153846154,-0.138461538461538,-0.123076923076923,-0.107692307692308,
-0.0923076923076923,-0.0769230769230769,-0.0615384615384615,-0.0461538461538462,
-0.0307692307692308,-0.0153846153846154,-0.00577184337451766),
 .UNSPECIFIED.)
CURVE()
GEOMETRIC_REPRESENTATION_ITEM()
RATIONAL_B_SPLINE_CURVE((1.,1.,1.,1.,1.,1.,1.,1.,1.,1.,1.,1.,1.,1.,1.,1.,
1.,1.,1.,1.,1.,1.,1.,1.,1.,1.,1.,1.,1.,1.,1.,1.,1.,1.,1.,1.,1.,1.,1.,1.,
1.,1.,1.,1.,1.,1.,1.,1.,1.,1.,1.,1.,1.,1.,1.,1.,1.,1.,1.,1.,1.,1.,1.,1.,
1.,1.,1.,1.,1.,1.))
REPRESENTATION_ITEM('')
);
#308=(
BOUNDED_CURVE()
B_SPLINE_CURVE(5,(#43865,#43866,#43867,#43868,#43869,#43870,#43871,#43872,
#43873,#43874,#43875,#43876,#43877,#43878,#43879,#43880,#43881,#43882,#43883,
#43884,#43885,#43886,#43887,#43888,#43889,#43890,#43891,#43892,#43893,#43894,
#43895,#43896,#43897,#43898,#43899,#43900,#43901,#43902,#43903,#43904,#43905,
#43906,#43907,#43908,#43909,#43910,#43911,#43912,#43913,#43914,#43915,#43916,
#43917,#43918,#43919,#43920,#43921,#43922,#43923,#43924,#43925,#43926,#43927,
#43928,#43929,#43930,#43931,#43932,#43933,#43934),.UNSPECIFIED.,.F.,.F.)
B_SPLINE_CURVE_WITH_KNOTS((6,1,1,1,1,1,1,1,1,1,1,1,1,1,1,1,1,1,1,1,1,1,
1,1,1,1,1,1,1,1,1,1,1,1,1,1,1,1,1,1,1,1,1,1,1,1,1,1,1,1,1,1,1,1,1,1,1,1,
1,1,1,1,1,1,1,6),(-0.994228156739687,-0.984615384615383,-0.969230769230768,
-0.953846153846152,-0.938461538461537,-0.923076923076922,-0.907692307692306,
-0.892307692307691,-0.876923076923076,-0.86153846153846,-0.846153846153845,
-0.83076923076923,-0.815384615384614,-0.799999999999999,-0.784615384615384,
-0.769230769230768,-0.753846153846153,-0.738461538461538,-0.723076923076922,
-0.707692307692307,-0.692307692307692,-0.676923076923076,-0.661538461538461,
-0.646153846153846,-0.63076923076923,-0.615384615384615,-0.6,-0.584615384615384,
-0.569230769230769,-0.553846153846154,-0.538461538461538,-0.523076923076923,
-0.507692307692308,-0.492307692307692,-0.476923076923077,-0.461538461538462,
-0.446153846153846,-0.430769230769231,-0.415384615384615,-0.4,-0.384615384615385,
-0.369230769230769,-0.353846153846154,-0.338461538461538,-0.323076923076923,
-0.307692307692308,-0.292307692307692,-0.276923076923077,-0.261538461538462,
-0.246153846153846,-0.230769230769231,-0.215384615384615,-0.2,-0.184615384615385,
-0.169230769230769,-0.153846153846154,-0.138461538461538,-0.123076923076923,
-0.107692307692308,-0.0923076923076923,-0.0769230769230769,-0.0615384615384615,
-0.0461538461538462,-0.0307692307692308,-0.0153846153846154,0.),
 .UNSPECIFIED.)
CURVE()
GEOMETRIC_REPRESENTATION_ITEM()
RATIONAL_B_SPLINE_CURVE((1.,1.,1.,1.,1.,1.,1.,1.,1.,1.,1.,1.,1.,1.,1.,1.,
1.,1.,1.,1.,1.,1.,1.,1.,1.,1.,1.,1.,1.,1.,1.,1.,1.,1.,1.,1.,1.,1.,1.,1.,
1.,1.,1.,1.,1.,1.,1.,1.,1.,1.,1.,1.,1.,1.,1.,1.,1.,1.,1.,1.,1.,1.,1.,1.,
1.,1.,1.,1.,1.,1.))
REPRESENTATION_ITEM('')
);
#309=(
BOUNDED_CURVE()
B_SPLINE_CURVE(5,(#44087,#44088,#44089,#44090,#44091,#44092,#44093,#44094,
#44095,#44096,#44097,#44098,#44099,#44100,#44101,#44102,#44103,#44104,#44105,
#44106,#44107,#44108,#44109,#44110,#44111,#44112,#44113,#44114,#44115,#44116,
#44117,#44118,#44119,#44120,#44121,#44122,#44123,#44124,#44125,#44126,#44127,
#44128,#44129,#44130,#44131,#44132,#44133,#44134,#44135,#44136,#44137,#44138,
#44139,#44140,#44141,#44142,#44143,#44144,#44145,#44146,#44147,#44148,#44149,
#44150,#44151,#44152,#44153,#44154,#44155,#44156),.UNSPECIFIED.,.F.,.F.)
B_SPLINE_CURVE_WITH_KNOTS((6,1,1,1,1,1,1,1,1,1,1,1,1,1,1,1,1,1,1,1,1,1,
1,1,1,1,1,1,1,1,1,1,1,1,1,1,1,1,1,1,1,1,1,1,1,1,1,1,1,1,1,1,1,1,1,1,1,1,
1,1,1,1,1,1,1,6),(-1.,-0.984615384615383,-0.969230769230768,-0.953846153846152,
-0.938461538461537,-0.923076923076922,-0.907692307692306,-0.892307692307691,
-0.876923076923076,-0.86153846153846,-0.846153846153845,-0.83076923076923,
-0.815384615384614,-0.799999999999999,-0.784615384615384,-0.769230769230768,
-0.753846153846153,-0.738461538461538,-0.723076923076922,-0.707692307692307,
-0.692307692307692,-0.676923076923076,-0.661538461538461,-0.646153846153846,
-0.63076923076923,-0.615384615384615,-0.6,-0.584615384615384,-0.569230769230769,
-0.553846153846154,-0.538461538461538,-0.523076923076923,-0.507692307692308,
-0.492307692307692,-0.476923076923077,-0.461538461538462,-0.446153846153846,
-0.430769230769231,-0.415384615384615,-0.4,-0.384615384615385,-0.369230769230769,
-0.353846153846154,-0.338461538461538,-0.323076923076923,-0.307692307692308,
-0.292307692307692,-0.276923076923077,-0.261538461538462,-0.246153846153846,
-0.230769230769231,-0.215384615384615,-0.2,-0.184615384615385,-0.169230769230769,
-0.153846153846154,-0.138461538461538,-0.123076923076923,-0.107692307692308,
-0.0923076923076923,-0.0769230769230769,-0.0615384615384615,-0.0461538461538462,
-0.0307692307692308,-0.0153846153846154,-0.00577184337452512),
 .UNSPECIFIED.)
CURVE()
GEOMETRIC_REPRESENTATION_ITEM()
RATIONAL_B_SPLINE_CURVE((1.,1.,1.,1.,1.,1.,1.,1.,1.,1.,1.,1.,1.,1.,1.,1.,
1.,1.,1.,1.,1.,1.,1.,1.,1.,1.,1.,1.,1.,1.,1.,1.,1.,1.,1.,1.,1.,1.,1.,1.,
1.,1.,1.,1.,1.,1.,1.,1.,1.,1.,1.,1.,1.,1.,1.,1.,1.,1.,1.,1.,1.,1.,1.,1.,
1.,1.,1.,1.,1.,1.))
REPRESENTATION_ITEM('')
);
#310=(
BOUNDED_CURVE()
B_SPLINE_CURVE(5,(#44307,#44308,#44309,#44310,#44311,#44312,#44313,#44314,
#44315,#44316,#44317,#44318,#44319,#44320,#44321,#44322,#44323,#44324,#44325,
#44326,#44327,#44328,#44329,#44330,#44331,#44332,#44333,#44334,#44335,#44336,
#44337,#44338,#44339,#44340,#44341,#44342,#44343,#44344,#44345,#44346,#44347,
#44348,#44349,#44350,#44351,#44352,#44353,#44354,#44355,#44356,#44357,#44358,
#44359,#44360,#44361,#44362,#44363,#44364,#44365,#44366,#44367,#44368,#44369,
#44370,#44371,#44372,#44373,#44374,#44375,#44376),.UNSPECIFIED.,.F.,.F.)
B_SPLINE_CURVE_WITH_KNOTS((6,1,1,1,1,1,1,1,1,1,1,1,1,1,1,1,1,1,1,1,1,1,
1,1,1,1,1,1,1,1,1,1,1,1,1,1,1,1,1,1,1,1,1,1,1,1,1,1,1,1,1,1,1,1,1,1,1,1,
1,1,1,1,1,1,1,6),(-0.994228156739691,-0.984615384615383,-0.969230769230768,
-0.953846153846152,-0.938461538461537,-0.923076923076922,-0.907692307692306,
-0.892307692307691,-0.876923076923076,-0.86153846153846,-0.846153846153845,
-0.83076923076923,-0.815384615384614,-0.799999999999999,-0.784615384615384,
-0.769230769230768,-0.753846153846153,-0.738461538461538,-0.723076923076922,
-0.707692307692307,-0.692307692307692,-0.676923076923076,-0.661538461538461,
-0.646153846153846,-0.63076923076923,-0.615384615384615,-0.6,-0.584615384615384,
-0.569230769230769,-0.553846153846154,-0.538461538461538,-0.523076923076923,
-0.507692307692308,-0.492307692307692,-0.476923076923077,-0.461538461538462,
-0.446153846153846,-0.430769230769231,-0.415384615384615,-0.4,-0.384615384615385,
-0.369230769230769,-0.353846153846154,-0.338461538461538,-0.323076923076923,
-0.307692307692308,-0.292307692307692,-0.276923076923077,-0.261538461538462,
-0.246153846153846,-0.230769230769231,-0.215384615384615,-0.2,-0.184615384615385,
-0.169230769230769,-0.153846153846154,-0.138461538461538,-0.123076923076923,
-0.107692307692308,-0.0923076923076923,-0.0769230769230769,-0.0615384615384615,
-0.0461538461538462,-0.0307692307692308,-0.0153846153846154,0.),
 .UNSPECIFIED.)
CURVE()
GEOMETRIC_REPRESENTATION_ITEM()
RATIONAL_B_SPLINE_CURVE((1.,1.,1.,1.,1.,1.,1.,1.,1.,1.,1.,1.,1.,1.,1.,1.,
1.,1.,1.,1.,1.,1.,1.,1.,1.,1.,1.,1.,1.,1.,1.,1.,1.,1.,1.,1.,1.,1.,1.,1.,
1.,1.,1.,1.,1.,1.,1.,1.,1.,1.,1.,1.,1.,1.,1.,1.,1.,1.,1.,1.,1.,1.,1.,1.,
1.,1.,1.,1.,1.,1.))
REPRESENTATION_ITEM('')
);
#311=(
BOUNDED_CURVE()
B_SPLINE_CURVE(5,(#44529,#44530,#44531,#44532,#44533,#44534,#44535,#44536,
#44537,#44538,#44539,#44540,#44541,#44542,#44543,#44544,#44545,#44546,#44547,
#44548,#44549,#44550,#44551,#44552,#44553,#44554,#44555,#44556,#44557,#44558,
#44559,#44560,#44561,#44562,#44563,#44564,#44565,#44566,#44567,#44568,#44569,
#44570,#44571,#44572,#44573,#44574,#44575,#44576,#44577,#44578,#44579,#44580,
#44581,#44582,#44583,#44584,#44585,#44586,#44587,#44588,#44589,#44590,#44591,
#44592,#44593,#44594,#44595,#44596,#44597,#44598),.UNSPECIFIED.,.F.,.F.)
B_SPLINE_CURVE_WITH_KNOTS((6,1,1,1,1,1,1,1,1,1,1,1,1,1,1,1,1,1,1,1,1,1,
1,1,1,1,1,1,1,1,1,1,1,1,1,1,1,1,1,1,1,1,1,1,1,1,1,1,1,1,1,1,1,1,1,1,1,1,
1,1,1,1,1,1,1,6),(-1.,-0.984615384615383,-0.969230769230768,-0.953846153846152,
-0.938461538461537,-0.923076923076922,-0.907692307692306,-0.892307692307691,
-0.876923076923076,-0.86153846153846,-0.846153846153845,-0.83076923076923,
-0.815384615384614,-0.799999999999999,-0.784615384615384,-0.769230769230768,
-0.753846153846153,-0.738461538461538,-0.723076923076922,-0.707692307692307,
-0.692307692307692,-0.676923076923076,-0.661538461538461,-0.646153846153846,
-0.63076923076923,-0.615384615384615,-0.6,-0.584615384615384,-0.569230769230769,
-0.553846153846154,-0.538461538461538,-0.523076923076923,-0.507692307692308,
-0.492307692307692,-0.476923076923077,-0.461538461538462,-0.446153846153846,
-0.430769230769231,-0.415384615384615,-0.4,-0.384615384615385,-0.369230769230769,
-0.353846153846154,-0.338461538461538,-0.323076923076923,-0.307692307692308,
-0.292307692307692,-0.276923076923077,-0.261538461538462,-0.246153846153846,
-0.230769230769231,-0.215384615384615,-0.2,-0.184615384615385,-0.169230769230769,
-0.153846153846154,-0.138461538461538,-0.123076923076923,-0.107692307692308,
-0.0923076923076923,-0.0769230769230769,-0.0615384615384615,-0.0461538461538462,
-0.0307692307692308,-0.0153846153846154,-0.00577184337448448),
 .UNSPECIFIED.)
CURVE()
GEOMETRIC_REPRESENTATION_ITEM()
RATIONAL_B_SPLINE_CURVE((1.,1.,1.,1.,1.,1.,1.,1.,1.,1.,1.,1.,1.,1.,1.,1.,
1.,1.,1.,1.,1.,1.,1.,1.,1.,1.,1.,1.,1.,1.,1.,1.,1.,1.,1.,1.,1.,1.,1.,1.,
1.,1.,1.,1.,1.,1.,1.,1.,1.,1.,1.,1.,1.,1.,1.,1.,1.,1.,1.,1.,1.,1.,1.,1.,
1.,1.,1.,1.,1.,1.))
REPRESENTATION_ITEM('')
);
#312=(
BOUNDED_CURVE()
B_SPLINE_CURVE(5,(#44749,#44750,#44751,#44752,#44753,#44754,#44755,#44756,
#44757,#44758,#44759,#44760,#44761,#44762,#44763,#44764,#44765,#44766,#44767,
#44768,#44769,#44770,#44771,#44772,#44773,#44774,#44775,#44776,#44777,#44778,
#44779,#44780,#44781,#44782,#44783,#44784,#44785,#44786,#44787,#44788,#44789,
#44790,#44791,#44792,#44793,#44794,#44795,#44796,#44797,#44798,#44799,#44800,
#44801,#44802,#44803,#44804,#44805,#44806,#44807,#44808,#44809,#44810,#44811,
#44812,#44813,#44814,#44815,#44816,#44817,#44818),.UNSPECIFIED.,.F.,.F.)
B_SPLINE_CURVE_WITH_KNOTS((6,1,1,1,1,1,1,1,1,1,1,1,1,1,1,1,1,1,1,1,1,1,
1,1,1,1,1,1,1,1,1,1,1,1,1,1,1,1,1,1,1,1,1,1,1,1,1,1,1,1,1,1,1,1,1,1,1,1,
1,1,1,1,1,1,1,6),(-0.99422815673972,-0.984615384615383,-0.969230769230768,
-0.953846153846152,-0.938461538461537,-0.923076923076922,-0.907692307692306,
-0.892307692307691,-0.876923076923076,-0.86153846153846,-0.846153846153845,
-0.83076923076923,-0.815384615384614,-0.799999999999999,-0.784615384615384,
-0.769230769230768,-0.753846153846153,-0.738461538461538,-0.723076923076922,
-0.707692307692307,-0.692307692307692,-0.676923076923076,-0.661538461538461,
-0.646153846153846,-0.63076923076923,-0.615384615384615,-0.6,-0.584615384615384,
-0.569230769230769,-0.553846153846154,-0.538461538461538,-0.523076923076923,
-0.507692307692308,-0.492307692307692,-0.476923076923077,-0.461538461538462,
-0.446153846153846,-0.430769230769231,-0.415384615384615,-0.4,-0.384615384615385,
-0.369230769230769,-0.353846153846154,-0.338461538461538,-0.323076923076923,
-0.307692307692308,-0.292307692307692,-0.276923076923077,-0.261538461538462,
-0.246153846153846,-0.230769230769231,-0.215384615384615,-0.2,-0.184615384615385,
-0.169230769230769,-0.153846153846154,-0.138461538461538,-0.123076923076923,
-0.107692307692308,-0.0923076923076923,-0.0769230769230769,-0.0615384615384615,
-0.0461538461538462,-0.0307692307692308,-0.0153846153846154,0.),
 .UNSPECIFIED.)
CURVE()
GEOMETRIC_REPRESENTATION_ITEM()
RATIONAL_B_SPLINE_CURVE((1.,1.,1.,1.,1.,1.,1.,1.,1.,1.,1.,1.,1.,1.,1.,1.,
1.,1.,1.,1.,1.,1.,1.,1.,1.,1.,1.,1.,1.,1.,1.,1.,1.,1.,1.,1.,1.,1.,1.,1.,
1.,1.,1.,1.,1.,1.,1.,1.,1.,1.,1.,1.,1.,1.,1.,1.,1.,1.,1.,1.,1.,1.,1.,1.,
1.,1.,1.,1.,1.,1.))
REPRESENTATION_ITEM('')
);
#313=(
BOUNDED_CURVE()
B_SPLINE_CURVE(5,(#44971,#44972,#44973,#44974,#44975,#44976,#44977,#44978,
#44979,#44980,#44981,#44982,#44983,#44984,#44985,#44986,#44987,#44988,#44989,
#44990,#44991,#44992,#44993,#44994,#44995,#44996,#44997,#44998,#44999,#45000,
#45001,#45002,#45003,#45004,#45005,#45006,#45007,#45008,#45009,#45010,#45011,
#45012,#45013,#45014,#45015,#45016,#45017,#45018,#45019,#45020,#45021,#45022,
#45023,#45024,#45025,#45026,#45027,#45028,#45029,#45030,#45031,#45032,#45033,
#45034,#45035,#45036,#45037,#45038,#45039,#45040),.UNSPECIFIED.,.F.,.F.)
B_SPLINE_CURVE_WITH_KNOTS((6,1,1,1,1,1,1,1,1,1,1,1,1,1,1,1,1,1,1,1,1,1,
1,1,1,1,1,1,1,1,1,1,1,1,1,1,1,1,1,1,1,1,1,1,1,1,1,1,1,1,1,1,1,1,1,1,1,1,
1,1,1,1,1,1,1,6),(-1.,-0.984615384615383,-0.969230769230768,-0.953846153846152,
-0.938461538461537,-0.923076923076922,-0.907692307692306,-0.892307692307691,
-0.876923076923076,-0.86153846153846,-0.846153846153845,-0.83076923076923,
-0.815384615384614,-0.799999999999999,-0.784615384615384,-0.769230769230768,
-0.753846153846153,-0.738461538461538,-0.723076923076922,-0.707692307692307,
-0.692307692307692,-0.676923076923076,-0.661538461538461,-0.646153846153846,
-0.63076923076923,-0.615384615384615,-0.6,-0.584615384615384,-0.569230769230769,
-0.553846153846154,-0.538461538461538,-0.523076923076923,-0.507692307692308,
-0.492307692307692,-0.476923076923077,-0.461538461538462,-0.446153846153846,
-0.430769230769231,-0.415384615384615,-0.4,-0.384615384615385,-0.369230769230769,
-0.353846153846154,-0.338461538461538,-0.323076923076923,-0.307692307692308,
-0.292307692307692,-0.276923076923077,-0.261538461538462,-0.246153846153846,
-0.230769230769231,-0.215384615384615,-0.2,-0.184615384615385,-0.169230769230769,
-0.153846153846154,-0.138461538461538,-0.123076923076923,-0.107692307692308,
-0.0923076923076923,-0.0769230769230769,-0.0615384615384615,-0.0461538461538462,
-0.0307692307692308,-0.0153846153846154,-0.00577184337448251),
 .UNSPECIFIED.)
CURVE()
GEOMETRIC_REPRESENTATION_ITEM()
RATIONAL_B_SPLINE_CURVE((1.,1.,1.,1.,1.,1.,1.,1.,1.,1.,1.,1.,1.,1.,1.,1.,
1.,1.,1.,1.,1.,1.,1.,1.,1.,1.,1.,1.,1.,1.,1.,1.,1.,1.,1.,1.,1.,1.,1.,1.,
1.,1.,1.,1.,1.,1.,1.,1.,1.,1.,1.,1.,1.,1.,1.,1.,1.,1.,1.,1.,1.,1.,1.,1.,
1.,1.,1.,1.,1.,1.))
REPRESENTATION_ITEM('')
);
#314=(
BOUNDED_CURVE()
B_SPLINE_CURVE(5,(#45191,#45192,#45193,#45194,#45195,#45196,#45197,#45198,
#45199,#45200,#45201,#45202,#45203,#45204,#45205,#45206,#45207,#45208,#45209,
#45210,#45211,#45212,#45213,#45214,#45215,#45216,#45217,#45218,#45219,#45220,
#45221,#45222,#45223,#45224,#45225,#45226,#45227,#45228,#45229,#45230,#45231,
#45232,#45233,#45234,#45235,#45236,#45237,#45238,#45239,#45240,#45241,#45242,
#45243,#45244,#45245,#45246,#45247,#45248,#45249,#45250,#45251,#45252,#45253,
#45254,#45255,#45256,#45257,#45258,#45259,#45260),.UNSPECIFIED.,.F.,.F.)
B_SPLINE_CURVE_WITH_KNOTS((6,1,1,1,1,1,1,1,1,1,1,1,1,1,1,1,1,1,1,1,1,1,
1,1,1,1,1,1,1,1,1,1,1,1,1,1,1,1,1,1,1,1,1,1,1,1,1,1,1,1,1,1,1,1,1,1,1,1,
1,1,1,1,1,1,1,6),(-0.994228156739703,-0.984615384615383,-0.969230769230768,
-0.953846153846152,-0.938461538461537,-0.923076923076922,-0.907692307692306,
-0.892307692307691,-0.876923076923076,-0.86153846153846,-0.846153846153845,
-0.83076923076923,-0.815384615384614,-0.799999999999999,-0.784615384615384,
-0.769230769230768,-0.753846153846153,-0.738461538461538,-0.723076923076922,
-0.707692307692307,-0.692307692307692,-0.676923076923076,-0.661538461538461,
-0.646153846153846,-0.63076923076923,-0.615384615384615,-0.6,-0.584615384615384,
-0.569230769230769,-0.553846153846154,-0.538461538461538,-0.523076923076923,
-0.507692307692308,-0.492307692307692,-0.476923076923077,-0.461538461538462,
-0.446153846153846,-0.430769230769231,-0.415384615384615,-0.4,-0.384615384615385,
-0.369230769230769,-0.353846153846154,-0.338461538461538,-0.323076923076923,
-0.307692307692308,-0.292307692307692,-0.276923076923077,-0.261538461538462,
-0.246153846153846,-0.230769230769231,-0.215384615384615,-0.2,-0.184615384615385,
-0.169230769230769,-0.153846153846154,-0.138461538461538,-0.123076923076923,
-0.107692307692308,-0.0923076923076923,-0.0769230769230769,-0.0615384615384615,
-0.0461538461538462,-0.0307692307692308,-0.0153846153846154,0.),
 .UNSPECIFIED.)
CURVE()
GEOMETRIC_REPRESENTATION_ITEM()
RATIONAL_B_SPLINE_CURVE((1.,1.,1.,1.,1.,1.,1.,1.,1.,1.,1.,1.,1.,1.,1.,1.,
1.,1.,1.,1.,1.,1.,1.,1.,1.,1.,1.,1.,1.,1.,1.,1.,1.,1.,1.,1.,1.,1.,1.,1.,
1.,1.,1.,1.,1.,1.,1.,1.,1.,1.,1.,1.,1.,1.,1.,1.,1.,1.,1.,1.,1.,1.,1.,1.,
1.,1.,1.,1.,1.,1.))
REPRESENTATION_ITEM('')
);
#315=(
BOUNDED_CURVE()
B_SPLINE_CURVE(5,(#45413,#45414,#45415,#45416,#45417,#45418,#45419,#45420,
#45421,#45422,#45423,#45424,#45425,#45426,#45427,#45428,#45429,#45430,#45431,
#45432,#45433,#45434,#45435,#45436,#45437,#45438,#45439,#45440,#45441,#45442,
#45443,#45444,#45445,#45446,#45447,#45448,#45449,#45450,#45451,#45452,#45453,
#45454,#45455,#45456,#45457,#45458,#45459,#45460,#45461,#45462,#45463,#45464,
#45465,#45466,#45467,#45468,#45469,#45470,#45471,#45472,#45473,#45474,#45475,
#45476,#45477,#45478,#45479,#45480,#45481,#45482),.UNSPECIFIED.,.F.,.F.)
B_SPLINE_CURVE_WITH_KNOTS((6,1,1,1,1,1,1,1,1,1,1,1,1,1,1,1,1,1,1,1,1,1,
1,1,1,1,1,1,1,1,1,1,1,1,1,1,1,1,1,1,1,1,1,1,1,1,1,1,1,1,1,1,1,1,1,1,1,1,
1,1,1,1,1,1,1,6),(-1.,-0.984615384615383,-0.969230769230768,-0.953846153846152,
-0.938461538461537,-0.923076923076922,-0.907692307692306,-0.892307692307691,
-0.876923076923076,-0.86153846153846,-0.846153846153845,-0.83076923076923,
-0.815384615384614,-0.799999999999999,-0.784615384615384,-0.769230769230768,
-0.753846153846153,-0.738461538461538,-0.723076923076922,-0.707692307692307,
-0.692307692307692,-0.676923076923076,-0.661538461538461,-0.646153846153846,
-0.63076923076923,-0.615384615384615,-0.6,-0.584615384615384,-0.569230769230769,
-0.553846153846154,-0.538461538461538,-0.523076923076923,-0.507692307692308,
-0.492307692307692,-0.476923076923077,-0.461538461538462,-0.446153846153846,
-0.430769230769231,-0.415384615384615,-0.4,-0.384615384615385,-0.369230769230769,
-0.353846153846154,-0.338461538461538,-0.323076923076923,-0.307692307692308,
-0.292307692307692,-0.276923076923077,-0.261538461538462,-0.246153846153846,
-0.230769230769231,-0.215384615384615,-0.2,-0.184615384615385,-0.169230769230769,
-0.153846153846154,-0.138461538461538,-0.123076923076923,-0.107692307692308,
-0.0923076923076923,-0.0769230769230769,-0.0615384615384615,-0.0461538461538462,
-0.0307692307692308,-0.0153846153846154,-0.00577184337449602),
 .UNSPECIFIED.)
CURVE()
GEOMETRIC_REPRESENTATION_ITEM()
RATIONAL_B_SPLINE_CURVE((1.,1.,1.,1.,1.,1.,1.,1.,1.,1.,1.,1.,1.,1.,1.,1.,
1.,1.,1.,1.,1.,1.,1.,1.,1.,1.,1.,1.,1.,1.,1.,1.,1.,1.,1.,1.,1.,1.,1.,1.,
1.,1.,1.,1.,1.,1.,1.,1.,1.,1.,1.,1.,1.,1.,1.,1.,1.,1.,1.,1.,1.,1.,1.,1.,
1.,1.,1.,1.,1.,1.))
REPRESENTATION_ITEM('')
);
#316=(
BOUNDED_CURVE()
B_SPLINE_CURVE(5,(#45633,#45634,#45635,#45636,#45637,#45638,#45639,#45640,
#45641,#45642,#45643,#45644,#45645,#45646,#45647,#45648,#45649,#45650,#45651,
#45652,#45653,#45654,#45655,#45656,#45657,#45658,#45659,#45660,#45661,#45662,
#45663,#45664,#45665,#45666,#45667,#45668,#45669,#45670,#45671,#45672,#45673,
#45674,#45675,#45676,#45677,#45678,#45679,#45680,#45681,#45682,#45683,#45684,
#45685,#45686,#45687,#45688,#45689,#45690,#45691,#45692,#45693,#45694,#45695,
#45696,#45697,#45698,#45699,#45700,#45701,#45702),.UNSPECIFIED.,.F.,.F.)
B_SPLINE_CURVE_WITH_KNOTS((6,1,1,1,1,1,1,1,1,1,1,1,1,1,1,1,1,1,1,1,1,1,
1,1,1,1,1,1,1,1,1,1,1,1,1,1,1,1,1,1,1,1,1,1,1,1,1,1,1,1,1,1,1,1,1,1,1,1,
1,1,1,1,1,1,1,6),(-0.994228156739695,-0.984615384615383,-0.969230769230768,
-0.953846153846152,-0.938461538461537,-0.923076923076922,-0.907692307692306,
-0.892307692307691,-0.876923076923076,-0.86153846153846,-0.846153846153845,
-0.83076923076923,-0.815384615384614,-0.799999999999999,-0.784615384615384,
-0.769230769230768,-0.753846153846153,-0.738461538461538,-0.723076923076922,
-0.707692307692307,-0.692307692307692,-0.676923076923076,-0.661538461538461,
-0.646153846153846,-0.63076923076923,-0.615384615384615,-0.6,-0.584615384615384,
-0.569230769230769,-0.553846153846154,-0.538461538461538,-0.523076923076923,
-0.507692307692308,-0.492307692307692,-0.476923076923077,-0.461538461538462,
-0.446153846153846,-0.430769230769231,-0.415384615384615,-0.4,-0.384615384615385,
-0.369230769230769,-0.353846153846154,-0.338461538461538,-0.323076923076923,
-0.307692307692308,-0.292307692307692,-0.276923076923077,-0.261538461538462,
-0.246153846153846,-0.230769230769231,-0.215384615384615,-0.2,-0.184615384615385,
-0.169230769230769,-0.153846153846154,-0.138461538461538,-0.123076923076923,
-0.107692307692308,-0.0923076923076923,-0.0769230769230769,-0.0615384615384615,
-0.0461538461538462,-0.0307692307692308,-0.0153846153846154,0.),
 .UNSPECIFIED.)
CURVE()
GEOMETRIC_REPRESENTATION_ITEM()
RATIONAL_B_SPLINE_CURVE((1.,1.,1.,1.,1.,1.,1.,1.,1.,1.,1.,1.,1.,1.,1.,1.,
1.,1.,1.,1.,1.,1.,1.,1.,1.,1.,1.,1.,1.,1.,1.,1.,1.,1.,1.,1.,1.,1.,1.,1.,
1.,1.,1.,1.,1.,1.,1.,1.,1.,1.,1.,1.,1.,1.,1.,1.,1.,1.,1.,1.,1.,1.,1.,1.,
1.,1.,1.,1.,1.,1.))
REPRESENTATION_ITEM('')
);
#317=(
BOUNDED_CURVE()
B_SPLINE_CURVE(5,(#45855,#45856,#45857,#45858,#45859,#45860,#45861,#45862,
#45863,#45864,#45865,#45866,#45867,#45868,#45869,#45870,#45871,#45872,#45873,
#45874,#45875,#45876,#45877,#45878,#45879,#45880,#45881,#45882,#45883,#45884,
#45885,#45886,#45887,#45888,#45889,#45890,#45891,#45892,#45893,#45894,#45895,
#45896,#45897,#45898,#45899,#45900,#45901,#45902,#45903,#45904,#45905,#45906,
#45907,#45908,#45909,#45910,#45911,#45912,#45913,#45914,#45915,#45916,#45917,
#45918,#45919,#45920,#45921,#45922,#45923,#45924),.UNSPECIFIED.,.F.,.F.)
B_SPLINE_CURVE_WITH_KNOTS((6,1,1,1,1,1,1,1,1,1,1,1,1,1,1,1,1,1,1,1,1,1,
1,1,1,1,1,1,1,1,1,1,1,1,1,1,1,1,1,1,1,1,1,1,1,1,1,1,1,1,1,1,1,1,1,1,1,1,
1,1,1,1,1,1,1,6),(-1.,-0.984615384615383,-0.969230769230768,-0.953846153846152,
-0.938461538461537,-0.923076923076922,-0.907692307692306,-0.892307692307691,
-0.876923076923076,-0.86153846153846,-0.846153846153845,-0.83076923076923,
-0.815384615384614,-0.799999999999999,-0.784615384615384,-0.769230769230768,
-0.753846153846153,-0.738461538461538,-0.723076923076922,-0.707692307692307,
-0.692307692307692,-0.676923076923076,-0.661538461538461,-0.646153846153846,
-0.63076923076923,-0.615384615384615,-0.6,-0.584615384615384,-0.569230769230769,
-0.553846153846154,-0.538461538461538,-0.523076923076923,-0.507692307692308,
-0.492307692307692,-0.476923076923077,-0.461538461538462,-0.446153846153846,
-0.430769230769231,-0.415384615384615,-0.4,-0.384615384615385,-0.369230769230769,
-0.353846153846154,-0.338461538461538,-0.323076923076923,-0.307692307692308,
-0.292307692307692,-0.276923076923077,-0.261538461538462,-0.246153846153846,
-0.230769230769231,-0.215384615384615,-0.2,-0.184615384615385,-0.169230769230769,
-0.153846153846154,-0.138461538461538,-0.123076923076923,-0.107692307692308,
-0.0923076923076923,-0.0769230769230769,-0.0615384615384615,-0.0461538461538462,
-0.0307692307692308,-0.0153846153846154,-0.00577184337450911),
 .UNSPECIFIED.)
CURVE()
GEOMETRIC_REPRESENTATION_ITEM()
RATIONAL_B_SPLINE_CURVE((1.,1.,1.,1.,1.,1.,1.,1.,1.,1.,1.,1.,1.,1.,1.,1.,
1.,1.,1.,1.,1.,1.,1.,1.,1.,1.,1.,1.,1.,1.,1.,1.,1.,1.,1.,1.,1.,1.,1.,1.,
1.,1.,1.,1.,1.,1.,1.,1.,1.,1.,1.,1.,1.,1.,1.,1.,1.,1.,1.,1.,1.,1.,1.,1.,
1.,1.,1.,1.,1.,1.))
REPRESENTATION_ITEM('')
);
#318=(
BOUNDED_CURVE()
B_SPLINE_CURVE(5,(#46075,#46076,#46077,#46078,#46079,#46080,#46081,#46082,
#46083,#46084,#46085,#46086,#46087,#46088,#46089,#46090,#46091,#46092,#46093,
#46094,#46095,#46096,#46097,#46098,#46099,#46100,#46101,#46102,#46103,#46104,
#46105,#46106,#46107,#46108,#46109,#46110,#46111,#46112,#46113,#46114,#46115,
#46116,#46117,#46118,#46119,#46120,#46121,#46122,#46123,#46124,#46125,#46126,
#46127,#46128,#46129,#46130,#46131,#46132,#46133,#46134,#46135,#46136,#46137,
#46138,#46139,#46140,#46141,#46142,#46143,#46144),.UNSPECIFIED.,.F.,.F.)
B_SPLINE_CURVE_WITH_KNOTS((6,1,1,1,1,1,1,1,1,1,1,1,1,1,1,1,1,1,1,1,1,1,
1,1,1,1,1,1,1,1,1,1,1,1,1,1,1,1,1,1,1,1,1,1,1,1,1,1,1,1,1,1,1,1,1,1,1,1,
1,1,1,1,1,1,1,6),(-0.994228156739712,-0.984615384615383,-0.969230769230768,
-0.953846153846152,-0.938461538461537,-0.923076923076922,-0.907692307692306,
-0.892307692307691,-0.876923076923076,-0.86153846153846,-0.846153846153845,
-0.83076923076923,-0.815384615384614,-0.799999999999999,-0.784615384615384,
-0.769230769230768,-0.753846153846153,-0.738461538461538,-0.723076923076922,
-0.707692307692307,-0.692307692307692,-0.676923076923076,-0.661538461538461,
-0.646153846153846,-0.63076923076923,-0.615384615384615,-0.6,-0.584615384615384,
-0.569230769230769,-0.553846153846154,-0.538461538461538,-0.523076923076923,
-0.507692307692308,-0.492307692307692,-0.476923076923077,-0.461538461538462,
-0.446153846153846,-0.430769230769231,-0.415384615384615,-0.4,-0.384615384615385,
-0.369230769230769,-0.353846153846154,-0.338461538461538,-0.323076923076923,
-0.307692307692308,-0.292307692307692,-0.276923076923077,-0.261538461538462,
-0.246153846153846,-0.230769230769231,-0.215384615384615,-0.2,-0.184615384615385,
-0.169230769230769,-0.153846153846154,-0.138461538461538,-0.123076923076923,
-0.107692307692308,-0.0923076923076923,-0.0769230769230769,-0.0615384615384615,
-0.0461538461538462,-0.0307692307692308,-0.0153846153846154,0.),
 .UNSPECIFIED.)
CURVE()
GEOMETRIC_REPRESENTATION_ITEM()
RATIONAL_B_SPLINE_CURVE((1.,1.,1.,1.,1.,1.,1.,1.,1.,1.,1.,1.,1.,1.,1.,1.,
1.,1.,1.,1.,1.,1.,1.,1.,1.,1.,1.,1.,1.,1.,1.,1.,1.,1.,1.,1.,1.,1.,1.,1.,
1.,1.,1.,1.,1.,1.,1.,1.,1.,1.,1.,1.,1.,1.,1.,1.,1.,1.,1.,1.,1.,1.,1.,1.,
1.,1.,1.,1.,1.,1.))
REPRESENTATION_ITEM('')
);
#319=(
BOUNDED_CURVE()
B_SPLINE_CURVE(5,(#46297,#46298,#46299,#46300,#46301,#46302,#46303,#46304,
#46305,#46306,#46307,#46308,#46309,#46310,#46311,#46312,#46313,#46314,#46315,
#46316,#46317,#46318,#46319,#46320,#46321,#46322,#46323,#46324,#46325,#46326,
#46327,#46328,#46329,#46330,#46331,#46332,#46333,#46334,#46335,#46336,#46337,
#46338,#46339,#46340,#46341,#46342,#46343,#46344,#46345,#46346,#46347,#46348,
#46349,#46350,#46351,#46352,#46353,#46354,#46355,#46356,#46357,#46358,#46359,
#46360,#46361,#46362,#46363,#46364,#46365,#46366),.UNSPECIFIED.,.F.,.F.)
B_SPLINE_CURVE_WITH_KNOTS((6,1,1,1,1,1,1,1,1,1,1,1,1,1,1,1,1,1,1,1,1,1,
1,1,1,1,1,1,1,1,1,1,1,1,1,1,1,1,1,1,1,1,1,1,1,1,1,1,1,1,1,1,1,1,1,1,1,1,
1,1,1,1,1,1,1,6),(-1.,-0.984615384615383,-0.969230769230768,-0.953846153846152,
-0.938461538461537,-0.923076923076922,-0.907692307692306,-0.892307692307691,
-0.876923076923076,-0.86153846153846,-0.846153846153845,-0.83076923076923,
-0.815384615384614,-0.799999999999999,-0.784615384615384,-0.769230769230768,
-0.753846153846153,-0.738461538461538,-0.723076923076922,-0.707692307692307,
-0.692307692307692,-0.676923076923076,-0.661538461538461,-0.646153846153846,
-0.63076923076923,-0.615384615384615,-0.6,-0.584615384615384,-0.569230769230769,
-0.553846153846154,-0.538461538461538,-0.523076923076923,-0.507692307692308,
-0.492307692307692,-0.476923076923077,-0.461538461538462,-0.446153846153846,
-0.430769230769231,-0.415384615384615,-0.4,-0.384615384615385,-0.369230769230769,
-0.353846153846154,-0.338461538461538,-0.323076923076923,-0.307692307692308,
-0.292307692307692,-0.276923076923077,-0.261538461538462,-0.246153846153846,
-0.230769230769231,-0.215384615384615,-0.2,-0.184615384615385,-0.169230769230769,
-0.153846153846154,-0.138461538461538,-0.123076923076923,-0.107692307692308,
-0.0923076923076923,-0.0769230769230769,-0.0615384615384615,-0.0461538461538462,
-0.0307692307692308,-0.0153846153846154,-0.00577184337451206),
 .UNSPECIFIED.)
CURVE()
GEOMETRIC_REPRESENTATION_ITEM()
RATIONAL_B_SPLINE_CURVE((1.,1.,1.,1.,1.,1.,1.,1.,1.,1.,1.,1.,1.,1.,1.,1.,
1.,1.,1.,1.,1.,1.,1.,1.,1.,1.,1.,1.,1.,1.,1.,1.,1.,1.,1.,1.,1.,1.,1.,1.,
1.,1.,1.,1.,1.,1.,1.,1.,1.,1.,1.,1.,1.,1.,1.,1.,1.,1.,1.,1.,1.,1.,1.,1.,
1.,1.,1.,1.,1.,1.))
REPRESENTATION_ITEM('')
);
#320=(
BOUNDED_CURVE()
B_SPLINE_CURVE(5,(#46517,#46518,#46519,#46520,#46521,#46522,#46523,#46524,
#46525,#46526,#46527,#46528,#46529,#46530,#46531,#46532,#46533,#46534,#46535,
#46536,#46537,#46538,#46539,#46540,#46541,#46542,#46543,#46544,#46545,#46546,
#46547,#46548,#46549,#46550,#46551,#46552,#46553,#46554,#46555,#46556,#46557,
#46558,#46559,#46560,#46561,#46562,#46563,#46564,#46565,#46566,#46567,#46568,
#46569,#46570,#46571,#46572,#46573,#46574,#46575,#46576,#46577,#46578,#46579,
#46580,#46581,#46582,#46583,#46584,#46585,#46586),.UNSPECIFIED.,.F.,.F.)
B_SPLINE_CURVE_WITH_KNOTS((6,1,1,1,1,1,1,1,1,1,1,1,1,1,1,1,1,1,1,1,1,1,
1,1,1,1,1,1,1,1,1,1,1,1,1,1,1,1,1,1,1,1,1,1,1,1,1,1,1,1,1,1,1,1,1,1,1,1,
1,1,1,1,1,1,1,6),(-0.994228156739717,-0.984615384615383,-0.969230769230768,
-0.953846153846152,-0.938461538461537,-0.923076923076922,-0.907692307692306,
-0.892307692307691,-0.876923076923076,-0.86153846153846,-0.846153846153845,
-0.83076923076923,-0.815384615384614,-0.799999999999999,-0.784615384615384,
-0.769230769230768,-0.753846153846153,-0.738461538461538,-0.723076923076922,
-0.707692307692307,-0.692307692307692,-0.676923076923076,-0.661538461538461,
-0.646153846153846,-0.63076923076923,-0.615384615384615,-0.6,-0.584615384615384,
-0.569230769230769,-0.553846153846154,-0.538461538461538,-0.523076923076923,
-0.507692307692308,-0.492307692307692,-0.476923076923077,-0.461538461538462,
-0.446153846153846,-0.430769230769231,-0.415384615384615,-0.4,-0.384615384615385,
-0.369230769230769,-0.353846153846154,-0.338461538461538,-0.323076923076923,
-0.307692307692308,-0.292307692307692,-0.276923076923077,-0.261538461538462,
-0.246153846153846,-0.230769230769231,-0.215384615384615,-0.2,-0.184615384615385,
-0.169230769230769,-0.153846153846154,-0.138461538461538,-0.123076923076923,
-0.107692307692308,-0.0923076923076923,-0.0769230769230769,-0.0615384615384615,
-0.0461538461538462,-0.0307692307692308,-0.0153846153846154,0.),
 .UNSPECIFIED.)
CURVE()
GEOMETRIC_REPRESENTATION_ITEM()
RATIONAL_B_SPLINE_CURVE((1.,1.,1.,1.,1.,1.,1.,1.,1.,1.,1.,1.,1.,1.,1.,1.,
1.,1.,1.,1.,1.,1.,1.,1.,1.,1.,1.,1.,1.,1.,1.,1.,1.,1.,1.,1.,1.,1.,1.,1.,
1.,1.,1.,1.,1.,1.,1.,1.,1.,1.,1.,1.,1.,1.,1.,1.,1.,1.,1.,1.,1.,1.,1.,1.,
1.,1.,1.,1.,1.,1.))
REPRESENTATION_ITEM('')
);
#321=(
BOUNDED_CURVE()
B_SPLINE_CURVE(5,(#46739,#46740,#46741,#46742,#46743,#46744,#46745,#46746,
#46747,#46748,#46749,#46750,#46751,#46752,#46753,#46754,#46755,#46756,#46757,
#46758,#46759,#46760,#46761,#46762,#46763,#46764,#46765,#46766,#46767,#46768,
#46769,#46770,#46771,#46772,#46773,#46774,#46775,#46776,#46777,#46778,#46779,
#46780,#46781,#46782,#46783,#46784,#46785,#46786,#46787,#46788,#46789,#46790,
#46791,#46792,#46793,#46794,#46795,#46796,#46797,#46798,#46799,#46800,#46801,
#46802,#46803,#46804,#46805,#46806,#46807,#46808),.UNSPECIFIED.,.F.,.F.)
B_SPLINE_CURVE_WITH_KNOTS((6,1,1,1,1,1,1,1,1,1,1,1,1,1,1,1,1,1,1,1,1,1,
1,1,1,1,1,1,1,1,1,1,1,1,1,1,1,1,1,1,1,1,1,1,1,1,1,1,1,1,1,1,1,1,1,1,1,1,
1,1,1,1,1,1,1,6),(-1.,-0.984615384615383,-0.969230769230768,-0.953846153846152,
-0.938461538461537,-0.923076923076922,-0.907692307692306,-0.892307692307691,
-0.876923076923076,-0.86153846153846,-0.846153846153845,-0.83076923076923,
-0.815384615384614,-0.799999999999999,-0.784615384615384,-0.769230769230768,
-0.753846153846153,-0.738461538461538,-0.723076923076922,-0.707692307692307,
-0.692307692307692,-0.676923076923076,-0.661538461538461,-0.646153846153846,
-0.63076923076923,-0.615384615384615,-0.6,-0.584615384615384,-0.569230769230769,
-0.553846153846154,-0.538461538461538,-0.523076923076923,-0.507692307692308,
-0.492307692307692,-0.476923076923077,-0.461538461538462,-0.446153846153846,
-0.430769230769231,-0.415384615384615,-0.4,-0.384615384615385,-0.369230769230769,
-0.353846153846154,-0.338461538461538,-0.323076923076923,-0.307692307692308,
-0.292307692307692,-0.276923076923077,-0.261538461538462,-0.246153846153846,
-0.230769230769231,-0.215384615384615,-0.2,-0.184615384615385,-0.169230769230769,
-0.153846153846154,-0.138461538461538,-0.123076923076923,-0.107692307692308,
-0.0923076923076923,-0.0769230769230769,-0.0615384615384615,-0.0461538461538462,
-0.0307692307692308,-0.0153846153846154,-0.00577184337448646),
 .UNSPECIFIED.)
CURVE()
GEOMETRIC_REPRESENTATION_ITEM()
RATIONAL_B_SPLINE_CURVE((1.,1.,1.,1.,1.,1.,1.,1.,1.,1.,1.,1.,1.,1.,1.,1.,
1.,1.,1.,1.,1.,1.,1.,1.,1.,1.,1.,1.,1.,1.,1.,1.,1.,1.,1.,1.,1.,1.,1.,1.,
1.,1.,1.,1.,1.,1.,1.,1.,1.,1.,1.,1.,1.,1.,1.,1.,1.,1.,1.,1.,1.,1.,1.,1.,
1.,1.,1.,1.,1.,1.))
REPRESENTATION_ITEM('')
);
#322=(
BOUNDED_CURVE()
B_SPLINE_CURVE(5,(#46959,#46960,#46961,#46962,#46963,#46964,#46965,#46966,
#46967,#46968,#46969,#46970,#46971,#46972,#46973,#46974,#46975,#46976,#46977,
#46978,#46979,#46980,#46981,#46982,#46983,#46984,#46985,#46986,#46987,#46988,
#46989,#46990,#46991,#46992,#46993,#46994,#46995,#46996,#46997,#46998,#46999,
#47000,#47001,#47002,#47003,#47004,#47005,#47006,#47007,#47008,#47009,#47010,
#47011,#47012,#47013,#47014,#47015,#47016,#47017,#47018,#47019,#47020,#47021,
#47022,#47023,#47024,#47025,#47026,#47027,#47028),.UNSPECIFIED.,.F.,.F.)
B_SPLINE_CURVE_WITH_KNOTS((6,1,1,1,1,1,1,1,1,1,1,1,1,1,1,1,1,1,1,1,1,1,
1,1,1,1,1,1,1,1,1,1,1,1,1,1,1,1,1,1,1,1,1,1,1,1,1,1,1,1,1,1,1,1,1,1,1,1,
1,1,1,1,1,1,1,6),(-0.994228156739708,-0.984615384615383,-0.969230769230768,
-0.953846153846152,-0.938461538461537,-0.923076923076922,-0.907692307692306,
-0.892307692307691,-0.876923076923076,-0.86153846153846,-0.846153846153845,
-0.83076923076923,-0.815384615384614,-0.799999999999999,-0.784615384615384,
-0.769230769230768,-0.753846153846153,-0.738461538461538,-0.723076923076922,
-0.707692307692307,-0.692307692307692,-0.676923076923076,-0.661538461538461,
-0.646153846153846,-0.63076923076923,-0.615384615384615,-0.6,-0.584615384615384,
-0.569230769230769,-0.553846153846154,-0.538461538461538,-0.523076923076923,
-0.507692307692308,-0.492307692307692,-0.476923076923077,-0.461538461538462,
-0.446153846153846,-0.430769230769231,-0.415384615384615,-0.4,-0.384615384615385,
-0.369230769230769,-0.353846153846154,-0.338461538461538,-0.323076923076923,
-0.307692307692308,-0.292307692307692,-0.276923076923077,-0.261538461538462,
-0.246153846153846,-0.230769230769231,-0.215384615384615,-0.2,-0.184615384615385,
-0.169230769230769,-0.153846153846154,-0.138461538461538,-0.123076923076923,
-0.107692307692308,-0.0923076923076923,-0.0769230769230769,-0.0615384615384615,
-0.0461538461538462,-0.0307692307692308,-0.0153846153846154,0.),
 .UNSPECIFIED.)
CURVE()
GEOMETRIC_REPRESENTATION_ITEM()
RATIONAL_B_SPLINE_CURVE((1.,1.,1.,1.,1.,1.,1.,1.,1.,1.,1.,1.,1.,1.,1.,1.,
1.,1.,1.,1.,1.,1.,1.,1.,1.,1.,1.,1.,1.,1.,1.,1.,1.,1.,1.,1.,1.,1.,1.,1.,
1.,1.,1.,1.,1.,1.,1.,1.,1.,1.,1.,1.,1.,1.,1.,1.,1.,1.,1.,1.,1.,1.,1.,1.,
1.,1.,1.,1.,1.,1.))
REPRESENTATION_ITEM('')
);
#323=(
BOUNDED_CURVE()
B_SPLINE_CURVE(5,(#47181,#47182,#47183,#47184,#47185,#47186,#47187,#47188,
#47189,#47190,#47191,#47192,#47193,#47194,#47195,#47196,#47197,#47198,#47199,
#47200,#47201,#47202,#47203,#47204,#47205,#47206,#47207,#47208,#47209,#47210,
#47211,#47212,#47213,#47214,#47215,#47216,#47217,#47218,#47219,#47220,#47221,
#47222,#47223,#47224,#47225,#47226,#47227,#47228,#47229,#47230,#47231,#47232,
#47233,#47234,#47235,#47236,#47237,#47238,#47239,#47240,#47241,#47242,#47243,
#47244,#47245,#47246,#47247,#47248,#47249,#47250),.UNSPECIFIED.,.F.,.F.)
B_SPLINE_CURVE_WITH_KNOTS((6,1,1,1,1,1,1,1,1,1,1,1,1,1,1,1,1,1,1,1,1,1,
1,1,1,1,1,1,1,1,1,1,1,1,1,1,1,1,1,1,1,1,1,1,1,1,1,1,1,1,1,1,1,1,1,1,1,1,
1,1,1,1,1,1,1,6),(-1.,-0.984615384615383,-0.969230769230768,-0.953846153846152,
-0.938461538461537,-0.923076923076922,-0.907692307692306,-0.892307692307691,
-0.876923076923076,-0.86153846153846,-0.846153846153845,-0.83076923076923,
-0.815384615384614,-0.799999999999999,-0.784615384615384,-0.769230769230768,
-0.753846153846153,-0.738461538461538,-0.723076923076922,-0.707692307692307,
-0.692307692307692,-0.676923076923076,-0.661538461538461,-0.646153846153846,
-0.63076923076923,-0.615384615384615,-0.6,-0.584615384615384,-0.569230769230769,
-0.553846153846154,-0.538461538461538,-0.523076923076923,-0.507692307692308,
-0.492307692307692,-0.476923076923077,-0.461538461538462,-0.446153846153846,
-0.430769230769231,-0.415384615384615,-0.4,-0.384615384615385,-0.369230769230769,
-0.353846153846154,-0.338461538461538,-0.323076923076923,-0.307692307692308,
-0.292307692307692,-0.276923076923077,-0.261538461538462,-0.246153846153846,
-0.230769230769231,-0.215384615384615,-0.2,-0.184615384615385,-0.169230769230769,
-0.153846153846154,-0.138461538461538,-0.123076923076923,-0.107692307692308,
-0.0923076923076923,-0.0769230769230769,-0.0615384615384615,-0.0461538461538462,
-0.0307692307692308,-0.0153846153846154,-0.00577184337451626),
 .UNSPECIFIED.)
CURVE()
GEOMETRIC_REPRESENTATION_ITEM()
RATIONAL_B_SPLINE_CURVE((1.,1.,1.,1.,1.,1.,1.,1.,1.,1.,1.,1.,1.,1.,1.,1.,
1.,1.,1.,1.,1.,1.,1.,1.,1.,1.,1.,1.,1.,1.,1.,1.,1.,1.,1.,1.,1.,1.,1.,1.,
1.,1.,1.,1.,1.,1.,1.,1.,1.,1.,1.,1.,1.,1.,1.,1.,1.,1.,1.,1.,1.,1.,1.,1.,
1.,1.,1.,1.,1.,1.))
REPRESENTATION_ITEM('')
);
#324=(
BOUNDED_CURVE()
B_SPLINE_CURVE(5,(#47401,#47402,#47403,#47404,#47405,#47406,#47407,#47408,
#47409,#47410,#47411,#47412,#47413,#47414,#47415,#47416,#47417,#47418,#47419,
#47420,#47421,#47422,#47423,#47424,#47425,#47426,#47427,#47428,#47429,#47430,
#47431,#47432,#47433,#47434,#47435,#47436,#47437,#47438,#47439,#47440,#47441,
#47442,#47443,#47444,#47445,#47446,#47447,#47448,#47449,#47450,#47451,#47452,
#47453,#47454,#47455,#47456,#47457,#47458,#47459,#47460,#47461,#47462,#47463,
#47464,#47465,#47466,#47467,#47468,#47469,#47470),.UNSPECIFIED.,.F.,.F.)
B_SPLINE_CURVE_WITH_KNOTS((6,1,1,1,1,1,1,1,1,1,1,1,1,1,1,1,1,1,1,1,1,1,
1,1,1,1,1,1,1,1,1,1,1,1,1,1,1,1,1,1,1,1,1,1,1,1,1,1,1,1,1,1,1,1,1,1,1,1,
1,1,1,1,1,1,1,6),(-0.994228156739708,-0.984615384615383,-0.969230769230768,
-0.953846153846152,-0.938461538461537,-0.923076923076922,-0.907692307692306,
-0.892307692307691,-0.876923076923076,-0.86153846153846,-0.846153846153845,
-0.83076923076923,-0.815384615384614,-0.799999999999999,-0.784615384615384,
-0.769230769230768,-0.753846153846153,-0.738461538461538,-0.723076923076922,
-0.707692307692307,-0.692307692307692,-0.676923076923076,-0.661538461538461,
-0.646153846153846,-0.63076923076923,-0.615384615384615,-0.6,-0.584615384615384,
-0.569230769230769,-0.553846153846154,-0.538461538461538,-0.523076923076923,
-0.507692307692308,-0.492307692307692,-0.476923076923077,-0.461538461538462,
-0.446153846153846,-0.430769230769231,-0.415384615384615,-0.4,-0.384615384615385,
-0.369230769230769,-0.353846153846154,-0.338461538461538,-0.323076923076923,
-0.307692307692308,-0.292307692307692,-0.276923076923077,-0.261538461538462,
-0.246153846153846,-0.230769230769231,-0.215384615384615,-0.2,-0.184615384615385,
-0.169230769230769,-0.153846153846154,-0.138461538461538,-0.123076923076923,
-0.107692307692308,-0.0923076923076923,-0.0769230769230769,-0.0615384615384615,
-0.0461538461538462,-0.0307692307692308,-0.0153846153846154,0.),
 .UNSPECIFIED.)
CURVE()
GEOMETRIC_REPRESENTATION_ITEM()
RATIONAL_B_SPLINE_CURVE((1.,1.,1.,1.,1.,1.,1.,1.,1.,1.,1.,1.,1.,1.,1.,1.,
1.,1.,1.,1.,1.,1.,1.,1.,1.,1.,1.,1.,1.,1.,1.,1.,1.,1.,1.,1.,1.,1.,1.,1.,
1.,1.,1.,1.,1.,1.,1.,1.,1.,1.,1.,1.,1.,1.,1.,1.,1.,1.,1.,1.,1.,1.,1.,1.,
1.,1.,1.,1.,1.,1.))
REPRESENTATION_ITEM('')
);
#325=(
BOUNDED_CURVE()
B_SPLINE_CURVE(5,(#47623,#47624,#47625,#47626,#47627,#47628,#47629,#47630,
#47631,#47632,#47633,#47634,#47635,#47636,#47637,#47638,#47639,#47640,#47641,
#47642,#47643,#47644,#47645,#47646,#47647,#47648,#47649,#47650,#47651,#47652,
#47653,#47654,#47655,#47656,#47657,#47658,#47659,#47660,#47661,#47662,#47663,
#47664,#47665,#47666,#47667,#47668,#47669,#47670,#47671,#47672,#47673,#47674,
#47675,#47676,#47677,#47678,#47679,#47680,#47681,#47682,#47683,#47684,#47685,
#47686,#47687,#47688,#47689,#47690,#47691,#47692),.UNSPECIFIED.,.F.,.F.)
B_SPLINE_CURVE_WITH_KNOTS((6,1,1,1,1,1,1,1,1,1,1,1,1,1,1,1,1,1,1,1,1,1,
1,1,1,1,1,1,1,1,1,1,1,1,1,1,1,1,1,1,1,1,1,1,1,1,1,1,1,1,1,1,1,1,1,1,1,1,
1,1,1,1,1,1,1,6),(-1.,-0.984615384615383,-0.969230769230768,-0.953846153846152,
-0.938461538461537,-0.923076923076922,-0.907692307692306,-0.892307692307691,
-0.876923076923076,-0.86153846153846,-0.846153846153845,-0.83076923076923,
-0.815384615384614,-0.799999999999999,-0.784615384615384,-0.769230769230768,
-0.753846153846153,-0.738461538461538,-0.723076923076922,-0.707692307692307,
-0.692307692307692,-0.676923076923076,-0.661538461538461,-0.646153846153846,
-0.63076923076923,-0.615384615384615,-0.6,-0.584615384615384,-0.569230769230769,
-0.553846153846154,-0.538461538461538,-0.523076923076923,-0.507692307692308,
-0.492307692307692,-0.476923076923077,-0.461538461538462,-0.446153846153846,
-0.430769230769231,-0.415384615384615,-0.4,-0.384615384615385,-0.369230769230769,
-0.353846153846154,-0.338461538461538,-0.323076923076923,-0.307692307692308,
-0.292307692307692,-0.276923076923077,-0.261538461538462,-0.246153846153846,
-0.230769230769231,-0.215384615384615,-0.2,-0.184615384615385,-0.169230769230769,
-0.153846153846154,-0.138461538461538,-0.123076923076923,-0.107692307692308,
-0.0923076923076923,-0.0769230769230769,-0.0615384615384615,-0.0461538461538462,
-0.0307692307692308,-0.0153846153846154,-0.00577184337451372),
 .UNSPECIFIED.)
CURVE()
GEOMETRIC_REPRESENTATION_ITEM()
RATIONAL_B_SPLINE_CURVE((1.,1.,1.,1.,1.,1.,1.,1.,1.,1.,1.,1.,1.,1.,1.,1.,
1.,1.,1.,1.,1.,1.,1.,1.,1.,1.,1.,1.,1.,1.,1.,1.,1.,1.,1.,1.,1.,1.,1.,1.,
1.,1.,1.,1.,1.,1.,1.,1.,1.,1.,1.,1.,1.,1.,1.,1.,1.,1.,1.,1.,1.,1.,1.,1.,
1.,1.,1.,1.,1.,1.))
REPRESENTATION_ITEM('')
);
#326=(
BOUNDED_CURVE()
B_SPLINE_CURVE(5,(#47843,#47844,#47845,#47846,#47847,#47848,#47849,#47850,
#47851,#47852,#47853,#47854,#47855,#47856,#47857,#47858,#47859,#47860,#47861,
#47862,#47863,#47864,#47865,#47866,#47867,#47868,#47869,#47870,#47871,#47872,
#47873,#47874,#47875,#47876,#47877,#47878,#47879,#47880,#47881,#47882,#47883,
#47884,#47885,#47886,#47887,#47888,#47889,#47890,#47891,#47892,#47893,#47894,
#47895,#47896,#47897,#47898,#47899,#47900,#47901,#47902,#47903,#47904,#47905,
#47906,#47907,#47908,#47909,#47910,#47911,#47912),.UNSPECIFIED.,.F.,.F.)
B_SPLINE_CURVE_WITH_KNOTS((6,1,1,1,1,1,1,1,1,1,1,1,1,1,1,1,1,1,1,1,1,1,
1,1,1,1,1,1,1,1,1,1,1,1,1,1,1,1,1,1,1,1,1,1,1,1,1,1,1,1,1,1,1,1,1,1,1,1,
1,1,1,1,1,1,1,6),(-0.994228156739703,-0.984615384615383,-0.969230769230768,
-0.953846153846152,-0.938461538461537,-0.923076923076922,-0.907692307692306,
-0.892307692307691,-0.876923076923076,-0.86153846153846,-0.846153846153845,
-0.83076923076923,-0.815384615384614,-0.799999999999999,-0.784615384615384,
-0.769230769230768,-0.753846153846153,-0.738461538461538,-0.723076923076922,
-0.707692307692307,-0.692307692307692,-0.676923076923076,-0.661538461538461,
-0.646153846153846,-0.63076923076923,-0.615384615384615,-0.6,-0.584615384615384,
-0.569230769230769,-0.553846153846154,-0.538461538461538,-0.523076923076923,
-0.507692307692308,-0.492307692307692,-0.476923076923077,-0.461538461538462,
-0.446153846153846,-0.430769230769231,-0.415384615384615,-0.4,-0.384615384615385,
-0.369230769230769,-0.353846153846154,-0.338461538461538,-0.323076923076923,
-0.307692307692308,-0.292307692307692,-0.276923076923077,-0.261538461538462,
-0.246153846153846,-0.230769230769231,-0.215384615384615,-0.2,-0.184615384615385,
-0.169230769230769,-0.153846153846154,-0.138461538461538,-0.123076923076923,
-0.107692307692308,-0.0923076923076923,-0.0769230769230769,-0.0615384615384615,
-0.0461538461538462,-0.0307692307692308,-0.0153846153846154,0.),
 .UNSPECIFIED.)
CURVE()
GEOMETRIC_REPRESENTATION_ITEM()
RATIONAL_B_SPLINE_CURVE((1.,1.,1.,1.,1.,1.,1.,1.,1.,1.,1.,1.,1.,1.,1.,1.,
1.,1.,1.,1.,1.,1.,1.,1.,1.,1.,1.,1.,1.,1.,1.,1.,1.,1.,1.,1.,1.,1.,1.,1.,
1.,1.,1.,1.,1.,1.,1.,1.,1.,1.,1.,1.,1.,1.,1.,1.,1.,1.,1.,1.,1.,1.,1.,1.,
1.,1.,1.,1.,1.,1.))
REPRESENTATION_ITEM('')
);
#327=(
BOUNDED_CURVE()
B_SPLINE_CURVE(5,(#48065,#48066,#48067,#48068,#48069,#48070,#48071,#48072,
#48073,#48074,#48075,#48076,#48077,#48078,#48079,#48080,#48081,#48082,#48083,
#48084,#48085,#48086,#48087,#48088,#48089,#48090,#48091,#48092,#48093,#48094,
#48095,#48096,#48097,#48098,#48099,#48100,#48101,#48102,#48103,#48104,#48105,
#48106,#48107,#48108,#48109,#48110,#48111,#48112,#48113,#48114,#48115,#48116,
#48117,#48118,#48119,#48120,#48121,#48122,#48123,#48124,#48125,#48126,#48127,
#48128,#48129,#48130,#48131,#48132,#48133,#48134),.UNSPECIFIED.,.F.,.F.)
B_SPLINE_CURVE_WITH_KNOTS((6,1,1,1,1,1,1,1,1,1,1,1,1,1,1,1,1,1,1,1,1,1,
1,1,1,1,1,1,1,1,1,1,1,1,1,1,1,1,1,1,1,1,1,1,1,1,1,1,1,1,1,1,1,1,1,1,1,1,
1,1,1,1,1,1,1,6),(-1.,-0.984615384615383,-0.969230769230768,-0.953846153846152,
-0.938461538461537,-0.923076923076922,-0.907692307692306,-0.892307692307691,
-0.876923076923076,-0.86153846153846,-0.846153846153845,-0.83076923076923,
-0.815384615384614,-0.799999999999999,-0.784615384615384,-0.769230769230768,
-0.753846153846153,-0.738461538461538,-0.723076923076922,-0.707692307692307,
-0.692307692307692,-0.676923076923076,-0.661538461538461,-0.646153846153846,
-0.63076923076923,-0.615384615384615,-0.6,-0.584615384615384,-0.569230769230769,
-0.553846153846154,-0.538461538461538,-0.523076923076923,-0.507692307692308,
-0.492307692307692,-0.476923076923077,-0.461538461538462,-0.446153846153846,
-0.430769230769231,-0.415384615384615,-0.4,-0.384615384615385,-0.369230769230769,
-0.353846153846154,-0.338461538461538,-0.323076923076923,-0.307692307692308,
-0.292307692307692,-0.276923076923077,-0.261538461538462,-0.246153846153846,
-0.230769230769231,-0.215384615384615,-0.2,-0.184615384615385,-0.169230769230769,
-0.153846153846154,-0.138461538461538,-0.123076923076923,-0.107692307692308,
-0.0923076923076923,-0.0769230769230769,-0.0615384615384615,-0.0461538461538462,
-0.0307692307692308,-0.0153846153846154,-0.00577184337451698),
 .UNSPECIFIED.)
CURVE()
GEOMETRIC_REPRESENTATION_ITEM()
RATIONAL_B_SPLINE_CURVE((1.,1.,1.,1.,1.,1.,1.,1.,1.,1.,1.,1.,1.,1.,1.,1.,
1.,1.,1.,1.,1.,1.,1.,1.,1.,1.,1.,1.,1.,1.,1.,1.,1.,1.,1.,1.,1.,1.,1.,1.,
1.,1.,1.,1.,1.,1.,1.,1.,1.,1.,1.,1.,1.,1.,1.,1.,1.,1.,1.,1.,1.,1.,1.,1.,
1.,1.,1.,1.,1.,1.))
REPRESENTATION_ITEM('')
);
#328=(
BOUNDED_CURVE()
B_SPLINE_CURVE(5,(#48285,#48286,#48287,#48288,#48289,#48290,#48291,#48292,
#48293,#48294,#48295,#48296,#48297,#48298,#48299,#48300,#48301,#48302,#48303,
#48304,#48305,#48306,#48307,#48308,#48309,#48310,#48311,#48312,#48313,#48314,
#48315,#48316,#48317,#48318,#48319,#48320,#48321,#48322,#48323,#48324,#48325,
#48326,#48327,#48328,#48329,#48330,#48331,#48332,#48333,#48334,#48335,#48336,
#48337,#48338,#48339,#48340,#48341,#48342,#48343,#48344,#48345,#48346,#48347,
#48348,#48349,#48350,#48351,#48352,#48353,#48354),.UNSPECIFIED.,.F.,.F.)
B_SPLINE_CURVE_WITH_KNOTS((6,1,1,1,1,1,1,1,1,1,1,1,1,1,1,1,1,1,1,1,1,1,
1,1,1,1,1,1,1,1,1,1,1,1,1,1,1,1,1,1,1,1,1,1,1,1,1,1,1,1,1,1,1,1,1,1,1,1,
1,1,1,1,1,1,1,6),(-0.994228156739706,-0.984615384615383,-0.969230769230768,
-0.953846153846152,-0.938461538461537,-0.923076923076922,-0.907692307692306,
-0.892307692307691,-0.876923076923076,-0.86153846153846,-0.846153846153845,
-0.83076923076923,-0.815384615384614,-0.799999999999999,-0.784615384615384,
-0.769230769230768,-0.753846153846153,-0.738461538461538,-0.723076923076922,
-0.707692307692307,-0.692307692307692,-0.676923076923076,-0.661538461538461,
-0.646153846153846,-0.63076923076923,-0.615384615384615,-0.6,-0.584615384615384,
-0.569230769230769,-0.553846153846154,-0.538461538461538,-0.523076923076923,
-0.507692307692308,-0.492307692307692,-0.476923076923077,-0.461538461538462,
-0.446153846153846,-0.430769230769231,-0.415384615384615,-0.4,-0.384615384615385,
-0.369230769230769,-0.353846153846154,-0.338461538461538,-0.323076923076923,
-0.307692307692308,-0.292307692307692,-0.276923076923077,-0.261538461538462,
-0.246153846153846,-0.230769230769231,-0.215384615384615,-0.2,-0.184615384615385,
-0.169230769230769,-0.153846153846154,-0.138461538461538,-0.123076923076923,
-0.107692307692308,-0.0923076923076923,-0.0769230769230769,-0.0615384615384615,
-0.0461538461538462,-0.0307692307692308,-0.0153846153846154,0.),
 .UNSPECIFIED.)
CURVE()
GEOMETRIC_REPRESENTATION_ITEM()
RATIONAL_B_SPLINE_CURVE((1.,1.,1.,1.,1.,1.,1.,1.,1.,1.,1.,1.,1.,1.,1.,1.,
1.,1.,1.,1.,1.,1.,1.,1.,1.,1.,1.,1.,1.,1.,1.,1.,1.,1.,1.,1.,1.,1.,1.,1.,
1.,1.,1.,1.,1.,1.,1.,1.,1.,1.,1.,1.,1.,1.,1.,1.,1.,1.,1.,1.,1.,1.,1.,1.,
1.,1.,1.,1.,1.,1.))
REPRESENTATION_ITEM('')
);
#329=(
BOUNDED_CURVE()
B_SPLINE_CURVE(5,(#48507,#48508,#48509,#48510,#48511,#48512,#48513,#48514,
#48515,#48516,#48517,#48518,#48519,#48520,#48521,#48522,#48523,#48524,#48525,
#48526,#48527,#48528,#48529,#48530,#48531,#48532,#48533,#48534,#48535,#48536,
#48537,#48538,#48539,#48540,#48541,#48542,#48543,#48544,#48545,#48546,#48547,
#48548,#48549,#48550,#48551,#48552,#48553,#48554,#48555,#48556,#48557,#48558,
#48559,#48560,#48561,#48562,#48563,#48564,#48565,#48566,#48567,#48568,#48569,
#48570,#48571,#48572,#48573,#48574,#48575,#48576),.UNSPECIFIED.,.F.,.F.)
B_SPLINE_CURVE_WITH_KNOTS((6,1,1,1,1,1,1,1,1,1,1,1,1,1,1,1,1,1,1,1,1,1,
1,1,1,1,1,1,1,1,1,1,1,1,1,1,1,1,1,1,1,1,1,1,1,1,1,1,1,1,1,1,1,1,1,1,1,1,
1,1,1,1,1,1,1,6),(-1.,-0.984615384615383,-0.969230769230768,-0.953846153846152,
-0.938461538461537,-0.923076923076922,-0.907692307692306,-0.892307692307691,
-0.876923076923076,-0.86153846153846,-0.846153846153845,-0.83076923076923,
-0.815384615384614,-0.799999999999999,-0.784615384615384,-0.769230769230768,
-0.753846153846153,-0.738461538461538,-0.723076923076922,-0.707692307692307,
-0.692307692307692,-0.676923076923076,-0.661538461538461,-0.646153846153846,
-0.63076923076923,-0.615384615384615,-0.6,-0.584615384615384,-0.569230769230769,
-0.553846153846154,-0.538461538461538,-0.523076923076923,-0.507692307692308,
-0.492307692307692,-0.476923076923077,-0.461538461538462,-0.446153846153846,
-0.430769230769231,-0.415384615384615,-0.4,-0.384615384615385,-0.369230769230769,
-0.353846153846154,-0.338461538461538,-0.323076923076923,-0.307692307692308,
-0.292307692307692,-0.276923076923077,-0.261538461538462,-0.246153846153846,
-0.230769230769231,-0.215384615384615,-0.2,-0.184615384615385,-0.169230769230769,
-0.153846153846154,-0.138461538461538,-0.123076923076923,-0.107692307692308,
-0.0923076923076923,-0.0769230769230769,-0.0615384615384615,-0.0461538461538462,
-0.0307692307692308,-0.0153846153846154,-0.00577184337452512),
 .UNSPECIFIED.)
CURVE()
GEOMETRIC_REPRESENTATION_ITEM()
RATIONAL_B_SPLINE_CURVE((1.,1.,1.,1.,1.,1.,1.,1.,1.,1.,1.,1.,1.,1.,1.,1.,
1.,1.,1.,1.,1.,1.,1.,1.,1.,1.,1.,1.,1.,1.,1.,1.,1.,1.,1.,1.,1.,1.,1.,1.,
1.,1.,1.,1.,1.,1.,1.,1.,1.,1.,1.,1.,1.,1.,1.,1.,1.,1.,1.,1.,1.,1.,1.,1.,
1.,1.,1.,1.,1.,1.))
REPRESENTATION_ITEM('')
);
#330=(
BOUNDED_CURVE()
B_SPLINE_CURVE(5,(#48727,#48728,#48729,#48730,#48731,#48732,#48733,#48734,
#48735,#48736,#48737,#48738,#48739,#48740,#48741,#48742,#48743,#48744,#48745,
#48746,#48747,#48748,#48749,#48750,#48751,#48752,#48753,#48754,#48755,#48756,
#48757,#48758,#48759,#48760,#48761,#48762,#48763,#48764,#48765,#48766,#48767,
#48768,#48769,#48770,#48771,#48772,#48773,#48774,#48775,#48776,#48777,#48778,
#48779,#48780,#48781,#48782,#48783,#48784,#48785,#48786,#48787,#48788,#48789,
#48790,#48791,#48792,#48793,#48794,#48795,#48796),.UNSPECIFIED.,.F.,.F.)
B_SPLINE_CURVE_WITH_KNOTS((6,1,1,1,1,1,1,1,1,1,1,1,1,1,1,1,1,1,1,1,1,1,
1,1,1,1,1,1,1,1,1,1,1,1,1,1,1,1,1,1,1,1,1,1,1,1,1,1,1,1,1,1,1,1,1,1,1,1,
1,1,1,1,1,1,1,6),(-0.994228156739713,-0.984615384615383,-0.969230769230768,
-0.953846153846152,-0.938461538461537,-0.923076923076922,-0.907692307692306,
-0.892307692307691,-0.876923076923076,-0.86153846153846,-0.846153846153845,
-0.83076923076923,-0.815384615384614,-0.799999999999999,-0.784615384615384,
-0.769230769230768,-0.753846153846153,-0.738461538461538,-0.723076923076922,
-0.707692307692307,-0.692307692307692,-0.676923076923076,-0.661538461538461,
-0.646153846153846,-0.63076923076923,-0.615384615384615,-0.6,-0.584615384615384,
-0.569230769230769,-0.553846153846154,-0.538461538461538,-0.523076923076923,
-0.507692307692308,-0.492307692307692,-0.476923076923077,-0.461538461538462,
-0.446153846153846,-0.430769230769231,-0.415384615384615,-0.4,-0.384615384615385,
-0.369230769230769,-0.353846153846154,-0.338461538461538,-0.323076923076923,
-0.307692307692308,-0.292307692307692,-0.276923076923077,-0.261538461538462,
-0.246153846153846,-0.230769230769231,-0.215384615384615,-0.2,-0.184615384615385,
-0.169230769230769,-0.153846153846154,-0.138461538461538,-0.123076923076923,
-0.107692307692308,-0.0923076923076923,-0.0769230769230769,-0.0615384615384615,
-0.0461538461538462,-0.0307692307692308,-0.0153846153846154,0.),
 .UNSPECIFIED.)
CURVE()
GEOMETRIC_REPRESENTATION_ITEM()
RATIONAL_B_SPLINE_CURVE((1.,1.,1.,1.,1.,1.,1.,1.,1.,1.,1.,1.,1.,1.,1.,1.,
1.,1.,1.,1.,1.,1.,1.,1.,1.,1.,1.,1.,1.,1.,1.,1.,1.,1.,1.,1.,1.,1.,1.,1.,
1.,1.,1.,1.,1.,1.,1.,1.,1.,1.,1.,1.,1.,1.,1.,1.,1.,1.,1.,1.,1.,1.,1.,1.,
1.,1.,1.,1.,1.,1.))
REPRESENTATION_ITEM('')
);
#331=(
BOUNDED_CURVE()
B_SPLINE_CURVE(5,(#48949,#48950,#48951,#48952,#48953,#48954,#48955,#48956,
#48957,#48958,#48959,#48960,#48961,#48962,#48963,#48964,#48965,#48966,#48967,
#48968,#48969,#48970,#48971,#48972,#48973,#48974,#48975,#48976,#48977,#48978,
#48979,#48980,#48981,#48982,#48983,#48984,#48985,#48986,#48987,#48988,#48989,
#48990,#48991,#48992,#48993,#48994,#48995,#48996,#48997,#48998,#48999,#49000,
#49001,#49002,#49003,#49004,#49005,#49006,#49007,#49008,#49009,#49010,#49011,
#49012,#49013,#49014,#49015,#49016,#49017,#49018),.UNSPECIFIED.,.F.,.F.)
B_SPLINE_CURVE_WITH_KNOTS((6,1,1,1,1,1,1,1,1,1,1,1,1,1,1,1,1,1,1,1,1,1,
1,1,1,1,1,1,1,1,1,1,1,1,1,1,1,1,1,1,1,1,1,1,1,1,1,1,1,1,1,1,1,1,1,1,1,1,
1,1,1,1,1,1,1,6),(-1.,-0.984615384615383,-0.969230769230768,-0.953846153846152,
-0.938461538461537,-0.923076923076922,-0.907692307692306,-0.892307692307691,
-0.876923076923076,-0.86153846153846,-0.846153846153845,-0.83076923076923,
-0.815384615384614,-0.799999999999999,-0.784615384615384,-0.769230769230768,
-0.753846153846153,-0.738461538461538,-0.723076923076922,-0.707692307692307,
-0.692307692307692,-0.676923076923076,-0.661538461538461,-0.646153846153846,
-0.63076923076923,-0.615384615384615,-0.6,-0.584615384615384,-0.569230769230769,
-0.553846153846154,-0.538461538461538,-0.523076923076923,-0.507692307692308,
-0.492307692307692,-0.476923076923077,-0.461538461538462,-0.446153846153846,
-0.430769230769231,-0.415384615384615,-0.4,-0.384615384615385,-0.369230769230769,
-0.353846153846154,-0.338461538461538,-0.323076923076923,-0.307692307692308,
-0.292307692307692,-0.276923076923077,-0.261538461538462,-0.246153846153846,
-0.230769230769231,-0.215384615384615,-0.2,-0.184615384615385,-0.169230769230769,
-0.153846153846154,-0.138461538461538,-0.123076923076923,-0.107692307692308,
-0.0923076923076923,-0.0769230769230769,-0.0615384615384615,-0.0461538461538462,
-0.0307692307692308,-0.0153846153846154,-0.00577184337450204),
 .UNSPECIFIED.)
CURVE()
GEOMETRIC_REPRESENTATION_ITEM()
RATIONAL_B_SPLINE_CURVE((1.,1.,1.,1.,1.,1.,1.,1.,1.,1.,1.,1.,1.,1.,1.,1.,
1.,1.,1.,1.,1.,1.,1.,1.,1.,1.,1.,1.,1.,1.,1.,1.,1.,1.,1.,1.,1.,1.,1.,1.,
1.,1.,1.,1.,1.,1.,1.,1.,1.,1.,1.,1.,1.,1.,1.,1.,1.,1.,1.,1.,1.,1.,1.,1.,
1.,1.,1.,1.,1.,1.))
REPRESENTATION_ITEM('')
);
#332=(
BOUNDED_CURVE()
B_SPLINE_CURVE(5,(#49169,#49170,#49171,#49172,#49173,#49174,#49175,#49176,
#49177,#49178,#49179,#49180,#49181,#49182,#49183,#49184,#49185,#49186,#49187,
#49188,#49189,#49190,#49191,#49192,#49193,#49194,#49195,#49196,#49197,#49198,
#49199,#49200,#49201,#49202,#49203,#49204,#49205,#49206,#49207,#49208,#49209,
#49210,#49211,#49212,#49213,#49214,#49215,#49216,#49217,#49218,#49219,#49220,
#49221,#49222,#49223,#49224,#49225,#49226,#49227,#49228,#49229,#49230,#49231,
#49232,#49233,#49234,#49235,#49236,#49237,#49238),.UNSPECIFIED.,.F.,.F.)
B_SPLINE_CURVE_WITH_KNOTS((6,1,1,1,1,1,1,1,1,1,1,1,1,1,1,1,1,1,1,1,1,1,
1,1,1,1,1,1,1,1,1,1,1,1,1,1,1,1,1,1,1,1,1,1,1,1,1,1,1,1,1,1,1,1,1,1,1,1,
1,1,1,1,1,1,1,6),(-0.99422815673972,-0.984615384615383,-0.969230769230768,
-0.953846153846152,-0.938461538461537,-0.923076923076922,-0.907692307692306,
-0.892307692307691,-0.876923076923076,-0.86153846153846,-0.846153846153845,
-0.83076923076923,-0.815384615384614,-0.799999999999999,-0.784615384615384,
-0.769230769230768,-0.753846153846153,-0.738461538461538,-0.723076923076922,
-0.707692307692307,-0.692307692307692,-0.676923076923076,-0.661538461538461,
-0.646153846153846,-0.63076923076923,-0.615384615384615,-0.6,-0.584615384615384,
-0.569230769230769,-0.553846153846154,-0.538461538461538,-0.523076923076923,
-0.507692307692308,-0.492307692307692,-0.476923076923077,-0.461538461538462,
-0.446153846153846,-0.430769230769231,-0.415384615384615,-0.4,-0.384615384615385,
-0.369230769230769,-0.353846153846154,-0.338461538461538,-0.323076923076923,
-0.307692307692308,-0.292307692307692,-0.276923076923077,-0.261538461538462,
-0.246153846153846,-0.230769230769231,-0.215384615384615,-0.2,-0.184615384615385,
-0.169230769230769,-0.153846153846154,-0.138461538461538,-0.123076923076923,
-0.107692307692308,-0.0923076923076923,-0.0769230769230769,-0.0615384615384615,
-0.0461538461538462,-0.0307692307692308,-0.0153846153846154,0.),
 .UNSPECIFIED.)
CURVE()
GEOMETRIC_REPRESENTATION_ITEM()
RATIONAL_B_SPLINE_CURVE((1.,1.,1.,1.,1.,1.,1.,1.,1.,1.,1.,1.,1.,1.,1.,1.,
1.,1.,1.,1.,1.,1.,1.,1.,1.,1.,1.,1.,1.,1.,1.,1.,1.,1.,1.,1.,1.,1.,1.,1.,
1.,1.,1.,1.,1.,1.,1.,1.,1.,1.,1.,1.,1.,1.,1.,1.,1.,1.,1.,1.,1.,1.,1.,1.,
1.,1.,1.,1.,1.,1.))
REPRESENTATION_ITEM('')
);
#333=(
BOUNDED_CURVE()
B_SPLINE_CURVE(5,(#49391,#49392,#49393,#49394,#49395,#49396,#49397,#49398,
#49399,#49400,#49401,#49402,#49403,#49404,#49405,#49406,#49407,#49408,#49409,
#49410,#49411,#49412,#49413,#49414,#49415,#49416,#49417,#49418,#49419,#49420,
#49421,#49422,#49423,#49424,#49425,#49426,#49427,#49428,#49429,#49430,#49431,
#49432,#49433,#49434,#49435,#49436,#49437,#49438,#49439,#49440,#49441,#49442,
#49443,#49444,#49445,#49446,#49447,#49448,#49449,#49450,#49451,#49452,#49453,
#49454,#49455,#49456,#49457,#49458,#49459,#49460),.UNSPECIFIED.,.F.,.F.)
B_SPLINE_CURVE_WITH_KNOTS((6,1,1,1,1,1,1,1,1,1,1,1,1,1,1,1,1,1,1,1,1,1,
1,1,1,1,1,1,1,1,1,1,1,1,1,1,1,1,1,1,1,1,1,1,1,1,1,1,1,1,1,1,1,1,1,1,1,1,
1,1,1,1,1,1,1,6),(-1.,-0.984615384615383,-0.969230769230768,-0.953846153846152,
-0.938461538461537,-0.923076923076922,-0.907692307692306,-0.892307692307691,
-0.876923076923076,-0.86153846153846,-0.846153846153845,-0.83076923076923,
-0.815384615384614,-0.799999999999999,-0.784615384615384,-0.769230769230768,
-0.753846153846153,-0.738461538461538,-0.723076923076922,-0.707692307692307,
-0.692307692307692,-0.676923076923076,-0.661538461538461,-0.646153846153846,
-0.63076923076923,-0.615384615384615,-0.6,-0.584615384615384,-0.569230769230769,
-0.553846153846154,-0.538461538461538,-0.523076923076923,-0.507692307692308,
-0.492307692307692,-0.476923076923077,-0.461538461538462,-0.446153846153846,
-0.430769230769231,-0.415384615384615,-0.4,-0.384615384615385,-0.369230769230769,
-0.353846153846154,-0.338461538461538,-0.323076923076923,-0.307692307692308,
-0.292307692307692,-0.276923076923077,-0.261538461538462,-0.246153846153846,
-0.230769230769231,-0.215384615384615,-0.2,-0.184615384615385,-0.169230769230769,
-0.153846153846154,-0.138461538461538,-0.123076923076923,-0.107692307692308,
-0.0923076923076923,-0.0769230769230769,-0.0615384615384615,-0.0461538461538462,
-0.0307692307692308,-0.0153846153846154,-0.0057718433745107),
 .UNSPECIFIED.)
CURVE()
GEOMETRIC_REPRESENTATION_ITEM()
RATIONAL_B_SPLINE_CURVE((1.,1.,1.,1.,1.,1.,1.,1.,1.,1.,1.,1.,1.,1.,1.,1.,
1.,1.,1.,1.,1.,1.,1.,1.,1.,1.,1.,1.,1.,1.,1.,1.,1.,1.,1.,1.,1.,1.,1.,1.,
1.,1.,1.,1.,1.,1.,1.,1.,1.,1.,1.,1.,1.,1.,1.,1.,1.,1.,1.,1.,1.,1.,1.,1.,
1.,1.,1.,1.,1.,1.))
REPRESENTATION_ITEM('')
);
#334=(
BOUNDED_CURVE()
B_SPLINE_CURVE(5,(#49611,#49612,#49613,#49614,#49615,#49616,#49617,#49618,
#49619,#49620,#49621,#49622,#49623,#49624,#49625,#49626,#49627,#49628,#49629,
#49630,#49631,#49632,#49633,#49634,#49635,#49636,#49637,#49638,#49639,#49640,
#49641,#49642,#49643,#49644,#49645,#49646,#49647,#49648,#49649,#49650,#49651,
#49652,#49653,#49654,#49655,#49656,#49657,#49658,#49659,#49660,#49661,#49662,
#49663,#49664,#49665,#49666,#49667,#49668,#49669,#49670,#49671,#49672,#49673,
#49674,#49675,#49676,#49677,#49678,#49679,#49680),.UNSPECIFIED.,.F.,.F.)
B_SPLINE_CURVE_WITH_KNOTS((6,1,1,1,1,1,1,1,1,1,1,1,1,1,1,1,1,1,1,1,1,1,
1,1,1,1,1,1,1,1,1,1,1,1,1,1,1,1,1,1,1,1,1,1,1,1,1,1,1,1,1,1,1,1,1,1,1,1,
1,1,1,1,1,1,1,6),(-0.994228156739708,-0.984615384615383,-0.969230769230768,
-0.953846153846152,-0.938461538461537,-0.923076923076922,-0.907692307692306,
-0.892307692307691,-0.876923076923076,-0.86153846153846,-0.846153846153845,
-0.83076923076923,-0.815384615384614,-0.799999999999999,-0.784615384615384,
-0.769230769230768,-0.753846153846153,-0.738461538461538,-0.723076923076922,
-0.707692307692307,-0.692307692307692,-0.676923076923076,-0.661538461538461,
-0.646153846153846,-0.63076923076923,-0.615384615384615,-0.6,-0.584615384615384,
-0.569230769230769,-0.553846153846154,-0.538461538461538,-0.523076923076923,
-0.507692307692308,-0.492307692307692,-0.476923076923077,-0.461538461538462,
-0.446153846153846,-0.430769230769231,-0.415384615384615,-0.4,-0.384615384615385,
-0.369230769230769,-0.353846153846154,-0.338461538461538,-0.323076923076923,
-0.307692307692308,-0.292307692307692,-0.276923076923077,-0.261538461538462,
-0.246153846153846,-0.230769230769231,-0.215384615384615,-0.2,-0.184615384615385,
-0.169230769230769,-0.153846153846154,-0.138461538461538,-0.123076923076923,
-0.107692307692308,-0.0923076923076923,-0.0769230769230769,-0.0615384615384615,
-0.0461538461538462,-0.0307692307692308,-0.0153846153846154,0.),
 .UNSPECIFIED.)
CURVE()
GEOMETRIC_REPRESENTATION_ITEM()
RATIONAL_B_SPLINE_CURVE((1.,1.,1.,1.,1.,1.,1.,1.,1.,1.,1.,1.,1.,1.,1.,1.,
1.,1.,1.,1.,1.,1.,1.,1.,1.,1.,1.,1.,1.,1.,1.,1.,1.,1.,1.,1.,1.,1.,1.,1.,
1.,1.,1.,1.,1.,1.,1.,1.,1.,1.,1.,1.,1.,1.,1.,1.,1.,1.,1.,1.,1.,1.,1.,1.,
1.,1.,1.,1.,1.,1.))
REPRESENTATION_ITEM('')
);
#335=(
BOUNDED_CURVE()
B_SPLINE_CURVE(5,(#49833,#49834,#49835,#49836,#49837,#49838,#49839,#49840,
#49841,#49842,#49843,#49844,#49845,#49846,#49847,#49848,#49849,#49850,#49851,
#49852,#49853,#49854,#49855,#49856,#49857,#49858,#49859,#49860,#49861,#49862,
#49863,#49864,#49865,#49866,#49867,#49868,#49869,#49870,#49871,#49872,#49873,
#49874,#49875,#49876,#49877,#49878,#49879,#49880,#49881,#49882,#49883,#49884,
#49885,#49886,#49887,#49888,#49889,#49890,#49891,#49892,#49893,#49894,#49895,
#49896,#49897,#49898,#49899,#49900,#49901,#49902),.UNSPECIFIED.,.F.,.F.)
B_SPLINE_CURVE_WITH_KNOTS((6,1,1,1,1,1,1,1,1,1,1,1,1,1,1,1,1,1,1,1,1,1,
1,1,1,1,1,1,1,1,1,1,1,1,1,1,1,1,1,1,1,1,1,1,1,1,1,1,1,1,1,1,1,1,1,1,1,1,
1,1,1,1,1,1,1,6),(-1.,-0.984615384615383,-0.969230769230768,-0.953846153846152,
-0.938461538461537,-0.923076923076922,-0.907692307692306,-0.892307692307691,
-0.876923076923076,-0.86153846153846,-0.846153846153845,-0.83076923076923,
-0.815384615384614,-0.799999999999999,-0.784615384615384,-0.769230769230768,
-0.753846153846153,-0.738461538461538,-0.723076923076922,-0.707692307692307,
-0.692307692307692,-0.676923076923076,-0.661538461538461,-0.646153846153846,
-0.63076923076923,-0.615384615384615,-0.6,-0.584615384615384,-0.569230769230769,
-0.553846153846154,-0.538461538461538,-0.523076923076923,-0.507692307692308,
-0.492307692307692,-0.476923076923077,-0.461538461538462,-0.446153846153846,
-0.430769230769231,-0.415384615384615,-0.4,-0.384615384615385,-0.369230769230769,
-0.353846153846154,-0.338461538461538,-0.323076923076923,-0.307692307692308,
-0.292307692307692,-0.276923076923077,-0.261538461538462,-0.246153846153846,
-0.230769230769231,-0.215384615384615,-0.2,-0.184615384615385,-0.169230769230769,
-0.153846153846154,-0.138461538461538,-0.123076923076923,-0.107692307692308,
-0.0923076923076923,-0.0769230769230769,-0.0615384615384615,-0.0461538461538462,
-0.0307692307692308,-0.0153846153846154,-0.00577184337451708),
 .UNSPECIFIED.)
CURVE()
GEOMETRIC_REPRESENTATION_ITEM()
RATIONAL_B_SPLINE_CURVE((1.,1.,1.,1.,1.,1.,1.,1.,1.,1.,1.,1.,1.,1.,1.,1.,
1.,1.,1.,1.,1.,1.,1.,1.,1.,1.,1.,1.,1.,1.,1.,1.,1.,1.,1.,1.,1.,1.,1.,1.,
1.,1.,1.,1.,1.,1.,1.,1.,1.,1.,1.,1.,1.,1.,1.,1.,1.,1.,1.,1.,1.,1.,1.,1.,
1.,1.,1.,1.,1.,1.))
REPRESENTATION_ITEM('')
);
#336=(
BOUNDED_CURVE()
B_SPLINE_CURVE(5,(#50053,#50054,#50055,#50056,#50057,#50058,#50059,#50060,
#50061,#50062,#50063,#50064,#50065,#50066,#50067,#50068,#50069,#50070,#50071,
#50072,#50073,#50074,#50075,#50076,#50077,#50078,#50079,#50080,#50081,#50082,
#50083,#50084,#50085,#50086,#50087,#50088,#50089,#50090,#50091,#50092,#50093,
#50094,#50095,#50096,#50097,#50098,#50099,#50100,#50101,#50102,#50103,#50104,
#50105,#50106,#50107,#50108,#50109,#50110,#50111,#50112,#50113,#50114,#50115,
#50116,#50117,#50118,#50119,#50120,#50121,#50122),.UNSPECIFIED.,.F.,.F.)
B_SPLINE_CURVE_WITH_KNOTS((6,1,1,1,1,1,1,1,1,1,1,1,1,1,1,1,1,1,1,1,1,1,
1,1,1,1,1,1,1,1,1,1,1,1,1,1,1,1,1,1,1,1,1,1,1,1,1,1,1,1,1,1,1,1,1,1,1,1,
1,1,1,1,1,1,1,6),(-0.994228156739669,-0.984615384615383,-0.969230769230768,
-0.953846153846152,-0.938461538461537,-0.923076923076922,-0.907692307692306,
-0.892307692307691,-0.876923076923076,-0.86153846153846,-0.846153846153845,
-0.83076923076923,-0.815384615384614,-0.799999999999999,-0.784615384615384,
-0.769230769230768,-0.753846153846153,-0.738461538461538,-0.723076923076922,
-0.707692307692307,-0.692307692307692,-0.676923076923076,-0.661538461538461,
-0.646153846153846,-0.63076923076923,-0.615384615384615,-0.6,-0.584615384615384,
-0.569230769230769,-0.553846153846154,-0.538461538461538,-0.523076923076923,
-0.507692307692308,-0.492307692307692,-0.476923076923077,-0.461538461538462,
-0.446153846153846,-0.430769230769231,-0.415384615384615,-0.4,-0.384615384615385,
-0.369230769230769,-0.353846153846154,-0.338461538461538,-0.323076923076923,
-0.307692307692308,-0.292307692307692,-0.276923076923077,-0.261538461538462,
-0.246153846153846,-0.230769230769231,-0.215384615384615,-0.2,-0.184615384615385,
-0.169230769230769,-0.153846153846154,-0.138461538461538,-0.123076923076923,
-0.107692307692308,-0.0923076923076923,-0.0769230769230769,-0.0615384615384615,
-0.0461538461538462,-0.0307692307692308,-0.0153846153846154,0.),
 .UNSPECIFIED.)
CURVE()
GEOMETRIC_REPRESENTATION_ITEM()
RATIONAL_B_SPLINE_CURVE((1.,1.,1.,1.,1.,1.,1.,1.,1.,1.,1.,1.,1.,1.,1.,1.,
1.,1.,1.,1.,1.,1.,1.,1.,1.,1.,1.,1.,1.,1.,1.,1.,1.,1.,1.,1.,1.,1.,1.,1.,
1.,1.,1.,1.,1.,1.,1.,1.,1.,1.,1.,1.,1.,1.,1.,1.,1.,1.,1.,1.,1.,1.,1.,1.,
1.,1.,1.,1.,1.,1.))
REPRESENTATION_ITEM('')
);
#337=(
BOUNDED_CURVE()
B_SPLINE_CURVE(5,(#50275,#50276,#50277,#50278,#50279,#50280,#50281,#50282,
#50283,#50284,#50285,#50286,#50287,#50288,#50289,#50290,#50291,#50292,#50293,
#50294,#50295,#50296,#50297,#50298,#50299,#50300,#50301,#50302,#50303,#50304,
#50305,#50306,#50307,#50308,#50309,#50310,#50311,#50312,#50313,#50314,#50315,
#50316,#50317,#50318,#50319,#50320,#50321,#50322,#50323,#50324,#50325,#50326,
#50327,#50328,#50329,#50330,#50331,#50332,#50333,#50334,#50335,#50336,#50337,
#50338,#50339,#50340,#50341,#50342,#50343,#50344),.UNSPECIFIED.,.F.,.F.)
B_SPLINE_CURVE_WITH_KNOTS((6,1,1,1,1,1,1,1,1,1,1,1,1,1,1,1,1,1,1,1,1,1,
1,1,1,1,1,1,1,1,1,1,1,1,1,1,1,1,1,1,1,1,1,1,1,1,1,1,1,1,1,1,1,1,1,1,1,1,
1,1,1,1,1,1,1,6),(-1.,-0.984615384615383,-0.969230769230768,-0.953846153846152,
-0.938461538461537,-0.923076923076922,-0.907692307692306,-0.892307692307691,
-0.876923076923076,-0.86153846153846,-0.846153846153845,-0.83076923076923,
-0.815384615384614,-0.799999999999999,-0.784615384615384,-0.769230769230768,
-0.753846153846153,-0.738461538461538,-0.723076923076922,-0.707692307692307,
-0.692307692307692,-0.676923076923076,-0.661538461538461,-0.646153846153846,
-0.63076923076923,-0.615384615384615,-0.6,-0.584615384615384,-0.569230769230769,
-0.553846153846154,-0.538461538461538,-0.523076923076923,-0.507692307692308,
-0.492307692307692,-0.476923076923077,-0.461538461538462,-0.446153846153846,
-0.430769230769231,-0.415384615384615,-0.4,-0.384615384615385,-0.369230769230769,
-0.353846153846154,-0.338461538461538,-0.323076923076923,-0.307692307692308,
-0.292307692307692,-0.276923076923077,-0.261538461538462,-0.246153846153846,
-0.230769230769231,-0.215384615384615,-0.2,-0.184615384615385,-0.169230769230769,
-0.153846153846154,-0.138461538461538,-0.123076923076923,-0.107692307692308,
-0.0923076923076923,-0.0769230769230769,-0.0615384615384615,-0.0461538461538462,
-0.0307692307692308,-0.0153846153846154,-0.0057718433744903),
 .UNSPECIFIED.)
CURVE()
GEOMETRIC_REPRESENTATION_ITEM()
RATIONAL_B_SPLINE_CURVE((1.,1.,1.,1.,1.,1.,1.,1.,1.,1.,1.,1.,1.,1.,1.,1.,
1.,1.,1.,1.,1.,1.,1.,1.,1.,1.,1.,1.,1.,1.,1.,1.,1.,1.,1.,1.,1.,1.,1.,1.,
1.,1.,1.,1.,1.,1.,1.,1.,1.,1.,1.,1.,1.,1.,1.,1.,1.,1.,1.,1.,1.,1.,1.,1.,
1.,1.,1.,1.,1.,1.))
REPRESENTATION_ITEM('')
);
#338=(
BOUNDED_CURVE()
B_SPLINE_CURVE(5,(#50495,#50496,#50497,#50498,#50499,#50500,#50501,#50502,
#50503,#50504,#50505,#50506,#50507,#50508,#50509,#50510,#50511,#50512,#50513,
#50514,#50515,#50516,#50517,#50518,#50519,#50520,#50521,#50522,#50523,#50524,
#50525,#50526,#50527,#50528,#50529,#50530,#50531,#50532,#50533,#50534,#50535,
#50536,#50537,#50538,#50539,#50540,#50541,#50542,#50543,#50544,#50545,#50546,
#50547,#50548,#50549,#50550,#50551,#50552,#50553,#50554,#50555,#50556,#50557,
#50558,#50559,#50560,#50561,#50562,#50563,#50564),.UNSPECIFIED.,.F.,.F.)
B_SPLINE_CURVE_WITH_KNOTS((6,1,1,1,1,1,1,1,1,1,1,1,1,1,1,1,1,1,1,1,1,1,
1,1,1,1,1,1,1,1,1,1,1,1,1,1,1,1,1,1,1,1,1,1,1,1,1,1,1,1,1,1,1,1,1,1,1,1,
1,1,1,1,1,1,1,6),(-0.994228156739712,-0.984615384615383,-0.969230769230768,
-0.953846153846152,-0.938461538461537,-0.923076923076922,-0.907692307692306,
-0.892307692307691,-0.876923076923076,-0.86153846153846,-0.846153846153845,
-0.83076923076923,-0.815384615384614,-0.799999999999999,-0.784615384615384,
-0.769230769230768,-0.753846153846153,-0.738461538461538,-0.723076923076922,
-0.707692307692307,-0.692307692307692,-0.676923076923076,-0.661538461538461,
-0.646153846153846,-0.63076923076923,-0.615384615384615,-0.6,-0.584615384615384,
-0.569230769230769,-0.553846153846154,-0.538461538461538,-0.523076923076923,
-0.507692307692308,-0.492307692307692,-0.476923076923077,-0.461538461538462,
-0.446153846153846,-0.430769230769231,-0.415384615384615,-0.4,-0.384615384615385,
-0.369230769230769,-0.353846153846154,-0.338461538461538,-0.323076923076923,
-0.307692307692308,-0.292307692307692,-0.276923076923077,-0.261538461538462,
-0.246153846153846,-0.230769230769231,-0.215384615384615,-0.2,-0.184615384615385,
-0.169230769230769,-0.153846153846154,-0.138461538461538,-0.123076923076923,
-0.107692307692308,-0.0923076923076923,-0.0769230769230769,-0.0615384615384615,
-0.0461538461538462,-0.0307692307692308,-0.0153846153846154,0.),
 .UNSPECIFIED.)
CURVE()
GEOMETRIC_REPRESENTATION_ITEM()
RATIONAL_B_SPLINE_CURVE((1.,1.,1.,1.,1.,1.,1.,1.,1.,1.,1.,1.,1.,1.,1.,1.,
1.,1.,1.,1.,1.,1.,1.,1.,1.,1.,1.,1.,1.,1.,1.,1.,1.,1.,1.,1.,1.,1.,1.,1.,
1.,1.,1.,1.,1.,1.,1.,1.,1.,1.,1.,1.,1.,1.,1.,1.,1.,1.,1.,1.,1.,1.,1.,1.,
1.,1.,1.,1.,1.,1.))
REPRESENTATION_ITEM('')
);
#339=(
BOUNDED_CURVE()
B_SPLINE_CURVE(5,(#50717,#50718,#50719,#50720,#50721,#50722,#50723,#50724,
#50725,#50726,#50727,#50728,#50729,#50730,#50731,#50732,#50733,#50734,#50735,
#50736,#50737,#50738,#50739,#50740,#50741,#50742,#50743,#50744,#50745,#50746,
#50747,#50748,#50749,#50750,#50751,#50752,#50753,#50754,#50755,#50756,#50757,
#50758,#50759,#50760,#50761,#50762,#50763,#50764,#50765,#50766,#50767,#50768,
#50769,#50770,#50771,#50772,#50773,#50774,#50775,#50776,#50777,#50778,#50779,
#50780,#50781,#50782,#50783,#50784,#50785,#50786),.UNSPECIFIED.,.F.,.F.)
B_SPLINE_CURVE_WITH_KNOTS((6,1,1,1,1,1,1,1,1,1,1,1,1,1,1,1,1,1,1,1,1,1,
1,1,1,1,1,1,1,1,1,1,1,1,1,1,1,1,1,1,1,1,1,1,1,1,1,1,1,1,1,1,1,1,1,1,1,1,
1,1,1,1,1,1,1,6),(-1.,-0.984615384615383,-0.969230769230768,-0.953846153846152,
-0.938461538461537,-0.923076923076922,-0.907692307692306,-0.892307692307691,
-0.876923076923076,-0.86153846153846,-0.846153846153845,-0.83076923076923,
-0.815384615384614,-0.799999999999999,-0.784615384615384,-0.769230769230768,
-0.753846153846153,-0.738461538461538,-0.723076923076922,-0.707692307692307,
-0.692307692307692,-0.676923076923076,-0.661538461538461,-0.646153846153846,
-0.63076923076923,-0.615384615384615,-0.6,-0.584615384615384,-0.569230769230769,
-0.553846153846154,-0.538461538461538,-0.523076923076923,-0.507692307692308,
-0.492307692307692,-0.476923076923077,-0.461538461538462,-0.446153846153846,
-0.430769230769231,-0.415384615384615,-0.4,-0.384615384615385,-0.369230769230769,
-0.353846153846154,-0.338461538461538,-0.323076923076923,-0.307692307692308,
-0.292307692307692,-0.276923076923077,-0.261538461538462,-0.246153846153846,
-0.230769230769231,-0.215384615384615,-0.2,-0.184615384615385,-0.169230769230769,
-0.153846153846154,-0.138461538461538,-0.123076923076923,-0.107692307692308,
-0.0923076923076923,-0.0769230769230769,-0.0615384615384615,-0.0461538461538462,
-0.0307692307692308,-0.0153846153846154,-0.0057718433745291),
 .UNSPECIFIED.)
CURVE()
GEOMETRIC_REPRESENTATION_ITEM()
RATIONAL_B_SPLINE_CURVE((1.,1.,1.,1.,1.,1.,1.,1.,1.,1.,1.,1.,1.,1.,1.,1.,
1.,1.,1.,1.,1.,1.,1.,1.,1.,1.,1.,1.,1.,1.,1.,1.,1.,1.,1.,1.,1.,1.,1.,1.,
1.,1.,1.,1.,1.,1.,1.,1.,1.,1.,1.,1.,1.,1.,1.,1.,1.,1.,1.,1.,1.,1.,1.,1.,
1.,1.,1.,1.,1.,1.))
REPRESENTATION_ITEM('')
);
#340=(
BOUNDED_CURVE()
B_SPLINE_CURVE(5,(#50937,#50938,#50939,#50940,#50941,#50942,#50943,#50944,
#50945,#50946,#50947,#50948,#50949,#50950,#50951,#50952,#50953,#50954,#50955,
#50956,#50957,#50958,#50959,#50960,#50961,#50962,#50963,#50964,#50965,#50966,
#50967,#50968,#50969,#50970,#50971,#50972,#50973,#50974,#50975,#50976,#50977,
#50978,#50979,#50980,#50981,#50982,#50983,#50984,#50985,#50986,#50987,#50988,
#50989,#50990,#50991,#50992,#50993,#50994,#50995,#50996,#50997,#50998,#50999,
#51000,#51001,#51002,#51003,#51004,#51005,#51006),.UNSPECIFIED.,.F.,.F.)
B_SPLINE_CURVE_WITH_KNOTS((6,1,1,1,1,1,1,1,1,1,1,1,1,1,1,1,1,1,1,1,1,1,
1,1,1,1,1,1,1,1,1,1,1,1,1,1,1,1,1,1,1,1,1,1,1,1,1,1,1,1,1,1,1,1,1,1,1,1,
1,1,1,1,1,1,1,6),(-0.994228156739695,-0.984615384615383,-0.969230769230768,
-0.953846153846152,-0.938461538461537,-0.923076923076922,-0.907692307692306,
-0.892307692307691,-0.876923076923076,-0.86153846153846,-0.846153846153845,
-0.83076923076923,-0.815384615384614,-0.799999999999999,-0.784615384615384,
-0.769230769230768,-0.753846153846153,-0.738461538461538,-0.723076923076922,
-0.707692307692307,-0.692307692307692,-0.676923076923076,-0.661538461538461,
-0.646153846153846,-0.63076923076923,-0.615384615384615,-0.6,-0.584615384615384,
-0.569230769230769,-0.553846153846154,-0.538461538461538,-0.523076923076923,
-0.507692307692308,-0.492307692307692,-0.476923076923077,-0.461538461538462,
-0.446153846153846,-0.430769230769231,-0.415384615384615,-0.4,-0.384615384615385,
-0.369230769230769,-0.353846153846154,-0.338461538461538,-0.323076923076923,
-0.307692307692308,-0.292307692307692,-0.276923076923077,-0.261538461538462,
-0.246153846153846,-0.230769230769231,-0.215384615384615,-0.2,-0.184615384615385,
-0.169230769230769,-0.153846153846154,-0.138461538461538,-0.123076923076923,
-0.107692307692308,-0.0923076923076923,-0.0769230769230769,-0.0615384615384615,
-0.0461538461538462,-0.0307692307692308,-0.0153846153846154,0.),
 .UNSPECIFIED.)
CURVE()
GEOMETRIC_REPRESENTATION_ITEM()
RATIONAL_B_SPLINE_CURVE((1.,1.,1.,1.,1.,1.,1.,1.,1.,1.,1.,1.,1.,1.,1.,1.,
1.,1.,1.,1.,1.,1.,1.,1.,1.,1.,1.,1.,1.,1.,1.,1.,1.,1.,1.,1.,1.,1.,1.,1.,
1.,1.,1.,1.,1.,1.,1.,1.,1.,1.,1.,1.,1.,1.,1.,1.,1.,1.,1.,1.,1.,1.,1.,1.,
1.,1.,1.,1.,1.,1.))
REPRESENTATION_ITEM('')
);
#341=(
BOUNDED_CURVE()
B_SPLINE_CURVE(5,(#51159,#51160,#51161,#51162,#51163,#51164,#51165,#51166,
#51167,#51168,#51169,#51170,#51171,#51172,#51173,#51174,#51175,#51176,#51177,
#51178,#51179,#51180,#51181,#51182,#51183,#51184,#51185,#51186,#51187,#51188,
#51189,#51190,#51191,#51192,#51193,#51194,#51195,#51196,#51197,#51198,#51199,
#51200,#51201,#51202,#51203,#51204,#51205,#51206,#51207,#51208,#51209,#51210,
#51211,#51212,#51213,#51214,#51215,#51216,#51217,#51218,#51219,#51220,#51221,
#51222,#51223,#51224,#51225,#51226,#51227,#51228),.UNSPECIFIED.,.F.,.F.)
B_SPLINE_CURVE_WITH_KNOTS((6,1,1,1,1,1,1,1,1,1,1,1,1,1,1,1,1,1,1,1,1,1,
1,1,1,1,1,1,1,1,1,1,1,1,1,1,1,1,1,1,1,1,1,1,1,1,1,1,1,1,1,1,1,1,1,1,1,1,
1,1,1,1,1,1,1,6),(-1.,-0.984615384615383,-0.969230769230768,-0.953846153846152,
-0.938461538461537,-0.923076923076922,-0.907692307692306,-0.892307692307691,
-0.876923076923076,-0.86153846153846,-0.846153846153845,-0.83076923076923,
-0.815384615384614,-0.799999999999999,-0.784615384615384,-0.769230769230768,
-0.753846153846153,-0.738461538461538,-0.723076923076922,-0.707692307692307,
-0.692307692307692,-0.676923076923076,-0.661538461538461,-0.646153846153846,
-0.63076923076923,-0.615384615384615,-0.6,-0.584615384615384,-0.569230769230769,
-0.553846153846154,-0.538461538461538,-0.523076923076923,-0.507692307692308,
-0.492307692307692,-0.476923076923077,-0.461538461538462,-0.446153846153846,
-0.430769230769231,-0.415384615384615,-0.4,-0.384615384615385,-0.369230769230769,
-0.353846153846154,-0.338461538461538,-0.323076923076923,-0.307692307692308,
-0.292307692307692,-0.276923076923077,-0.261538461538462,-0.246153846153846,
-0.230769230769231,-0.215384615384615,-0.2,-0.184615384615385,-0.169230769230769,
-0.153846153846154,-0.138461538461538,-0.123076923076923,-0.107692307692308,
-0.0923076923076923,-0.0769230769230769,-0.0615384615384615,-0.0461538461538462,
-0.0307692307692308,-0.0153846153846154,-0.00577184337450344),
 .UNSPECIFIED.)
CURVE()
GEOMETRIC_REPRESENTATION_ITEM()
RATIONAL_B_SPLINE_CURVE((1.,1.,1.,1.,1.,1.,1.,1.,1.,1.,1.,1.,1.,1.,1.,1.,
1.,1.,1.,1.,1.,1.,1.,1.,1.,1.,1.,1.,1.,1.,1.,1.,1.,1.,1.,1.,1.,1.,1.,1.,
1.,1.,1.,1.,1.,1.,1.,1.,1.,1.,1.,1.,1.,1.,1.,1.,1.,1.,1.,1.,1.,1.,1.,1.,
1.,1.,1.,1.,1.,1.))
REPRESENTATION_ITEM('')
);
#342=(
BOUNDED_CURVE()
B_SPLINE_CURVE(5,(#51379,#51380,#51381,#51382,#51383,#51384,#51385,#51386,
#51387,#51388,#51389,#51390,#51391,#51392,#51393,#51394,#51395,#51396,#51397,
#51398,#51399,#51400,#51401,#51402,#51403,#51404,#51405,#51406,#51407,#51408,
#51409,#51410,#51411,#51412,#51413,#51414,#51415,#51416,#51417,#51418,#51419,
#51420,#51421,#51422,#51423,#51424,#51425,#51426,#51427,#51428,#51429,#51430,
#51431,#51432,#51433,#51434,#51435,#51436,#51437,#51438,#51439,#51440,#51441,
#51442,#51443,#51444,#51445,#51446,#51447,#51448),.UNSPECIFIED.,.F.,.F.)
B_SPLINE_CURVE_WITH_KNOTS((6,1,1,1,1,1,1,1,1,1,1,1,1,1,1,1,1,1,1,1,1,1,
1,1,1,1,1,1,1,1,1,1,1,1,1,1,1,1,1,1,1,1,1,1,1,1,1,1,1,1,1,1,1,1,1,1,1,1,
1,1,1,1,1,1,1,6),(-0.994228156739669,-0.984615384615383,-0.969230769230768,
-0.953846153846152,-0.938461538461537,-0.923076923076922,-0.907692307692306,
-0.892307692307691,-0.876923076923076,-0.86153846153846,-0.846153846153845,
-0.83076923076923,-0.815384615384614,-0.799999999999999,-0.784615384615384,
-0.769230769230768,-0.753846153846153,-0.738461538461538,-0.723076923076922,
-0.707692307692307,-0.692307692307692,-0.676923076923076,-0.661538461538461,
-0.646153846153846,-0.63076923076923,-0.615384615384615,-0.6,-0.584615384615384,
-0.569230769230769,-0.553846153846154,-0.538461538461538,-0.523076923076923,
-0.507692307692308,-0.492307692307692,-0.476923076923077,-0.461538461538462,
-0.446153846153846,-0.430769230769231,-0.415384615384615,-0.4,-0.384615384615385,
-0.369230769230769,-0.353846153846154,-0.338461538461538,-0.323076923076923,
-0.307692307692308,-0.292307692307692,-0.276923076923077,-0.261538461538462,
-0.246153846153846,-0.230769230769231,-0.215384615384615,-0.2,-0.184615384615385,
-0.169230769230769,-0.153846153846154,-0.138461538461538,-0.123076923076923,
-0.107692307692308,-0.0923076923076923,-0.0769230769230769,-0.0615384615384615,
-0.0461538461538462,-0.0307692307692308,-0.0153846153846154,0.),
 .UNSPECIFIED.)
CURVE()
GEOMETRIC_REPRESENTATION_ITEM()
RATIONAL_B_SPLINE_CURVE((1.,1.,1.,1.,1.,1.,1.,1.,1.,1.,1.,1.,1.,1.,1.,1.,
1.,1.,1.,1.,1.,1.,1.,1.,1.,1.,1.,1.,1.,1.,1.,1.,1.,1.,1.,1.,1.,1.,1.,1.,
1.,1.,1.,1.,1.,1.,1.,1.,1.,1.,1.,1.,1.,1.,1.,1.,1.,1.,1.,1.,1.,1.,1.,1.,
1.,1.,1.,1.,1.,1.))
REPRESENTATION_ITEM('')
);
#343=(
BOUNDED_CURVE()
B_SPLINE_CURVE(5,(#51601,#51602,#51603,#51604,#51605,#51606,#51607,#51608,
#51609,#51610,#51611,#51612,#51613,#51614,#51615,#51616,#51617,#51618,#51619,
#51620,#51621,#51622,#51623,#51624,#51625,#51626,#51627,#51628,#51629,#51630,
#51631,#51632,#51633,#51634,#51635,#51636,#51637,#51638,#51639,#51640,#51641,
#51642,#51643,#51644,#51645,#51646,#51647,#51648,#51649,#51650,#51651,#51652,
#51653,#51654,#51655,#51656,#51657,#51658,#51659,#51660,#51661,#51662,#51663,
#51664,#51665,#51666,#51667,#51668,#51669,#51670),.UNSPECIFIED.,.F.,.F.)
B_SPLINE_CURVE_WITH_KNOTS((6,1,1,1,1,1,1,1,1,1,1,1,1,1,1,1,1,1,1,1,1,1,
1,1,1,1,1,1,1,1,1,1,1,1,1,1,1,1,1,1,1,1,1,1,1,1,1,1,1,1,1,1,1,1,1,1,1,1,
1,1,1,1,1,1,1,6),(-1.,-0.984615384615383,-0.969230769230768,-0.953846153846152,
-0.938461538461537,-0.923076923076922,-0.907692307692306,-0.892307692307691,
-0.876923076923076,-0.86153846153846,-0.846153846153845,-0.83076923076923,
-0.815384615384614,-0.799999999999999,-0.784615384615384,-0.769230769230768,
-0.753846153846153,-0.738461538461538,-0.723076923076922,-0.707692307692307,
-0.692307692307692,-0.676923076923076,-0.661538461538461,-0.646153846153846,
-0.63076923076923,-0.615384615384615,-0.6,-0.584615384615384,-0.569230769230769,
-0.553846153846154,-0.538461538461538,-0.523076923076923,-0.507692307692308,
-0.492307692307692,-0.476923076923077,-0.461538461538462,-0.446153846153846,
-0.430769230769231,-0.415384615384615,-0.4,-0.384615384615385,-0.369230769230769,
-0.353846153846154,-0.338461538461538,-0.323076923076923,-0.307692307692308,
-0.292307692307692,-0.276923076923077,-0.261538461538462,-0.246153846153846,
-0.230769230769231,-0.215384615384615,-0.2,-0.184615384615385,-0.169230769230769,
-0.153846153846154,-0.138461538461538,-0.123076923076923,-0.107692307692308,
-0.0923076923076923,-0.0769230769230769,-0.0615384615384615,-0.0461538461538462,
-0.0307692307692308,-0.0153846153846154,-0.00577184337450876),
 .UNSPECIFIED.)
CURVE()
GEOMETRIC_REPRESENTATION_ITEM()
RATIONAL_B_SPLINE_CURVE((1.,1.,1.,1.,1.,1.,1.,1.,1.,1.,1.,1.,1.,1.,1.,1.,
1.,1.,1.,1.,1.,1.,1.,1.,1.,1.,1.,1.,1.,1.,1.,1.,1.,1.,1.,1.,1.,1.,1.,1.,
1.,1.,1.,1.,1.,1.,1.,1.,1.,1.,1.,1.,1.,1.,1.,1.,1.,1.,1.,1.,1.,1.,1.,1.,
1.,1.,1.,1.,1.,1.))
REPRESENTATION_ITEM('')
);
#344=(
BOUNDED_CURVE()
B_SPLINE_CURVE(5,(#51821,#51822,#51823,#51824,#51825,#51826,#51827,#51828,
#51829,#51830,#51831,#51832,#51833,#51834,#51835,#51836,#51837,#51838,#51839,
#51840,#51841,#51842,#51843,#51844,#51845,#51846,#51847,#51848,#51849,#51850,
#51851,#51852,#51853,#51854,#51855,#51856,#51857,#51858,#51859,#51860,#51861,
#51862,#51863,#51864,#51865,#51866,#51867,#51868,#51869,#51870,#51871,#51872,
#51873,#51874,#51875,#51876,#51877,#51878,#51879,#51880,#51881,#51882,#51883,
#51884,#51885,#51886,#51887,#51888,#51889,#51890),.UNSPECIFIED.,.F.,.F.)
B_SPLINE_CURVE_WITH_KNOTS((6,1,1,1,1,1,1,1,1,1,1,1,1,1,1,1,1,1,1,1,1,1,
1,1,1,1,1,1,1,1,1,1,1,1,1,1,1,1,1,1,1,1,1,1,1,1,1,1,1,1,1,1,1,1,1,1,1,1,
1,1,1,1,1,1,1,6),(-0.99422815673966,-0.984615384615383,-0.969230769230768,
-0.953846153846152,-0.938461538461537,-0.923076923076922,-0.907692307692306,
-0.892307692307691,-0.876923076923076,-0.86153846153846,-0.846153846153845,
-0.83076923076923,-0.815384615384614,-0.799999999999999,-0.784615384615384,
-0.769230769230768,-0.753846153846153,-0.738461538461538,-0.723076923076922,
-0.707692307692307,-0.692307692307692,-0.676923076923076,-0.661538461538461,
-0.646153846153846,-0.63076923076923,-0.615384615384615,-0.6,-0.584615384615384,
-0.569230769230769,-0.553846153846154,-0.538461538461538,-0.523076923076923,
-0.507692307692308,-0.492307692307692,-0.476923076923077,-0.461538461538462,
-0.446153846153846,-0.430769230769231,-0.415384615384615,-0.4,-0.384615384615385,
-0.369230769230769,-0.353846153846154,-0.338461538461538,-0.323076923076923,
-0.307692307692308,-0.292307692307692,-0.276923076923077,-0.261538461538462,
-0.246153846153846,-0.230769230769231,-0.215384615384615,-0.2,-0.184615384615385,
-0.169230769230769,-0.153846153846154,-0.138461538461538,-0.123076923076923,
-0.107692307692308,-0.0923076923076923,-0.0769230769230769,-0.0615384615384615,
-0.0461538461538462,-0.0307692307692308,-0.0153846153846154,0.),
 .UNSPECIFIED.)
CURVE()
GEOMETRIC_REPRESENTATION_ITEM()
RATIONAL_B_SPLINE_CURVE((1.,1.,1.,1.,1.,1.,1.,1.,1.,1.,1.,1.,1.,1.,1.,1.,
1.,1.,1.,1.,1.,1.,1.,1.,1.,1.,1.,1.,1.,1.,1.,1.,1.,1.,1.,1.,1.,1.,1.,1.,
1.,1.,1.,1.,1.,1.,1.,1.,1.,1.,1.,1.,1.,1.,1.,1.,1.,1.,1.,1.,1.,1.,1.,1.,
1.,1.,1.,1.,1.,1.))
REPRESENTATION_ITEM('')
);
#345=(
BOUNDED_CURVE()
B_SPLINE_CURVE(5,(#52043,#52044,#52045,#52046,#52047,#52048,#52049,#52050,
#52051,#52052,#52053,#52054,#52055,#52056,#52057,#52058,#52059,#52060,#52061,
#52062,#52063,#52064,#52065,#52066,#52067,#52068,#52069,#52070,#52071,#52072,
#52073,#52074,#52075,#52076,#52077,#52078,#52079,#52080,#52081,#52082,#52083,
#52084,#52085,#52086,#52087,#52088,#52089,#52090,#52091,#52092,#52093,#52094,
#52095,#52096,#52097,#52098,#52099,#52100,#52101,#52102,#52103,#52104,#52105,
#52106,#52107,#52108,#52109,#52110,#52111,#52112),.UNSPECIFIED.,.F.,.F.)
B_SPLINE_CURVE_WITH_KNOTS((6,1,1,1,1,1,1,1,1,1,1,1,1,1,1,1,1,1,1,1,1,1,
1,1,1,1,1,1,1,1,1,1,1,1,1,1,1,1,1,1,1,1,1,1,1,1,1,1,1,1,1,1,1,1,1,1,1,1,
1,1,1,1,1,1,1,6),(-1.,-0.984615384615383,-0.969230769230768,-0.953846153846152,
-0.938461538461537,-0.923076923076922,-0.907692307692306,-0.892307692307691,
-0.876923076923076,-0.86153846153846,-0.846153846153845,-0.83076923076923,
-0.815384615384614,-0.799999999999999,-0.784615384615384,-0.769230769230768,
-0.753846153846153,-0.738461538461538,-0.723076923076922,-0.707692307692307,
-0.692307692307692,-0.676923076923076,-0.661538461538461,-0.646153846153846,
-0.63076923076923,-0.615384615384615,-0.6,-0.584615384615384,-0.569230769230769,
-0.553846153846154,-0.538461538461538,-0.523076923076923,-0.507692307692308,
-0.492307692307692,-0.476923076923077,-0.461538461538462,-0.446153846153846,
-0.430769230769231,-0.415384615384615,-0.4,-0.384615384615385,-0.369230769230769,
-0.353846153846154,-0.338461538461538,-0.323076923076923,-0.307692307692308,
-0.292307692307692,-0.276923076923077,-0.261538461538462,-0.246153846153846,
-0.230769230769231,-0.215384615384615,-0.2,-0.184615384615385,-0.169230769230769,
-0.153846153846154,-0.138461538461538,-0.123076923076923,-0.107692307692308,
-0.0923076923076923,-0.0769230769230769,-0.0615384615384615,-0.0461538461538462,
-0.0307692307692308,-0.0153846153846154,-0.00577184337451051),
 .UNSPECIFIED.)
CURVE()
GEOMETRIC_REPRESENTATION_ITEM()
RATIONAL_B_SPLINE_CURVE((1.,1.,1.,1.,1.,1.,1.,1.,1.,1.,1.,1.,1.,1.,1.,1.,
1.,1.,1.,1.,1.,1.,1.,1.,1.,1.,1.,1.,1.,1.,1.,1.,1.,1.,1.,1.,1.,1.,1.,1.,
1.,1.,1.,1.,1.,1.,1.,1.,1.,1.,1.,1.,1.,1.,1.,1.,1.,1.,1.,1.,1.,1.,1.,1.,
1.,1.,1.,1.,1.,1.))
REPRESENTATION_ITEM('')
);
#346=(
BOUNDED_CURVE()
B_SPLINE_CURVE(5,(#52263,#52264,#52265,#52266,#52267,#52268,#52269,#52270,
#52271,#52272,#52273,#52274,#52275,#52276,#52277,#52278,#52279,#52280,#52281,
#52282,#52283,#52284,#52285,#52286,#52287,#52288,#52289,#52290,#52291,#52292,
#52293,#52294,#52295,#52296,#52297,#52298,#52299,#52300,#52301,#52302,#52303,
#52304,#52305,#52306,#52307,#52308,#52309,#52310,#52311,#52312,#52313,#52314,
#52315,#52316,#52317,#52318,#52319,#52320,#52321,#52322,#52323,#52324,#52325,
#52326,#52327,#52328,#52329,#52330,#52331,#52332),.UNSPECIFIED.,.F.,.F.)
B_SPLINE_CURVE_WITH_KNOTS((6,1,1,1,1,1,1,1,1,1,1,1,1,1,1,1,1,1,1,1,1,1,
1,1,1,1,1,1,1,1,1,1,1,1,1,1,1,1,1,1,1,1,1,1,1,1,1,1,1,1,1,1,1,1,1,1,1,1,
1,1,1,1,1,1,1,6),(-0.994228156739678,-0.984615384615383,-0.969230769230768,
-0.953846153846152,-0.938461538461537,-0.923076923076922,-0.907692307692306,
-0.892307692307691,-0.876923076923076,-0.86153846153846,-0.846153846153845,
-0.83076923076923,-0.815384615384614,-0.799999999999999,-0.784615384615384,
-0.769230769230768,-0.753846153846153,-0.738461538461538,-0.723076923076922,
-0.707692307692307,-0.692307692307692,-0.676923076923076,-0.661538461538461,
-0.646153846153846,-0.63076923076923,-0.615384615384615,-0.6,-0.584615384615384,
-0.569230769230769,-0.553846153846154,-0.538461538461538,-0.523076923076923,
-0.507692307692308,-0.492307692307692,-0.476923076923077,-0.461538461538462,
-0.446153846153846,-0.430769230769231,-0.415384615384615,-0.4,-0.384615384615385,
-0.369230769230769,-0.353846153846154,-0.338461538461538,-0.323076923076923,
-0.307692307692308,-0.292307692307692,-0.276923076923077,-0.261538461538462,
-0.246153846153846,-0.230769230769231,-0.215384615384615,-0.2,-0.184615384615385,
-0.169230769230769,-0.153846153846154,-0.138461538461538,-0.123076923076923,
-0.107692307692308,-0.0923076923076923,-0.0769230769230769,-0.0615384615384615,
-0.0461538461538462,-0.0307692307692308,-0.0153846153846154,0.),
 .UNSPECIFIED.)
CURVE()
GEOMETRIC_REPRESENTATION_ITEM()
RATIONAL_B_SPLINE_CURVE((1.,1.,1.,1.,1.,1.,1.,1.,1.,1.,1.,1.,1.,1.,1.,1.,
1.,1.,1.,1.,1.,1.,1.,1.,1.,1.,1.,1.,1.,1.,1.,1.,1.,1.,1.,1.,1.,1.,1.,1.,
1.,1.,1.,1.,1.,1.,1.,1.,1.,1.,1.,1.,1.,1.,1.,1.,1.,1.,1.,1.,1.,1.,1.,1.,
1.,1.,1.,1.,1.,1.))
REPRESENTATION_ITEM('')
);
#347=(
BOUNDED_CURVE()
B_SPLINE_CURVE(5,(#52485,#52486,#52487,#52488,#52489,#52490,#52491,#52492,
#52493,#52494,#52495,#52496,#52497,#52498,#52499,#52500,#52501,#52502,#52503,
#52504,#52505,#52506,#52507,#52508,#52509,#52510,#52511,#52512,#52513,#52514,
#52515,#52516,#52517,#52518,#52519,#52520,#52521,#52522,#52523,#52524,#52525,
#52526,#52527,#52528,#52529,#52530,#52531,#52532,#52533,#52534,#52535,#52536,
#52537,#52538,#52539,#52540,#52541,#52542,#52543,#52544,#52545,#52546,#52547,
#52548,#52549,#52550,#52551,#52552,#52553,#52554),.UNSPECIFIED.,.F.,.F.)
B_SPLINE_CURVE_WITH_KNOTS((6,1,1,1,1,1,1,1,1,1,1,1,1,1,1,1,1,1,1,1,1,1,
1,1,1,1,1,1,1,1,1,1,1,1,1,1,1,1,1,1,1,1,1,1,1,1,1,1,1,1,1,1,1,1,1,1,1,1,
1,1,1,1,1,1,1,6),(-1.,-0.984615384615383,-0.969230769230768,-0.953846153846152,
-0.938461538461537,-0.923076923076922,-0.907692307692306,-0.892307692307691,
-0.876923076923076,-0.86153846153846,-0.846153846153845,-0.83076923076923,
-0.815384615384614,-0.799999999999999,-0.784615384615384,-0.769230769230768,
-0.753846153846153,-0.738461538461538,-0.723076923076922,-0.707692307692307,
-0.692307692307692,-0.676923076923076,-0.661538461538461,-0.646153846153846,
-0.63076923076923,-0.615384615384615,-0.6,-0.584615384615384,-0.569230769230769,
-0.553846153846154,-0.538461538461538,-0.523076923076923,-0.507692307692308,
-0.492307692307692,-0.476923076923077,-0.461538461538462,-0.446153846153846,
-0.430769230769231,-0.415384615384615,-0.4,-0.384615384615385,-0.369230769230769,
-0.353846153846154,-0.338461538461538,-0.323076923076923,-0.307692307692308,
-0.292307692307692,-0.276923076923077,-0.261538461538462,-0.246153846153846,
-0.230769230769231,-0.215384615384615,-0.2,-0.184615384615385,-0.169230769230769,
-0.153846153846154,-0.138461538461538,-0.123076923076923,-0.107692307692308,
-0.0923076923076923,-0.0769230769230769,-0.0615384615384615,-0.0461538461538462,
-0.0307692307692308,-0.0153846153846154,-0.0057718433745179),
 .UNSPECIFIED.)
CURVE()
GEOMETRIC_REPRESENTATION_ITEM()
RATIONAL_B_SPLINE_CURVE((1.,1.,1.,1.,1.,1.,1.,1.,1.,1.,1.,1.,1.,1.,1.,1.,
1.,1.,1.,1.,1.,1.,1.,1.,1.,1.,1.,1.,1.,1.,1.,1.,1.,1.,1.,1.,1.,1.,1.,1.,
1.,1.,1.,1.,1.,1.,1.,1.,1.,1.,1.,1.,1.,1.,1.,1.,1.,1.,1.,1.,1.,1.,1.,1.,
1.,1.,1.,1.,1.,1.))
REPRESENTATION_ITEM('')
);
#348=(
BOUNDED_CURVE()
B_SPLINE_CURVE(5,(#52705,#52706,#52707,#52708,#52709,#52710,#52711,#52712,
#52713,#52714,#52715,#52716,#52717,#52718,#52719,#52720,#52721,#52722,#52723,
#52724,#52725,#52726,#52727,#52728,#52729,#52730,#52731,#52732,#52733,#52734,
#52735,#52736,#52737,#52738,#52739,#52740,#52741,#52742,#52743,#52744,#52745,
#52746,#52747,#52748,#52749,#52750,#52751,#52752,#52753,#52754,#52755,#52756,
#52757,#52758,#52759,#52760,#52761,#52762,#52763,#52764,#52765,#52766,#52767,
#52768,#52769,#52770,#52771,#52772,#52773,#52774),.UNSPECIFIED.,.F.,.F.)
B_SPLINE_CURVE_WITH_KNOTS((6,1,1,1,1,1,1,1,1,1,1,1,1,1,1,1,1,1,1,1,1,1,
1,1,1,1,1,1,1,1,1,1,1,1,1,1,1,1,1,1,1,1,1,1,1,1,1,1,1,1,1,1,1,1,1,1,1,1,
1,1,1,1,1,1,1,6),(-0.99422815673967,-0.984615384615383,-0.969230769230768,
-0.953846153846152,-0.938461538461537,-0.923076923076922,-0.907692307692306,
-0.892307692307691,-0.876923076923076,-0.86153846153846,-0.846153846153845,
-0.83076923076923,-0.815384615384614,-0.799999999999999,-0.784615384615384,
-0.769230769230768,-0.753846153846153,-0.738461538461538,-0.723076923076922,
-0.707692307692307,-0.692307692307692,-0.676923076923076,-0.661538461538461,
-0.646153846153846,-0.63076923076923,-0.615384615384615,-0.6,-0.584615384615384,
-0.569230769230769,-0.553846153846154,-0.538461538461538,-0.523076923076923,
-0.507692307692308,-0.492307692307692,-0.476923076923077,-0.461538461538462,
-0.446153846153846,-0.430769230769231,-0.415384615384615,-0.4,-0.384615384615385,
-0.369230769230769,-0.353846153846154,-0.338461538461538,-0.323076923076923,
-0.307692307692308,-0.292307692307692,-0.276923076923077,-0.261538461538462,
-0.246153846153846,-0.230769230769231,-0.215384615384615,-0.2,-0.184615384615385,
-0.169230769230769,-0.153846153846154,-0.138461538461538,-0.123076923076923,
-0.107692307692308,-0.0923076923076923,-0.0769230769230769,-0.0615384615384615,
-0.0461538461538462,-0.0307692307692308,-0.0153846153846154,0.),
 .UNSPECIFIED.)
CURVE()
GEOMETRIC_REPRESENTATION_ITEM()
RATIONAL_B_SPLINE_CURVE((1.,1.,1.,1.,1.,1.,1.,1.,1.,1.,1.,1.,1.,1.,1.,1.,
1.,1.,1.,1.,1.,1.,1.,1.,1.,1.,1.,1.,1.,1.,1.,1.,1.,1.,1.,1.,1.,1.,1.,1.,
1.,1.,1.,1.,1.,1.,1.,1.,1.,1.,1.,1.,1.,1.,1.,1.,1.,1.,1.,1.,1.,1.,1.,1.,
1.,1.,1.,1.,1.,1.))
REPRESENTATION_ITEM('')
);
#349=(
BOUNDED_CURVE()
B_SPLINE_CURVE(5,(#52927,#52928,#52929,#52930,#52931,#52932,#52933,#52934,
#52935,#52936,#52937,#52938,#52939,#52940,#52941,#52942,#52943,#52944,#52945,
#52946,#52947,#52948,#52949,#52950,#52951,#52952,#52953,#52954,#52955,#52956,
#52957,#52958,#52959,#52960,#52961,#52962,#52963,#52964,#52965,#52966,#52967,
#52968,#52969,#52970,#52971,#52972,#52973,#52974,#52975,#52976,#52977,#52978,
#52979,#52980,#52981,#52982,#52983,#52984,#52985,#52986,#52987,#52988,#52989,
#52990,#52991,#52992,#52993,#52994,#52995,#52996),.UNSPECIFIED.,.F.,.F.)
B_SPLINE_CURVE_WITH_KNOTS((6,1,1,1,1,1,1,1,1,1,1,1,1,1,1,1,1,1,1,1,1,1,
1,1,1,1,1,1,1,1,1,1,1,1,1,1,1,1,1,1,1,1,1,1,1,1,1,1,1,1,1,1,1,1,1,1,1,1,
1,1,1,1,1,1,1,6),(-1.,-0.984615384615383,-0.969230769230768,-0.953846153846152,
-0.938461538461537,-0.923076923076922,-0.907692307692306,-0.892307692307691,
-0.876923076923076,-0.86153846153846,-0.846153846153845,-0.83076923076923,
-0.815384615384614,-0.799999999999999,-0.784615384615384,-0.769230769230768,
-0.753846153846153,-0.738461538461538,-0.723076923076922,-0.707692307692307,
-0.692307692307692,-0.676923076923076,-0.661538461538461,-0.646153846153846,
-0.63076923076923,-0.615384615384615,-0.6,-0.584615384615384,-0.569230769230769,
-0.553846153846154,-0.538461538461538,-0.523076923076923,-0.507692307692308,
-0.492307692307692,-0.476923076923077,-0.461538461538462,-0.446153846153846,
-0.430769230769231,-0.415384615384615,-0.4,-0.384615384615385,-0.369230769230769,
-0.353846153846154,-0.338461538461538,-0.323076923076923,-0.307692307692308,
-0.292307692307692,-0.276923076923077,-0.261538461538462,-0.246153846153846,
-0.230769230769231,-0.215384615384615,-0.2,-0.184615384615385,-0.169230769230769,
-0.153846153846154,-0.138461538461538,-0.123076923076923,-0.107692307692308,
-0.0923076923076923,-0.0769230769230769,-0.0615384615384615,-0.0461538461538462,
-0.0307692307692308,-0.0153846153846154,-0.00577184337452479),
 .UNSPECIFIED.)
CURVE()
GEOMETRIC_REPRESENTATION_ITEM()
RATIONAL_B_SPLINE_CURVE((1.,1.,1.,1.,1.,1.,1.,1.,1.,1.,1.,1.,1.,1.,1.,1.,
1.,1.,1.,1.,1.,1.,1.,1.,1.,1.,1.,1.,1.,1.,1.,1.,1.,1.,1.,1.,1.,1.,1.,1.,
1.,1.,1.,1.,1.,1.,1.,1.,1.,1.,1.,1.,1.,1.,1.,1.,1.,1.,1.,1.,1.,1.,1.,1.,
1.,1.,1.,1.,1.,1.))
REPRESENTATION_ITEM('')
);
#350=(
BOUNDED_CURVE()
B_SPLINE_CURVE(5,(#53147,#53148,#53149,#53150,#53151,#53152,#53153,#53154,
#53155,#53156,#53157,#53158,#53159,#53160,#53161,#53162,#53163,#53164,#53165,
#53166,#53167,#53168,#53169,#53170,#53171,#53172,#53173,#53174,#53175,#53176,
#53177,#53178,#53179,#53180,#53181,#53182,#53183,#53184,#53185,#53186,#53187,
#53188,#53189,#53190,#53191,#53192,#53193,#53194,#53195,#53196,#53197,#53198,
#53199,#53200,#53201,#53202,#53203,#53204,#53205,#53206,#53207,#53208,#53209,
#53210,#53211,#53212,#53213,#53214,#53215,#53216),.UNSPECIFIED.,.F.,.F.)
B_SPLINE_CURVE_WITH_KNOTS((6,1,1,1,1,1,1,1,1,1,1,1,1,1,1,1,1,1,1,1,1,1,
1,1,1,1,1,1,1,1,1,1,1,1,1,1,1,1,1,1,1,1,1,1,1,1,1,1,1,1,1,1,1,1,1,1,1,1,
1,1,1,1,1,1,1,6),(-0.99422815673967,-0.984615384615383,-0.969230769230768,
-0.953846153846152,-0.938461538461537,-0.923076923076922,-0.907692307692306,
-0.892307692307691,-0.876923076923076,-0.86153846153846,-0.846153846153845,
-0.83076923076923,-0.815384615384614,-0.799999999999999,-0.784615384615384,
-0.769230769230768,-0.753846153846153,-0.738461538461538,-0.723076923076922,
-0.707692307692307,-0.692307692307692,-0.676923076923076,-0.661538461538461,
-0.646153846153846,-0.63076923076923,-0.615384615384615,-0.6,-0.584615384615384,
-0.569230769230769,-0.553846153846154,-0.538461538461538,-0.523076923076923,
-0.507692307692308,-0.492307692307692,-0.476923076923077,-0.461538461538462,
-0.446153846153846,-0.430769230769231,-0.415384615384615,-0.4,-0.384615384615385,
-0.369230769230769,-0.353846153846154,-0.338461538461538,-0.323076923076923,
-0.307692307692308,-0.292307692307692,-0.276923076923077,-0.261538461538462,
-0.246153846153846,-0.230769230769231,-0.215384615384615,-0.2,-0.184615384615385,
-0.169230769230769,-0.153846153846154,-0.138461538461538,-0.123076923076923,
-0.107692307692308,-0.0923076923076923,-0.0769230769230769,-0.0615384615384615,
-0.0461538461538462,-0.0307692307692308,-0.0153846153846154,0.),
 .UNSPECIFIED.)
CURVE()
GEOMETRIC_REPRESENTATION_ITEM()
RATIONAL_B_SPLINE_CURVE((1.,1.,1.,1.,1.,1.,1.,1.,1.,1.,1.,1.,1.,1.,1.,1.,
1.,1.,1.,1.,1.,1.,1.,1.,1.,1.,1.,1.,1.,1.,1.,1.,1.,1.,1.,1.,1.,1.,1.,1.,
1.,1.,1.,1.,1.,1.,1.,1.,1.,1.,1.,1.,1.,1.,1.,1.,1.,1.,1.,1.,1.,1.,1.,1.,
1.,1.,1.,1.,1.,1.))
REPRESENTATION_ITEM('')
);
#351=(
BOUNDED_CURVE()
B_SPLINE_CURVE(5,(#53369,#53370,#53371,#53372,#53373,#53374,#53375,#53376,
#53377,#53378,#53379,#53380,#53381,#53382,#53383,#53384,#53385,#53386,#53387,
#53388,#53389,#53390,#53391,#53392,#53393,#53394,#53395,#53396,#53397,#53398,
#53399,#53400,#53401,#53402,#53403,#53404,#53405,#53406,#53407,#53408,#53409,
#53410,#53411,#53412,#53413,#53414,#53415,#53416,#53417,#53418,#53419,#53420,
#53421,#53422,#53423,#53424,#53425,#53426,#53427,#53428,#53429,#53430,#53431,
#53432,#53433,#53434,#53435,#53436,#53437,#53438),.UNSPECIFIED.,.F.,.F.)
B_SPLINE_CURVE_WITH_KNOTS((6,1,1,1,1,1,1,1,1,1,1,1,1,1,1,1,1,1,1,1,1,1,
1,1,1,1,1,1,1,1,1,1,1,1,1,1,1,1,1,1,1,1,1,1,1,1,1,1,1,1,1,1,1,1,1,1,1,1,
1,1,1,1,1,1,1,6),(-1.,-0.984615384615383,-0.969230769230768,-0.953846153846152,
-0.938461538461537,-0.923076923076922,-0.907692307692306,-0.892307692307691,
-0.876923076923076,-0.86153846153846,-0.846153846153845,-0.83076923076923,
-0.815384615384614,-0.799999999999999,-0.784615384615384,-0.769230769230768,
-0.753846153846153,-0.738461538461538,-0.723076923076922,-0.707692307692307,
-0.692307692307692,-0.676923076923076,-0.661538461538461,-0.646153846153846,
-0.63076923076923,-0.615384615384615,-0.6,-0.584615384615384,-0.569230769230769,
-0.553846153846154,-0.538461538461538,-0.523076923076923,-0.507692307692308,
-0.492307692307692,-0.476923076923077,-0.461538461538462,-0.446153846153846,
-0.430769230769231,-0.415384615384615,-0.4,-0.384615384615385,-0.369230769230769,
-0.353846153846154,-0.338461538461538,-0.323076923076923,-0.307692307692308,
-0.292307692307692,-0.276923076923077,-0.261538461538462,-0.246153846153846,
-0.230769230769231,-0.215384615384615,-0.2,-0.184615384615385,-0.169230769230769,
-0.153846153846154,-0.138461538461538,-0.123076923076923,-0.107692307692308,
-0.0923076923076923,-0.0769230769230769,-0.0615384615384615,-0.0461538461538462,
-0.0307692307692308,-0.0153846153846154,-0.0057718433745009),
 .UNSPECIFIED.)
CURVE()
GEOMETRIC_REPRESENTATION_ITEM()
RATIONAL_B_SPLINE_CURVE((1.,1.,1.,1.,1.,1.,1.,1.,1.,1.,1.,1.,1.,1.,1.,1.,
1.,1.,1.,1.,1.,1.,1.,1.,1.,1.,1.,1.,1.,1.,1.,1.,1.,1.,1.,1.,1.,1.,1.,1.,
1.,1.,1.,1.,1.,1.,1.,1.,1.,1.,1.,1.,1.,1.,1.,1.,1.,1.,1.,1.,1.,1.,1.,1.,
1.,1.,1.,1.,1.,1.))
REPRESENTATION_ITEM('')
);
#352=(
BOUNDED_CURVE()
B_SPLINE_CURVE(5,(#53589,#53590,#53591,#53592,#53593,#53594,#53595,#53596,
#53597,#53598,#53599,#53600,#53601,#53602,#53603,#53604,#53605,#53606,#53607,
#53608,#53609,#53610,#53611,#53612,#53613,#53614,#53615,#53616,#53617,#53618,
#53619,#53620,#53621,#53622,#53623,#53624,#53625,#53626,#53627,#53628,#53629,
#53630,#53631,#53632,#53633,#53634,#53635,#53636,#53637,#53638,#53639,#53640,
#53641,#53642,#53643,#53644,#53645,#53646,#53647,#53648,#53649,#53650,#53651,
#53652,#53653,#53654,#53655,#53656,#53657,#53658),.UNSPECIFIED.,.F.,.F.)
B_SPLINE_CURVE_WITH_KNOTS((6,1,1,1,1,1,1,1,1,1,1,1,1,1,1,1,1,1,1,1,1,1,
1,1,1,1,1,1,1,1,1,1,1,1,1,1,1,1,1,1,1,1,1,1,1,1,1,1,1,1,1,1,1,1,1,1,1,1,
1,1,1,1,1,1,1,6),(-0.99422815673967,-0.984615384615383,-0.969230769230768,
-0.953846153846152,-0.938461538461537,-0.923076923076922,-0.907692307692306,
-0.892307692307691,-0.876923076923076,-0.86153846153846,-0.846153846153845,
-0.83076923076923,-0.815384615384614,-0.799999999999999,-0.784615384615384,
-0.769230769230768,-0.753846153846153,-0.738461538461538,-0.723076923076922,
-0.707692307692307,-0.692307692307692,-0.676923076923076,-0.661538461538461,
-0.646153846153846,-0.63076923076923,-0.615384615384615,-0.6,-0.584615384615384,
-0.569230769230769,-0.553846153846154,-0.538461538461538,-0.523076923076923,
-0.507692307692308,-0.492307692307692,-0.476923076923077,-0.461538461538462,
-0.446153846153846,-0.430769230769231,-0.415384615384615,-0.4,-0.384615384615385,
-0.369230769230769,-0.353846153846154,-0.338461538461538,-0.323076923076923,
-0.307692307692308,-0.292307692307692,-0.276923076923077,-0.261538461538462,
-0.246153846153846,-0.230769230769231,-0.215384615384615,-0.2,-0.184615384615385,
-0.169230769230769,-0.153846153846154,-0.138461538461538,-0.123076923076923,
-0.107692307692308,-0.0923076923076923,-0.0769230769230769,-0.0615384615384615,
-0.0461538461538462,-0.0307692307692308,-0.0153846153846154,0.),
 .UNSPECIFIED.)
CURVE()
GEOMETRIC_REPRESENTATION_ITEM()
RATIONAL_B_SPLINE_CURVE((1.,1.,1.,1.,1.,1.,1.,1.,1.,1.,1.,1.,1.,1.,1.,1.,
1.,1.,1.,1.,1.,1.,1.,1.,1.,1.,1.,1.,1.,1.,1.,1.,1.,1.,1.,1.,1.,1.,1.,1.,
1.,1.,1.,1.,1.,1.,1.,1.,1.,1.,1.,1.,1.,1.,1.,1.,1.,1.,1.,1.,1.,1.,1.,1.,
1.,1.,1.,1.,1.,1.))
REPRESENTATION_ITEM('')
);
#353=(
BOUNDED_CURVE()
B_SPLINE_CURVE(5,(#53811,#53812,#53813,#53814,#53815,#53816,#53817,#53818,
#53819,#53820,#53821,#53822,#53823,#53824,#53825,#53826,#53827,#53828,#53829,
#53830,#53831,#53832,#53833,#53834,#53835,#53836,#53837,#53838,#53839,#53840,
#53841,#53842,#53843,#53844,#53845,#53846,#53847,#53848,#53849,#53850,#53851,
#53852,#53853,#53854,#53855,#53856,#53857,#53858,#53859,#53860,#53861,#53862,
#53863,#53864,#53865,#53866,#53867,#53868,#53869,#53870,#53871,#53872,#53873,
#53874,#53875,#53876,#53877,#53878,#53879,#53880),.UNSPECIFIED.,.F.,.F.)
B_SPLINE_CURVE_WITH_KNOTS((6,1,1,1,1,1,1,1,1,1,1,1,1,1,1,1,1,1,1,1,1,1,
1,1,1,1,1,1,1,1,1,1,1,1,1,1,1,1,1,1,1,1,1,1,1,1,1,1,1,1,1,1,1,1,1,1,1,1,
1,1,1,1,1,1,1,6),(-1.,-0.984615384615383,-0.969230769230768,-0.953846153846152,
-0.938461538461537,-0.923076923076922,-0.907692307692306,-0.892307692307691,
-0.876923076923076,-0.86153846153846,-0.846153846153845,-0.83076923076923,
-0.815384615384614,-0.799999999999999,-0.784615384615384,-0.769230769230768,
-0.753846153846153,-0.738461538461538,-0.723076923076922,-0.707692307692307,
-0.692307692307692,-0.676923076923076,-0.661538461538461,-0.646153846153846,
-0.63076923076923,-0.615384615384615,-0.6,-0.584615384615384,-0.569230769230769,
-0.553846153846154,-0.538461538461538,-0.523076923076923,-0.507692307692308,
-0.492307692307692,-0.476923076923077,-0.461538461538462,-0.446153846153846,
-0.430769230769231,-0.415384615384615,-0.4,-0.384615384615385,-0.369230769230769,
-0.353846153846154,-0.338461538461538,-0.323076923076923,-0.307692307692308,
-0.292307692307692,-0.276923076923077,-0.261538461538462,-0.246153846153846,
-0.230769230769231,-0.215384615384615,-0.2,-0.184615384615385,-0.169230769230769,
-0.153846153846154,-0.138461538461538,-0.123076923076923,-0.107692307692308,
-0.0923076923076923,-0.0769230769230769,-0.0615384615384615,-0.0461538461538462,
-0.0307692307692308,-0.0153846153846154,-0.00577184337450701),
 .UNSPECIFIED.)
CURVE()
GEOMETRIC_REPRESENTATION_ITEM()
RATIONAL_B_SPLINE_CURVE((1.,1.,1.,1.,1.,1.,1.,1.,1.,1.,1.,1.,1.,1.,1.,1.,
1.,1.,1.,1.,1.,1.,1.,1.,1.,1.,1.,1.,1.,1.,1.,1.,1.,1.,1.,1.,1.,1.,1.,1.,
1.,1.,1.,1.,1.,1.,1.,1.,1.,1.,1.,1.,1.,1.,1.,1.,1.,1.,1.,1.,1.,1.,1.,1.,
1.,1.,1.,1.,1.,1.))
REPRESENTATION_ITEM('')
);
#354=(
BOUNDED_CURVE()
B_SPLINE_CURVE(5,(#54031,#54032,#54033,#54034,#54035,#54036,#54037,#54038,
#54039,#54040,#54041,#54042,#54043,#54044,#54045,#54046,#54047,#54048,#54049,
#54050,#54051,#54052,#54053,#54054,#54055,#54056,#54057,#54058,#54059,#54060,
#54061,#54062,#54063,#54064,#54065,#54066,#54067,#54068,#54069,#54070,#54071,
#54072,#54073,#54074,#54075,#54076,#54077,#54078,#54079,#54080,#54081,#54082,
#54083,#54084,#54085,#54086,#54087,#54088,#54089,#54090,#54091,#54092,#54093,
#54094,#54095,#54096,#54097,#54098,#54099,#54100),.UNSPECIFIED.,.F.,.F.)
B_SPLINE_CURVE_WITH_KNOTS((6,1,1,1,1,1,1,1,1,1,1,1,1,1,1,1,1,1,1,1,1,1,
1,1,1,1,1,1,1,1,1,1,1,1,1,1,1,1,1,1,1,1,1,1,1,1,1,1,1,1,1,1,1,1,1,1,1,1,
1,1,1,1,1,1,1,6),(-0.994228156739689,-0.984615384615383,-0.969230769230768,
-0.953846153846152,-0.938461538461537,-0.923076923076922,-0.907692307692306,
-0.892307692307691,-0.876923076923076,-0.86153846153846,-0.846153846153845,
-0.83076923076923,-0.815384615384614,-0.799999999999999,-0.784615384615384,
-0.769230769230768,-0.753846153846153,-0.738461538461538,-0.723076923076922,
-0.707692307692307,-0.692307692307692,-0.676923076923076,-0.661538461538461,
-0.646153846153846,-0.63076923076923,-0.615384615384615,-0.6,-0.584615384615384,
-0.569230769230769,-0.553846153846154,-0.538461538461538,-0.523076923076923,
-0.507692307692308,-0.492307692307692,-0.476923076923077,-0.461538461538462,
-0.446153846153846,-0.430769230769231,-0.415384615384615,-0.4,-0.384615384615385,
-0.369230769230769,-0.353846153846154,-0.338461538461538,-0.323076923076923,
-0.307692307692308,-0.292307692307692,-0.276923076923077,-0.261538461538462,
-0.246153846153846,-0.230769230769231,-0.215384615384615,-0.2,-0.184615384615385,
-0.169230769230769,-0.153846153846154,-0.138461538461538,-0.123076923076923,
-0.107692307692308,-0.0923076923076923,-0.0769230769230769,-0.0615384615384615,
-0.0461538461538462,-0.0307692307692308,-0.0153846153846154,0.),
 .UNSPECIFIED.)
CURVE()
GEOMETRIC_REPRESENTATION_ITEM()
RATIONAL_B_SPLINE_CURVE((1.,1.,1.,1.,1.,1.,1.,1.,1.,1.,1.,1.,1.,1.,1.,1.,
1.,1.,1.,1.,1.,1.,1.,1.,1.,1.,1.,1.,1.,1.,1.,1.,1.,1.,1.,1.,1.,1.,1.,1.,
1.,1.,1.,1.,1.,1.,1.,1.,1.,1.,1.,1.,1.,1.,1.,1.,1.,1.,1.,1.,1.,1.,1.,1.,
1.,1.,1.,1.,1.,1.))
REPRESENTATION_ITEM('')
);
#355=(
BOUNDED_CURVE()
B_SPLINE_CURVE(5,(#54253,#54254,#54255,#54256,#54257,#54258,#54259,#54260,
#54261,#54262,#54263,#54264,#54265,#54266,#54267,#54268,#54269,#54270,#54271,
#54272,#54273,#54274,#54275,#54276,#54277,#54278,#54279,#54280,#54281,#54282,
#54283,#54284,#54285,#54286,#54287,#54288,#54289,#54290,#54291,#54292,#54293,
#54294,#54295,#54296,#54297,#54298,#54299,#54300,#54301,#54302,#54303,#54304,
#54305,#54306,#54307,#54308,#54309,#54310,#54311,#54312,#54313,#54314,#54315,
#54316,#54317,#54318,#54319,#54320,#54321,#54322),.UNSPECIFIED.,.F.,.F.)
B_SPLINE_CURVE_WITH_KNOTS((6,1,1,1,1,1,1,1,1,1,1,1,1,1,1,1,1,1,1,1,1,1,
1,1,1,1,1,1,1,1,1,1,1,1,1,1,1,1,1,1,1,1,1,1,1,1,1,1,1,1,1,1,1,1,1,1,1,1,
1,1,1,1,1,1,1,6),(-1.,-0.984615384615383,-0.969230769230768,-0.953846153846152,
-0.938461538461537,-0.923076923076922,-0.907692307692306,-0.892307692307691,
-0.876923076923076,-0.86153846153846,-0.846153846153845,-0.83076923076923,
-0.815384615384614,-0.799999999999999,-0.784615384615384,-0.769230769230768,
-0.753846153846153,-0.738461538461538,-0.723076923076922,-0.707692307692307,
-0.692307692307692,-0.676923076923076,-0.661538461538461,-0.646153846153846,
-0.63076923076923,-0.615384615384615,-0.6,-0.584615384615384,-0.569230769230769,
-0.553846153846154,-0.538461538461538,-0.523076923076923,-0.507692307692308,
-0.492307692307692,-0.476923076923077,-0.461538461538462,-0.446153846153846,
-0.430769230769231,-0.415384615384615,-0.4,-0.384615384615385,-0.369230769230769,
-0.353846153846154,-0.338461538461538,-0.323076923076923,-0.307692307692308,
-0.292307692307692,-0.276923076923077,-0.261538461538462,-0.246153846153846,
-0.230769230769231,-0.215384615384615,-0.2,-0.184615384615385,-0.169230769230769,
-0.153846153846154,-0.138461538461538,-0.123076923076923,-0.107692307692308,
-0.0923076923076923,-0.0769230769230769,-0.0615384615384615,-0.0461538461538462,
-0.0307692307692308,-0.0153846153846154,-0.00577184337452382),
 .UNSPECIFIED.)
CURVE()
GEOMETRIC_REPRESENTATION_ITEM()
RATIONAL_B_SPLINE_CURVE((1.,1.,1.,1.,1.,1.,1.,1.,1.,1.,1.,1.,1.,1.,1.,1.,
1.,1.,1.,1.,1.,1.,1.,1.,1.,1.,1.,1.,1.,1.,1.,1.,1.,1.,1.,1.,1.,1.,1.,1.,
1.,1.,1.,1.,1.,1.,1.,1.,1.,1.,1.,1.,1.,1.,1.,1.,1.,1.,1.,1.,1.,1.,1.,1.,
1.,1.,1.,1.,1.,1.))
REPRESENTATION_ITEM('')
);
#356=(
BOUNDED_CURVE()
B_SPLINE_CURVE(5,(#54473,#54474,#54475,#54476,#54477,#54478,#54479,#54480,
#54481,#54482,#54483,#54484,#54485,#54486,#54487,#54488,#54489,#54490,#54491,
#54492,#54493,#54494,#54495,#54496,#54497,#54498,#54499,#54500,#54501,#54502,
#54503,#54504,#54505,#54506,#54507,#54508,#54509,#54510,#54511,#54512,#54513,
#54514,#54515,#54516,#54517,#54518,#54519,#54520,#54521,#54522,#54523,#54524,
#54525,#54526,#54527,#54528,#54529,#54530,#54531,#54532,#54533,#54534,#54535,
#54536,#54537,#54538,#54539,#54540,#54541,#54542),.UNSPECIFIED.,.F.,.F.)
B_SPLINE_CURVE_WITH_KNOTS((6,1,1,1,1,1,1,1,1,1,1,1,1,1,1,1,1,1,1,1,1,1,
1,1,1,1,1,1,1,1,1,1,1,1,1,1,1,1,1,1,1,1,1,1,1,1,1,1,1,1,1,1,1,1,1,1,1,1,
1,1,1,1,1,1,1,6),(-0.994228156739677,-0.984615384615383,-0.969230769230768,
-0.953846153846152,-0.938461538461537,-0.923076923076922,-0.907692307692306,
-0.892307692307691,-0.876923076923076,-0.86153846153846,-0.846153846153845,
-0.83076923076923,-0.815384615384614,-0.799999999999999,-0.784615384615384,
-0.769230769230768,-0.753846153846153,-0.738461538461538,-0.723076923076922,
-0.707692307692307,-0.692307692307692,-0.676923076923076,-0.661538461538461,
-0.646153846153846,-0.63076923076923,-0.615384615384615,-0.6,-0.584615384615384,
-0.569230769230769,-0.553846153846154,-0.538461538461538,-0.523076923076923,
-0.507692307692308,-0.492307692307692,-0.476923076923077,-0.461538461538462,
-0.446153846153846,-0.430769230769231,-0.415384615384615,-0.4,-0.384615384615385,
-0.369230769230769,-0.353846153846154,-0.338461538461538,-0.323076923076923,
-0.307692307692308,-0.292307692307692,-0.276923076923077,-0.261538461538462,
-0.246153846153846,-0.230769230769231,-0.215384615384615,-0.2,-0.184615384615385,
-0.169230769230769,-0.153846153846154,-0.138461538461538,-0.123076923076923,
-0.107692307692308,-0.0923076923076923,-0.0769230769230769,-0.0615384615384615,
-0.0461538461538462,-0.0307692307692308,-0.0153846153846154,0.),
 .UNSPECIFIED.)
CURVE()
GEOMETRIC_REPRESENTATION_ITEM()
RATIONAL_B_SPLINE_CURVE((1.,1.,1.,1.,1.,1.,1.,1.,1.,1.,1.,1.,1.,1.,1.,1.,
1.,1.,1.,1.,1.,1.,1.,1.,1.,1.,1.,1.,1.,1.,1.,1.,1.,1.,1.,1.,1.,1.,1.,1.,
1.,1.,1.,1.,1.,1.,1.,1.,1.,1.,1.,1.,1.,1.,1.,1.,1.,1.,1.,1.,1.,1.,1.,1.,
1.,1.,1.,1.,1.,1.))
REPRESENTATION_ITEM('')
);
#357=(
BOUNDED_CURVE()
B_SPLINE_CURVE(5,(#54695,#54696,#54697,#54698,#54699,#54700,#54701,#54702,
#54703,#54704,#54705,#54706,#54707,#54708,#54709,#54710,#54711,#54712,#54713,
#54714,#54715,#54716,#54717,#54718,#54719,#54720,#54721,#54722,#54723,#54724,
#54725,#54726,#54727,#54728,#54729,#54730,#54731,#54732,#54733,#54734,#54735,
#54736,#54737,#54738,#54739,#54740,#54741,#54742,#54743,#54744,#54745,#54746,
#54747,#54748,#54749,#54750,#54751,#54752,#54753,#54754,#54755,#54756,#54757,
#54758,#54759,#54760,#54761,#54762,#54763,#54764),.UNSPECIFIED.,.F.,.F.)
B_SPLINE_CURVE_WITH_KNOTS((6,1,1,1,1,1,1,1,1,1,1,1,1,1,1,1,1,1,1,1,1,1,
1,1,1,1,1,1,1,1,1,1,1,1,1,1,1,1,1,1,1,1,1,1,1,1,1,1,1,1,1,1,1,1,1,1,1,1,
1,1,1,1,1,1,1,6),(-1.,-0.984615384615383,-0.969230769230768,-0.953846153846152,
-0.938461538461537,-0.923076923076922,-0.907692307692306,-0.892307692307691,
-0.876923076923076,-0.86153846153846,-0.846153846153845,-0.83076923076923,
-0.815384615384614,-0.799999999999999,-0.784615384615384,-0.769230769230768,
-0.753846153846153,-0.738461538461538,-0.723076923076922,-0.707692307692307,
-0.692307692307692,-0.676923076923076,-0.661538461538461,-0.646153846153846,
-0.63076923076923,-0.615384615384615,-0.6,-0.584615384615384,-0.569230769230769,
-0.553846153846154,-0.538461538461538,-0.523076923076923,-0.507692307692308,
-0.492307692307692,-0.476923076923077,-0.461538461538462,-0.446153846153846,
-0.430769230769231,-0.415384615384615,-0.4,-0.384615384615385,-0.369230769230769,
-0.353846153846154,-0.338461538461538,-0.323076923076923,-0.307692307692308,
-0.292307692307692,-0.276923076923077,-0.261538461538462,-0.246153846153846,
-0.230769230769231,-0.215384615384615,-0.2,-0.184615384615385,-0.169230769230769,
-0.153846153846154,-0.138461538461538,-0.123076923076923,-0.107692307692308,
-0.0923076923076923,-0.0769230769230769,-0.0615384615384615,-0.0461538461538462,
-0.0307692307692308,-0.0153846153846154,-0.0057718433744938),
 .UNSPECIFIED.)
CURVE()
GEOMETRIC_REPRESENTATION_ITEM()
RATIONAL_B_SPLINE_CURVE((1.,1.,1.,1.,1.,1.,1.,1.,1.,1.,1.,1.,1.,1.,1.,1.,
1.,1.,1.,1.,1.,1.,1.,1.,1.,1.,1.,1.,1.,1.,1.,1.,1.,1.,1.,1.,1.,1.,1.,1.,
1.,1.,1.,1.,1.,1.,1.,1.,1.,1.,1.,1.,1.,1.,1.,1.,1.,1.,1.,1.,1.,1.,1.,1.,
1.,1.,1.,1.,1.,1.))
REPRESENTATION_ITEM('')
);
#358=(
BOUNDED_CURVE()
B_SPLINE_CURVE(5,(#54915,#54916,#54917,#54918,#54919,#54920,#54921,#54922,
#54923,#54924,#54925,#54926,#54927,#54928,#54929,#54930,#54931,#54932,#54933,
#54934,#54935,#54936,#54937,#54938,#54939,#54940,#54941,#54942,#54943,#54944,
#54945,#54946,#54947,#54948,#54949,#54950,#54951,#54952,#54953,#54954,#54955,
#54956,#54957,#54958,#54959,#54960,#54961,#54962,#54963,#54964,#54965,#54966,
#54967,#54968,#54969,#54970,#54971,#54972,#54973,#54974,#54975,#54976,#54977,
#54978,#54979,#54980,#54981,#54982,#54983,#54984),.UNSPECIFIED.,.F.,.F.)
B_SPLINE_CURVE_WITH_KNOTS((6,1,1,1,1,1,1,1,1,1,1,1,1,1,1,1,1,1,1,1,1,1,
1,1,1,1,1,1,1,1,1,1,1,1,1,1,1,1,1,1,1,1,1,1,1,1,1,1,1,1,1,1,1,1,1,1,1,1,
1,1,1,1,1,1,1,6),(-0.994228156739743,-0.984615384615383,-0.969230769230768,
-0.953846153846152,-0.938461538461537,-0.923076923076922,-0.907692307692306,
-0.892307692307691,-0.876923076923076,-0.86153846153846,-0.846153846153845,
-0.83076923076923,-0.815384615384614,-0.799999999999999,-0.784615384615384,
-0.769230769230768,-0.753846153846153,-0.738461538461538,-0.723076923076922,
-0.707692307692307,-0.692307692307692,-0.676923076923076,-0.661538461538461,
-0.646153846153846,-0.63076923076923,-0.615384615384615,-0.6,-0.584615384615384,
-0.569230769230769,-0.553846153846154,-0.538461538461538,-0.523076923076923,
-0.507692307692308,-0.492307692307692,-0.476923076923077,-0.461538461538462,
-0.446153846153846,-0.430769230769231,-0.415384615384615,-0.4,-0.384615384615385,
-0.369230769230769,-0.353846153846154,-0.338461538461538,-0.323076923076923,
-0.307692307692308,-0.292307692307692,-0.276923076923077,-0.261538461538462,
-0.246153846153846,-0.230769230769231,-0.215384615384615,-0.2,-0.184615384615385,
-0.169230769230769,-0.153846153846154,-0.138461538461538,-0.123076923076923,
-0.107692307692308,-0.0923076923076923,-0.0769230769230769,-0.0615384615384615,
-0.0461538461538462,-0.0307692307692308,-0.0153846153846154,0.),
 .UNSPECIFIED.)
CURVE()
GEOMETRIC_REPRESENTATION_ITEM()
RATIONAL_B_SPLINE_CURVE((1.,1.,1.,1.,1.,1.,1.,1.,1.,1.,1.,1.,1.,1.,1.,1.,
1.,1.,1.,1.,1.,1.,1.,1.,1.,1.,1.,1.,1.,1.,1.,1.,1.,1.,1.,1.,1.,1.,1.,1.,
1.,1.,1.,1.,1.,1.,1.,1.,1.,1.,1.,1.,1.,1.,1.,1.,1.,1.,1.,1.,1.,1.,1.,1.,
1.,1.,1.,1.,1.,1.))
REPRESENTATION_ITEM('')
);
#359=(
BOUNDED_CURVE()
B_SPLINE_CURVE(5,(#55137,#55138,#55139,#55140,#55141,#55142,#55143,#55144,
#55145,#55146,#55147,#55148,#55149,#55150,#55151,#55152,#55153,#55154,#55155,
#55156,#55157,#55158,#55159,#55160,#55161,#55162,#55163,#55164,#55165,#55166,
#55167,#55168,#55169,#55170,#55171,#55172,#55173,#55174,#55175,#55176,#55177,
#55178,#55179,#55180,#55181,#55182,#55183,#55184,#55185,#55186,#55187,#55188,
#55189,#55190,#55191,#55192,#55193,#55194,#55195,#55196,#55197,#55198,#55199,
#55200,#55201,#55202,#55203,#55204,#55205,#55206),.UNSPECIFIED.,.F.,.F.)
B_SPLINE_CURVE_WITH_KNOTS((6,1,1,1,1,1,1,1,1,1,1,1,1,1,1,1,1,1,1,1,1,1,
1,1,1,1,1,1,1,1,1,1,1,1,1,1,1,1,1,1,1,1,1,1,1,1,1,1,1,1,1,1,1,1,1,1,1,1,
1,1,1,1,1,1,1,6),(-1.,-0.984615384615383,-0.969230769230768,-0.953846153846152,
-0.938461538461537,-0.923076923076922,-0.907692307692306,-0.892307692307691,
-0.876923076923076,-0.86153846153846,-0.846153846153845,-0.83076923076923,
-0.815384615384614,-0.799999999999999,-0.784615384615384,-0.769230769230768,
-0.753846153846153,-0.738461538461538,-0.723076923076922,-0.707692307692307,
-0.692307692307692,-0.676923076923076,-0.661538461538461,-0.646153846153846,
-0.63076923076923,-0.615384615384615,-0.6,-0.584615384615384,-0.569230769230769,
-0.553846153846154,-0.538461538461538,-0.523076923076923,-0.507692307692308,
-0.492307692307692,-0.476923076923077,-0.461538461538462,-0.446153846153846,
-0.430769230769231,-0.415384615384615,-0.4,-0.384615384615385,-0.369230769230769,
-0.353846153846154,-0.338461538461538,-0.323076923076923,-0.307692307692308,
-0.292307692307692,-0.276923076923077,-0.261538461538462,-0.246153846153846,
-0.230769230769231,-0.215384615384615,-0.2,-0.184615384615385,-0.169230769230769,
-0.153846153846154,-0.138461538461538,-0.123076923076923,-0.107692307692308,
-0.0923076923076923,-0.0769230769230769,-0.0615384615384615,-0.0461538461538462,
-0.0307692307692308,-0.0153846153846154,-0.0057718433745291),
 .UNSPECIFIED.)
CURVE()
GEOMETRIC_REPRESENTATION_ITEM()
RATIONAL_B_SPLINE_CURVE((1.,1.,1.,1.,1.,1.,1.,1.,1.,1.,1.,1.,1.,1.,1.,1.,
1.,1.,1.,1.,1.,1.,1.,1.,1.,1.,1.,1.,1.,1.,1.,1.,1.,1.,1.,1.,1.,1.,1.,1.,
1.,1.,1.,1.,1.,1.,1.,1.,1.,1.,1.,1.,1.,1.,1.,1.,1.,1.,1.,1.,1.,1.,1.,1.,
1.,1.,1.,1.,1.,1.))
REPRESENTATION_ITEM('')
);
#360=(
BOUNDED_CURVE()
B_SPLINE_CURVE(5,(#55357,#55358,#55359,#55360,#55361,#55362,#55363,#55364,
#55365,#55366,#55367,#55368,#55369,#55370,#55371,#55372,#55373,#55374,#55375,
#55376,#55377,#55378,#55379,#55380,#55381,#55382,#55383,#55384,#55385,#55386,
#55387,#55388,#55389,#55390,#55391,#55392,#55393,#55394,#55395,#55396,#55397,
#55398,#55399,#55400,#55401,#55402,#55403,#55404,#55405,#55406,#55407,#55408,
#55409,#55410,#55411,#55412,#55413,#55414,#55415,#55416,#55417,#55418,#55419,
#55420,#55421,#55422,#55423,#55424,#55425,#55426),.UNSPECIFIED.,.F.,.F.)
B_SPLINE_CURVE_WITH_KNOTS((6,1,1,1,1,1,1,1,1,1,1,1,1,1,1,1,1,1,1,1,1,1,
1,1,1,1,1,1,1,1,1,1,1,1,1,1,1,1,1,1,1,1,1,1,1,1,1,1,1,1,1,1,1,1,1,1,1,1,
1,1,1,1,1,1,1,6),(-0.994228156739665,-0.984615384615383,-0.969230769230768,
-0.953846153846152,-0.938461538461537,-0.923076923076922,-0.907692307692306,
-0.892307692307691,-0.876923076923076,-0.86153846153846,-0.846153846153845,
-0.83076923076923,-0.815384615384614,-0.799999999999999,-0.784615384615384,
-0.769230769230768,-0.753846153846153,-0.738461538461538,-0.723076923076922,
-0.707692307692307,-0.692307692307692,-0.676923076923076,-0.661538461538461,
-0.646153846153846,-0.63076923076923,-0.615384615384615,-0.6,-0.584615384615384,
-0.569230769230769,-0.553846153846154,-0.538461538461538,-0.523076923076923,
-0.507692307692308,-0.492307692307692,-0.476923076923077,-0.461538461538462,
-0.446153846153846,-0.430769230769231,-0.415384615384615,-0.4,-0.384615384615385,
-0.369230769230769,-0.353846153846154,-0.338461538461538,-0.323076923076923,
-0.307692307692308,-0.292307692307692,-0.276923076923077,-0.261538461538462,
-0.246153846153846,-0.230769230769231,-0.215384615384615,-0.2,-0.184615384615385,
-0.169230769230769,-0.153846153846154,-0.138461538461538,-0.123076923076923,
-0.107692307692308,-0.0923076923076923,-0.0769230769230769,-0.0615384615384615,
-0.0461538461538462,-0.0307692307692308,-0.0153846153846154,0.),
 .UNSPECIFIED.)
CURVE()
GEOMETRIC_REPRESENTATION_ITEM()
RATIONAL_B_SPLINE_CURVE((1.,1.,1.,1.,1.,1.,1.,1.,1.,1.,1.,1.,1.,1.,1.,1.,
1.,1.,1.,1.,1.,1.,1.,1.,1.,1.,1.,1.,1.,1.,1.,1.,1.,1.,1.,1.,1.,1.,1.,1.,
1.,1.,1.,1.,1.,1.,1.,1.,1.,1.,1.,1.,1.,1.,1.,1.,1.,1.,1.,1.,1.,1.,1.,1.,
1.,1.,1.,1.,1.,1.))
REPRESENTATION_ITEM('')
);
#361=(
BOUNDED_CURVE()
B_SPLINE_CURVE(5,(#55579,#55580,#55581,#55582,#55583,#55584,#55585,#55586,
#55587,#55588,#55589,#55590,#55591,#55592,#55593,#55594,#55595,#55596,#55597,
#55598,#55599,#55600,#55601,#55602,#55603,#55604,#55605,#55606,#55607,#55608,
#55609,#55610,#55611,#55612,#55613,#55614,#55615,#55616,#55617,#55618,#55619,
#55620,#55621,#55622,#55623,#55624,#55625,#55626,#55627,#55628,#55629,#55630,
#55631,#55632,#55633,#55634,#55635,#55636,#55637,#55638,#55639,#55640,#55641,
#55642,#55643,#55644,#55645,#55646,#55647,#55648),.UNSPECIFIED.,.F.,.F.)
B_SPLINE_CURVE_WITH_KNOTS((6,1,1,1,1,1,1,1,1,1,1,1,1,1,1,1,1,1,1,1,1,1,
1,1,1,1,1,1,1,1,1,1,1,1,1,1,1,1,1,1,1,1,1,1,1,1,1,1,1,1,1,1,1,1,1,1,1,1,
1,1,1,1,1,1,1,6),(-1.,-0.984615384615383,-0.969230769230768,-0.953846153846152,
-0.938461538461537,-0.923076923076922,-0.907692307692306,-0.892307692307691,
-0.876923076923076,-0.86153846153846,-0.846153846153845,-0.83076923076923,
-0.815384615384614,-0.799999999999999,-0.784615384615384,-0.769230769230768,
-0.753846153846153,-0.738461538461538,-0.723076923076922,-0.707692307692307,
-0.692307692307692,-0.676923076923076,-0.661538461538461,-0.646153846153846,
-0.63076923076923,-0.615384615384615,-0.6,-0.584615384615384,-0.569230769230769,
-0.553846153846154,-0.538461538461538,-0.523076923076923,-0.507692307692308,
-0.492307692307692,-0.476923076923077,-0.461538461538462,-0.446153846153846,
-0.430769230769231,-0.415384615384615,-0.4,-0.384615384615385,-0.369230769230769,
-0.353846153846154,-0.338461538461538,-0.323076923076923,-0.307692307692308,
-0.292307692307692,-0.276923076923077,-0.261538461538462,-0.246153846153846,
-0.230769230769231,-0.215384615384615,-0.2,-0.184615384615385,-0.169230769230769,
-0.153846153846154,-0.138461538461538,-0.123076923076923,-0.107692307692308,
-0.0923076923076923,-0.0769230769230769,-0.0615384615384615,-0.0461538461538462,
-0.0307692307692308,-0.0153846153846154,-0.00577184337450666),
 .UNSPECIFIED.)
CURVE()
GEOMETRIC_REPRESENTATION_ITEM()
RATIONAL_B_SPLINE_CURVE((1.,1.,1.,1.,1.,1.,1.,1.,1.,1.,1.,1.,1.,1.,1.,1.,
1.,1.,1.,1.,1.,1.,1.,1.,1.,1.,1.,1.,1.,1.,1.,1.,1.,1.,1.,1.,1.,1.,1.,1.,
1.,1.,1.,1.,1.,1.,1.,1.,1.,1.,1.,1.,1.,1.,1.,1.,1.,1.,1.,1.,1.,1.,1.,1.,
1.,1.,1.,1.,1.,1.))
REPRESENTATION_ITEM('')
);
#362=(
BOUNDED_CURVE()
B_SPLINE_CURVE(5,(#55799,#55800,#55801,#55802,#55803,#55804,#55805,#55806,
#55807,#55808,#55809,#55810,#55811,#55812,#55813,#55814,#55815,#55816,#55817,
#55818,#55819,#55820,#55821,#55822,#55823,#55824,#55825,#55826,#55827,#55828,
#55829,#55830,#55831,#55832,#55833,#55834,#55835,#55836,#55837,#55838,#55839,
#55840,#55841,#55842,#55843,#55844,#55845,#55846,#55847,#55848,#55849,#55850,
#55851,#55852,#55853,#55854,#55855,#55856,#55857,#55858,#55859,#55860,#55861,
#55862,#55863,#55864,#55865,#55866,#55867,#55868),.UNSPECIFIED.,.F.,.F.)
B_SPLINE_CURVE_WITH_KNOTS((6,1,1,1,1,1,1,1,1,1,1,1,1,1,1,1,1,1,1,1,1,1,
1,1,1,1,1,1,1,1,1,1,1,1,1,1,1,1,1,1,1,1,1,1,1,1,1,1,1,1,1,1,1,1,1,1,1,1,
1,1,1,1,1,1,1,6),(-0.994228156739758,-0.984615384615383,-0.969230769230768,
-0.953846153846152,-0.938461538461537,-0.923076923076922,-0.907692307692306,
-0.892307692307691,-0.876923076923076,-0.86153846153846,-0.846153846153845,
-0.83076923076923,-0.815384615384614,-0.799999999999999,-0.784615384615384,
-0.769230769230768,-0.753846153846153,-0.738461538461538,-0.723076923076922,
-0.707692307692307,-0.692307692307692,-0.676923076923076,-0.661538461538461,
-0.646153846153846,-0.63076923076923,-0.615384615384615,-0.6,-0.584615384615384,
-0.569230769230769,-0.553846153846154,-0.538461538461538,-0.523076923076923,
-0.507692307692308,-0.492307692307692,-0.476923076923077,-0.461538461538462,
-0.446153846153846,-0.430769230769231,-0.415384615384615,-0.4,-0.384615384615385,
-0.369230769230769,-0.353846153846154,-0.338461538461538,-0.323076923076923,
-0.307692307692308,-0.292307692307692,-0.276923076923077,-0.261538461538462,
-0.246153846153846,-0.230769230769231,-0.215384615384615,-0.2,-0.184615384615385,
-0.169230769230769,-0.153846153846154,-0.138461538461538,-0.123076923076923,
-0.107692307692308,-0.0923076923076923,-0.0769230769230769,-0.0615384615384615,
-0.0461538461538462,-0.0307692307692308,-0.0153846153846154,0.),
 .UNSPECIFIED.)
CURVE()
GEOMETRIC_REPRESENTATION_ITEM()
RATIONAL_B_SPLINE_CURVE((1.,1.,1.,1.,1.,1.,1.,1.,1.,1.,1.,1.,1.,1.,1.,1.,
1.,1.,1.,1.,1.,1.,1.,1.,1.,1.,1.,1.,1.,1.,1.,1.,1.,1.,1.,1.,1.,1.,1.,1.,
1.,1.,1.,1.,1.,1.,1.,1.,1.,1.,1.,1.,1.,1.,1.,1.,1.,1.,1.,1.,1.,1.,1.,1.,
1.,1.,1.,1.,1.,1.))
REPRESENTATION_ITEM('')
);
#363=(
BOUNDED_CURVE()
B_SPLINE_CURVE(5,(#56021,#56022,#56023,#56024,#56025,#56026,#56027,#56028,
#56029,#56030,#56031,#56032,#56033,#56034,#56035,#56036,#56037,#56038,#56039,
#56040,#56041,#56042,#56043,#56044,#56045,#56046,#56047,#56048,#56049,#56050,
#56051,#56052,#56053,#56054,#56055,#56056,#56057,#56058,#56059,#56060,#56061,
#56062,#56063,#56064,#56065,#56066,#56067,#56068,#56069,#56070,#56071,#56072,
#56073,#56074,#56075,#56076,#56077,#56078,#56079,#56080,#56081,#56082,#56083,
#56084,#56085,#56086,#56087,#56088,#56089,#56090),.UNSPECIFIED.,.F.,.F.)
B_SPLINE_CURVE_WITH_KNOTS((6,1,1,1,1,1,1,1,1,1,1,1,1,1,1,1,1,1,1,1,1,1,
1,1,1,1,1,1,1,1,1,1,1,1,1,1,1,1,1,1,1,1,1,1,1,1,1,1,1,1,1,1,1,1,1,1,1,1,
1,1,1,1,1,1,1,6),(-1.,-0.984615384615383,-0.969230769230768,-0.953846153846152,
-0.938461538461537,-0.923076923076922,-0.907692307692306,-0.892307692307691,
-0.876923076923076,-0.86153846153846,-0.846153846153845,-0.83076923076923,
-0.815384615384614,-0.799999999999999,-0.784615384615384,-0.769230769230768,
-0.753846153846153,-0.738461538461538,-0.723076923076922,-0.707692307692307,
-0.692307692307692,-0.676923076923076,-0.661538461538461,-0.646153846153846,
-0.63076923076923,-0.615384615384615,-0.6,-0.584615384615384,-0.569230769230769,
-0.553846153846154,-0.538461538461538,-0.523076923076923,-0.507692307692308,
-0.492307692307692,-0.476923076923077,-0.461538461538462,-0.446153846153846,
-0.430769230769231,-0.415384615384615,-0.4,-0.384615384615385,-0.369230769230769,
-0.353846153846154,-0.338461538461538,-0.323076923076923,-0.307692307692308,
-0.292307692307692,-0.276923076923077,-0.261538461538462,-0.246153846153846,
-0.230769230769231,-0.215384615384615,-0.2,-0.184615384615385,-0.169230769230769,
-0.153846153846154,-0.138461538461538,-0.123076923076923,-0.107692307692308,
-0.0923076923076923,-0.0769230769230769,-0.0615384615384615,-0.0461538461538462,
-0.0307692307692308,-0.0153846153846154,-0.00577184337451981),
 .UNSPECIFIED.)
CURVE()
GEOMETRIC_REPRESENTATION_ITEM()
RATIONAL_B_SPLINE_CURVE((1.,1.,1.,1.,1.,1.,1.,1.,1.,1.,1.,1.,1.,1.,1.,1.,
1.,1.,1.,1.,1.,1.,1.,1.,1.,1.,1.,1.,1.,1.,1.,1.,1.,1.,1.,1.,1.,1.,1.,1.,
1.,1.,1.,1.,1.,1.,1.,1.,1.,1.,1.,1.,1.,1.,1.,1.,1.,1.,1.,1.,1.,1.,1.,1.,
1.,1.,1.,1.,1.,1.))
REPRESENTATION_ITEM('')
);
#364=(
BOUNDED_CURVE()
B_SPLINE_CURVE(5,(#56241,#56242,#56243,#56244,#56245,#56246,#56247,#56248,
#56249,#56250,#56251,#56252,#56253,#56254,#56255,#56256,#56257,#56258,#56259,
#56260,#56261,#56262,#56263,#56264,#56265,#56266,#56267,#56268,#56269,#56270,
#56271,#56272,#56273,#56274,#56275,#56276,#56277,#56278,#56279,#56280,#56281,
#56282,#56283,#56284,#56285,#56286,#56287,#56288,#56289,#56290,#56291,#56292,
#56293,#56294,#56295,#56296,#56297,#56298,#56299,#56300,#56301,#56302,#56303,
#56304,#56305,#56306,#56307,#56308,#56309,#56310),.UNSPECIFIED.,.F.,.F.)
B_SPLINE_CURVE_WITH_KNOTS((6,1,1,1,1,1,1,1,1,1,1,1,1,1,1,1,1,1,1,1,1,1,
1,1,1,1,1,1,1,1,1,1,1,1,1,1,1,1,1,1,1,1,1,1,1,1,1,1,1,1,1,1,1,1,1,1,1,1,
1,1,1,1,1,1,1,6),(-0.994228156739659,-0.984615384615383,-0.969230769230768,
-0.953846153846152,-0.938461538461537,-0.923076923076922,-0.907692307692306,
-0.892307692307691,-0.876923076923076,-0.86153846153846,-0.846153846153845,
-0.83076923076923,-0.815384615384614,-0.799999999999999,-0.784615384615384,
-0.769230769230768,-0.753846153846153,-0.738461538461538,-0.723076923076922,
-0.707692307692307,-0.692307692307692,-0.676923076923076,-0.661538461538461,
-0.646153846153846,-0.63076923076923,-0.615384615384615,-0.6,-0.584615384615384,
-0.569230769230769,-0.553846153846154,-0.538461538461538,-0.523076923076923,
-0.507692307692308,-0.492307692307692,-0.476923076923077,-0.461538461538462,
-0.446153846153846,-0.430769230769231,-0.415384615384615,-0.4,-0.384615384615385,
-0.369230769230769,-0.353846153846154,-0.338461538461538,-0.323076923076923,
-0.307692307692308,-0.292307692307692,-0.276923076923077,-0.261538461538462,
-0.246153846153846,-0.230769230769231,-0.215384615384615,-0.2,-0.184615384615385,
-0.169230769230769,-0.153846153846154,-0.138461538461538,-0.123076923076923,
-0.107692307692308,-0.0923076923076923,-0.0769230769230769,-0.0615384615384615,
-0.0461538461538462,-0.0307692307692308,-0.0153846153846154,0.),
 .UNSPECIFIED.)
CURVE()
GEOMETRIC_REPRESENTATION_ITEM()
RATIONAL_B_SPLINE_CURVE((1.,1.,1.,1.,1.,1.,1.,1.,1.,1.,1.,1.,1.,1.,1.,1.,
1.,1.,1.,1.,1.,1.,1.,1.,1.,1.,1.,1.,1.,1.,1.,1.,1.,1.,1.,1.,1.,1.,1.,1.,
1.,1.,1.,1.,1.,1.,1.,1.,1.,1.,1.,1.,1.,1.,1.,1.,1.,1.,1.,1.,1.,1.,1.,1.,
1.,1.,1.,1.,1.,1.))
REPRESENTATION_ITEM('')
);
#365=(
BOUNDED_CURVE()
B_SPLINE_CURVE(5,(#56463,#56464,#56465,#56466,#56467,#56468,#56469,#56470,
#56471,#56472,#56473,#56474,#56475,#56476,#56477,#56478,#56479,#56480,#56481,
#56482,#56483,#56484,#56485,#56486,#56487,#56488,#56489,#56490,#56491,#56492,
#56493,#56494,#56495,#56496,#56497,#56498,#56499,#56500,#56501,#56502,#56503,
#56504,#56505,#56506,#56507,#56508,#56509,#56510,#56511,#56512,#56513,#56514,
#56515,#56516,#56517,#56518,#56519,#56520,#56521,#56522,#56523,#56524,#56525,
#56526,#56527,#56528,#56529,#56530,#56531,#56532),.UNSPECIFIED.,.F.,.F.)
B_SPLINE_CURVE_WITH_KNOTS((6,1,1,1,1,1,1,1,1,1,1,1,1,1,1,1,1,1,1,1,1,1,
1,1,1,1,1,1,1,1,1,1,1,1,1,1,1,1,1,1,1,1,1,1,1,1,1,1,1,1,1,1,1,1,1,1,1,1,
1,1,1,1,1,1,1,6),(-1.,-0.984615384615383,-0.969230769230768,-0.953846153846152,
-0.938461538461537,-0.923076923076922,-0.907692307692306,-0.892307692307691,
-0.876923076923076,-0.86153846153846,-0.846153846153845,-0.83076923076923,
-0.815384615384614,-0.799999999999999,-0.784615384615384,-0.769230769230768,
-0.753846153846153,-0.738461538461538,-0.723076923076922,-0.707692307692307,
-0.692307692307692,-0.676923076923076,-0.661538461538461,-0.646153846153846,
-0.63076923076923,-0.615384615384615,-0.6,-0.584615384615384,-0.569230769230769,
-0.553846153846154,-0.538461538461538,-0.523076923076923,-0.507692307692308,
-0.492307692307692,-0.476923076923077,-0.461538461538462,-0.446153846153846,
-0.430769230769231,-0.415384615384615,-0.4,-0.384615384615385,-0.369230769230769,
-0.353846153846154,-0.338461538461538,-0.323076923076923,-0.307692307692308,
-0.292307692307692,-0.276923076923077,-0.261538461538462,-0.246153846153846,
-0.230769230769231,-0.215384615384615,-0.2,-0.184615384615385,-0.169230769230769,
-0.153846153846154,-0.138461538461538,-0.123076923076923,-0.107692307692308,
-0.0923076923076923,-0.0769230769230769,-0.0615384615384615,-0.0461538461538462,
-0.0307692307692308,-0.0153846153846154,-0.00577184337450306),
 .UNSPECIFIED.)
CURVE()
GEOMETRIC_REPRESENTATION_ITEM()
RATIONAL_B_SPLINE_CURVE((1.,1.,1.,1.,1.,1.,1.,1.,1.,1.,1.,1.,1.,1.,1.,1.,
1.,1.,1.,1.,1.,1.,1.,1.,1.,1.,1.,1.,1.,1.,1.,1.,1.,1.,1.,1.,1.,1.,1.,1.,
1.,1.,1.,1.,1.,1.,1.,1.,1.,1.,1.,1.,1.,1.,1.,1.,1.,1.,1.,1.,1.,1.,1.,1.,
1.,1.,1.,1.,1.,1.))
REPRESENTATION_ITEM('')
);
#366=(
BOUNDED_CURVE()
B_SPLINE_CURVE(5,(#56683,#56684,#56685,#56686,#56687,#56688,#56689,#56690,
#56691,#56692,#56693,#56694,#56695,#56696,#56697,#56698,#56699,#56700,#56701,
#56702,#56703,#56704,#56705,#56706,#56707,#56708,#56709,#56710,#56711,#56712,
#56713,#56714,#56715,#56716,#56717,#56718,#56719,#56720,#56721,#56722,#56723,
#56724,#56725,#56726,#56727,#56728,#56729,#56730,#56731,#56732,#56733,#56734,
#56735,#56736,#56737,#56738,#56739,#56740,#56741,#56742,#56743,#56744,#56745,
#56746,#56747,#56748,#56749,#56750,#56751,#56752),.UNSPECIFIED.,.F.,.F.)
B_SPLINE_CURVE_WITH_KNOTS((6,1,1,1,1,1,1,1,1,1,1,1,1,1,1,1,1,1,1,1,1,1,
1,1,1,1,1,1,1,1,1,1,1,1,1,1,1,1,1,1,1,1,1,1,1,1,1,1,1,1,1,1,1,1,1,1,1,1,
1,1,1,1,1,1,1,6),(-0.994228156739675,-0.984615384615383,-0.969230769230768,
-0.953846153846152,-0.938461538461537,-0.923076923076922,-0.907692307692306,
-0.892307692307691,-0.876923076923076,-0.86153846153846,-0.846153846153845,
-0.83076923076923,-0.815384615384614,-0.799999999999999,-0.784615384615384,
-0.769230769230768,-0.753846153846153,-0.738461538461538,-0.723076923076922,
-0.707692307692307,-0.692307692307692,-0.676923076923076,-0.661538461538461,
-0.646153846153846,-0.63076923076923,-0.615384615384615,-0.6,-0.584615384615384,
-0.569230769230769,-0.553846153846154,-0.538461538461538,-0.523076923076923,
-0.507692307692308,-0.492307692307692,-0.476923076923077,-0.461538461538462,
-0.446153846153846,-0.430769230769231,-0.415384615384615,-0.4,-0.384615384615385,
-0.369230769230769,-0.353846153846154,-0.338461538461538,-0.323076923076923,
-0.307692307692308,-0.292307692307692,-0.276923076923077,-0.261538461538462,
-0.246153846153846,-0.230769230769231,-0.215384615384615,-0.2,-0.184615384615385,
-0.169230769230769,-0.153846153846154,-0.138461538461538,-0.123076923076923,
-0.107692307692308,-0.0923076923076923,-0.0769230769230769,-0.0615384615384615,
-0.0461538461538462,-0.0307692307692308,-0.0153846153846154,0.),
 .UNSPECIFIED.)
CURVE()
GEOMETRIC_REPRESENTATION_ITEM()
RATIONAL_B_SPLINE_CURVE((1.,1.,1.,1.,1.,1.,1.,1.,1.,1.,1.,1.,1.,1.,1.,1.,
1.,1.,1.,1.,1.,1.,1.,1.,1.,1.,1.,1.,1.,1.,1.,1.,1.,1.,1.,1.,1.,1.,1.,1.,
1.,1.,1.,1.,1.,1.,1.,1.,1.,1.,1.,1.,1.,1.,1.,1.,1.,1.,1.,1.,1.,1.,1.,1.,
1.,1.,1.,1.,1.,1.))
REPRESENTATION_ITEM('')
);
#367=(
BOUNDED_CURVE()
B_SPLINE_CURVE(5,(#56905,#56906,#56907,#56908,#56909,#56910,#56911,#56912,
#56913,#56914,#56915,#56916,#56917,#56918,#56919,#56920,#56921,#56922,#56923,
#56924,#56925,#56926,#56927,#56928,#56929,#56930,#56931,#56932,#56933,#56934,
#56935,#56936,#56937,#56938,#56939,#56940,#56941,#56942,#56943,#56944,#56945,
#56946,#56947,#56948,#56949,#56950,#56951,#56952,#56953,#56954,#56955,#56956,
#56957,#56958,#56959,#56960,#56961,#56962,#56963,#56964,#56965,#56966,#56967,
#56968,#56969,#56970,#56971,#56972,#56973,#56974),.UNSPECIFIED.,.F.,.F.)
B_SPLINE_CURVE_WITH_KNOTS((6,1,1,1,1,1,1,1,1,1,1,1,1,1,1,1,1,1,1,1,1,1,
1,1,1,1,1,1,1,1,1,1,1,1,1,1,1,1,1,1,1,1,1,1,1,1,1,1,1,1,1,1,1,1,1,1,1,1,
1,1,1,1,1,1,1,6),(-1.,-0.984615384615383,-0.969230769230768,-0.953846153846152,
-0.938461538461537,-0.923076923076922,-0.907692307692306,-0.892307692307691,
-0.876923076923076,-0.86153846153846,-0.846153846153845,-0.83076923076923,
-0.815384615384614,-0.799999999999999,-0.784615384615384,-0.769230769230768,
-0.753846153846153,-0.738461538461538,-0.723076923076922,-0.707692307692307,
-0.692307692307692,-0.676923076923076,-0.661538461538461,-0.646153846153846,
-0.63076923076923,-0.615384615384615,-0.6,-0.584615384615384,-0.569230769230769,
-0.553846153846154,-0.538461538461538,-0.523076923076923,-0.507692307692308,
-0.492307692307692,-0.476923076923077,-0.461538461538462,-0.446153846153846,
-0.430769230769231,-0.415384615384615,-0.4,-0.384615384615385,-0.369230769230769,
-0.353846153846154,-0.338461538461538,-0.323076923076923,-0.307692307692308,
-0.292307692307692,-0.276923076923077,-0.261538461538462,-0.246153846153846,
-0.230769230769231,-0.215384615384615,-0.2,-0.184615384615385,-0.169230769230769,
-0.153846153846154,-0.138461538461538,-0.123076923076923,-0.107692307692308,
-0.0923076923076923,-0.0769230769230769,-0.0615384615384615,-0.0461538461538462,
-0.0307692307692308,-0.0153846153846154,-0.00577184337450328),
 .UNSPECIFIED.)
CURVE()
GEOMETRIC_REPRESENTATION_ITEM()
RATIONAL_B_SPLINE_CURVE((1.,1.,1.,1.,1.,1.,1.,1.,1.,1.,1.,1.,1.,1.,1.,1.,
1.,1.,1.,1.,1.,1.,1.,1.,1.,1.,1.,1.,1.,1.,1.,1.,1.,1.,1.,1.,1.,1.,1.,1.,
1.,1.,1.,1.,1.,1.,1.,1.,1.,1.,1.,1.,1.,1.,1.,1.,1.,1.,1.,1.,1.,1.,1.,1.,
1.,1.,1.,1.,1.,1.))
REPRESENTATION_ITEM('')
);
#368=(
BOUNDED_CURVE()
B_SPLINE_CURVE(5,(#57127,#57128,#57129,#57130,#57131,#57132,#57133,#57134,
#57135,#57136,#57137,#57138,#57139,#57140,#57141,#57142,#57143,#57144,#57145,
#57146,#57147,#57148,#57149,#57150,#57151,#57152,#57153,#57154,#57155,#57156,
#57157,#57158,#57159,#57160,#57161,#57162,#57163,#57164,#57165,#57166,#57167,
#57168,#57169,#57170,#57171,#57172,#57173,#57174,#57175,#57176,#57177,#57178,
#57179,#57180,#57181,#57182,#57183,#57184,#57185,#57186,#57187,#57188,#57189,
#57190,#57191,#57192,#57193,#57194,#57195,#57196),.UNSPECIFIED.,.F.,.F.)
B_SPLINE_CURVE_WITH_KNOTS((6,1,1,1,1,1,1,1,1,1,1,1,1,1,1,1,1,1,1,1,1,1,
1,1,1,1,1,1,1,1,1,1,1,1,1,1,1,1,1,1,1,1,1,1,1,1,1,1,1,1,1,1,1,1,1,1,1,1,
1,1,1,1,1,1,1,6),(-0.994228156739672,-0.984615384615383,-0.969230769230768,
-0.953846153846152,-0.938461538461537,-0.923076923076922,-0.907692307692306,
-0.892307692307691,-0.876923076923076,-0.86153846153846,-0.846153846153845,
-0.83076923076923,-0.815384615384614,-0.799999999999999,-0.784615384615384,
-0.769230769230768,-0.753846153846153,-0.738461538461538,-0.723076923076922,
-0.707692307692307,-0.692307692307692,-0.676923076923076,-0.661538461538461,
-0.646153846153846,-0.63076923076923,-0.615384615384615,-0.6,-0.584615384615384,
-0.569230769230769,-0.553846153846154,-0.538461538461538,-0.523076923076923,
-0.507692307692308,-0.492307692307692,-0.476923076923077,-0.461538461538462,
-0.446153846153846,-0.430769230769231,-0.415384615384615,-0.4,-0.384615384615385,
-0.369230769230769,-0.353846153846154,-0.338461538461538,-0.323076923076923,
-0.307692307692308,-0.292307692307692,-0.276923076923077,-0.261538461538462,
-0.246153846153846,-0.230769230769231,-0.215384615384615,-0.2,-0.184615384615385,
-0.169230769230769,-0.153846153846154,-0.138461538461538,-0.123076923076923,
-0.107692307692308,-0.0923076923076923,-0.0769230769230769,-0.0615384615384615,
-0.0461538461538462,-0.0307692307692308,-0.0153846153846154,0.),
 .UNSPECIFIED.)
CURVE()
GEOMETRIC_REPRESENTATION_ITEM()
RATIONAL_B_SPLINE_CURVE((1.,1.,1.,1.,1.,1.,1.,1.,1.,1.,1.,1.,1.,1.,1.,1.,
1.,1.,1.,1.,1.,1.,1.,1.,1.,1.,1.,1.,1.,1.,1.,1.,1.,1.,1.,1.,1.,1.,1.,1.,
1.,1.,1.,1.,1.,1.,1.,1.,1.,1.,1.,1.,1.,1.,1.,1.,1.,1.,1.,1.,1.,1.,1.,1.,
1.,1.,1.,1.,1.,1.))
REPRESENTATION_ITEM('')
);
#369=(
BOUNDED_CURVE()
B_SPLINE_CURVE(5,(#57355,#57356,#57357,#57358,#57359,#57360,#57361,#57362,
#57363,#57364,#57365,#57366,#57367,#57368,#57369,#57370,#57371,#57372,#57373,
#57374,#57375,#57376,#57377,#57378,#57379,#57380,#57381,#57382,#57383,#57384,
#57385,#57386,#57387,#57388,#57389,#57390,#57391,#57392,#57393,#57394,#57395,
#57396,#57397,#57398,#57399,#57400,#57401,#57402,#57403,#57404,#57405,#57406,
#57407,#57408,#57409,#57410,#57411,#57412,#57413,#57414,#57415,#57416,#57417,
#57418,#57419,#57420,#57421,#57422,#57423,#57424),.UNSPECIFIED.,.F.,.F.)
B_SPLINE_CURVE_WITH_KNOTS((6,1,1,1,1,1,1,1,1,1,1,1,1,1,1,1,1,1,1,1,1,1,
1,1,1,1,1,1,1,1,1,1,1,1,1,1,1,1,1,1,1,1,1,1,1,1,1,1,1,1,1,1,1,1,1,1,1,1,
1,1,1,1,1,1,1,6),(-0.994228156739704,-0.984615384615383,-0.969230769230768,
-0.953846153846152,-0.938461538461537,-0.923076923076922,-0.907692307692306,
-0.892307692307691,-0.876923076923076,-0.86153846153846,-0.846153846153845,
-0.83076923076923,-0.815384615384614,-0.799999999999999,-0.784615384615384,
-0.769230769230768,-0.753846153846153,-0.738461538461538,-0.723076923076922,
-0.707692307692307,-0.692307692307692,-0.676923076923076,-0.661538461538461,
-0.646153846153846,-0.63076923076923,-0.615384615384615,-0.6,-0.584615384615384,
-0.569230769230769,-0.553846153846154,-0.538461538461538,-0.523076923076923,
-0.507692307692308,-0.492307692307692,-0.476923076923077,-0.461538461538462,
-0.446153846153846,-0.430769230769231,-0.415384615384615,-0.4,-0.384615384615385,
-0.369230769230769,-0.353846153846154,-0.338461538461538,-0.323076923076923,
-0.307692307692308,-0.292307692307692,-0.276923076923077,-0.261538461538462,
-0.246153846153846,-0.230769230769231,-0.215384615384615,-0.2,-0.184615384615385,
-0.169230769230769,-0.153846153846154,-0.138461538461538,-0.123076923076923,
-0.107692307692308,-0.0923076923076923,-0.0769230769230769,-0.0615384615384615,
-0.0461538461538462,-0.0307692307692308,-0.0153846153846154,0.),
 .UNSPECIFIED.)
CURVE()
GEOMETRIC_REPRESENTATION_ITEM()
RATIONAL_B_SPLINE_CURVE((1.,1.,1.,1.,1.,1.,1.,1.,1.,1.,1.,1.,1.,1.,1.,1.,
1.,1.,1.,1.,1.,1.,1.,1.,1.,1.,1.,1.,1.,1.,1.,1.,1.,1.,1.,1.,1.,1.,1.,1.,
1.,1.,1.,1.,1.,1.,1.,1.,1.,1.,1.,1.,1.,1.,1.,1.,1.,1.,1.,1.,1.,1.,1.,1.,
1.,1.,1.,1.,1.,1.))
REPRESENTATION_ITEM('')
);
#370=(
BOUNDED_CURVE()
B_SPLINE_CURVE(5,(#57566,#57567,#57568,#57569,#57570,#57571,#57572,#57573,
#57574,#57575,#57576,#57577,#57578,#57579,#57580,#57581,#57582,#57583,#57584,
#57585,#57586,#57587,#57588,#57589,#57590,#57591,#57592,#57593,#57594,#57595,
#57596,#57597,#57598,#57599,#57600,#57601,#57602,#57603,#57604,#57605,#57606,
#57607,#57608,#57609,#57610,#57611,#57612,#57613,#57614,#57615,#57616,#57617,
#57618,#57619,#57620,#57621,#57622,#57623,#57624,#57625,#57626,#57627,#57628,
#57629,#57630,#57631,#57632,#57633,#57634,#57635),.UNSPECIFIED.,.F.,.F.)
B_SPLINE_CURVE_WITH_KNOTS((6,1,1,1,1,1,1,1,1,1,1,1,1,1,1,1,1,1,1,1,1,1,
1,1,1,1,1,1,1,1,1,1,1,1,1,1,1,1,1,1,1,1,1,1,1,1,1,1,1,1,1,1,1,1,1,1,1,1,
1,1,1,1,1,1,1,6),(-1.,-0.984615384615383,-0.969230769230768,-0.953846153846152,
-0.938461538461537,-0.923076923076922,-0.907692307692306,-0.892307692307691,
-0.876923076923076,-0.86153846153846,-0.846153846153845,-0.83076923076923,
-0.815384615384614,-0.799999999999999,-0.784615384615384,-0.769230769230768,
-0.753846153846153,-0.738461538461538,-0.723076923076922,-0.707692307692307,
-0.692307692307692,-0.676923076923076,-0.661538461538461,-0.646153846153846,
-0.63076923076923,-0.615384615384615,-0.6,-0.584615384615384,-0.569230769230769,
-0.553846153846154,-0.538461538461538,-0.523076923076923,-0.507692307692308,
-0.492307692307692,-0.476923076923077,-0.461538461538462,-0.446153846153846,
-0.430769230769231,-0.415384615384615,-0.4,-0.384615384615385,-0.369230769230769,
-0.353846153846154,-0.338461538461538,-0.323076923076923,-0.307692307692308,
-0.292307692307692,-0.276923076923077,-0.261538461538462,-0.246153846153846,
-0.230769230769231,-0.215384615384615,-0.2,-0.184615384615385,-0.169230769230769,
-0.153846153846154,-0.138461538461538,-0.123076923076923,-0.107692307692308,
-0.0923076923076923,-0.0769230769230769,-0.0615384615384615,-0.0461538461538462,
-0.0307692307692308,-0.0153846153846154,-0.00577184337451611),
 .UNSPECIFIED.)
CURVE()
GEOMETRIC_REPRESENTATION_ITEM()
RATIONAL_B_SPLINE_CURVE((1.,1.,1.,1.,1.,1.,1.,1.,1.,1.,1.,1.,1.,1.,1.,1.,
1.,1.,1.,1.,1.,1.,1.,1.,1.,1.,1.,1.,1.,1.,1.,1.,1.,1.,1.,1.,1.,1.,1.,1.,
1.,1.,1.,1.,1.,1.,1.,1.,1.,1.,1.,1.,1.,1.,1.,1.,1.,1.,1.,1.,1.,1.,1.,1.,
1.,1.,1.,1.,1.,1.))
REPRESENTATION_ITEM('')
);
#836=B_SPLINE_CURVE_WITH_KNOTS('',3,(#40102,#40103,#40104,#40105,#40106,
#40107),.UNSPECIFIED.,.F.,.F.,(4,2,4),(0.,1.,2.),.UNSPECIFIED.);
#837=B_SPLINE_CURVE_WITH_KNOTS('',3,(#40321,#40322,#40323,#40324,#40325,
#40326),.UNSPECIFIED.,.F.,.F.,(4,2,4),(0.,1.,2.),.UNSPECIFIED.);
#838=B_SPLINE_CURVE_WITH_KNOTS('',3,(#40404,#40405,#40406,#40407,#40408,
#40409),.UNSPECIFIED.,.F.,.F.,(4,2,4),(0.,1.,2.),.UNSPECIFIED.);
#839=B_SPLINE_CURVE_WITH_KNOTS('',3,(#40763,#40764,#40765,#40766,#40767,
#40768),.UNSPECIFIED.,.F.,.F.,(4,2,4),(0.,1.,2.),.UNSPECIFIED.);
#840=B_SPLINE_CURVE_WITH_KNOTS('',3,(#40846,#40847,#40848,#40849,#40850,
#40851),.UNSPECIFIED.,.F.,.F.,(4,2,4),(0.,1.,2.),.UNSPECIFIED.);
#841=B_SPLINE_CURVE_WITH_KNOTS('',3,(#41205,#41206,#41207,#41208,#41209,
#41210),.UNSPECIFIED.,.F.,.F.,(4,2,4),(0.,1.,2.),.UNSPECIFIED.);
#842=B_SPLINE_CURVE_WITH_KNOTS('',3,(#41288,#41289,#41290,#41291,#41292,
#41293),.UNSPECIFIED.,.F.,.F.,(4,2,4),(0.,1.,2.),.UNSPECIFIED.);
#843=B_SPLINE_CURVE_WITH_KNOTS('',3,(#41647,#41648,#41649,#41650,#41651,
#41652),.UNSPECIFIED.,.F.,.F.,(4,2,4),(0.,1.,2.),.UNSPECIFIED.);
#844=B_SPLINE_CURVE_WITH_KNOTS('',3,(#41730,#41731,#41732,#41733,#41734,
#41735),.UNSPECIFIED.,.F.,.F.,(4,2,4),(0.,1.,2.),.UNSPECIFIED.);
#845=B_SPLINE_CURVE_WITH_KNOTS('',3,(#42089,#42090,#42091,#42092,#42093,
#42094),.UNSPECIFIED.,.F.,.F.,(4,2,4),(0.,1.,2.),.UNSPECIFIED.);
#846=B_SPLINE_CURVE_WITH_KNOTS('',3,(#42172,#42173,#42174,#42175,#42176,
#42177),.UNSPECIFIED.,.F.,.F.,(4,2,4),(0.,1.,2.),.UNSPECIFIED.);
#847=B_SPLINE_CURVE_WITH_KNOTS('',3,(#42531,#42532,#42533,#42534,#42535,
#42536),.UNSPECIFIED.,.F.,.F.,(4,2,4),(0.,1.,2.),.UNSPECIFIED.);
#848=B_SPLINE_CURVE_WITH_KNOTS('',3,(#42614,#42615,#42616,#42617,#42618,
#42619),.UNSPECIFIED.,.F.,.F.,(4,2,4),(0.,1.,2.),.UNSPECIFIED.);
#849=B_SPLINE_CURVE_WITH_KNOTS('',3,(#42973,#42974,#42975,#42976,#42977,
#42978),.UNSPECIFIED.,.F.,.F.,(4,2,4),(0.,1.,2.),.UNSPECIFIED.);
#850=B_SPLINE_CURVE_WITH_KNOTS('',3,(#43056,#43057,#43058,#43059,#43060,
#43061),.UNSPECIFIED.,.F.,.F.,(4,2,4),(0.,1.,2.),.UNSPECIFIED.);
#851=B_SPLINE_CURVE_WITH_KNOTS('',3,(#43415,#43416,#43417,#43418,#43419,
#43420),.UNSPECIFIED.,.F.,.F.,(4,2,4),(0.,1.,2.),.UNSPECIFIED.);
#852=B_SPLINE_CURVE_WITH_KNOTS('',3,(#43498,#43499,#43500,#43501,#43502,
#43503),.UNSPECIFIED.,.F.,.F.,(4,2,4),(0.,1.,2.),.UNSPECIFIED.);
#853=B_SPLINE_CURVE_WITH_KNOTS('',3,(#43857,#43858,#43859,#43860,#43861,
#43862),.UNSPECIFIED.,.F.,.F.,(4,2,4),(0.,1.,2.),.UNSPECIFIED.);
#854=B_SPLINE_CURVE_WITH_KNOTS('',3,(#43940,#43941,#43942,#43943,#43944,
#43945),.UNSPECIFIED.,.F.,.F.,(4,2,4),(0.,1.,2.),.UNSPECIFIED.);
#855=B_SPLINE_CURVE_WITH_KNOTS('',3,(#44299,#44300,#44301,#44302,#44303,
#44304),.UNSPECIFIED.,.F.,.F.,(4,2,4),(0.,1.,2.),.UNSPECIFIED.);
#856=B_SPLINE_CURVE_WITH_KNOTS('',3,(#44382,#44383,#44384,#44385,#44386,
#44387),.UNSPECIFIED.,.F.,.F.,(4,2,4),(0.,1.,2.),.UNSPECIFIED.);
#857=B_SPLINE_CURVE_WITH_KNOTS('',3,(#44741,#44742,#44743,#44744,#44745,
#44746),.UNSPECIFIED.,.F.,.F.,(4,2,4),(0.,1.,2.),.UNSPECIFIED.);
#858=B_SPLINE_CURVE_WITH_KNOTS('',3,(#44824,#44825,#44826,#44827,#44828,
#44829),.UNSPECIFIED.,.F.,.F.,(4,2,4),(0.,1.,2.),.UNSPECIFIED.);
#859=B_SPLINE_CURVE_WITH_KNOTS('',3,(#45183,#45184,#45185,#45186,#45187,
#45188),.UNSPECIFIED.,.F.,.F.,(4,2,4),(0.,1.,2.),.UNSPECIFIED.);
#860=B_SPLINE_CURVE_WITH_KNOTS('',3,(#45266,#45267,#45268,#45269,#45270,
#45271),.UNSPECIFIED.,.F.,.F.,(4,2,4),(0.,1.,2.),.UNSPECIFIED.);
#861=B_SPLINE_CURVE_WITH_KNOTS('',3,(#45625,#45626,#45627,#45628,#45629,
#45630),.UNSPECIFIED.,.F.,.F.,(4,2,4),(0.,1.,2.),.UNSPECIFIED.);
#862=B_SPLINE_CURVE_WITH_KNOTS('',3,(#45708,#45709,#45710,#45711,#45712,
#45713),.UNSPECIFIED.,.F.,.F.,(4,2,4),(0.,1.,2.),.UNSPECIFIED.);
#863=B_SPLINE_CURVE_WITH_KNOTS('',3,(#46067,#46068,#46069,#46070,#46071,
#46072),.UNSPECIFIED.,.F.,.F.,(4,2,4),(0.,1.,2.),.UNSPECIFIED.);
#864=B_SPLINE_CURVE_WITH_KNOTS('',3,(#46150,#46151,#46152,#46153,#46154,
#46155),.UNSPECIFIED.,.F.,.F.,(4,2,4),(0.,1.,2.),.UNSPECIFIED.);
#865=B_SPLINE_CURVE_WITH_KNOTS('',3,(#46509,#46510,#46511,#46512,#46513,
#46514),.UNSPECIFIED.,.F.,.F.,(4,2,4),(0.,1.,2.),.UNSPECIFIED.);
#866=B_SPLINE_CURVE_WITH_KNOTS('',3,(#46592,#46593,#46594,#46595,#46596,
#46597),.UNSPECIFIED.,.F.,.F.,(4,2,4),(0.,1.,2.),.UNSPECIFIED.);
#867=B_SPLINE_CURVE_WITH_KNOTS('',3,(#46951,#46952,#46953,#46954,#46955,
#46956),.UNSPECIFIED.,.F.,.F.,(4,2,4),(0.,1.,2.),.UNSPECIFIED.);
#868=B_SPLINE_CURVE_WITH_KNOTS('',3,(#47034,#47035,#47036,#47037,#47038,
#47039),.UNSPECIFIED.,.F.,.F.,(4,2,4),(0.,1.,2.),.UNSPECIFIED.);
#869=B_SPLINE_CURVE_WITH_KNOTS('',3,(#47393,#47394,#47395,#47396,#47397,
#47398),.UNSPECIFIED.,.F.,.F.,(4,2,4),(0.,1.,2.),.UNSPECIFIED.);
#870=B_SPLINE_CURVE_WITH_KNOTS('',3,(#47476,#47477,#47478,#47479,#47480,
#47481),.UNSPECIFIED.,.F.,.F.,(4,2,4),(0.,1.,2.),.UNSPECIFIED.);
#871=B_SPLINE_CURVE_WITH_KNOTS('',3,(#47835,#47836,#47837,#47838,#47839,
#47840),.UNSPECIFIED.,.F.,.F.,(4,2,4),(0.,1.,2.),.UNSPECIFIED.);
#872=B_SPLINE_CURVE_WITH_KNOTS('',3,(#47918,#47919,#47920,#47921,#47922,
#47923),.UNSPECIFIED.,.F.,.F.,(4,2,4),(0.,1.,2.),.UNSPECIFIED.);
#873=B_SPLINE_CURVE_WITH_KNOTS('',3,(#48277,#48278,#48279,#48280,#48281,
#48282),.UNSPECIFIED.,.F.,.F.,(4,2,4),(0.,1.,2.),.UNSPECIFIED.);
#874=B_SPLINE_CURVE_WITH_KNOTS('',3,(#48360,#48361,#48362,#48363,#48364,
#48365),.UNSPECIFIED.,.F.,.F.,(4,2,4),(0.,1.,2.),.UNSPECIFIED.);
#875=B_SPLINE_CURVE_WITH_KNOTS('',3,(#48719,#48720,#48721,#48722,#48723,
#48724),.UNSPECIFIED.,.F.,.F.,(4,2,4),(0.,1.,2.),.UNSPECIFIED.);
#876=B_SPLINE_CURVE_WITH_KNOTS('',3,(#48802,#48803,#48804,#48805,#48806,
#48807),.UNSPECIFIED.,.F.,.F.,(4,2,4),(0.,1.,2.),.UNSPECIFIED.);
#877=B_SPLINE_CURVE_WITH_KNOTS('',3,(#49161,#49162,#49163,#49164,#49165,
#49166),.UNSPECIFIED.,.F.,.F.,(4,2,4),(0.,1.,2.),.UNSPECIFIED.);
#878=B_SPLINE_CURVE_WITH_KNOTS('',3,(#49244,#49245,#49246,#49247,#49248,
#49249),.UNSPECIFIED.,.F.,.F.,(4,2,4),(0.,1.,2.),.UNSPECIFIED.);
#879=B_SPLINE_CURVE_WITH_KNOTS('',3,(#49603,#49604,#49605,#49606,#49607,
#49608),.UNSPECIFIED.,.F.,.F.,(4,2,4),(0.,1.,2.),.UNSPECIFIED.);
#880=B_SPLINE_CURVE_WITH_KNOTS('',3,(#49686,#49687,#49688,#49689,#49690,
#49691),.UNSPECIFIED.,.F.,.F.,(4,2,4),(0.,1.,2.),.UNSPECIFIED.);
#881=B_SPLINE_CURVE_WITH_KNOTS('',3,(#50045,#50046,#50047,#50048,#50049,
#50050),.UNSPECIFIED.,.F.,.F.,(4,2,4),(0.,1.,2.),.UNSPECIFIED.);
#882=B_SPLINE_CURVE_WITH_KNOTS('',3,(#50128,#50129,#50130,#50131,#50132,
#50133),.UNSPECIFIED.,.F.,.F.,(4,2,4),(0.,1.,2.),.UNSPECIFIED.);
#883=B_SPLINE_CURVE_WITH_KNOTS('',3,(#50487,#50488,#50489,#50490,#50491,
#50492),.UNSPECIFIED.,.F.,.F.,(4,2,4),(0.,1.,2.),.UNSPECIFIED.);
#884=B_SPLINE_CURVE_WITH_KNOTS('',3,(#50570,#50571,#50572,#50573,#50574,
#50575),.UNSPECIFIED.,.F.,.F.,(4,2,4),(0.,1.,2.),.UNSPECIFIED.);
#885=B_SPLINE_CURVE_WITH_KNOTS('',3,(#50929,#50930,#50931,#50932,#50933,
#50934),.UNSPECIFIED.,.F.,.F.,(4,2,4),(0.,1.,2.),.UNSPECIFIED.);
#886=B_SPLINE_CURVE_WITH_KNOTS('',3,(#51012,#51013,#51014,#51015,#51016,
#51017),.UNSPECIFIED.,.F.,.F.,(4,2,4),(0.,1.,2.),.UNSPECIFIED.);
#887=B_SPLINE_CURVE_WITH_KNOTS('',3,(#51371,#51372,#51373,#51374,#51375,
#51376),.UNSPECIFIED.,.F.,.F.,(4,2,4),(0.,1.,2.),.UNSPECIFIED.);
#888=B_SPLINE_CURVE_WITH_KNOTS('',3,(#51454,#51455,#51456,#51457,#51458,
#51459),.UNSPECIFIED.,.F.,.F.,(4,2,4),(0.,1.,2.),.UNSPECIFIED.);
#889=B_SPLINE_CURVE_WITH_KNOTS('',3,(#51813,#51814,#51815,#51816,#51817,
#51818),.UNSPECIFIED.,.F.,.F.,(4,2,4),(0.,1.,2.),.UNSPECIFIED.);
#890=B_SPLINE_CURVE_WITH_KNOTS('',3,(#51896,#51897,#51898,#51899,#51900,
#51901),.UNSPECIFIED.,.F.,.F.,(4,2,4),(0.,1.,2.),.UNSPECIFIED.);
#891=B_SPLINE_CURVE_WITH_KNOTS('',3,(#52255,#52256,#52257,#52258,#52259,
#52260),.UNSPECIFIED.,.F.,.F.,(4,2,4),(0.,1.,2.),.UNSPECIFIED.);
#892=B_SPLINE_CURVE_WITH_KNOTS('',3,(#52338,#52339,#52340,#52341,#52342,
#52343),.UNSPECIFIED.,.F.,.F.,(4,2,4),(0.,1.,2.),.UNSPECIFIED.);
#893=B_SPLINE_CURVE_WITH_KNOTS('',3,(#52697,#52698,#52699,#52700,#52701,
#52702),.UNSPECIFIED.,.F.,.F.,(4,2,4),(0.,1.,2.),.UNSPECIFIED.);
#894=B_SPLINE_CURVE_WITH_KNOTS('',3,(#52780,#52781,#52782,#52783,#52784,
#52785),.UNSPECIFIED.,.F.,.F.,(4,2,4),(0.,1.,2.),.UNSPECIFIED.);
#895=B_SPLINE_CURVE_WITH_KNOTS('',3,(#53139,#53140,#53141,#53142,#53143,
#53144),.UNSPECIFIED.,.F.,.F.,(4,2,4),(0.,1.,2.),.UNSPECIFIED.);
#896=B_SPLINE_CURVE_WITH_KNOTS('',3,(#53222,#53223,#53224,#53225,#53226,
#53227),.UNSPECIFIED.,.F.,.F.,(4,2,4),(0.,1.,2.),.UNSPECIFIED.);
#897=B_SPLINE_CURVE_WITH_KNOTS('',3,(#53581,#53582,#53583,#53584,#53585,
#53586),.UNSPECIFIED.,.F.,.F.,(4,2,4),(0.,1.,2.),.UNSPECIFIED.);
#898=B_SPLINE_CURVE_WITH_KNOTS('',3,(#53664,#53665,#53666,#53667,#53668,
#53669),.UNSPECIFIED.,.F.,.F.,(4,2,4),(0.,1.,2.),.UNSPECIFIED.);
#899=B_SPLINE_CURVE_WITH_KNOTS('',3,(#54023,#54024,#54025,#54026,#54027,
#54028),.UNSPECIFIED.,.F.,.F.,(4,2,4),(0.,1.,2.),.UNSPECIFIED.);
#900=B_SPLINE_CURVE_WITH_KNOTS('',3,(#54106,#54107,#54108,#54109,#54110,
#54111),.UNSPECIFIED.,.F.,.F.,(4,2,4),(0.,1.,2.),.UNSPECIFIED.);
#901=B_SPLINE_CURVE_WITH_KNOTS('',3,(#54465,#54466,#54467,#54468,#54469,
#54470),.UNSPECIFIED.,.F.,.F.,(4,2,4),(0.,1.,2.),.UNSPECIFIED.);
#902=B_SPLINE_CURVE_WITH_KNOTS('',3,(#54548,#54549,#54550,#54551,#54552,
#54553),.UNSPECIFIED.,.F.,.F.,(4,2,4),(0.,1.,2.),.UNSPECIFIED.);
#903=B_SPLINE_CURVE_WITH_KNOTS('',3,(#54907,#54908,#54909,#54910,#54911,
#54912),.UNSPECIFIED.,.F.,.F.,(4,2,4),(0.,1.,2.),.UNSPECIFIED.);
#904=B_SPLINE_CURVE_WITH_KNOTS('',3,(#54990,#54991,#54992,#54993,#54994,
#54995),.UNSPECIFIED.,.F.,.F.,(4,2,4),(0.,1.,2.),.UNSPECIFIED.);
#905=B_SPLINE_CURVE_WITH_KNOTS('',3,(#55349,#55350,#55351,#55352,#55353,
#55354),.UNSPECIFIED.,.F.,.F.,(4,2,4),(0.,1.,2.),.UNSPECIFIED.);
#906=B_SPLINE_CURVE_WITH_KNOTS('',3,(#55432,#55433,#55434,#55435,#55436,
#55437),.UNSPECIFIED.,.F.,.F.,(4,2,4),(0.,1.,2.),.UNSPECIFIED.);
#907=B_SPLINE_CURVE_WITH_KNOTS('',3,(#55791,#55792,#55793,#55794,#55795,
#55796),.UNSPECIFIED.,.F.,.F.,(4,2,4),(0.,1.,2.),.UNSPECIFIED.);
#908=B_SPLINE_CURVE_WITH_KNOTS('',3,(#55874,#55875,#55876,#55877,#55878,
#55879),.UNSPECIFIED.,.F.,.F.,(4,2,4),(0.,1.,2.),.UNSPECIFIED.);
#909=B_SPLINE_CURVE_WITH_KNOTS('',3,(#56233,#56234,#56235,#56236,#56237,
#56238),.UNSPECIFIED.,.F.,.F.,(4,2,4),(0.,1.,2.),.UNSPECIFIED.);
#910=B_SPLINE_CURVE_WITH_KNOTS('',3,(#56316,#56317,#56318,#56319,#56320,
#56321),.UNSPECIFIED.,.F.,.F.,(4,2,4),(0.,1.,2.),.UNSPECIFIED.);
#911=B_SPLINE_CURVE_WITH_KNOTS('',3,(#56675,#56676,#56677,#56678,#56679,
#56680),.UNSPECIFIED.,.F.,.F.,(4,2,4),(0.,1.,2.),.UNSPECIFIED.);
#912=B_SPLINE_CURVE_WITH_KNOTS('',3,(#56758,#56759,#56760,#56761,#56762,
#56763),.UNSPECIFIED.,.F.,.F.,(4,2,4),(0.,1.,2.),.UNSPECIFIED.);
#913=B_SPLINE_CURVE_WITH_KNOTS('',3,(#57121,#57122,#57123,#57124,#57125,
#57126),.UNSPECIFIED.,.F.,.F.,(4,2,4),(0.,1.,2.),.UNSPECIFIED.);
#914=B_SPLINE_CURVE_WITH_KNOTS('',3,(#57200,#57201,#57202,#57203,#57204,
#57205),.UNSPECIFIED.,.F.,.F.,(4,2,4),(0.,1.,2.),.UNSPECIFIED.);
#915=B_SPLINE_CURVE_WITH_KNOTS('',3,(#57347,#57348,#57349,#57350,#57351,
#57352),.UNSPECIFIED.,.F.,.F.,(4,2,4),(0.,1.,2.),.UNSPECIFIED.);
#964=SHAPE_REPRESENTATION_RELATIONSHIP('SRR','None',#58165,#1014);
#1014=ADVANCED_BREP_SHAPE_REPRESENTATION('',(#1142),#57898);
#1079=STYLED_ITEM('',(#58458),#1142);
#1142=MANIFOLD_SOLID_BREP('Body1',#13641);
#1326=FACE_BOUND('',#3227,.T.);
#1327=FACE_BOUND('',#3231,.T.);
#1328=FACE_BOUND('',#3392,.T.);
#1637=PLANE('',#15307);
#1638=PLANE('',#15308);
#1639=PLANE('',#15309);
#1640=PLANE('',#15310);
#1641=PLANE('',#15357);
#1642=PLANE('',#15358);
#1643=PLANE('',#15361);
#1644=PLANE('',#15364);
#1645=PLANE('',#15367);
#1646=PLANE('',#15370);
#1647=PLANE('',#15373);
#1648=PLANE('',#15376);
#1649=PLANE('',#15379);
#1650=PLANE('',#15382);
#1651=PLANE('',#15385);
#1652=PLANE('',#15388);
#1653=PLANE('',#15391);
#1654=PLANE('',#15394);
#1655=PLANE('',#15397);
#1656=PLANE('',#15400);
#1657=PLANE('',#15403);
#1658=PLANE('',#15406);
#1659=PLANE('',#15409);
#1660=PLANE('',#15412);
#1661=PLANE('',#15415);
#1662=PLANE('',#15418);
#1663=PLANE('',#15421);
#1664=PLANE('',#15424);
#1665=PLANE('',#15427);
#1666=PLANE('',#15430);
#1667=PLANE('',#15433);
#1668=PLANE('',#15436);
#1669=PLANE('',#15439);
#1670=PLANE('',#15442);
#1671=PLANE('',#15445);
#1672=PLANE('',#15448);
#1673=PLANE('',#15451);
#1674=PLANE('',#15454);
#1675=PLANE('',#15457);
#1676=PLANE('',#15460);
#1677=PLANE('',#15463);
#1678=PLANE('',#15466);
#1679=PLANE('',#15469);
#1680=PLANE('',#15472);
#1681=PLANE('',#15475);
#1682=PLANE('',#15476);
#2275=FACE_OUTER_BOUND('',#3223,.T.);
#2276=FACE_OUTER_BOUND('',#3224,.T.);
#2277=FACE_OUTER_BOUND('',#3225,.T.);
#2278=FACE_OUTER_BOUND('',#3226,.T.);
#2279=FACE_OUTER_BOUND('',#3228,.T.);
#2280=FACE_OUTER_BOUND('',#3229,.T.);
#2281=FACE_OUTER_BOUND('',#3230,.T.);
#2282=FACE_OUTER_BOUND('',#3232,.T.);
#2283=FACE_OUTER_BOUND('',#3233,.T.);
#2284=FACE_OUTER_BOUND('',#3234,.T.);
#2285=FACE_OUTER_BOUND('',#3235,.T.);
#2286=FACE_OUTER_BOUND('',#3236,.T.);
#2287=FACE_OUTER_BOUND('',#3237,.T.);
#2288=FACE_OUTER_BOUND('',#3238,.T.);
#2289=FACE_OUTER_BOUND('',#3239,.T.);
#2290=FACE_OUTER_BOUND('',#3240,.T.);
#2291=FACE_OUTER_BOUND('',#3241,.T.);
#2292=FACE_OUTER_BOUND('',#3242,.T.);
#2293=FACE_OUTER_BOUND('',#3243,.T.);
#2294=FACE_OUTER_BOUND('',#3244,.T.);
#2295=FACE_OUTER_BOUND('',#3245,.T.);
#2296=FACE_OUTER_BOUND('',#3246,.T.);
#2297=FACE_OUTER_BOUND('',#3247,.T.);
#2298=FACE_OUTER_BOUND('',#3248,.T.);
#2299=FACE_OUTER_BOUND('',#3249,.T.);
#2300=FACE_OUTER_BOUND('',#3250,.T.);
#2301=FACE_OUTER_BOUND('',#3251,.T.);
#2302=FACE_OUTER_BOUND('',#3252,.T.);
#2303=FACE_OUTER_BOUND('',#3253,.T.);
#2304=FACE_OUTER_BOUND('',#3254,.T.);
#2305=FACE_OUTER_BOUND('',#3255,.T.);
#2306=FACE_OUTER_BOUND('',#3256,.T.);
#2307=FACE_OUTER_BOUND('',#3257,.T.);
#2308=FACE_OUTER_BOUND('',#3258,.T.);
#2309=FACE_OUTER_BOUND('',#3259,.T.);
#2310=FACE_OUTER_BOUND('',#3260,.T.);
#2311=FACE_OUTER_BOUND('',#3261,.T.);
#2312=FACE_OUTER_BOUND('',#3262,.T.);
#2313=FACE_OUTER_BOUND('',#3263,.T.);
#2314=FACE_OUTER_BOUND('',#3264,.T.);
#2315=FACE_OUTER_BOUND('',#3265,.T.);
#2316=FACE_OUTER_BOUND('',#3266,.T.);
#2317=FACE_OUTER_BOUND('',#3267,.T.);
#2318=FACE_OUTER_BOUND('',#3268,.T.);
#2319=FACE_OUTER_BOUND('',#3269,.T.);
#2320=FACE_OUTER_BOUND('',#3270,.T.);
#2321=FACE_OUTER_BOUND('',#3271,.T.);
#2322=FACE_OUTER_BOUND('',#3272,.T.);
#2323=FACE_OUTER_BOUND('',#3273,.T.);
#2324=FACE_OUTER_BOUND('',#3274,.T.);
#2325=FACE_OUTER_BOUND('',#3275,.T.);
#2326=FACE_OUTER_BOUND('',#3276,.T.);
#2327=FACE_OUTER_BOUND('',#3277,.T.);
#2328=FACE_OUTER_BOUND('',#3278,.T.);
#2329=FACE_OUTER_BOUND('',#3279,.T.);
#2330=FACE_OUTER_BOUND('',#3280,.T.);
#2331=FACE_OUTER_BOUND('',#3281,.T.);
#2332=FACE_OUTER_BOUND('',#3282,.T.);
#2333=FACE_OUTER_BOUND('',#3283,.T.);
#2334=FACE_OUTER_BOUND('',#3284,.T.);
#2335=FACE_OUTER_BOUND('',#3285,.T.);
#2336=FACE_OUTER_BOUND('',#3286,.T.);
#2337=FACE_OUTER_BOUND('',#3287,.T.);
#2338=FACE_OUTER_BOUND('',#3288,.T.);
#2339=FACE_OUTER_BOUND('',#3289,.T.);
#2340=FACE_OUTER_BOUND('',#3290,.T.);
#2341=FACE_OUTER_BOUND('',#3291,.T.);
#2342=FACE_OUTER_BOUND('',#3292,.T.);
#2343=FACE_OUTER_BOUND('',#3293,.T.);
#2344=FACE_OUTER_BOUND('',#3294,.T.);
#2345=FACE_OUTER_BOUND('',#3295,.T.);
#2346=FACE_OUTER_BOUND('',#3296,.T.);
#2347=FACE_OUTER_BOUND('',#3297,.T.);
#2348=FACE_OUTER_BOUND('',#3298,.T.);
#2349=FACE_OUTER_BOUND('',#3299,.T.);
#2350=FACE_OUTER_BOUND('',#3300,.T.);
#2351=FACE_OUTER_BOUND('',#3301,.T.);
#2352=FACE_OUTER_BOUND('',#3302,.T.);
#2353=FACE_OUTER_BOUND('',#3303,.T.);
#2354=FACE_OUTER_BOUND('',#3304,.T.);
#2355=FACE_OUTER_BOUND('',#3305,.T.);
#2356=FACE_OUTER_BOUND('',#3306,.T.);
#2357=FACE_OUTER_BOUND('',#3307,.T.);
#2358=FACE_OUTER_BOUND('',#3308,.T.);
#2359=FACE_OUTER_BOUND('',#3309,.T.);
#2360=FACE_OUTER_BOUND('',#3310,.T.);
#2361=FACE_OUTER_BOUND('',#3311,.T.);
#2362=FACE_OUTER_BOUND('',#3312,.T.);
#2363=FACE_OUTER_BOUND('',#3313,.T.);
#2364=FACE_OUTER_BOUND('',#3314,.T.);
#2365=FACE_OUTER_BOUND('',#3315,.T.);
#2366=FACE_OUTER_BOUND('',#3316,.T.);
#2367=FACE_OUTER_BOUND('',#3317,.T.);
#2368=FACE_OUTER_BOUND('',#3318,.T.);
#2369=FACE_OUTER_BOUND('',#3319,.T.);
#2370=FACE_OUTER_BOUND('',#3320,.T.);
#2371=FACE_OUTER_BOUND('',#3321,.T.);
#2372=FACE_OUTER_BOUND('',#3322,.T.);
#2373=FACE_OUTER_BOUND('',#3323,.T.);
#2374=FACE_OUTER_BOUND('',#3324,.T.);
#2375=FACE_OUTER_BOUND('',#3325,.T.);
#2376=FACE_OUTER_BOUND('',#3326,.T.);
#2377=FACE_OUTER_BOUND('',#3327,.T.);
#2378=FACE_OUTER_BOUND('',#3328,.T.);
#2379=FACE_OUTER_BOUND('',#3329,.T.);
#2380=FACE_OUTER_BOUND('',#3330,.T.);
#2381=FACE_OUTER_BOUND('',#3331,.T.);
#2382=FACE_OUTER_BOUND('',#3332,.T.);
#2383=FACE_OUTER_BOUND('',#3333,.T.);
#2384=FACE_OUTER_BOUND('',#3334,.T.);
#2385=FACE_OUTER_BOUND('',#3335,.T.);
#2386=FACE_OUTER_BOUND('',#3336,.T.);
#2387=FACE_OUTER_BOUND('',#3337,.T.);
#2388=FACE_OUTER_BOUND('',#3338,.T.);
#2389=FACE_OUTER_BOUND('',#3339,.T.);
#2390=FACE_OUTER_BOUND('',#3340,.T.);
#2391=FACE_OUTER_BOUND('',#3341,.T.);
#2392=FACE_OUTER_BOUND('',#3342,.T.);
#2393=FACE_OUTER_BOUND('',#3343,.T.);
#2394=FACE_OUTER_BOUND('',#3344,.T.);
#2395=FACE_OUTER_BOUND('',#3345,.T.);
#2396=FACE_OUTER_BOUND('',#3346,.T.);
#2397=FACE_OUTER_BOUND('',#3347,.T.);
#2398=FACE_OUTER_BOUND('',#3348,.T.);
#2399=FACE_OUTER_BOUND('',#3349,.T.);
#2400=FACE_OUTER_BOUND('',#3350,.T.);
#2401=FACE_OUTER_BOUND('',#3351,.T.);
#2402=FACE_OUTER_BOUND('',#3352,.T.);
#2403=FACE_OUTER_BOUND('',#3353,.T.);
#2404=FACE_OUTER_BOUND('',#3354,.T.);
#2405=FACE_OUTER_BOUND('',#3355,.T.);
#2406=FACE_OUTER_BOUND('',#3356,.T.);
#2407=FACE_OUTER_BOUND('',#3357,.T.);
#2408=FACE_OUTER_BOUND('',#3358,.T.);
#2409=FACE_OUTER_BOUND('',#3359,.T.);
#2410=FACE_OUTER_BOUND('',#3360,.T.);
#2411=FACE_OUTER_BOUND('',#3361,.T.);
#2412=FACE_OUTER_BOUND('',#3362,.T.);
#2413=FACE_OUTER_BOUND('',#3363,.T.);
#2414=FACE_OUTER_BOUND('',#3364,.T.);
#2415=FACE_OUTER_BOUND('',#3365,.T.);
#2416=FACE_OUTER_BOUND('',#3366,.T.);
#2417=FACE_OUTER_BOUND('',#3367,.T.);
#2418=FACE_OUTER_BOUND('',#3368,.T.);
#2419=FACE_OUTER_BOUND('',#3369,.T.);
#2420=FACE_OUTER_BOUND('',#3370,.T.);
#2421=FACE_OUTER_BOUND('',#3371,.T.);
#2422=FACE_OUTER_BOUND('',#3372,.T.);
#2423=FACE_OUTER_BOUND('',#3373,.T.);
#2424=FACE_OUTER_BOUND('',#3374,.T.);
#2425=FACE_OUTER_BOUND('',#3375,.T.);
#2426=FACE_OUTER_BOUND('',#3376,.T.);
#2427=FACE_OUTER_BOUND('',#3377,.T.);
#2428=FACE_OUTER_BOUND('',#3378,.T.);
#2429=FACE_OUTER_BOUND('',#3379,.T.);
#2430=FACE_OUTER_BOUND('',#3380,.T.);
#2431=FACE_OUTER_BOUND('',#3381,.T.);
#2432=FACE_OUTER_BOUND('',#3382,.T.);
#2433=FACE_OUTER_BOUND('',#3383,.T.);
#2434=FACE_OUTER_BOUND('',#3384,.T.);
#2435=FACE_OUTER_BOUND('',#3385,.T.);
#2436=FACE_OUTER_BOUND('',#3386,.T.);
#2437=FACE_OUTER_BOUND('',#3387,.T.);
#2438=FACE_OUTER_BOUND('',#3388,.T.);
#2439=FACE_OUTER_BOUND('',#3389,.T.);
#2440=FACE_OUTER_BOUND('',#3390,.T.);
#2441=FACE_OUTER_BOUND('',#3391,.T.);
#2442=FACE_OUTER_BOUND('',#3393,.T.);
#3223=EDGE_LOOP('',(#11535,#11536,#11537,#11538));
#3224=EDGE_LOOP('',(#11539,#11540,#11541,#11542));
#3225=EDGE_LOOP('',(#11543,#11544,#11545,#11546));
#3226=EDGE_LOOP('',(#11547,#11548,#11549,#11550,#11551,#11552,#11553,#11554,
#11555,#11556,#11557,#11558,#11559,#11560,#11561,#11562,#11563,#11564,#11565,
#11566,#11567,#11568,#11569,#11570,#11571,#11572,#11573,#11574,#11575,#11576,
#11577,#11578,#11579,#11580,#11581,#11582,#11583,#11584,#11585,#11586,#11587,
#11588,#11589,#11590,#11591,#11592,#11593,#11594,#11595,#11596,#11597,#11598,
#11599,#11600,#11601,#11602,#11603,#11604,#11605,#11606,#11607,#11608,#11609,
#11610,#11611,#11612,#11613,#11614,#11615,#11616,#11617,#11618,#11619,#11620,
#11621,#11622,#11623,#11624,#11625,#11626,#11627,#11628,#11629,#11630,#11631,
#11632,#11633,#11634,#11635,#11636,#11637,#11638,#11639,#11640,#11641,#11642,
#11643,#11644,#11645,#11646,#11647,#11648,#11649,#11650,#11651,#11652,#11653,
#11654,#11655,#11656,#11657,#11658,#11659,#11660,#11661,#11662,#11663,#11664,
#11665,#11666,#11667,#11668,#11669,#11670,#11671,#11672,#11673,#11674,#11675,
#11676,#11677,#11678,#11679,#11680,#11681,#11682,#11683,#11684,#11685,#11686,
#11687,#11688,#11689,#11690,#11691,#11692,#11693,#11694,#11695,#11696,#11697,
#11698,#11699,#11700,#11701,#11702,#11703,#11704,#11705,#11706));
#3227=EDGE_LOOP('',(#11707,#11708,#11709,#11710));
#3228=EDGE_LOOP('',(#11711,#11712,#11713,#11714));
#3229=EDGE_LOOP('',(#11715,#11716,#11717,#11718));
#3230=EDGE_LOOP('',(#11719));
#3231=EDGE_LOOP('',(#11720,#11721,#11722,#11723));
#3232=EDGE_LOOP('',(#11724,#11725,#11726,#11727));
#3233=EDGE_LOOP('',(#11728,#11729,#11730,#11731));
#3234=EDGE_LOOP('',(#11732,#11733,#11734,#11735));
#3235=EDGE_LOOP('',(#11736,#11737,#11738,#11739));
#3236=EDGE_LOOP('',(#11740,#11741,#11742,#11743));
#3237=EDGE_LOOP('',(#11744,#11745,#11746,#11747));
#3238=EDGE_LOOP('',(#11748,#11749,#11750,#11751));
#3239=EDGE_LOOP('',(#11752,#11753,#11754,#11755));
#3240=EDGE_LOOP('',(#11756,#11757,#11758,#11759));
#3241=EDGE_LOOP('',(#11760,#11761,#11762,#11763));
#3242=EDGE_LOOP('',(#11764,#11765,#11766,#11767));
#3243=EDGE_LOOP('',(#11768,#11769,#11770,#11771));
#3244=EDGE_LOOP('',(#11772,#11773,#11774,#11775));
#3245=EDGE_LOOP('',(#11776,#11777,#11778,#11779));
#3246=EDGE_LOOP('',(#11780,#11781,#11782,#11783));
#3247=EDGE_LOOP('',(#11784,#11785,#11786,#11787));
#3248=EDGE_LOOP('',(#11788,#11789,#11790,#11791));
#3249=EDGE_LOOP('',(#11792,#11793,#11794,#11795));
#3250=EDGE_LOOP('',(#11796,#11797,#11798,#11799));
#3251=EDGE_LOOP('',(#11800,#11801,#11802,#11803));
#3252=EDGE_LOOP('',(#11804,#11805,#11806,#11807));
#3253=EDGE_LOOP('',(#11808,#11809,#11810,#11811));
#3254=EDGE_LOOP('',(#11812,#11813,#11814,#11815));
#3255=EDGE_LOOP('',(#11816,#11817,#11818,#11819));
#3256=EDGE_LOOP('',(#11820,#11821,#11822,#11823));
#3257=EDGE_LOOP('',(#11824,#11825,#11826,#11827));
#3258=EDGE_LOOP('',(#11828,#11829,#11830,#11831));
#3259=EDGE_LOOP('',(#11832,#11833,#11834,#11835));
#3260=EDGE_LOOP('',(#11836,#11837,#11838,#11839));
#3261=EDGE_LOOP('',(#11840,#11841,#11842,#11843));
#3262=EDGE_LOOP('',(#11844,#11845,#11846,#11847));
#3263=EDGE_LOOP('',(#11848,#11849,#11850,#11851));
#3264=EDGE_LOOP('',(#11852,#11853,#11854,#11855));
#3265=EDGE_LOOP('',(#11856,#11857,#11858,#11859));
#3266=EDGE_LOOP('',(#11860,#11861,#11862,#11863));
#3267=EDGE_LOOP('',(#11864,#11865,#11866,#11867));
#3268=EDGE_LOOP('',(#11868,#11869,#11870,#11871));
#3269=EDGE_LOOP('',(#11872,#11873,#11874,#11875));
#3270=EDGE_LOOP('',(#11876,#11877,#11878,#11879));
#3271=EDGE_LOOP('',(#11880,#11881,#11882,#11883));
#3272=EDGE_LOOP('',(#11884,#11885,#11886,#11887));
#3273=EDGE_LOOP('',(#11888,#11889,#11890,#11891));
#3274=EDGE_LOOP('',(#11892,#11893,#11894,#11895));
#3275=EDGE_LOOP('',(#11896,#11897,#11898,#11899));
#3276=EDGE_LOOP('',(#11900,#11901,#11902,#11903));
#3277=EDGE_LOOP('',(#11904,#11905,#11906,#11907));
#3278=EDGE_LOOP('',(#11908,#11909,#11910,#11911));
#3279=EDGE_LOOP('',(#11912,#11913,#11914,#11915));
#3280=EDGE_LOOP('',(#11916,#11917,#11918,#11919));
#3281=EDGE_LOOP('',(#11920,#11921,#11922,#11923));
#3282=EDGE_LOOP('',(#11924,#11925,#11926,#11927));
#3283=EDGE_LOOP('',(#11928,#11929,#11930,#11931));
#3284=EDGE_LOOP('',(#11932,#11933,#11934,#11935));
#3285=EDGE_LOOP('',(#11936,#11937,#11938,#11939));
#3286=EDGE_LOOP('',(#11940,#11941,#11942,#11943));
#3287=EDGE_LOOP('',(#11944,#11945,#11946,#11947));
#3288=EDGE_LOOP('',(#11948,#11949,#11950,#11951));
#3289=EDGE_LOOP('',(#11952,#11953,#11954,#11955));
#3290=EDGE_LOOP('',(#11956,#11957,#11958,#11959));
#3291=EDGE_LOOP('',(#11960,#11961,#11962,#11963));
#3292=EDGE_LOOP('',(#11964,#11965,#11966,#11967));
#3293=EDGE_LOOP('',(#11968,#11969,#11970,#11971));
#3294=EDGE_LOOP('',(#11972,#11973,#11974,#11975));
#3295=EDGE_LOOP('',(#11976,#11977,#11978,#11979));
#3296=EDGE_LOOP('',(#11980,#11981,#11982,#11983));
#3297=EDGE_LOOP('',(#11984,#11985,#11986,#11987));
#3298=EDGE_LOOP('',(#11988,#11989,#11990,#11991));
#3299=EDGE_LOOP('',(#11992,#11993,#11994,#11995));
#3300=EDGE_LOOP('',(#11996,#11997,#11998,#11999));
#3301=EDGE_LOOP('',(#12000,#12001,#12002,#12003));
#3302=EDGE_LOOP('',(#12004,#12005,#12006,#12007));
#3303=EDGE_LOOP('',(#12008,#12009,#12010,#12011));
#3304=EDGE_LOOP('',(#12012,#12013,#12014,#12015));
#3305=EDGE_LOOP('',(#12016,#12017,#12018,#12019));
#3306=EDGE_LOOP('',(#12020,#12021,#12022,#12023));
#3307=EDGE_LOOP('',(#12024,#12025,#12026,#12027));
#3308=EDGE_LOOP('',(#12028,#12029,#12030,#12031));
#3309=EDGE_LOOP('',(#12032,#12033,#12034,#12035));
#3310=EDGE_LOOP('',(#12036,#12037,#12038,#12039));
#3311=EDGE_LOOP('',(#12040,#12041,#12042,#12043));
#3312=EDGE_LOOP('',(#12044,#12045,#12046,#12047));
#3313=EDGE_LOOP('',(#12048,#12049,#12050,#12051));
#3314=EDGE_LOOP('',(#12052,#12053,#12054,#12055));
#3315=EDGE_LOOP('',(#12056,#12057,#12058,#12059));
#3316=EDGE_LOOP('',(#12060,#12061,#12062,#12063));
#3317=EDGE_LOOP('',(#12064,#12065,#12066,#12067));
#3318=EDGE_LOOP('',(#12068,#12069,#12070,#12071));
#3319=EDGE_LOOP('',(#12072,#12073,#12074,#12075));
#3320=EDGE_LOOP('',(#12076,#12077,#12078,#12079));
#3321=EDGE_LOOP('',(#12080,#12081,#12082,#12083));
#3322=EDGE_LOOP('',(#12084,#12085,#12086,#12087));
#3323=EDGE_LOOP('',(#12088,#12089,#12090,#12091));
#3324=EDGE_LOOP('',(#12092,#12093,#12094,#12095));
#3325=EDGE_LOOP('',(#12096,#12097,#12098,#12099));
#3326=EDGE_LOOP('',(#12100,#12101,#12102,#12103));
#3327=EDGE_LOOP('',(#12104,#12105,#12106,#12107));
#3328=EDGE_LOOP('',(#12108,#12109,#12110,#12111));
#3329=EDGE_LOOP('',(#12112,#12113,#12114,#12115));
#3330=EDGE_LOOP('',(#12116,#12117,#12118,#12119));
#3331=EDGE_LOOP('',(#12120,#12121,#12122,#12123));
#3332=EDGE_LOOP('',(#12124,#12125,#12126,#12127));
#3333=EDGE_LOOP('',(#12128,#12129,#12130,#12131));
#3334=EDGE_LOOP('',(#12132,#12133,#12134,#12135));
#3335=EDGE_LOOP('',(#12136,#12137,#12138,#12139));
#3336=EDGE_LOOP('',(#12140,#12141,#12142,#12143));
#3337=EDGE_LOOP('',(#12144,#12145,#12146,#12147));
#3338=EDGE_LOOP('',(#12148,#12149,#12150,#12151));
#3339=EDGE_LOOP('',(#12152,#12153,#12154,#12155));
#3340=EDGE_LOOP('',(#12156,#12157,#12158,#12159));
#3341=EDGE_LOOP('',(#12160,#12161,#12162,#12163));
#3342=EDGE_LOOP('',(#12164,#12165,#12166,#12167));
#3343=EDGE_LOOP('',(#12168,#12169,#12170,#12171));
#3344=EDGE_LOOP('',(#12172,#12173,#12174,#12175));
#3345=EDGE_LOOP('',(#12176,#12177,#12178,#12179));
#3346=EDGE_LOOP('',(#12180,#12181,#12182,#12183));
#3347=EDGE_LOOP('',(#12184,#12185,#12186,#12187));
#3348=EDGE_LOOP('',(#12188,#12189,#12190,#12191));
#3349=EDGE_LOOP('',(#12192,#12193,#12194,#12195));
#3350=EDGE_LOOP('',(#12196,#12197,#12198,#12199));
#3351=EDGE_LOOP('',(#12200,#12201,#12202,#12203));
#3352=EDGE_LOOP('',(#12204,#12205,#12206,#12207));
#3353=EDGE_LOOP('',(#12208,#12209,#12210,#12211));
#3354=EDGE_LOOP('',(#12212,#12213,#12214,#12215));
#3355=EDGE_LOOP('',(#12216,#12217,#12218,#12219));
#3356=EDGE_LOOP('',(#12220,#12221,#12222,#12223));
#3357=EDGE_LOOP('',(#12224,#12225,#12226,#12227));
#3358=EDGE_LOOP('',(#12228,#12229,#12230,#12231));
#3359=EDGE_LOOP('',(#12232,#12233,#12234,#12235));
#3360=EDGE_LOOP('',(#12236,#12237,#12238,#12239));
#3361=EDGE_LOOP('',(#12240,#12241,#12242,#12243));
#3362=EDGE_LOOP('',(#12244,#12245,#12246,#12247));
#3363=EDGE_LOOP('',(#12248,#12249,#12250,#12251));
#3364=EDGE_LOOP('',(#12252,#12253,#12254,#12255));
#3365=EDGE_LOOP('',(#12256,#12257,#12258,#12259));
#3366=EDGE_LOOP('',(#12260,#12261,#12262,#12263));
#3367=EDGE_LOOP('',(#12264,#12265,#12266,#12267));
#3368=EDGE_LOOP('',(#12268,#12269,#12270,#12271));
#3369=EDGE_LOOP('',(#12272,#12273,#12274,#12275));
#3370=EDGE_LOOP('',(#12276,#12277,#12278,#12279));
#3371=EDGE_LOOP('',(#12280,#12281,#12282,#12283));
#3372=EDGE_LOOP('',(#12284,#12285,#12286,#12287));
#3373=EDGE_LOOP('',(#12288,#12289,#12290,#12291));
#3374=EDGE_LOOP('',(#12292,#12293,#12294,#12295));
#3375=EDGE_LOOP('',(#12296,#12297,#12298,#12299));
#3376=EDGE_LOOP('',(#12300,#12301,#12302,#12303));
#3377=EDGE_LOOP('',(#12304,#12305,#12306,#12307));
#3378=EDGE_LOOP('',(#12308,#12309,#12310,#12311));
#3379=EDGE_LOOP('',(#12312,#12313,#12314,#12315));
#3380=EDGE_LOOP('',(#12316,#12317,#12318,#12319));
#3381=EDGE_LOOP('',(#12320,#12321,#12322,#12323));
#3382=EDGE_LOOP('',(#12324,#12325,#12326,#12327));
#3383=EDGE_LOOP('',(#12328,#12329,#12330,#12331));
#3384=EDGE_LOOP('',(#12332,#12333,#12334,#12335));
#3385=EDGE_LOOP('',(#12336,#12337,#12338,#12339));
#3386=EDGE_LOOP('',(#12340,#12341,#12342,#12343));
#3387=EDGE_LOOP('',(#12344,#12345,#12346,#12347));
#3388=EDGE_LOOP('',(#12348,#12349,#12350,#12351));
#3389=EDGE_LOOP('',(#12352,#12353,#12354,#12355));
#3390=EDGE_LOOP('',(#12356,#12357,#12358,#12359));
#3391=EDGE_LOOP('',(#12360,#12361,#12362,#12363,#12364,#12365,#12366,#12367,
#12368,#12369,#12370,#12371,#12372,#12373,#12374,#12375,#12376,#12377,#12378,
#12379,#12380,#12381,#12382,#12383,#12384,#12385,#12386,#12387,#12388,#12389,
#12390,#12391,#12392,#12393,#12394,#12395,#12396,#12397,#12398,#12399,#12400,
#12401,#12402,#12403,#12404,#12405,#12406,#12407,#12408,#12409,#12410,#12411,
#12412,#12413,#12414,#12415,#12416,#12417,#12418,#12419,#12420,#12421,#12422,
#12423,#12424,#12425,#12426,#12427,#12428,#12429,#12430,#12431,#12432,#12433,
#12434,#12435,#12436,#12437,#12438,#12439,#12440,#12441,#12442,#12443,#12444,
#12445,#12446,#12447,#12448,#12449,#12450,#12451,#12452,#12453,#12454,#12455,
#12456,#12457,#12458,#12459,#12460,#12461,#12462,#12463,#12464,#12465,#12466,
#12467,#12468,#12469,#12470,#12471,#12472,#12473,#12474,#12475,#12476,#12477,
#12478,#12479,#12480,#12481,#12482,#12483,#12484,#12485,#12486,#12487,#12488,
#12489,#12490,#12491,#12492,#12493,#12494,#12495,#12496,#12497,#12498,#12499,
#12500,#12501,#12502,#12503,#12504,#12505,#12506,#12507,#12508,#12509,#12510,
#12511,#12512,#12513,#12514,#12515,#12516,#12517,#12518,#12519));
#3392=EDGE_LOOP('',(#12520));
#3393=EDGE_LOOP('',(#12521,#12522,#12523,#12524));
#4106=LINE('',#34092,#4995);
#4107=LINE('',#34094,#4996);
#4108=LINE('',#34096,#4997);
#4109=LINE('',#34097,#4998);
#4110=LINE('',#34100,#4999);
#4111=LINE('',#34102,#5000);
#4112=LINE('',#34103,#5001);
#4113=LINE('',#34106,#5002);
#4114=LINE('',#34108,#5003);
#4115=LINE('',#34109,#5004);
#4116=LINE('',#34186,#5005);
#4117=LINE('',#34332,#5006);
#4118=LINE('',#34478,#5007);
#4119=LINE('',#34624,#5008);
#4120=LINE('',#34770,#5009);
#4121=LINE('',#34916,#5010);
#4122=LINE('',#35062,#5011);
#4123=LINE('',#35208,#5012);
#4124=LINE('',#35354,#5013);
#4125=LINE('',#35500,#5014);
#4126=LINE('',#35646,#5015);
#4127=LINE('',#35792,#5016);
#4128=LINE('',#35938,#5017);
#4129=LINE('',#36084,#5018);
#4130=LINE('',#36230,#5019);
#4131=LINE('',#36376,#5020);
#4132=LINE('',#36522,#5021);
#4133=LINE('',#36668,#5022);
#4134=LINE('',#36814,#5023);
#4135=LINE('',#36960,#5024);
#4136=LINE('',#37106,#5025);
#4137=LINE('',#37252,#5026);
#4138=LINE('',#37398,#5027);
#4139=LINE('',#37544,#5028);
#4140=LINE('',#37690,#5029);
#4141=LINE('',#37836,#5030);
#4142=LINE('',#37982,#5031);
#4143=LINE('',#38128,#5032);
#4144=LINE('',#38274,#5033);
#4145=LINE('',#38420,#5034);
#4146=LINE('',#38566,#5035);
#4147=LINE('',#38712,#5036);
#4148=LINE('',#38858,#5037);
#4149=LINE('',#39004,#5038);
#4150=LINE('',#39150,#5039);
#4151=LINE('',#39296,#5040);
#4152=LINE('',#39442,#5041);
#4153=LINE('',#39588,#5042);
#4154=LINE('',#39734,#5043);
#4155=LINE('',#39880,#5044);
#4156=LINE('',#39958,#5045);
#4157=LINE('',#40179,#5046);
#4158=LINE('',#40328,#5047);
#4159=LINE('',#40400,#5048);
#4160=LINE('',#40621,#5049);
#4161=LINE('',#40770,#5050);
#4162=LINE('',#40842,#5051);
#4163=LINE('',#41063,#5052);
#4164=LINE('',#41212,#5053);
#4165=LINE('',#41284,#5054);
#4166=LINE('',#41505,#5055);
#4167=LINE('',#41654,#5056);
#4168=LINE('',#41726,#5057);
#4169=LINE('',#41947,#5058);
#4170=LINE('',#42096,#5059);
#4171=LINE('',#42168,#5060);
#4172=LINE('',#42389,#5061);
#4173=LINE('',#42538,#5062);
#4174=LINE('',#42610,#5063);
#4175=LINE('',#42831,#5064);
#4176=LINE('',#42980,#5065);
#4177=LINE('',#43052,#5066);
#4178=LINE('',#43273,#5067);
#4179=LINE('',#43422,#5068);
#4180=LINE('',#43494,#5069);
#4181=LINE('',#43715,#5070);
#4182=LINE('',#43864,#5071);
#4183=LINE('',#43936,#5072);
#4184=LINE('',#44157,#5073);
#4185=LINE('',#44306,#5074);
#4186=LINE('',#44378,#5075);
#4187=LINE('',#44599,#5076);
#4188=LINE('',#44748,#5077);
#4189=LINE('',#44820,#5078);
#4190=LINE('',#45041,#5079);
#4191=LINE('',#45190,#5080);
#4192=LINE('',#45262,#5081);
#4193=LINE('',#45483,#5082);
#4194=LINE('',#45632,#5083);
#4195=LINE('',#45704,#5084);
#4196=LINE('',#45925,#5085);
#4197=LINE('',#46074,#5086);
#4198=LINE('',#46146,#5087);
#4199=LINE('',#46367,#5088);
#4200=LINE('',#46516,#5089);
#4201=LINE('',#46588,#5090);
#4202=LINE('',#46809,#5091);
#4203=LINE('',#46958,#5092);
#4204=LINE('',#47030,#5093);
#4205=LINE('',#47251,#5094);
#4206=LINE('',#47400,#5095);
#4207=LINE('',#47472,#5096);
#4208=LINE('',#47693,#5097);
#4209=LINE('',#47842,#5098);
#4210=LINE('',#47914,#5099);
#4211=LINE('',#48135,#5100);
#4212=LINE('',#48284,#5101);
#4213=LINE('',#48356,#5102);
#4214=LINE('',#48577,#5103);
#4215=LINE('',#48726,#5104);
#4216=LINE('',#48798,#5105);
#4217=LINE('',#49019,#5106);
#4218=LINE('',#49168,#5107);
#4219=LINE('',#49240,#5108);
#4220=LINE('',#49461,#5109);
#4221=LINE('',#49610,#5110);
#4222=LINE('',#49682,#5111);
#4223=LINE('',#49903,#5112);
#4224=LINE('',#50052,#5113);
#4225=LINE('',#50124,#5114);
#4226=LINE('',#50345,#5115);
#4227=LINE('',#50494,#5116);
#4228=LINE('',#50566,#5117);
#4229=LINE('',#50787,#5118);
#4230=LINE('',#50936,#5119);
#4231=LINE('',#51008,#5120);
#4232=LINE('',#51229,#5121);
#4233=LINE('',#51378,#5122);
#4234=LINE('',#51450,#5123);
#4235=LINE('',#51671,#5124);
#4236=LINE('',#51820,#5125);
#4237=LINE('',#51892,#5126);
#4238=LINE('',#52113,#5127);
#4239=LINE('',#52262,#5128);
#4240=LINE('',#52334,#5129);
#4241=LINE('',#52555,#5130);
#4242=LINE('',#52704,#5131);
#4243=LINE('',#52776,#5132);
#4244=LINE('',#52997,#5133);
#4245=LINE('',#53146,#5134);
#4246=LINE('',#53218,#5135);
#4247=LINE('',#53439,#5136);
#4248=LINE('',#53588,#5137);
#4249=LINE('',#53660,#5138);
#4250=LINE('',#53881,#5139);
#4251=LINE('',#54030,#5140);
#4252=LINE('',#54102,#5141);
#4253=LINE('',#54323,#5142);
#4254=LINE('',#54472,#5143);
#4255=LINE('',#54544,#5144);
#4256=LINE('',#54765,#5145);
#4257=LINE('',#54914,#5146);
#4258=LINE('',#54986,#5147);
#4259=LINE('',#55207,#5148);
#4260=LINE('',#55356,#5149);
#4261=LINE('',#55428,#5150);
#4262=LINE('',#55649,#5151);
#4263=LINE('',#55798,#5152);
#4264=LINE('',#55870,#5153);
#4265=LINE('',#56091,#5154);
#4266=LINE('',#56240,#5155);
#4267=LINE('',#56312,#5156);
#4268=LINE('',#56533,#5157);
#4269=LINE('',#56682,#5158);
#4270=LINE('',#56754,#5159);
#4271=LINE('',#56975,#5160);
#4272=LINE('',#56978,#5161);
#4273=LINE('',#56979,#5162);
#4274=LINE('',#57354,#5163);
#4275=LINE('',#57636,#5164);
#4276=LINE('',#57638,#5165);
#4995=VECTOR('',#18499,1.);
#4996=VECTOR('',#18500,1.);
#4997=VECTOR('',#18501,1.);
#4998=VECTOR('',#18502,1.);
#4999=VECTOR('',#18505,1.);
#5000=VECTOR('',#18506,1.);
#5001=VECTOR('',#18507,1.);
#5002=VECTOR('',#18510,1.);
#5003=VECTOR('',#18511,1.);
#5004=VECTOR('',#18512,1.);
#5005=VECTOR('',#18517,1.);
#5006=VECTOR('',#18520,1.);
#5007=VECTOR('',#18523,1.);
#5008=VECTOR('',#18526,1.);
#5009=VECTOR('',#18529,1.);
#5010=VECTOR('',#18532,1.);
#5011=VECTOR('',#18535,1.);
#5012=VECTOR('',#18538,1.);
#5013=VECTOR('',#18541,1.);
#5014=VECTOR('',#18544,1.);
#5015=VECTOR('',#18547,1.);
#5016=VECTOR('',#18550,1.);
#5017=VECTOR('',#18553,1.);
#5018=VECTOR('',#18556,1.);
#5019=VECTOR('',#18559,1.);
#5020=VECTOR('',#18562,1.);
#5021=VECTOR('',#18565,1.);
#5022=VECTOR('',#18568,1.);
#5023=VECTOR('',#18571,1.);
#5024=VECTOR('',#18574,1.);
#5025=VECTOR('',#18577,1.);
#5026=VECTOR('',#18580,1.);
#5027=VECTOR('',#18583,1.);
#5028=VECTOR('',#18586,1.);
#5029=VECTOR('',#18589,1.);
#5030=VECTOR('',#18592,1.);
#5031=VECTOR('',#18595,1.);
#5032=VECTOR('',#18598,1.);
#5033=VECTOR('',#18601,1.);
#5034=VECTOR('',#18604,1.);
#5035=VECTOR('',#18607,1.);
#5036=VECTOR('',#18610,1.);
#5037=VECTOR('',#18613,1.);
#5038=VECTOR('',#18616,1.);
#5039=VECTOR('',#18619,1.);
#5040=VECTOR('',#18622,1.);
#5041=VECTOR('',#18625,1.);
#5042=VECTOR('',#18628,1.);
#5043=VECTOR('',#18631,1.);
#5044=VECTOR('',#18634,1.);
#5045=VECTOR('',#18645,2.);
#5046=VECTOR('',#18650,1.);
#5047=VECTOR('',#18651,1.);
#5048=VECTOR('',#18654,1.);
#5049=VECTOR('',#18659,1.);
#5050=VECTOR('',#18660,1.);
#5051=VECTOR('',#18663,1.);
#5052=VECTOR('',#18668,1.);
#5053=VECTOR('',#18669,1.);
#5054=VECTOR('',#18672,1.);
#5055=VECTOR('',#18677,1.);
#5056=VECTOR('',#18678,1.);
#5057=VECTOR('',#18681,1.);
#5058=VECTOR('',#18686,1.);
#5059=VECTOR('',#18687,1.);
#5060=VECTOR('',#18690,1.);
#5061=VECTOR('',#18695,1.);
#5062=VECTOR('',#18696,1.);
#5063=VECTOR('',#18699,1.);
#5064=VECTOR('',#18704,1.);
#5065=VECTOR('',#18705,1.);
#5066=VECTOR('',#18708,1.);
#5067=VECTOR('',#18713,1.);
#5068=VECTOR('',#18714,1.);
#5069=VECTOR('',#18717,1.);
#5070=VECTOR('',#18722,1.);
#5071=VECTOR('',#18723,1.);
#5072=VECTOR('',#18726,1.);
#5073=VECTOR('',#18731,1.);
#5074=VECTOR('',#18732,1.);
#5075=VECTOR('',#18735,1.);
#5076=VECTOR('',#18740,1.);
#5077=VECTOR('',#18741,1.);
#5078=VECTOR('',#18744,1.);
#5079=VECTOR('',#18749,1.);
#5080=VECTOR('',#18750,1.);
#5081=VECTOR('',#18753,1.);
#5082=VECTOR('',#18758,1.);
#5083=VECTOR('',#18759,1.);
#5084=VECTOR('',#18762,1.);
#5085=VECTOR('',#18767,1.);
#5086=VECTOR('',#18768,1.);
#5087=VECTOR('',#18771,1.);
#5088=VECTOR('',#18776,1.);
#5089=VECTOR('',#18777,1.);
#5090=VECTOR('',#18780,1.);
#5091=VECTOR('',#18785,1.);
#5092=VECTOR('',#18786,1.);
#5093=VECTOR('',#18789,1.);
#5094=VECTOR('',#18794,1.);
#5095=VECTOR('',#18795,1.);
#5096=VECTOR('',#18798,1.);
#5097=VECTOR('',#18803,1.);
#5098=VECTOR('',#18804,1.);
#5099=VECTOR('',#18807,1.);
#5100=VECTOR('',#18812,1.);
#5101=VECTOR('',#18813,1.);
#5102=VECTOR('',#18816,1.);
#5103=VECTOR('',#18821,1.);
#5104=VECTOR('',#18822,1.);
#5105=VECTOR('',#18825,1.);
#5106=VECTOR('',#18830,1.);
#5107=VECTOR('',#18831,1.);
#5108=VECTOR('',#18834,1.);
#5109=VECTOR('',#18839,1.);
#5110=VECTOR('',#18840,1.);
#5111=VECTOR('',#18843,1.);
#5112=VECTOR('',#18848,1.);
#5113=VECTOR('',#18849,1.);
#5114=VECTOR('',#18852,1.);
#5115=VECTOR('',#18857,1.);
#5116=VECTOR('',#18858,1.);
#5117=VECTOR('',#18861,1.);
#5118=VECTOR('',#18866,1.);
#5119=VECTOR('',#18867,1.);
#5120=VECTOR('',#18870,1.);
#5121=VECTOR('',#18875,1.);
#5122=VECTOR('',#18876,1.);
#5123=VECTOR('',#18879,1.);
#5124=VECTOR('',#18884,1.);
#5125=VECTOR('',#18885,1.);
#5126=VECTOR('',#18888,1.);
#5127=VECTOR('',#18893,1.);
#5128=VECTOR('',#18894,1.);
#5129=VECTOR('',#18897,1.);
#5130=VECTOR('',#18902,1.);
#5131=VECTOR('',#18903,1.);
#5132=VECTOR('',#18906,1.);
#5133=VECTOR('',#18911,1.);
#5134=VECTOR('',#18912,1.);
#5135=VECTOR('',#18915,1.);
#5136=VECTOR('',#18920,1.);
#5137=VECTOR('',#18921,1.);
#5138=VECTOR('',#18924,1.);
#5139=VECTOR('',#18929,1.);
#5140=VECTOR('',#18930,1.);
#5141=VECTOR('',#18933,1.);
#5142=VECTOR('',#18938,1.);
#5143=VECTOR('',#18939,1.);
#5144=VECTOR('',#18942,1.);
#5145=VECTOR('',#18947,1.);
#5146=VECTOR('',#18948,1.);
#5147=VECTOR('',#18951,1.);
#5148=VECTOR('',#18956,1.);
#5149=VECTOR('',#18957,1.);
#5150=VECTOR('',#18960,1.);
#5151=VECTOR('',#18965,1.);
#5152=VECTOR('',#18966,1.);
#5153=VECTOR('',#18969,1.);
#5154=VECTOR('',#18974,1.);
#5155=VECTOR('',#18975,1.);
#5156=VECTOR('',#18978,1.);
#5157=VECTOR('',#18983,1.);
#5158=VECTOR('',#18984,1.);
#5159=VECTOR('',#18987,1.);
#5160=VECTOR('',#18992,1.);
#5161=VECTOR('',#18995,1.);
#5162=VECTOR('',#18996,1.);
#5163=VECTOR('',#19001,1.);
#5164=VECTOR('',#19002,1.);
#5165=VECTOR('',#19005,1.);
#5690=CIRCLE('',#15311,3.75);
#5691=CIRCLE('',#15312,3.75);
#5692=CIRCLE('',#15313,3.75);
#5693=CIRCLE('',#15314,3.75);
#5694=CIRCLE('',#15315,3.75);
#5695=CIRCLE('',#15316,3.75);
#5696=CIRCLE('',#15317,3.75);
#5697=CIRCLE('',#15318,3.75);
#5698=CIRCLE('',#15319,3.75);
#5699=CIRCLE('',#15320,3.75);
#5700=CIRCLE('',#15321,3.75);
#5701=CIRCLE('',#15322,3.75);
#5702=CIRCLE('',#15323,3.75);
#5703=CIRCLE('',#15324,3.75);
#5704=CIRCLE('',#15325,3.75);
#5705=CIRCLE('',#15326,3.75);
#5706=CIRCLE('',#15327,3.75);
#5707=CIRCLE('',#15328,3.75);
#5708=CIRCLE('',#15329,3.75);
#5709=CIRCLE('',#15330,3.75);
#5710=CIRCLE('',#15331,3.75);
#5711=CIRCLE('',#15332,3.75);
#5712=CIRCLE('',#15333,3.75);
#5713=CIRCLE('',#15334,3.75);
#5714=CIRCLE('',#15335,3.75);
#5715=CIRCLE('',#15336,3.75);
#5716=CIRCLE('',#15337,3.75);
#5717=CIRCLE('',#15338,3.75);
#5718=CIRCLE('',#15339,3.75);
#5719=CIRCLE('',#15340,3.75);
#5720=CIRCLE('',#15341,3.75);
#5721=CIRCLE('',#15342,3.75);
#5722=CIRCLE('',#15343,3.75);
#5723=CIRCLE('',#15344,3.75);
#5724=CIRCLE('',#15345,3.75);
#5725=CIRCLE('',#15346,3.75);
#5726=CIRCLE('',#15347,3.75);
#5727=CIRCLE('',#15348,3.75);
#5728=CIRCLE('',#15349,3.75);
#5729=CIRCLE('',#15350,3.75);
#5730=CIRCLE('',#15351,1.);
#5731=CIRCLE('',#15353,1.);
#5732=CIRCLE('',#15355,2.);
#5733=CIRCLE('',#15356,2.);
#5734=CIRCLE('',#15360,3.75);
#5735=CIRCLE('',#15363,3.75);
#5736=CIRCLE('',#15366,3.75);
#5737=CIRCLE('',#15369,3.75);
#5738=CIRCLE('',#15372,3.75);
#5739=CIRCLE('',#15375,3.75);
#5740=CIRCLE('',#15378,3.75);
#5741=CIRCLE('',#15381,3.75);
#5742=CIRCLE('',#15384,3.75);
#5743=CIRCLE('',#15387,3.75);
#5744=CIRCLE('',#15390,3.75);
#5745=CIRCLE('',#15393,3.75);
#5746=CIRCLE('',#15396,3.75);
#5747=CIRCLE('',#15399,3.75);
#5748=CIRCLE('',#15402,3.75);
#5749=CIRCLE('',#15405,3.75);
#5750=CIRCLE('',#15408,3.75);
#5751=CIRCLE('',#15411,3.75);
#5752=CIRCLE('',#15414,3.75);
#5753=CIRCLE('',#15417,3.75);
#5754=CIRCLE('',#15420,3.75);
#5755=CIRCLE('',#15423,3.75);
#5756=CIRCLE('',#15426,3.75);
#5757=CIRCLE('',#15429,3.75);
#5758=CIRCLE('',#15432,3.75);
#5759=CIRCLE('',#15435,3.75);
#5760=CIRCLE('',#15438,3.75);
#5761=CIRCLE('',#15441,3.75);
#5762=CIRCLE('',#15444,3.75);
#5763=CIRCLE('',#15447,3.75);
#5764=CIRCLE('',#15450,3.75);
#5765=CIRCLE('',#15453,3.75);
#5766=CIRCLE('',#15456,3.75);
#5767=CIRCLE('',#15459,3.75);
#5768=CIRCLE('',#15462,3.75);
#5769=CIRCLE('',#15465,3.75);
#5770=CIRCLE('',#15468,3.75);
#5771=CIRCLE('',#15471,3.75);
#5772=CIRCLE('',#15474,3.75);
#5773=CIRCLE('',#15477,3.75);
#6677=VERTEX_POINT('',#34090);
#6678=VERTEX_POINT('',#34091);
#6679=VERTEX_POINT('',#34093);
#6680=VERTEX_POINT('',#34095);
#6681=VERTEX_POINT('',#34099);
#6682=VERTEX_POINT('',#34101);
#6683=VERTEX_POINT('',#34105);
#6684=VERTEX_POINT('',#34107);
#6685=VERTEX_POINT('',#34111);
#6686=VERTEX_POINT('',#34112);
#6687=VERTEX_POINT('',#34114);
#6688=VERTEX_POINT('',#34185);
#6689=VERTEX_POINT('',#34187);
#6690=VERTEX_POINT('',#34258);
#6691=VERTEX_POINT('',#34260);
#6692=VERTEX_POINT('',#34331);
#6693=VERTEX_POINT('',#34333);
#6694=VERTEX_POINT('',#34404);
#6695=VERTEX_POINT('',#34406);
#6696=VERTEX_POINT('',#34477);
#6697=VERTEX_POINT('',#34479);
#6698=VERTEX_POINT('',#34550);
#6699=VERTEX_POINT('',#34552);
#6700=VERTEX_POINT('',#34623);
#6701=VERTEX_POINT('',#34625);
#6702=VERTEX_POINT('',#34696);
#6703=VERTEX_POINT('',#34698);
#6704=VERTEX_POINT('',#34769);
#6705=VERTEX_POINT('',#34771);
#6706=VERTEX_POINT('',#34842);
#6707=VERTEX_POINT('',#34844);
#6708=VERTEX_POINT('',#34915);
#6709=VERTEX_POINT('',#34917);
#6710=VERTEX_POINT('',#34988);
#6711=VERTEX_POINT('',#34990);
#6712=VERTEX_POINT('',#35061);
#6713=VERTEX_POINT('',#35063);
#6714=VERTEX_POINT('',#35134);
#6715=VERTEX_POINT('',#35136);
#6716=VERTEX_POINT('',#35207);
#6717=VERTEX_POINT('',#35209);
#6718=VERTEX_POINT('',#35280);
#6719=VERTEX_POINT('',#35282);
#6720=VERTEX_POINT('',#35353);
#6721=VERTEX_POINT('',#35355);
#6722=VERTEX_POINT('',#35426);
#6723=VERTEX_POINT('',#35428);
#6724=VERTEX_POINT('',#35499);
#6725=VERTEX_POINT('',#35501);
#6726=VERTEX_POINT('',#35572);
#6727=VERTEX_POINT('',#35574);
#6728=VERTEX_POINT('',#35645);
#6729=VERTEX_POINT('',#35647);
#6730=VERTEX_POINT('',#35718);
#6731=VERTEX_POINT('',#35720);
#6732=VERTEX_POINT('',#35791);
#6733=VERTEX_POINT('',#35793);
#6734=VERTEX_POINT('',#35864);
#6735=VERTEX_POINT('',#35866);
#6736=VERTEX_POINT('',#35937);
#6737=VERTEX_POINT('',#35939);
#6738=VERTEX_POINT('',#36010);
#6739=VERTEX_POINT('',#36012);
#6740=VERTEX_POINT('',#36083);
#6741=VERTEX_POINT('',#36085);
#6742=VERTEX_POINT('',#36156);
#6743=VERTEX_POINT('',#36158);
#6744=VERTEX_POINT('',#36229);
#6745=VERTEX_POINT('',#36231);
#6746=VERTEX_POINT('',#36302);
#6747=VERTEX_POINT('',#36304);
#6748=VERTEX_POINT('',#36375);
#6749=VERTEX_POINT('',#36377);
#6750=VERTEX_POINT('',#36448);
#6751=VERTEX_POINT('',#36450);
#6752=VERTEX_POINT('',#36521);
#6753=VERTEX_POINT('',#36523);
#6754=VERTEX_POINT('',#36594);
#6755=VERTEX_POINT('',#36596);
#6756=VERTEX_POINT('',#36667);
#6757=VERTEX_POINT('',#36669);
#6758=VERTEX_POINT('',#36740);
#6759=VERTEX_POINT('',#36742);
#6760=VERTEX_POINT('',#36813);
#6761=VERTEX_POINT('',#36815);
#6762=VERTEX_POINT('',#36886);
#6763=VERTEX_POINT('',#36888);
#6764=VERTEX_POINT('',#36959);
#6765=VERTEX_POINT('',#36961);
#6766=VERTEX_POINT('',#37032);
#6767=VERTEX_POINT('',#37034);
#6768=VERTEX_POINT('',#37105);
#6769=VERTEX_POINT('',#37107);
#6770=VERTEX_POINT('',#37178);
#6771=VERTEX_POINT('',#37180);
#6772=VERTEX_POINT('',#37251);
#6773=VERTEX_POINT('',#37253);
#6774=VERTEX_POINT('',#37324);
#6775=VERTEX_POINT('',#37326);
#6776=VERTEX_POINT('',#37397);
#6777=VERTEX_POINT('',#37399);
#6778=VERTEX_POINT('',#37470);
#6779=VERTEX_POINT('',#37472);
#6780=VERTEX_POINT('',#37543);
#6781=VERTEX_POINT('',#37545);
#6782=VERTEX_POINT('',#37616);
#6783=VERTEX_POINT('',#37618);
#6784=VERTEX_POINT('',#37689);
#6785=VERTEX_POINT('',#37691);
#6786=VERTEX_POINT('',#37762);
#6787=VERTEX_POINT('',#37764);
#6788=VERTEX_POINT('',#37835);
#6789=VERTEX_POINT('',#37837);
#6790=VERTEX_POINT('',#37908);
#6791=VERTEX_POINT('',#37910);
#6792=VERTEX_POINT('',#37981);
#6793=VERTEX_POINT('',#37983);
#6794=VERTEX_POINT('',#38054);
#6795=VERTEX_POINT('',#38056);
#6796=VERTEX_POINT('',#38127);
#6797=VERTEX_POINT('',#38129);
#6798=VERTEX_POINT('',#38200);
#6799=VERTEX_POINT('',#38202);
#6800=VERTEX_POINT('',#38273);
#6801=VERTEX_POINT('',#38275);
#6802=VERTEX_POINT('',#38346);
#6803=VERTEX_POINT('',#38348);
#6804=VERTEX_POINT('',#38419);
#6805=VERTEX_POINT('',#38421);
#6806=VERTEX_POINT('',#38492);
#6807=VERTEX_POINT('',#38494);
#6808=VERTEX_POINT('',#38565);
#6809=VERTEX_POINT('',#38567);
#6810=VERTEX_POINT('',#38638);
#6811=VERTEX_POINT('',#38640);
#6812=VERTEX_POINT('',#38711);
#6813=VERTEX_POINT('',#38713);
#6814=VERTEX_POINT('',#38784);
#6815=VERTEX_POINT('',#38786);
#6816=VERTEX_POINT('',#38857);
#6817=VERTEX_POINT('',#38859);
#6818=VERTEX_POINT('',#38930);
#6819=VERTEX_POINT('',#38932);
#6820=VERTEX_POINT('',#39003);
#6821=VERTEX_POINT('',#39005);
#6822=VERTEX_POINT('',#39076);
#6823=VERTEX_POINT('',#39078);
#6824=VERTEX_POINT('',#39149);
#6825=VERTEX_POINT('',#39151);
#6826=VERTEX_POINT('',#39222);
#6827=VERTEX_POINT('',#39224);
#6828=VERTEX_POINT('',#39295);
#6829=VERTEX_POINT('',#39297);
#6830=VERTEX_POINT('',#39368);
#6831=VERTEX_POINT('',#39370);
#6832=VERTEX_POINT('',#39441);
#6833=VERTEX_POINT('',#39443);
#6834=VERTEX_POINT('',#39514);
#6835=VERTEX_POINT('',#39516);
#6836=VERTEX_POINT('',#39587);
#6837=VERTEX_POINT('',#39589);
#6838=VERTEX_POINT('',#39660);
#6839=VERTEX_POINT('',#39662);
#6840=VERTEX_POINT('',#39733);
#6841=VERTEX_POINT('',#39735);
#6842=VERTEX_POINT('',#39806);
#6843=VERTEX_POINT('',#39808);
#6844=VERTEX_POINT('',#39879);
#6845=VERTEX_POINT('',#39955);
#6846=VERTEX_POINT('',#39957);
#6847=VERTEX_POINT('',#40101);
#6848=VERTEX_POINT('',#40108);
#6849=VERTEX_POINT('',#40320);
#6850=VERTEX_POINT('',#40327);
#6851=VERTEX_POINT('',#40402);
#6852=VERTEX_POINT('',#40550);
#6853=VERTEX_POINT('',#40762);
#6854=VERTEX_POINT('',#40769);
#6855=VERTEX_POINT('',#40844);
#6856=VERTEX_POINT('',#40992);
#6857=VERTEX_POINT('',#41204);
#6858=VERTEX_POINT('',#41211);
#6859=VERTEX_POINT('',#41286);
#6860=VERTEX_POINT('',#41434);
#6861=VERTEX_POINT('',#41646);
#6862=VERTEX_POINT('',#41653);
#6863=VERTEX_POINT('',#41728);
#6864=VERTEX_POINT('',#41876);
#6865=VERTEX_POINT('',#42088);
#6866=VERTEX_POINT('',#42095);
#6867=VERTEX_POINT('',#42170);
#6868=VERTEX_POINT('',#42318);
#6869=VERTEX_POINT('',#42530);
#6870=VERTEX_POINT('',#42537);
#6871=VERTEX_POINT('',#42612);
#6872=VERTEX_POINT('',#42760);
#6873=VERTEX_POINT('',#42972);
#6874=VERTEX_POINT('',#42979);
#6875=VERTEX_POINT('',#43054);
#6876=VERTEX_POINT('',#43202);
#6877=VERTEX_POINT('',#43414);
#6878=VERTEX_POINT('',#43421);
#6879=VERTEX_POINT('',#43496);
#6880=VERTEX_POINT('',#43644);
#6881=VERTEX_POINT('',#43856);
#6882=VERTEX_POINT('',#43863);
#6883=VERTEX_POINT('',#43938);
#6884=VERTEX_POINT('',#44086);
#6885=VERTEX_POINT('',#44298);
#6886=VERTEX_POINT('',#44305);
#6887=VERTEX_POINT('',#44380);
#6888=VERTEX_POINT('',#44528);
#6889=VERTEX_POINT('',#44740);
#6890=VERTEX_POINT('',#44747);
#6891=VERTEX_POINT('',#44822);
#6892=VERTEX_POINT('',#44970);
#6893=VERTEX_POINT('',#45182);
#6894=VERTEX_POINT('',#45189);
#6895=VERTEX_POINT('',#45264);
#6896=VERTEX_POINT('',#45412);
#6897=VERTEX_POINT('',#45624);
#6898=VERTEX_POINT('',#45631);
#6899=VERTEX_POINT('',#45706);
#6900=VERTEX_POINT('',#45854);
#6901=VERTEX_POINT('',#46066);
#6902=VERTEX_POINT('',#46073);
#6903=VERTEX_POINT('',#46148);
#6904=VERTEX_POINT('',#46296);
#6905=VERTEX_POINT('',#46508);
#6906=VERTEX_POINT('',#46515);
#6907=VERTEX_POINT('',#46590);
#6908=VERTEX_POINT('',#46738);
#6909=VERTEX_POINT('',#46950);
#6910=VERTEX_POINT('',#46957);
#6911=VERTEX_POINT('',#47032);
#6912=VERTEX_POINT('',#47180);
#6913=VERTEX_POINT('',#47392);
#6914=VERTEX_POINT('',#47399);
#6915=VERTEX_POINT('',#47474);
#6916=VERTEX_POINT('',#47622);
#6917=VERTEX_POINT('',#47834);
#6918=VERTEX_POINT('',#47841);
#6919=VERTEX_POINT('',#47916);
#6920=VERTEX_POINT('',#48064);
#6921=VERTEX_POINT('',#48276);
#6922=VERTEX_POINT('',#48283);
#6923=VERTEX_POINT('',#48358);
#6924=VERTEX_POINT('',#48506);
#6925=VERTEX_POINT('',#48718);
#6926=VERTEX_POINT('',#48725);
#6927=VERTEX_POINT('',#48800);
#6928=VERTEX_POINT('',#48948);
#6929=VERTEX_POINT('',#49160);
#6930=VERTEX_POINT('',#49167);
#6931=VERTEX_POINT('',#49242);
#6932=VERTEX_POINT('',#49390);
#6933=VERTEX_POINT('',#49602);
#6934=VERTEX_POINT('',#49609);
#6935=VERTEX_POINT('',#49684);
#6936=VERTEX_POINT('',#49832);
#6937=VERTEX_POINT('',#50044);
#6938=VERTEX_POINT('',#50051);
#6939=VERTEX_POINT('',#50126);
#6940=VERTEX_POINT('',#50274);
#6941=VERTEX_POINT('',#50486);
#6942=VERTEX_POINT('',#50493);
#6943=VERTEX_POINT('',#50568);
#6944=VERTEX_POINT('',#50716);
#6945=VERTEX_POINT('',#50928);
#6946=VERTEX_POINT('',#50935);
#6947=VERTEX_POINT('',#51010);
#6948=VERTEX_POINT('',#51158);
#6949=VERTEX_POINT('',#51370);
#6950=VERTEX_POINT('',#51377);
#6951=VERTEX_POINT('',#51452);
#6952=VERTEX_POINT('',#51600);
#6953=VERTEX_POINT('',#51812);
#6954=VERTEX_POINT('',#51819);
#6955=VERTEX_POINT('',#51894);
#6956=VERTEX_POINT('',#52042);
#6957=VERTEX_POINT('',#52254);
#6958=VERTEX_POINT('',#52261);
#6959=VERTEX_POINT('',#52336);
#6960=VERTEX_POINT('',#52484);
#6961=VERTEX_POINT('',#52696);
#6962=VERTEX_POINT('',#52703);
#6963=VERTEX_POINT('',#52778);
#6964=VERTEX_POINT('',#52926);
#6965=VERTEX_POINT('',#53138);
#6966=VERTEX_POINT('',#53145);
#6967=VERTEX_POINT('',#53220);
#6968=VERTEX_POINT('',#53368);
#6969=VERTEX_POINT('',#53580);
#6970=VERTEX_POINT('',#53587);
#6971=VERTEX_POINT('',#53662);
#6972=VERTEX_POINT('',#53810);
#6973=VERTEX_POINT('',#54022);
#6974=VERTEX_POINT('',#54029);
#6975=VERTEX_POINT('',#54104);
#6976=VERTEX_POINT('',#54252);
#6977=VERTEX_POINT('',#54464);
#6978=VERTEX_POINT('',#54471);
#6979=VERTEX_POINT('',#54546);
#6980=VERTEX_POINT('',#54694);
#6981=VERTEX_POINT('',#54906);
#6982=VERTEX_POINT('',#54913);
#6983=VERTEX_POINT('',#54988);
#6984=VERTEX_POINT('',#55136);
#6985=VERTEX_POINT('',#55348);
#6986=VERTEX_POINT('',#55355);
#6987=VERTEX_POINT('',#55430);
#6988=VERTEX_POINT('',#55578);
#6989=VERTEX_POINT('',#55790);
#6990=VERTEX_POINT('',#55797);
#6991=VERTEX_POINT('',#55872);
#6992=VERTEX_POINT('',#56020);
#6993=VERTEX_POINT('',#56232);
#6994=VERTEX_POINT('',#56239);
#6995=VERTEX_POINT('',#56314);
#6996=VERTEX_POINT('',#56462);
#6997=VERTEX_POINT('',#56674);
#6998=VERTEX_POINT('',#56681);
#6999=VERTEX_POINT('',#56756);
#7000=VERTEX_POINT('',#56904);
#7001=VERTEX_POINT('',#56977);
#7002=VERTEX_POINT('',#57120);
#7003=VERTEX_POINT('',#57198);
#7004=VERTEX_POINT('',#57346);
#7005=VERTEX_POINT('',#57353);
#7006=VERTEX_POINT('',#57565);
#8354=EDGE_CURVE('',#6677,#6678,#4106,.T.);
#8355=EDGE_CURVE('',#6679,#6677,#4107,.T.);
#8356=EDGE_CURVE('',#6680,#6679,#4108,.T.);
#8357=EDGE_CURVE('',#6678,#6680,#4109,.T.);
#8358=EDGE_CURVE('',#6681,#6677,#4110,.T.);
#8359=EDGE_CURVE('',#6681,#6682,#4111,.T.);
#8360=EDGE_CURVE('',#6679,#6682,#4112,.T.);
#8361=EDGE_CURVE('',#6683,#6681,#4113,.T.);
#8362=EDGE_CURVE('',#6684,#6683,#4114,.T.);
#8363=EDGE_CURVE('',#6682,#6684,#4115,.T.);
#8364=EDGE_CURVE('',#6685,#6686,#5690,.T.);
#8365=EDGE_CURVE('',#6686,#6687,#211,.T.);
#8366=EDGE_CURVE('',#6687,#6688,#4116,.T.);
#8367=EDGE_CURVE('',#6688,#6689,#212,.T.);
#8368=EDGE_CURVE('',#6689,#6690,#5691,.T.);
#8369=EDGE_CURVE('',#6690,#6691,#213,.T.);
#8370=EDGE_CURVE('',#6691,#6692,#4117,.T.);
#8371=EDGE_CURVE('',#6692,#6693,#214,.T.);
#8372=EDGE_CURVE('',#6693,#6694,#5692,.T.);
#8373=EDGE_CURVE('',#6694,#6695,#215,.T.);
#8374=EDGE_CURVE('',#6695,#6696,#4118,.T.);
#8375=EDGE_CURVE('',#6696,#6697,#216,.T.);
#8376=EDGE_CURVE('',#6697,#6698,#5693,.T.);
#8377=EDGE_CURVE('',#6698,#6699,#217,.T.);
#8378=EDGE_CURVE('',#6699,#6700,#4119,.T.);
#8379=EDGE_CURVE('',#6700,#6701,#218,.T.);
#8380=EDGE_CURVE('',#6701,#6702,#5694,.T.);
#8381=EDGE_CURVE('',#6702,#6703,#219,.T.);
#8382=EDGE_CURVE('',#6703,#6704,#4120,.T.);
#8383=EDGE_CURVE('',#6704,#6705,#220,.T.);
#8384=EDGE_CURVE('',#6705,#6706,#5695,.T.);
#8385=EDGE_CURVE('',#6706,#6707,#221,.T.);
#8386=EDGE_CURVE('',#6707,#6708,#4121,.T.);
#8387=EDGE_CURVE('',#6708,#6709,#222,.T.);
#8388=EDGE_CURVE('',#6709,#6710,#5696,.T.);
#8389=EDGE_CURVE('',#6710,#6711,#223,.T.);
#8390=EDGE_CURVE('',#6711,#6712,#4122,.T.);
#8391=EDGE_CURVE('',#6712,#6713,#224,.T.);
#8392=EDGE_CURVE('',#6713,#6714,#5697,.T.);
#8393=EDGE_CURVE('',#6714,#6715,#225,.T.);
#8394=EDGE_CURVE('',#6715,#6716,#4123,.T.);
#8395=EDGE_CURVE('',#6716,#6717,#226,.T.);
#8396=EDGE_CURVE('',#6717,#6718,#5698,.T.);
#8397=EDGE_CURVE('',#6718,#6719,#227,.T.);
#8398=EDGE_CURVE('',#6719,#6720,#4124,.T.);
#8399=EDGE_CURVE('',#6720,#6721,#228,.T.);
#8400=EDGE_CURVE('',#6721,#6722,#5699,.T.);
#8401=EDGE_CURVE('',#6722,#6723,#229,.T.);
#8402=EDGE_CURVE('',#6723,#6724,#4125,.T.);
#8403=EDGE_CURVE('',#6724,#6725,#230,.T.);
#8404=EDGE_CURVE('',#6725,#6726,#5700,.T.);
#8405=EDGE_CURVE('',#6726,#6727,#231,.T.);
#8406=EDGE_CURVE('',#6727,#6728,#4126,.T.);
#8407=EDGE_CURVE('',#6728,#6729,#232,.T.);
#8408=EDGE_CURVE('',#6729,#6730,#5701,.T.);
#8409=EDGE_CURVE('',#6730,#6731,#233,.T.);
#8410=EDGE_CURVE('',#6731,#6732,#4127,.T.);
#8411=EDGE_CURVE('',#6732,#6733,#234,.T.);
#8412=EDGE_CURVE('',#6733,#6734,#5702,.T.);
#8413=EDGE_CURVE('',#6734,#6735,#235,.T.);
#8414=EDGE_CURVE('',#6735,#6736,#4128,.T.);
#8415=EDGE_CURVE('',#6736,#6737,#236,.T.);
#8416=EDGE_CURVE('',#6737,#6738,#5703,.T.);
#8417=EDGE_CURVE('',#6738,#6739,#237,.T.);
#8418=EDGE_CURVE('',#6739,#6740,#4129,.T.);
#8419=EDGE_CURVE('',#6740,#6741,#238,.T.);
#8420=EDGE_CURVE('',#6741,#6742,#5704,.T.);
#8421=EDGE_CURVE('',#6742,#6743,#239,.T.);
#8422=EDGE_CURVE('',#6743,#6744,#4130,.T.);
#8423=EDGE_CURVE('',#6744,#6745,#240,.T.);
#8424=EDGE_CURVE('',#6745,#6746,#5705,.T.);
#8425=EDGE_CURVE('',#6746,#6747,#241,.T.);
#8426=EDGE_CURVE('',#6747,#6748,#4131,.T.);
#8427=EDGE_CURVE('',#6748,#6749,#242,.T.);
#8428=EDGE_CURVE('',#6749,#6750,#5706,.T.);
#8429=EDGE_CURVE('',#6750,#6751,#243,.T.);
#8430=EDGE_CURVE('',#6751,#6752,#4132,.T.);
#8431=EDGE_CURVE('',#6752,#6753,#244,.T.);
#8432=EDGE_CURVE('',#6753,#6754,#5707,.T.);
#8433=EDGE_CURVE('',#6754,#6755,#245,.T.);
#8434=EDGE_CURVE('',#6755,#6756,#4133,.T.);
#8435=EDGE_CURVE('',#6756,#6757,#246,.T.);
#8436=EDGE_CURVE('',#6757,#6758,#5708,.T.);
#8437=EDGE_CURVE('',#6758,#6759,#247,.T.);
#8438=EDGE_CURVE('',#6759,#6760,#4134,.T.);
#8439=EDGE_CURVE('',#6760,#6761,#248,.T.);
#8440=EDGE_CURVE('',#6761,#6762,#5709,.T.);
#8441=EDGE_CURVE('',#6762,#6763,#249,.T.);
#8442=EDGE_CURVE('',#6763,#6764,#4135,.T.);
#8443=EDGE_CURVE('',#6764,#6765,#250,.T.);
#8444=EDGE_CURVE('',#6765,#6766,#5710,.T.);
#8445=EDGE_CURVE('',#6766,#6767,#251,.T.);
#8446=EDGE_CURVE('',#6767,#6768,#4136,.T.);
#8447=EDGE_CURVE('',#6768,#6769,#252,.T.);
#8448=EDGE_CURVE('',#6769,#6770,#5711,.T.);
#8449=EDGE_CURVE('',#6770,#6771,#253,.T.);
#8450=EDGE_CURVE('',#6771,#6772,#4137,.T.);
#8451=EDGE_CURVE('',#6772,#6773,#254,.T.);
#8452=EDGE_CURVE('',#6773,#6774,#5712,.T.);
#8453=EDGE_CURVE('',#6774,#6775,#255,.T.);
#8454=EDGE_CURVE('',#6775,#6776,#4138,.T.);
#8455=EDGE_CURVE('',#6776,#6777,#256,.T.);
#8456=EDGE_CURVE('',#6777,#6778,#5713,.T.);
#8457=EDGE_CURVE('',#6778,#6779,#257,.T.);
#8458=EDGE_CURVE('',#6779,#6780,#4139,.T.);
#8459=EDGE_CURVE('',#6780,#6781,#258,.T.);
#8460=EDGE_CURVE('',#6781,#6782,#5714,.T.);
#8461=EDGE_CURVE('',#6782,#6783,#259,.T.);
#8462=EDGE_CURVE('',#6783,#6784,#4140,.T.);
#8463=EDGE_CURVE('',#6784,#6785,#260,.T.);
#8464=EDGE_CURVE('',#6785,#6786,#5715,.T.);
#8465=EDGE_CURVE('',#6786,#6787,#261,.T.);
#8466=EDGE_CURVE('',#6787,#6788,#4141,.T.);
#8467=EDGE_CURVE('',#6788,#6789,#262,.T.);
#8468=EDGE_CURVE('',#6789,#6790,#5716,.T.);
#8469=EDGE_CURVE('',#6790,#6791,#263,.T.);
#8470=EDGE_CURVE('',#6791,#6792,#4142,.T.);
#8471=EDGE_CURVE('',#6792,#6793,#264,.T.);
#8472=EDGE_CURVE('',#6793,#6794,#5717,.T.);
#8473=EDGE_CURVE('',#6794,#6795,#265,.T.);
#8474=EDGE_CURVE('',#6795,#6796,#4143,.T.);
#8475=EDGE_CURVE('',#6796,#6797,#266,.T.);
#8476=EDGE_CURVE('',#6797,#6798,#5718,.T.);
#8477=EDGE_CURVE('',#6798,#6799,#267,.T.);
#8478=EDGE_CURVE('',#6799,#6800,#4144,.T.);
#8479=EDGE_CURVE('',#6800,#6801,#268,.T.);
#8480=EDGE_CURVE('',#6801,#6802,#5719,.T.);
#8481=EDGE_CURVE('',#6802,#6803,#269,.T.);
#8482=EDGE_CURVE('',#6803,#6804,#4145,.T.);
#8483=EDGE_CURVE('',#6804,#6805,#270,.T.);
#8484=EDGE_CURVE('',#6805,#6806,#5720,.T.);
#8485=EDGE_CURVE('',#6806,#6807,#271,.T.);
#8486=EDGE_CURVE('',#6807,#6808,#4146,.T.);
#8487=EDGE_CURVE('',#6808,#6809,#272,.T.);
#8488=EDGE_CURVE('',#6809,#6810,#5721,.T.);
#8489=EDGE_CURVE('',#6810,#6811,#273,.T.);
#8490=EDGE_CURVE('',#6811,#6812,#4147,.T.);
#8491=EDGE_CURVE('',#6812,#6813,#274,.T.);
#8492=EDGE_CURVE('',#6813,#6814,#5722,.T.);
#8493=EDGE_CURVE('',#6814,#6815,#275,.T.);
#8494=EDGE_CURVE('',#6815,#6816,#4148,.T.);
#8495=EDGE_CURVE('',#6816,#6817,#276,.T.);
#8496=EDGE_CURVE('',#6817,#6818,#5723,.T.);
#8497=EDGE_CURVE('',#6818,#6819,#277,.T.);
#8498=EDGE_CURVE('',#6819,#6820,#4149,.T.);
#8499=EDGE_CURVE('',#6820,#6821,#278,.T.);
#8500=EDGE_CURVE('',#6821,#6822,#5724,.T.);
#8501=EDGE_CURVE('',#6822,#6823,#279,.T.);
#8502=EDGE_CURVE('',#6823,#6824,#4150,.T.);
#8503=EDGE_CURVE('',#6824,#6825,#280,.T.);
#8504=EDGE_CURVE('',#6825,#6826,#5725,.T.);
#8505=EDGE_CURVE('',#6826,#6827,#281,.T.);
#8506=EDGE_CURVE('',#6827,#6828,#4151,.T.);
#8507=EDGE_CURVE('',#6828,#6829,#282,.T.);
#8508=EDGE_CURVE('',#6829,#6830,#5726,.T.);
#8509=EDGE_CURVE('',#6830,#6831,#283,.T.);
#8510=EDGE_CURVE('',#6831,#6832,#4152,.T.);
#8511=EDGE_CURVE('',#6832,#6833,#284,.T.);
#8512=EDGE_CURVE('',#6833,#6834,#5727,.T.);
#8513=EDGE_CURVE('',#6834,#6835,#285,.T.);
#8514=EDGE_CURVE('',#6835,#6836,#4153,.T.);
#8515=EDGE_CURVE('',#6836,#6837,#286,.T.);
#8516=EDGE_CURVE('',#6837,#6838,#5728,.T.);
#8517=EDGE_CURVE('',#6838,#6839,#287,.T.);
#8518=EDGE_CURVE('',#6839,#6840,#4154,.T.);
#8519=EDGE_CURVE('',#6840,#6841,#288,.T.);
#8520=EDGE_CURVE('',#6841,#6842,#5729,.T.);
#8521=EDGE_CURVE('',#6842,#6843,#289,.T.);
#8522=EDGE_CURVE('',#6843,#6844,#4155,.T.);
#8523=EDGE_CURVE('',#6844,#6685,#290,.T.);
#8524=EDGE_CURVE('',#6684,#6680,#5730,.T.);
#8525=EDGE_CURVE('',#6678,#6683,#5731,.T.);
#8526=EDGE_CURVE('',#6845,#6845,#5732,.T.);
#8527=EDGE_CURVE('',#6845,#6846,#4156,.T.);
#8528=EDGE_CURVE('',#6846,#6846,#5733,.T.);
#8529=EDGE_CURVE('',#6847,#6842,#836,.T.);
#8530=EDGE_CURVE('',#6848,#6847,#291,.T.);
#8531=EDGE_CURVE('',#6843,#6848,#4157,.T.);
#8532=EDGE_CURVE('',#6685,#6849,#837,.T.);
#8533=EDGE_CURVE('',#6844,#6850,#4158,.T.);
#8534=EDGE_CURVE('',#6849,#6850,#292,.T.);
#8535=EDGE_CURVE('',#6850,#6848,#4159,.T.);
#8536=EDGE_CURVE('',#6851,#6849,#5734,.T.);
#8537=EDGE_CURVE('',#6851,#6686,#838,.T.);
#8538=EDGE_CURVE('',#6852,#6851,#293,.T.);
#8539=EDGE_CURVE('',#6687,#6852,#4160,.T.);
#8540=EDGE_CURVE('',#6689,#6853,#839,.T.);
#8541=EDGE_CURVE('',#6688,#6854,#4161,.T.);
#8542=EDGE_CURVE('',#6853,#6854,#294,.T.);
#8543=EDGE_CURVE('',#6854,#6852,#4162,.T.);
#8544=EDGE_CURVE('',#6855,#6853,#5735,.T.);
#8545=EDGE_CURVE('',#6855,#6690,#840,.T.);
#8546=EDGE_CURVE('',#6856,#6855,#295,.T.);
#8547=EDGE_CURVE('',#6691,#6856,#4163,.T.);
#8548=EDGE_CURVE('',#6693,#6857,#841,.T.);
#8549=EDGE_CURVE('',#6692,#6858,#4164,.T.);
#8550=EDGE_CURVE('',#6857,#6858,#296,.T.);
#8551=EDGE_CURVE('',#6858,#6856,#4165,.T.);
#8552=EDGE_CURVE('',#6859,#6857,#5736,.T.);
#8553=EDGE_CURVE('',#6859,#6694,#842,.T.);
#8554=EDGE_CURVE('',#6860,#6859,#297,.T.);
#8555=EDGE_CURVE('',#6695,#6860,#4166,.T.);
#8556=EDGE_CURVE('',#6697,#6861,#843,.T.);
#8557=EDGE_CURVE('',#6696,#6862,#4167,.T.);
#8558=EDGE_CURVE('',#6861,#6862,#298,.T.);
#8559=EDGE_CURVE('',#6862,#6860,#4168,.T.);
#8560=EDGE_CURVE('',#6863,#6861,#5737,.T.);
#8561=EDGE_CURVE('',#6863,#6698,#844,.T.);
#8562=EDGE_CURVE('',#6864,#6863,#299,.T.);
#8563=EDGE_CURVE('',#6699,#6864,#4169,.T.);
#8564=EDGE_CURVE('',#6701,#6865,#845,.T.);
#8565=EDGE_CURVE('',#6700,#6866,#4170,.T.);
#8566=EDGE_CURVE('',#6865,#6866,#300,.T.);
#8567=EDGE_CURVE('',#6866,#6864,#4171,.T.);
#8568=EDGE_CURVE('',#6867,#6865,#5738,.T.);
#8569=EDGE_CURVE('',#6867,#6702,#846,.T.);
#8570=EDGE_CURVE('',#6868,#6867,#301,.T.);
#8571=EDGE_CURVE('',#6703,#6868,#4172,.T.);
#8572=EDGE_CURVE('',#6705,#6869,#847,.T.);
#8573=EDGE_CURVE('',#6704,#6870,#4173,.T.);
#8574=EDGE_CURVE('',#6869,#6870,#302,.T.);
#8575=EDGE_CURVE('',#6870,#6868,#4174,.T.);
#8576=EDGE_CURVE('',#6871,#6869,#5739,.T.);
#8577=EDGE_CURVE('',#6871,#6706,#848,.T.);
#8578=EDGE_CURVE('',#6872,#6871,#303,.T.);
#8579=EDGE_CURVE('',#6707,#6872,#4175,.T.);
#8580=EDGE_CURVE('',#6709,#6873,#849,.T.);
#8581=EDGE_CURVE('',#6708,#6874,#4176,.T.);
#8582=EDGE_CURVE('',#6873,#6874,#304,.T.);
#8583=EDGE_CURVE('',#6874,#6872,#4177,.T.);
#8584=EDGE_CURVE('',#6875,#6873,#5740,.T.);
#8585=EDGE_CURVE('',#6875,#6710,#850,.T.);
#8586=EDGE_CURVE('',#6876,#6875,#305,.T.);
#8587=EDGE_CURVE('',#6711,#6876,#4178,.T.);
#8588=EDGE_CURVE('',#6713,#6877,#851,.T.);
#8589=EDGE_CURVE('',#6712,#6878,#4179,.T.);
#8590=EDGE_CURVE('',#6877,#6878,#306,.T.);
#8591=EDGE_CURVE('',#6878,#6876,#4180,.T.);
#8592=EDGE_CURVE('',#6879,#6877,#5741,.T.);
#8593=EDGE_CURVE('',#6879,#6714,#852,.T.);
#8594=EDGE_CURVE('',#6880,#6879,#307,.T.);
#8595=EDGE_CURVE('',#6715,#6880,#4181,.T.);
#8596=EDGE_CURVE('',#6717,#6881,#853,.T.);
#8597=EDGE_CURVE('',#6716,#6882,#4182,.T.);
#8598=EDGE_CURVE('',#6881,#6882,#308,.T.);
#8599=EDGE_CURVE('',#6882,#6880,#4183,.T.);
#8600=EDGE_CURVE('',#6883,#6881,#5742,.T.);
#8601=EDGE_CURVE('',#6883,#6718,#854,.T.);
#8602=EDGE_CURVE('',#6884,#6883,#309,.T.);
#8603=EDGE_CURVE('',#6719,#6884,#4184,.T.);
#8604=EDGE_CURVE('',#6721,#6885,#855,.T.);
#8605=EDGE_CURVE('',#6720,#6886,#4185,.T.);
#8606=EDGE_CURVE('',#6885,#6886,#310,.T.);
#8607=EDGE_CURVE('',#6886,#6884,#4186,.T.);
#8608=EDGE_CURVE('',#6887,#6885,#5743,.T.);
#8609=EDGE_CURVE('',#6887,#6722,#856,.T.);
#8610=EDGE_CURVE('',#6888,#6887,#311,.T.);
#8611=EDGE_CURVE('',#6723,#6888,#4187,.T.);
#8612=EDGE_CURVE('',#6725,#6889,#857,.T.);
#8613=EDGE_CURVE('',#6724,#6890,#4188,.T.);
#8614=EDGE_CURVE('',#6889,#6890,#312,.T.);
#8615=EDGE_CURVE('',#6890,#6888,#4189,.T.);
#8616=EDGE_CURVE('',#6891,#6889,#5744,.T.);
#8617=EDGE_CURVE('',#6891,#6726,#858,.T.);
#8618=EDGE_CURVE('',#6892,#6891,#313,.T.);
#8619=EDGE_CURVE('',#6727,#6892,#4190,.T.);
#8620=EDGE_CURVE('',#6729,#6893,#859,.T.);
#8621=EDGE_CURVE('',#6728,#6894,#4191,.T.);
#8622=EDGE_CURVE('',#6893,#6894,#314,.T.);
#8623=EDGE_CURVE('',#6894,#6892,#4192,.T.);
#8624=EDGE_CURVE('',#6895,#6893,#5745,.T.);
#8625=EDGE_CURVE('',#6895,#6730,#860,.T.);
#8626=EDGE_CURVE('',#6896,#6895,#315,.T.);
#8627=EDGE_CURVE('',#6731,#6896,#4193,.T.);
#8628=EDGE_CURVE('',#6733,#6897,#861,.T.);
#8629=EDGE_CURVE('',#6732,#6898,#4194,.T.);
#8630=EDGE_CURVE('',#6897,#6898,#316,.T.);
#8631=EDGE_CURVE('',#6898,#6896,#4195,.T.);
#8632=EDGE_CURVE('',#6899,#6897,#5746,.T.);
#8633=EDGE_CURVE('',#6899,#6734,#862,.T.);
#8634=EDGE_CURVE('',#6900,#6899,#317,.T.);
#8635=EDGE_CURVE('',#6735,#6900,#4196,.T.);
#8636=EDGE_CURVE('',#6737,#6901,#863,.T.);
#8637=EDGE_CURVE('',#6736,#6902,#4197,.T.);
#8638=EDGE_CURVE('',#6901,#6902,#318,.T.);
#8639=EDGE_CURVE('',#6902,#6900,#4198,.T.);
#8640=EDGE_CURVE('',#6903,#6901,#5747,.T.);
#8641=EDGE_CURVE('',#6903,#6738,#864,.T.);
#8642=EDGE_CURVE('',#6904,#6903,#319,.T.);
#8643=EDGE_CURVE('',#6739,#6904,#4199,.T.);
#8644=EDGE_CURVE('',#6741,#6905,#865,.T.);
#8645=EDGE_CURVE('',#6740,#6906,#4200,.T.);
#8646=EDGE_CURVE('',#6905,#6906,#320,.T.);
#8647=EDGE_CURVE('',#6906,#6904,#4201,.T.);
#8648=EDGE_CURVE('',#6907,#6905,#5748,.T.);
#8649=EDGE_CURVE('',#6907,#6742,#866,.T.);
#8650=EDGE_CURVE('',#6908,#6907,#321,.T.);
#8651=EDGE_CURVE('',#6743,#6908,#4202,.T.);
#8652=EDGE_CURVE('',#6745,#6909,#867,.T.);
#8653=EDGE_CURVE('',#6744,#6910,#4203,.T.);
#8654=EDGE_CURVE('',#6909,#6910,#322,.T.);
#8655=EDGE_CURVE('',#6910,#6908,#4204,.T.);
#8656=EDGE_CURVE('',#6911,#6909,#5749,.T.);
#8657=EDGE_CURVE('',#6911,#6746,#868,.T.);
#8658=EDGE_CURVE('',#6912,#6911,#323,.T.);
#8659=EDGE_CURVE('',#6747,#6912,#4205,.T.);
#8660=EDGE_CURVE('',#6749,#6913,#869,.T.);
#8661=EDGE_CURVE('',#6748,#6914,#4206,.T.);
#8662=EDGE_CURVE('',#6913,#6914,#324,.T.);
#8663=EDGE_CURVE('',#6914,#6912,#4207,.T.);
#8664=EDGE_CURVE('',#6915,#6913,#5750,.T.);
#8665=EDGE_CURVE('',#6915,#6750,#870,.T.);
#8666=EDGE_CURVE('',#6916,#6915,#325,.T.);
#8667=EDGE_CURVE('',#6751,#6916,#4208,.T.);
#8668=EDGE_CURVE('',#6753,#6917,#871,.T.);
#8669=EDGE_CURVE('',#6752,#6918,#4209,.T.);
#8670=EDGE_CURVE('',#6917,#6918,#326,.T.);
#8671=EDGE_CURVE('',#6918,#6916,#4210,.T.);
#8672=EDGE_CURVE('',#6919,#6917,#5751,.T.);
#8673=EDGE_CURVE('',#6919,#6754,#872,.T.);
#8674=EDGE_CURVE('',#6920,#6919,#327,.T.);
#8675=EDGE_CURVE('',#6755,#6920,#4211,.T.);
#8676=EDGE_CURVE('',#6757,#6921,#873,.T.);
#8677=EDGE_CURVE('',#6756,#6922,#4212,.T.);
#8678=EDGE_CURVE('',#6921,#6922,#328,.T.);
#8679=EDGE_CURVE('',#6922,#6920,#4213,.T.);
#8680=EDGE_CURVE('',#6923,#6921,#5752,.T.);
#8681=EDGE_CURVE('',#6923,#6758,#874,.T.);
#8682=EDGE_CURVE('',#6924,#6923,#329,.T.);
#8683=EDGE_CURVE('',#6759,#6924,#4214,.T.);
#8684=EDGE_CURVE('',#6761,#6925,#875,.T.);
#8685=EDGE_CURVE('',#6760,#6926,#4215,.T.);
#8686=EDGE_CURVE('',#6925,#6926,#330,.T.);
#8687=EDGE_CURVE('',#6926,#6924,#4216,.T.);
#8688=EDGE_CURVE('',#6927,#6925,#5753,.T.);
#8689=EDGE_CURVE('',#6927,#6762,#876,.T.);
#8690=EDGE_CURVE('',#6928,#6927,#331,.T.);
#8691=EDGE_CURVE('',#6763,#6928,#4217,.T.);
#8692=EDGE_CURVE('',#6765,#6929,#877,.T.);
#8693=EDGE_CURVE('',#6764,#6930,#4218,.T.);
#8694=EDGE_CURVE('',#6929,#6930,#332,.T.);
#8695=EDGE_CURVE('',#6930,#6928,#4219,.T.);
#8696=EDGE_CURVE('',#6931,#6929,#5754,.T.);
#8697=EDGE_CURVE('',#6931,#6766,#878,.T.);
#8698=EDGE_CURVE('',#6932,#6931,#333,.T.);
#8699=EDGE_CURVE('',#6767,#6932,#4220,.T.);
#8700=EDGE_CURVE('',#6769,#6933,#879,.T.);
#8701=EDGE_CURVE('',#6768,#6934,#4221,.T.);
#8702=EDGE_CURVE('',#6933,#6934,#334,.T.);
#8703=EDGE_CURVE('',#6934,#6932,#4222,.T.);
#8704=EDGE_CURVE('',#6935,#6933,#5755,.T.);
#8705=EDGE_CURVE('',#6935,#6770,#880,.T.);
#8706=EDGE_CURVE('',#6936,#6935,#335,.T.);
#8707=EDGE_CURVE('',#6771,#6936,#4223,.T.);
#8708=EDGE_CURVE('',#6773,#6937,#881,.T.);
#8709=EDGE_CURVE('',#6772,#6938,#4224,.T.);
#8710=EDGE_CURVE('',#6937,#6938,#336,.T.);
#8711=EDGE_CURVE('',#6938,#6936,#4225,.T.);
#8712=EDGE_CURVE('',#6939,#6937,#5756,.T.);
#8713=EDGE_CURVE('',#6939,#6774,#882,.T.);
#8714=EDGE_CURVE('',#6940,#6939,#337,.T.);
#8715=EDGE_CURVE('',#6775,#6940,#4226,.T.);
#8716=EDGE_CURVE('',#6777,#6941,#883,.T.);
#8717=EDGE_CURVE('',#6776,#6942,#4227,.T.);
#8718=EDGE_CURVE('',#6941,#6942,#338,.T.);
#8719=EDGE_CURVE('',#6942,#6940,#4228,.T.);
#8720=EDGE_CURVE('',#6943,#6941,#5757,.T.);
#8721=EDGE_CURVE('',#6943,#6778,#884,.T.);
#8722=EDGE_CURVE('',#6944,#6943,#339,.T.);
#8723=EDGE_CURVE('',#6779,#6944,#4229,.T.);
#8724=EDGE_CURVE('',#6781,#6945,#885,.T.);
#8725=EDGE_CURVE('',#6780,#6946,#4230,.T.);
#8726=EDGE_CURVE('',#6945,#6946,#340,.T.);
#8727=EDGE_CURVE('',#6946,#6944,#4231,.T.);
#8728=EDGE_CURVE('',#6947,#6945,#5758,.T.);
#8729=EDGE_CURVE('',#6947,#6782,#886,.T.);
#8730=EDGE_CURVE('',#6948,#6947,#341,.T.);
#8731=EDGE_CURVE('',#6783,#6948,#4232,.T.);
#8732=EDGE_CURVE('',#6785,#6949,#887,.T.);
#8733=EDGE_CURVE('',#6784,#6950,#4233,.T.);
#8734=EDGE_CURVE('',#6949,#6950,#342,.T.);
#8735=EDGE_CURVE('',#6950,#6948,#4234,.T.);
#8736=EDGE_CURVE('',#6951,#6949,#5759,.T.);
#8737=EDGE_CURVE('',#6951,#6786,#888,.T.);
#8738=EDGE_CURVE('',#6952,#6951,#343,.T.);
#8739=EDGE_CURVE('',#6787,#6952,#4235,.T.);
#8740=EDGE_CURVE('',#6789,#6953,#889,.T.);
#8741=EDGE_CURVE('',#6788,#6954,#4236,.T.);
#8742=EDGE_CURVE('',#6953,#6954,#344,.T.);
#8743=EDGE_CURVE('',#6954,#6952,#4237,.T.);
#8744=EDGE_CURVE('',#6955,#6953,#5760,.T.);
#8745=EDGE_CURVE('',#6955,#6790,#890,.T.);
#8746=EDGE_CURVE('',#6956,#6955,#345,.T.);
#8747=EDGE_CURVE('',#6791,#6956,#4238,.T.);
#8748=EDGE_CURVE('',#6793,#6957,#891,.T.);
#8749=EDGE_CURVE('',#6792,#6958,#4239,.T.);
#8750=EDGE_CURVE('',#6957,#6958,#346,.T.);
#8751=EDGE_CURVE('',#6958,#6956,#4240,.T.);
#8752=EDGE_CURVE('',#6959,#6957,#5761,.T.);
#8753=EDGE_CURVE('',#6959,#6794,#892,.T.);
#8754=EDGE_CURVE('',#6960,#6959,#347,.T.);
#8755=EDGE_CURVE('',#6795,#6960,#4241,.T.);
#8756=EDGE_CURVE('',#6797,#6961,#893,.T.);
#8757=EDGE_CURVE('',#6796,#6962,#4242,.T.);
#8758=EDGE_CURVE('',#6961,#6962,#348,.T.);
#8759=EDGE_CURVE('',#6962,#6960,#4243,.T.);
#8760=EDGE_CURVE('',#6963,#6961,#5762,.T.);
#8761=EDGE_CURVE('',#6963,#6798,#894,.T.);
#8762=EDGE_CURVE('',#6964,#6963,#349,.T.);
#8763=EDGE_CURVE('',#6799,#6964,#4244,.T.);
#8764=EDGE_CURVE('',#6801,#6965,#895,.T.);
#8765=EDGE_CURVE('',#6800,#6966,#4245,.T.);
#8766=EDGE_CURVE('',#6965,#6966,#350,.T.);
#8767=EDGE_CURVE('',#6966,#6964,#4246,.T.);
#8768=EDGE_CURVE('',#6967,#6965,#5763,.T.);
#8769=EDGE_CURVE('',#6967,#6802,#896,.T.);
#8770=EDGE_CURVE('',#6968,#6967,#351,.T.);
#8771=EDGE_CURVE('',#6803,#6968,#4247,.T.);
#8772=EDGE_CURVE('',#6805,#6969,#897,.T.);
#8773=EDGE_CURVE('',#6804,#6970,#4248,.T.);
#8774=EDGE_CURVE('',#6969,#6970,#352,.T.);
#8775=EDGE_CURVE('',#6970,#6968,#4249,.T.);
#8776=EDGE_CURVE('',#6971,#6969,#5764,.T.);
#8777=EDGE_CURVE('',#6971,#6806,#898,.T.);
#8778=EDGE_CURVE('',#6972,#6971,#353,.T.);
#8779=EDGE_CURVE('',#6807,#6972,#4250,.T.);
#8780=EDGE_CURVE('',#6809,#6973,#899,.T.);
#8781=EDGE_CURVE('',#6808,#6974,#4251,.T.);
#8782=EDGE_CURVE('',#6973,#6974,#354,.T.);
#8783=EDGE_CURVE('',#6974,#6972,#4252,.T.);
#8784=EDGE_CURVE('',#6975,#6973,#5765,.T.);
#8785=EDGE_CURVE('',#6975,#6810,#900,.T.);
#8786=EDGE_CURVE('',#6976,#6975,#355,.T.);
#8787=EDGE_CURVE('',#6811,#6976,#4253,.T.);
#8788=EDGE_CURVE('',#6813,#6977,#901,.T.);
#8789=EDGE_CURVE('',#6812,#6978,#4254,.T.);
#8790=EDGE_CURVE('',#6977,#6978,#356,.T.);
#8791=EDGE_CURVE('',#6978,#6976,#4255,.T.);
#8792=EDGE_CURVE('',#6979,#6977,#5766,.T.);
#8793=EDGE_CURVE('',#6979,#6814,#902,.T.);
#8794=EDGE_CURVE('',#6980,#6979,#357,.T.);
#8795=EDGE_CURVE('',#6815,#6980,#4256,.T.);
#8796=EDGE_CURVE('',#6817,#6981,#903,.T.);
#8797=EDGE_CURVE('',#6816,#6982,#4257,.T.);
#8798=EDGE_CURVE('',#6981,#6982,#358,.T.);
#8799=EDGE_CURVE('',#6982,#6980,#4258,.T.);
#8800=EDGE_CURVE('',#6983,#6981,#5767,.T.);
#8801=EDGE_CURVE('',#6983,#6818,#904,.T.);
#8802=EDGE_CURVE('',#6984,#6983,#359,.T.);
#8803=EDGE_CURVE('',#6819,#6984,#4259,.T.);
#8804=EDGE_CURVE('',#6821,#6985,#905,.T.);
#8805=EDGE_CURVE('',#6820,#6986,#4260,.T.);
#8806=EDGE_CURVE('',#6985,#6986,#360,.T.);
#8807=EDGE_CURVE('',#6986,#6984,#4261,.T.);
#8808=EDGE_CURVE('',#6987,#6985,#5768,.T.);
#8809=EDGE_CURVE('',#6987,#6822,#906,.T.);
#8810=EDGE_CURVE('',#6988,#6987,#361,.T.);
#8811=EDGE_CURVE('',#6823,#6988,#4262,.T.);
#8812=EDGE_CURVE('',#6825,#6989,#907,.T.);
#8813=EDGE_CURVE('',#6824,#6990,#4263,.T.);
#8814=EDGE_CURVE('',#6989,#6990,#362,.T.);
#8815=EDGE_CURVE('',#6990,#6988,#4264,.T.);
#8816=EDGE_CURVE('',#6991,#6989,#5769,.T.);
#8817=EDGE_CURVE('',#6991,#6826,#908,.T.);
#8818=EDGE_CURVE('',#6992,#6991,#363,.T.);
#8819=EDGE_CURVE('',#6827,#6992,#4265,.T.);
#8820=EDGE_CURVE('',#6829,#6993,#909,.T.);
#8821=EDGE_CURVE('',#6828,#6994,#4266,.T.);
#8822=EDGE_CURVE('',#6993,#6994,#364,.T.);
#8823=EDGE_CURVE('',#6994,#6992,#4267,.T.);
#8824=EDGE_CURVE('',#6995,#6993,#5770,.T.);
#8825=EDGE_CURVE('',#6995,#6830,#910,.T.);
#8826=EDGE_CURVE('',#6996,#6995,#365,.T.);
#8827=EDGE_CURVE('',#6831,#6996,#4268,.T.);
#8828=EDGE_CURVE('',#6833,#6997,#911,.T.);
#8829=EDGE_CURVE('',#6832,#6998,#4269,.T.);
#8830=EDGE_CURVE('',#6997,#6998,#366,.T.);
#8831=EDGE_CURVE('',#6998,#6996,#4270,.T.);
#8832=EDGE_CURVE('',#6999,#6997,#5771,.T.);
#8833=EDGE_CURVE('',#6999,#6834,#912,.T.);
#8834=EDGE_CURVE('',#7000,#6999,#367,.T.);
#8835=EDGE_CURVE('',#6835,#7000,#4271,.T.);
#8836=EDGE_CURVE('',#7001,#7000,#4272,.T.);
#8837=EDGE_CURVE('',#6836,#7001,#4273,.T.);
#8838=EDGE_CURVE('',#6837,#7002,#913,.T.);
#8839=EDGE_CURVE('',#7002,#7001,#368,.T.);
#8840=EDGE_CURVE('',#7003,#7002,#5772,.T.);
#8841=EDGE_CURVE('',#7003,#6838,#914,.T.);
#8842=EDGE_CURVE('',#6841,#7004,#915,.T.);
#8843=EDGE_CURVE('',#6840,#7005,#4274,.T.);
#8844=EDGE_CURVE('',#7004,#7005,#369,.T.);
#8845=EDGE_CURVE('',#7006,#7003,#370,.T.);
#8846=EDGE_CURVE('',#6839,#7006,#4275,.T.);
#8847=EDGE_CURVE('',#7005,#7006,#4276,.T.);
#8848=EDGE_CURVE('',#6847,#7004,#5773,.T.);
#11535=ORIENTED_EDGE('',*,*,#8354,.F.);
#11536=ORIENTED_EDGE('',*,*,#8355,.F.);
#11537=ORIENTED_EDGE('',*,*,#8356,.F.);
#11538=ORIENTED_EDGE('',*,*,#8357,.F.);
#11539=ORIENTED_EDGE('',*,*,#8358,.F.);
#11540=ORIENTED_EDGE('',*,*,#8359,.T.);
#11541=ORIENTED_EDGE('',*,*,#8360,.F.);
#11542=ORIENTED_EDGE('',*,*,#8355,.T.);
#11543=ORIENTED_EDGE('',*,*,#8361,.F.);
#11544=ORIENTED_EDGE('',*,*,#8362,.F.);
#11545=ORIENTED_EDGE('',*,*,#8363,.F.);
#11546=ORIENTED_EDGE('',*,*,#8359,.F.);
#11547=ORIENTED_EDGE('',*,*,#8364,.T.);
#11548=ORIENTED_EDGE('',*,*,#8365,.T.);
#11549=ORIENTED_EDGE('',*,*,#8366,.T.);
#11550=ORIENTED_EDGE('',*,*,#8367,.T.);
#11551=ORIENTED_EDGE('',*,*,#8368,.T.);
#11552=ORIENTED_EDGE('',*,*,#8369,.T.);
#11553=ORIENTED_EDGE('',*,*,#8370,.T.);
#11554=ORIENTED_EDGE('',*,*,#8371,.T.);
#11555=ORIENTED_EDGE('',*,*,#8372,.T.);
#11556=ORIENTED_EDGE('',*,*,#8373,.T.);
#11557=ORIENTED_EDGE('',*,*,#8374,.T.);
#11558=ORIENTED_EDGE('',*,*,#8375,.T.);
#11559=ORIENTED_EDGE('',*,*,#8376,.T.);
#11560=ORIENTED_EDGE('',*,*,#8377,.T.);
#11561=ORIENTED_EDGE('',*,*,#8378,.T.);
#11562=ORIENTED_EDGE('',*,*,#8379,.T.);
#11563=ORIENTED_EDGE('',*,*,#8380,.T.);
#11564=ORIENTED_EDGE('',*,*,#8381,.T.);
#11565=ORIENTED_EDGE('',*,*,#8382,.T.);
#11566=ORIENTED_EDGE('',*,*,#8383,.T.);
#11567=ORIENTED_EDGE('',*,*,#8384,.T.);
#11568=ORIENTED_EDGE('',*,*,#8385,.T.);
#11569=ORIENTED_EDGE('',*,*,#8386,.T.);
#11570=ORIENTED_EDGE('',*,*,#8387,.T.);
#11571=ORIENTED_EDGE('',*,*,#8388,.T.);
#11572=ORIENTED_EDGE('',*,*,#8389,.T.);
#11573=ORIENTED_EDGE('',*,*,#8390,.T.);
#11574=ORIENTED_EDGE('',*,*,#8391,.T.);
#11575=ORIENTED_EDGE('',*,*,#8392,.T.);
#11576=ORIENTED_EDGE('',*,*,#8393,.T.);
#11577=ORIENTED_EDGE('',*,*,#8394,.T.);
#11578=ORIENTED_EDGE('',*,*,#8395,.T.);
#11579=ORIENTED_EDGE('',*,*,#8396,.T.);
#11580=ORIENTED_EDGE('',*,*,#8397,.T.);
#11581=ORIENTED_EDGE('',*,*,#8398,.T.);
#11582=ORIENTED_EDGE('',*,*,#8399,.T.);
#11583=ORIENTED_EDGE('',*,*,#8400,.T.);
#11584=ORIENTED_EDGE('',*,*,#8401,.T.);
#11585=ORIENTED_EDGE('',*,*,#8402,.T.);
#11586=ORIENTED_EDGE('',*,*,#8403,.T.);
#11587=ORIENTED_EDGE('',*,*,#8404,.T.);
#11588=ORIENTED_EDGE('',*,*,#8405,.T.);
#11589=ORIENTED_EDGE('',*,*,#8406,.T.);
#11590=ORIENTED_EDGE('',*,*,#8407,.T.);
#11591=ORIENTED_EDGE('',*,*,#8408,.T.);
#11592=ORIENTED_EDGE('',*,*,#8409,.T.);
#11593=ORIENTED_EDGE('',*,*,#8410,.T.);
#11594=ORIENTED_EDGE('',*,*,#8411,.T.);
#11595=ORIENTED_EDGE('',*,*,#8412,.T.);
#11596=ORIENTED_EDGE('',*,*,#8413,.T.);
#11597=ORIENTED_EDGE('',*,*,#8414,.T.);
#11598=ORIENTED_EDGE('',*,*,#8415,.T.);
#11599=ORIENTED_EDGE('',*,*,#8416,.T.);
#11600=ORIENTED_EDGE('',*,*,#8417,.T.);
#11601=ORIENTED_EDGE('',*,*,#8418,.T.);
#11602=ORIENTED_EDGE('',*,*,#8419,.T.);
#11603=ORIENTED_EDGE('',*,*,#8420,.T.);
#11604=ORIENTED_EDGE('',*,*,#8421,.T.);
#11605=ORIENTED_EDGE('',*,*,#8422,.T.);
#11606=ORIENTED_EDGE('',*,*,#8423,.T.);
#11607=ORIENTED_EDGE('',*,*,#8424,.T.);
#11608=ORIENTED_EDGE('',*,*,#8425,.T.);
#11609=ORIENTED_EDGE('',*,*,#8426,.T.);
#11610=ORIENTED_EDGE('',*,*,#8427,.T.);
#11611=ORIENTED_EDGE('',*,*,#8428,.T.);
#11612=ORIENTED_EDGE('',*,*,#8429,.T.);
#11613=ORIENTED_EDGE('',*,*,#8430,.T.);
#11614=ORIENTED_EDGE('',*,*,#8431,.T.);
#11615=ORIENTED_EDGE('',*,*,#8432,.T.);
#11616=ORIENTED_EDGE('',*,*,#8433,.T.);
#11617=ORIENTED_EDGE('',*,*,#8434,.T.);
#11618=ORIENTED_EDGE('',*,*,#8435,.T.);
#11619=ORIENTED_EDGE('',*,*,#8436,.T.);
#11620=ORIENTED_EDGE('',*,*,#8437,.T.);
#11621=ORIENTED_EDGE('',*,*,#8438,.T.);
#11622=ORIENTED_EDGE('',*,*,#8439,.T.);
#11623=ORIENTED_EDGE('',*,*,#8440,.T.);
#11624=ORIENTED_EDGE('',*,*,#8441,.T.);
#11625=ORIENTED_EDGE('',*,*,#8442,.T.);
#11626=ORIENTED_EDGE('',*,*,#8443,.T.);
#11627=ORIENTED_EDGE('',*,*,#8444,.T.);
#11628=ORIENTED_EDGE('',*,*,#8445,.T.);
#11629=ORIENTED_EDGE('',*,*,#8446,.T.);
#11630=ORIENTED_EDGE('',*,*,#8447,.T.);
#11631=ORIENTED_EDGE('',*,*,#8448,.T.);
#11632=ORIENTED_EDGE('',*,*,#8449,.T.);
#11633=ORIENTED_EDGE('',*,*,#8450,.T.);
#11634=ORIENTED_EDGE('',*,*,#8451,.T.);
#11635=ORIENTED_EDGE('',*,*,#8452,.T.);
#11636=ORIENTED_EDGE('',*,*,#8453,.T.);
#11637=ORIENTED_EDGE('',*,*,#8454,.T.);
#11638=ORIENTED_EDGE('',*,*,#8455,.T.);
#11639=ORIENTED_EDGE('',*,*,#8456,.T.);
#11640=ORIENTED_EDGE('',*,*,#8457,.T.);
#11641=ORIENTED_EDGE('',*,*,#8458,.T.);
#11642=ORIENTED_EDGE('',*,*,#8459,.T.);
#11643=ORIENTED_EDGE('',*,*,#8460,.T.);
#11644=ORIENTED_EDGE('',*,*,#8461,.T.);
#11645=ORIENTED_EDGE('',*,*,#8462,.T.);
#11646=ORIENTED_EDGE('',*,*,#8463,.T.);
#11647=ORIENTED_EDGE('',*,*,#8464,.T.);
#11648=ORIENTED_EDGE('',*,*,#8465,.T.);
#11649=ORIENTED_EDGE('',*,*,#8466,.T.);
#11650=ORIENTED_EDGE('',*,*,#8467,.T.);
#11651=ORIENTED_EDGE('',*,*,#8468,.T.);
#11652=ORIENTED_EDGE('',*,*,#8469,.T.);
#11653=ORIENTED_EDGE('',*,*,#8470,.T.);
#11654=ORIENTED_EDGE('',*,*,#8471,.T.);
#11655=ORIENTED_EDGE('',*,*,#8472,.T.);
#11656=ORIENTED_EDGE('',*,*,#8473,.T.);
#11657=ORIENTED_EDGE('',*,*,#8474,.T.);
#11658=ORIENTED_EDGE('',*,*,#8475,.T.);
#11659=ORIENTED_EDGE('',*,*,#8476,.T.);
#11660=ORIENTED_EDGE('',*,*,#8477,.T.);
#11661=ORIENTED_EDGE('',*,*,#8478,.T.);
#11662=ORIENTED_EDGE('',*,*,#8479,.T.);
#11663=ORIENTED_EDGE('',*,*,#8480,.T.);
#11664=ORIENTED_EDGE('',*,*,#8481,.T.);
#11665=ORIENTED_EDGE('',*,*,#8482,.T.);
#11666=ORIENTED_EDGE('',*,*,#8483,.T.);
#11667=ORIENTED_EDGE('',*,*,#8484,.T.);
#11668=ORIENTED_EDGE('',*,*,#8485,.T.);
#11669=ORIENTED_EDGE('',*,*,#8486,.T.);
#11670=ORIENTED_EDGE('',*,*,#8487,.T.);
#11671=ORIENTED_EDGE('',*,*,#8488,.T.);
#11672=ORIENTED_EDGE('',*,*,#8489,.T.);
#11673=ORIENTED_EDGE('',*,*,#8490,.T.);
#11674=ORIENTED_EDGE('',*,*,#8491,.T.);
#11675=ORIENTED_EDGE('',*,*,#8492,.T.);
#11676=ORIENTED_EDGE('',*,*,#8493,.T.);
#11677=ORIENTED_EDGE('',*,*,#8494,.T.);
#11678=ORIENTED_EDGE('',*,*,#8495,.T.);
#11679=ORIENTED_EDGE('',*,*,#8496,.T.);
#11680=ORIENTED_EDGE('',*,*,#8497,.T.);
#11681=ORIENTED_EDGE('',*,*,#8498,.T.);
#11682=ORIENTED_EDGE('',*,*,#8499,.T.);
#11683=ORIENTED_EDGE('',*,*,#8500,.T.);
#11684=ORIENTED_EDGE('',*,*,#8501,.T.);
#11685=ORIENTED_EDGE('',*,*,#8502,.T.);
#11686=ORIENTED_EDGE('',*,*,#8503,.T.);
#11687=ORIENTED_EDGE('',*,*,#8504,.T.);
#11688=ORIENTED_EDGE('',*,*,#8505,.T.);
#11689=ORIENTED_EDGE('',*,*,#8506,.T.);
#11690=ORIENTED_EDGE('',*,*,#8507,.T.);
#11691=ORIENTED_EDGE('',*,*,#8508,.T.);
#11692=ORIENTED_EDGE('',*,*,#8509,.T.);
#11693=ORIENTED_EDGE('',*,*,#8510,.T.);
#11694=ORIENTED_EDGE('',*,*,#8511,.T.);
#11695=ORIENTED_EDGE('',*,*,#8512,.T.);
#11696=ORIENTED_EDGE('',*,*,#8513,.T.);
#11697=ORIENTED_EDGE('',*,*,#8514,.T.);
#11698=ORIENTED_EDGE('',*,*,#8515,.T.);
#11699=ORIENTED_EDGE('',*,*,#8516,.T.);
#11700=ORIENTED_EDGE('',*,*,#8517,.T.);
#11701=ORIENTED_EDGE('',*,*,#8518,.T.);
#11702=ORIENTED_EDGE('',*,*,#8519,.T.);
#11703=ORIENTED_EDGE('',*,*,#8520,.T.);
#11704=ORIENTED_EDGE('',*,*,#8521,.T.);
#11705=ORIENTED_EDGE('',*,*,#8522,.T.);
#11706=ORIENTED_EDGE('',*,*,#8523,.T.);
#11707=ORIENTED_EDGE('',*,*,#8356,.T.);
#11708=ORIENTED_EDGE('',*,*,#8360,.T.);
#11709=ORIENTED_EDGE('',*,*,#8363,.T.);
#11710=ORIENTED_EDGE('',*,*,#8524,.T.);
#11711=ORIENTED_EDGE('',*,*,#8357,.T.);
#11712=ORIENTED_EDGE('',*,*,#8524,.F.);
#11713=ORIENTED_EDGE('',*,*,#8362,.T.);
#11714=ORIENTED_EDGE('',*,*,#8525,.F.);
#11715=ORIENTED_EDGE('',*,*,#8526,.F.);
#11716=ORIENTED_EDGE('',*,*,#8527,.T.);
#11717=ORIENTED_EDGE('',*,*,#8528,.F.);
#11718=ORIENTED_EDGE('',*,*,#8527,.F.);
#11719=ORIENTED_EDGE('',*,*,#8526,.T.);
#11720=ORIENTED_EDGE('',*,*,#8354,.T.);
#11721=ORIENTED_EDGE('',*,*,#8525,.T.);
#11722=ORIENTED_EDGE('',*,*,#8361,.T.);
#11723=ORIENTED_EDGE('',*,*,#8358,.T.);
#11724=ORIENTED_EDGE('',*,*,#8529,.F.);
#11725=ORIENTED_EDGE('',*,*,#8530,.F.);
#11726=ORIENTED_EDGE('',*,*,#8531,.F.);
#11727=ORIENTED_EDGE('',*,*,#8521,.F.);
#11728=ORIENTED_EDGE('',*,*,#8532,.F.);
#11729=ORIENTED_EDGE('',*,*,#8523,.F.);
#11730=ORIENTED_EDGE('',*,*,#8533,.T.);
#11731=ORIENTED_EDGE('',*,*,#8534,.F.);
#11732=ORIENTED_EDGE('',*,*,#8531,.T.);
#11733=ORIENTED_EDGE('',*,*,#8535,.F.);
#11734=ORIENTED_EDGE('',*,*,#8533,.F.);
#11735=ORIENTED_EDGE('',*,*,#8522,.F.);
#11736=ORIENTED_EDGE('',*,*,#8532,.T.);
#11737=ORIENTED_EDGE('',*,*,#8536,.F.);
#11738=ORIENTED_EDGE('',*,*,#8537,.T.);
#11739=ORIENTED_EDGE('',*,*,#8364,.F.);
#11740=ORIENTED_EDGE('',*,*,#8537,.F.);
#11741=ORIENTED_EDGE('',*,*,#8538,.F.);
#11742=ORIENTED_EDGE('',*,*,#8539,.F.);
#11743=ORIENTED_EDGE('',*,*,#8365,.F.);
#11744=ORIENTED_EDGE('',*,*,#8540,.F.);
#11745=ORIENTED_EDGE('',*,*,#8367,.F.);
#11746=ORIENTED_EDGE('',*,*,#8541,.T.);
#11747=ORIENTED_EDGE('',*,*,#8542,.F.);
#11748=ORIENTED_EDGE('',*,*,#8539,.T.);
#11749=ORIENTED_EDGE('',*,*,#8543,.F.);
#11750=ORIENTED_EDGE('',*,*,#8541,.F.);
#11751=ORIENTED_EDGE('',*,*,#8366,.F.);
#11752=ORIENTED_EDGE('',*,*,#8540,.T.);
#11753=ORIENTED_EDGE('',*,*,#8544,.F.);
#11754=ORIENTED_EDGE('',*,*,#8545,.T.);
#11755=ORIENTED_EDGE('',*,*,#8368,.F.);
#11756=ORIENTED_EDGE('',*,*,#8545,.F.);
#11757=ORIENTED_EDGE('',*,*,#8546,.F.);
#11758=ORIENTED_EDGE('',*,*,#8547,.F.);
#11759=ORIENTED_EDGE('',*,*,#8369,.F.);
#11760=ORIENTED_EDGE('',*,*,#8548,.F.);
#11761=ORIENTED_EDGE('',*,*,#8371,.F.);
#11762=ORIENTED_EDGE('',*,*,#8549,.T.);
#11763=ORIENTED_EDGE('',*,*,#8550,.F.);
#11764=ORIENTED_EDGE('',*,*,#8547,.T.);
#11765=ORIENTED_EDGE('',*,*,#8551,.F.);
#11766=ORIENTED_EDGE('',*,*,#8549,.F.);
#11767=ORIENTED_EDGE('',*,*,#8370,.F.);
#11768=ORIENTED_EDGE('',*,*,#8548,.T.);
#11769=ORIENTED_EDGE('',*,*,#8552,.F.);
#11770=ORIENTED_EDGE('',*,*,#8553,.T.);
#11771=ORIENTED_EDGE('',*,*,#8372,.F.);
#11772=ORIENTED_EDGE('',*,*,#8553,.F.);
#11773=ORIENTED_EDGE('',*,*,#8554,.F.);
#11774=ORIENTED_EDGE('',*,*,#8555,.F.);
#11775=ORIENTED_EDGE('',*,*,#8373,.F.);
#11776=ORIENTED_EDGE('',*,*,#8556,.F.);
#11777=ORIENTED_EDGE('',*,*,#8375,.F.);
#11778=ORIENTED_EDGE('',*,*,#8557,.T.);
#11779=ORIENTED_EDGE('',*,*,#8558,.F.);
#11780=ORIENTED_EDGE('',*,*,#8555,.T.);
#11781=ORIENTED_EDGE('',*,*,#8559,.F.);
#11782=ORIENTED_EDGE('',*,*,#8557,.F.);
#11783=ORIENTED_EDGE('',*,*,#8374,.F.);
#11784=ORIENTED_EDGE('',*,*,#8556,.T.);
#11785=ORIENTED_EDGE('',*,*,#8560,.F.);
#11786=ORIENTED_EDGE('',*,*,#8561,.T.);
#11787=ORIENTED_EDGE('',*,*,#8376,.F.);
#11788=ORIENTED_EDGE('',*,*,#8561,.F.);
#11789=ORIENTED_EDGE('',*,*,#8562,.F.);
#11790=ORIENTED_EDGE('',*,*,#8563,.F.);
#11791=ORIENTED_EDGE('',*,*,#8377,.F.);
#11792=ORIENTED_EDGE('',*,*,#8564,.F.);
#11793=ORIENTED_EDGE('',*,*,#8379,.F.);
#11794=ORIENTED_EDGE('',*,*,#8565,.T.);
#11795=ORIENTED_EDGE('',*,*,#8566,.F.);
#11796=ORIENTED_EDGE('',*,*,#8563,.T.);
#11797=ORIENTED_EDGE('',*,*,#8567,.F.);
#11798=ORIENTED_EDGE('',*,*,#8565,.F.);
#11799=ORIENTED_EDGE('',*,*,#8378,.F.);
#11800=ORIENTED_EDGE('',*,*,#8564,.T.);
#11801=ORIENTED_EDGE('',*,*,#8568,.F.);
#11802=ORIENTED_EDGE('',*,*,#8569,.T.);
#11803=ORIENTED_EDGE('',*,*,#8380,.F.);
#11804=ORIENTED_EDGE('',*,*,#8569,.F.);
#11805=ORIENTED_EDGE('',*,*,#8570,.F.);
#11806=ORIENTED_EDGE('',*,*,#8571,.F.);
#11807=ORIENTED_EDGE('',*,*,#8381,.F.);
#11808=ORIENTED_EDGE('',*,*,#8572,.F.);
#11809=ORIENTED_EDGE('',*,*,#8383,.F.);
#11810=ORIENTED_EDGE('',*,*,#8573,.T.);
#11811=ORIENTED_EDGE('',*,*,#8574,.F.);
#11812=ORIENTED_EDGE('',*,*,#8571,.T.);
#11813=ORIENTED_EDGE('',*,*,#8575,.F.);
#11814=ORIENTED_EDGE('',*,*,#8573,.F.);
#11815=ORIENTED_EDGE('',*,*,#8382,.F.);
#11816=ORIENTED_EDGE('',*,*,#8572,.T.);
#11817=ORIENTED_EDGE('',*,*,#8576,.F.);
#11818=ORIENTED_EDGE('',*,*,#8577,.T.);
#11819=ORIENTED_EDGE('',*,*,#8384,.F.);
#11820=ORIENTED_EDGE('',*,*,#8577,.F.);
#11821=ORIENTED_EDGE('',*,*,#8578,.F.);
#11822=ORIENTED_EDGE('',*,*,#8579,.F.);
#11823=ORIENTED_EDGE('',*,*,#8385,.F.);
#11824=ORIENTED_EDGE('',*,*,#8580,.F.);
#11825=ORIENTED_EDGE('',*,*,#8387,.F.);
#11826=ORIENTED_EDGE('',*,*,#8581,.T.);
#11827=ORIENTED_EDGE('',*,*,#8582,.F.);
#11828=ORIENTED_EDGE('',*,*,#8579,.T.);
#11829=ORIENTED_EDGE('',*,*,#8583,.F.);
#11830=ORIENTED_EDGE('',*,*,#8581,.F.);
#11831=ORIENTED_EDGE('',*,*,#8386,.F.);
#11832=ORIENTED_EDGE('',*,*,#8580,.T.);
#11833=ORIENTED_EDGE('',*,*,#8584,.F.);
#11834=ORIENTED_EDGE('',*,*,#8585,.T.);
#11835=ORIENTED_EDGE('',*,*,#8388,.F.);
#11836=ORIENTED_EDGE('',*,*,#8585,.F.);
#11837=ORIENTED_EDGE('',*,*,#8586,.F.);
#11838=ORIENTED_EDGE('',*,*,#8587,.F.);
#11839=ORIENTED_EDGE('',*,*,#8389,.F.);
#11840=ORIENTED_EDGE('',*,*,#8588,.F.);
#11841=ORIENTED_EDGE('',*,*,#8391,.F.);
#11842=ORIENTED_EDGE('',*,*,#8589,.T.);
#11843=ORIENTED_EDGE('',*,*,#8590,.F.);
#11844=ORIENTED_EDGE('',*,*,#8587,.T.);
#11845=ORIENTED_EDGE('',*,*,#8591,.F.);
#11846=ORIENTED_EDGE('',*,*,#8589,.F.);
#11847=ORIENTED_EDGE('',*,*,#8390,.F.);
#11848=ORIENTED_EDGE('',*,*,#8588,.T.);
#11849=ORIENTED_EDGE('',*,*,#8592,.F.);
#11850=ORIENTED_EDGE('',*,*,#8593,.T.);
#11851=ORIENTED_EDGE('',*,*,#8392,.F.);
#11852=ORIENTED_EDGE('',*,*,#8593,.F.);
#11853=ORIENTED_EDGE('',*,*,#8594,.F.);
#11854=ORIENTED_EDGE('',*,*,#8595,.F.);
#11855=ORIENTED_EDGE('',*,*,#8393,.F.);
#11856=ORIENTED_EDGE('',*,*,#8596,.F.);
#11857=ORIENTED_EDGE('',*,*,#8395,.F.);
#11858=ORIENTED_EDGE('',*,*,#8597,.T.);
#11859=ORIENTED_EDGE('',*,*,#8598,.F.);
#11860=ORIENTED_EDGE('',*,*,#8595,.T.);
#11861=ORIENTED_EDGE('',*,*,#8599,.F.);
#11862=ORIENTED_EDGE('',*,*,#8597,.F.);
#11863=ORIENTED_EDGE('',*,*,#8394,.F.);
#11864=ORIENTED_EDGE('',*,*,#8596,.T.);
#11865=ORIENTED_EDGE('',*,*,#8600,.F.);
#11866=ORIENTED_EDGE('',*,*,#8601,.T.);
#11867=ORIENTED_EDGE('',*,*,#8396,.F.);
#11868=ORIENTED_EDGE('',*,*,#8601,.F.);
#11869=ORIENTED_EDGE('',*,*,#8602,.F.);
#11870=ORIENTED_EDGE('',*,*,#8603,.F.);
#11871=ORIENTED_EDGE('',*,*,#8397,.F.);
#11872=ORIENTED_EDGE('',*,*,#8604,.F.);
#11873=ORIENTED_EDGE('',*,*,#8399,.F.);
#11874=ORIENTED_EDGE('',*,*,#8605,.T.);
#11875=ORIENTED_EDGE('',*,*,#8606,.F.);
#11876=ORIENTED_EDGE('',*,*,#8603,.T.);
#11877=ORIENTED_EDGE('',*,*,#8607,.F.);
#11878=ORIENTED_EDGE('',*,*,#8605,.F.);
#11879=ORIENTED_EDGE('',*,*,#8398,.F.);
#11880=ORIENTED_EDGE('',*,*,#8604,.T.);
#11881=ORIENTED_EDGE('',*,*,#8608,.F.);
#11882=ORIENTED_EDGE('',*,*,#8609,.T.);
#11883=ORIENTED_EDGE('',*,*,#8400,.F.);
#11884=ORIENTED_EDGE('',*,*,#8609,.F.);
#11885=ORIENTED_EDGE('',*,*,#8610,.F.);
#11886=ORIENTED_EDGE('',*,*,#8611,.F.);
#11887=ORIENTED_EDGE('',*,*,#8401,.F.);
#11888=ORIENTED_EDGE('',*,*,#8612,.F.);
#11889=ORIENTED_EDGE('',*,*,#8403,.F.);
#11890=ORIENTED_EDGE('',*,*,#8613,.T.);
#11891=ORIENTED_EDGE('',*,*,#8614,.F.);
#11892=ORIENTED_EDGE('',*,*,#8611,.T.);
#11893=ORIENTED_EDGE('',*,*,#8615,.F.);
#11894=ORIENTED_EDGE('',*,*,#8613,.F.);
#11895=ORIENTED_EDGE('',*,*,#8402,.F.);
#11896=ORIENTED_EDGE('',*,*,#8612,.T.);
#11897=ORIENTED_EDGE('',*,*,#8616,.F.);
#11898=ORIENTED_EDGE('',*,*,#8617,.T.);
#11899=ORIENTED_EDGE('',*,*,#8404,.F.);
#11900=ORIENTED_EDGE('',*,*,#8617,.F.);
#11901=ORIENTED_EDGE('',*,*,#8618,.F.);
#11902=ORIENTED_EDGE('',*,*,#8619,.F.);
#11903=ORIENTED_EDGE('',*,*,#8405,.F.);
#11904=ORIENTED_EDGE('',*,*,#8620,.F.);
#11905=ORIENTED_EDGE('',*,*,#8407,.F.);
#11906=ORIENTED_EDGE('',*,*,#8621,.T.);
#11907=ORIENTED_EDGE('',*,*,#8622,.F.);
#11908=ORIENTED_EDGE('',*,*,#8619,.T.);
#11909=ORIENTED_EDGE('',*,*,#8623,.F.);
#11910=ORIENTED_EDGE('',*,*,#8621,.F.);
#11911=ORIENTED_EDGE('',*,*,#8406,.F.);
#11912=ORIENTED_EDGE('',*,*,#8620,.T.);
#11913=ORIENTED_EDGE('',*,*,#8624,.F.);
#11914=ORIENTED_EDGE('',*,*,#8625,.T.);
#11915=ORIENTED_EDGE('',*,*,#8408,.F.);
#11916=ORIENTED_EDGE('',*,*,#8625,.F.);
#11917=ORIENTED_EDGE('',*,*,#8626,.F.);
#11918=ORIENTED_EDGE('',*,*,#8627,.F.);
#11919=ORIENTED_EDGE('',*,*,#8409,.F.);
#11920=ORIENTED_EDGE('',*,*,#8628,.F.);
#11921=ORIENTED_EDGE('',*,*,#8411,.F.);
#11922=ORIENTED_EDGE('',*,*,#8629,.T.);
#11923=ORIENTED_EDGE('',*,*,#8630,.F.);
#11924=ORIENTED_EDGE('',*,*,#8627,.T.);
#11925=ORIENTED_EDGE('',*,*,#8631,.F.);
#11926=ORIENTED_EDGE('',*,*,#8629,.F.);
#11927=ORIENTED_EDGE('',*,*,#8410,.F.);
#11928=ORIENTED_EDGE('',*,*,#8628,.T.);
#11929=ORIENTED_EDGE('',*,*,#8632,.F.);
#11930=ORIENTED_EDGE('',*,*,#8633,.T.);
#11931=ORIENTED_EDGE('',*,*,#8412,.F.);
#11932=ORIENTED_EDGE('',*,*,#8633,.F.);
#11933=ORIENTED_EDGE('',*,*,#8634,.F.);
#11934=ORIENTED_EDGE('',*,*,#8635,.F.);
#11935=ORIENTED_EDGE('',*,*,#8413,.F.);
#11936=ORIENTED_EDGE('',*,*,#8636,.F.);
#11937=ORIENTED_EDGE('',*,*,#8415,.F.);
#11938=ORIENTED_EDGE('',*,*,#8637,.T.);
#11939=ORIENTED_EDGE('',*,*,#8638,.F.);
#11940=ORIENTED_EDGE('',*,*,#8635,.T.);
#11941=ORIENTED_EDGE('',*,*,#8639,.F.);
#11942=ORIENTED_EDGE('',*,*,#8637,.F.);
#11943=ORIENTED_EDGE('',*,*,#8414,.F.);
#11944=ORIENTED_EDGE('',*,*,#8636,.T.);
#11945=ORIENTED_EDGE('',*,*,#8640,.F.);
#11946=ORIENTED_EDGE('',*,*,#8641,.T.);
#11947=ORIENTED_EDGE('',*,*,#8416,.F.);
#11948=ORIENTED_EDGE('',*,*,#8641,.F.);
#11949=ORIENTED_EDGE('',*,*,#8642,.F.);
#11950=ORIENTED_EDGE('',*,*,#8643,.F.);
#11951=ORIENTED_EDGE('',*,*,#8417,.F.);
#11952=ORIENTED_EDGE('',*,*,#8644,.F.);
#11953=ORIENTED_EDGE('',*,*,#8419,.F.);
#11954=ORIENTED_EDGE('',*,*,#8645,.T.);
#11955=ORIENTED_EDGE('',*,*,#8646,.F.);
#11956=ORIENTED_EDGE('',*,*,#8643,.T.);
#11957=ORIENTED_EDGE('',*,*,#8647,.F.);
#11958=ORIENTED_EDGE('',*,*,#8645,.F.);
#11959=ORIENTED_EDGE('',*,*,#8418,.F.);
#11960=ORIENTED_EDGE('',*,*,#8644,.T.);
#11961=ORIENTED_EDGE('',*,*,#8648,.F.);
#11962=ORIENTED_EDGE('',*,*,#8649,.T.);
#11963=ORIENTED_EDGE('',*,*,#8420,.F.);
#11964=ORIENTED_EDGE('',*,*,#8649,.F.);
#11965=ORIENTED_EDGE('',*,*,#8650,.F.);
#11966=ORIENTED_EDGE('',*,*,#8651,.F.);
#11967=ORIENTED_EDGE('',*,*,#8421,.F.);
#11968=ORIENTED_EDGE('',*,*,#8652,.F.);
#11969=ORIENTED_EDGE('',*,*,#8423,.F.);
#11970=ORIENTED_EDGE('',*,*,#8653,.T.);
#11971=ORIENTED_EDGE('',*,*,#8654,.F.);
#11972=ORIENTED_EDGE('',*,*,#8651,.T.);
#11973=ORIENTED_EDGE('',*,*,#8655,.F.);
#11974=ORIENTED_EDGE('',*,*,#8653,.F.);
#11975=ORIENTED_EDGE('',*,*,#8422,.F.);
#11976=ORIENTED_EDGE('',*,*,#8652,.T.);
#11977=ORIENTED_EDGE('',*,*,#8656,.F.);
#11978=ORIENTED_EDGE('',*,*,#8657,.T.);
#11979=ORIENTED_EDGE('',*,*,#8424,.F.);
#11980=ORIENTED_EDGE('',*,*,#8657,.F.);
#11981=ORIENTED_EDGE('',*,*,#8658,.F.);
#11982=ORIENTED_EDGE('',*,*,#8659,.F.);
#11983=ORIENTED_EDGE('',*,*,#8425,.F.);
#11984=ORIENTED_EDGE('',*,*,#8660,.F.);
#11985=ORIENTED_EDGE('',*,*,#8427,.F.);
#11986=ORIENTED_EDGE('',*,*,#8661,.T.);
#11987=ORIENTED_EDGE('',*,*,#8662,.F.);
#11988=ORIENTED_EDGE('',*,*,#8659,.T.);
#11989=ORIENTED_EDGE('',*,*,#8663,.F.);
#11990=ORIENTED_EDGE('',*,*,#8661,.F.);
#11991=ORIENTED_EDGE('',*,*,#8426,.F.);
#11992=ORIENTED_EDGE('',*,*,#8660,.T.);
#11993=ORIENTED_EDGE('',*,*,#8664,.F.);
#11994=ORIENTED_EDGE('',*,*,#8665,.T.);
#11995=ORIENTED_EDGE('',*,*,#8428,.F.);
#11996=ORIENTED_EDGE('',*,*,#8665,.F.);
#11997=ORIENTED_EDGE('',*,*,#8666,.F.);
#11998=ORIENTED_EDGE('',*,*,#8667,.F.);
#11999=ORIENTED_EDGE('',*,*,#8429,.F.);
#12000=ORIENTED_EDGE('',*,*,#8668,.F.);
#12001=ORIENTED_EDGE('',*,*,#8431,.F.);
#12002=ORIENTED_EDGE('',*,*,#8669,.T.);
#12003=ORIENTED_EDGE('',*,*,#8670,.F.);
#12004=ORIENTED_EDGE('',*,*,#8667,.T.);
#12005=ORIENTED_EDGE('',*,*,#8671,.F.);
#12006=ORIENTED_EDGE('',*,*,#8669,.F.);
#12007=ORIENTED_EDGE('',*,*,#8430,.F.);
#12008=ORIENTED_EDGE('',*,*,#8668,.T.);
#12009=ORIENTED_EDGE('',*,*,#8672,.F.);
#12010=ORIENTED_EDGE('',*,*,#8673,.T.);
#12011=ORIENTED_EDGE('',*,*,#8432,.F.);
#12012=ORIENTED_EDGE('',*,*,#8673,.F.);
#12013=ORIENTED_EDGE('',*,*,#8674,.F.);
#12014=ORIENTED_EDGE('',*,*,#8675,.F.);
#12015=ORIENTED_EDGE('',*,*,#8433,.F.);
#12016=ORIENTED_EDGE('',*,*,#8676,.F.);
#12017=ORIENTED_EDGE('',*,*,#8435,.F.);
#12018=ORIENTED_EDGE('',*,*,#8677,.T.);
#12019=ORIENTED_EDGE('',*,*,#8678,.F.);
#12020=ORIENTED_EDGE('',*,*,#8675,.T.);
#12021=ORIENTED_EDGE('',*,*,#8679,.F.);
#12022=ORIENTED_EDGE('',*,*,#8677,.F.);
#12023=ORIENTED_EDGE('',*,*,#8434,.F.);
#12024=ORIENTED_EDGE('',*,*,#8676,.T.);
#12025=ORIENTED_EDGE('',*,*,#8680,.F.);
#12026=ORIENTED_EDGE('',*,*,#8681,.T.);
#12027=ORIENTED_EDGE('',*,*,#8436,.F.);
#12028=ORIENTED_EDGE('',*,*,#8681,.F.);
#12029=ORIENTED_EDGE('',*,*,#8682,.F.);
#12030=ORIENTED_EDGE('',*,*,#8683,.F.);
#12031=ORIENTED_EDGE('',*,*,#8437,.F.);
#12032=ORIENTED_EDGE('',*,*,#8684,.F.);
#12033=ORIENTED_EDGE('',*,*,#8439,.F.);
#12034=ORIENTED_EDGE('',*,*,#8685,.T.);
#12035=ORIENTED_EDGE('',*,*,#8686,.F.);
#12036=ORIENTED_EDGE('',*,*,#8683,.T.);
#12037=ORIENTED_EDGE('',*,*,#8687,.F.);
#12038=ORIENTED_EDGE('',*,*,#8685,.F.);
#12039=ORIENTED_EDGE('',*,*,#8438,.F.);
#12040=ORIENTED_EDGE('',*,*,#8684,.T.);
#12041=ORIENTED_EDGE('',*,*,#8688,.F.);
#12042=ORIENTED_EDGE('',*,*,#8689,.T.);
#12043=ORIENTED_EDGE('',*,*,#8440,.F.);
#12044=ORIENTED_EDGE('',*,*,#8689,.F.);
#12045=ORIENTED_EDGE('',*,*,#8690,.F.);
#12046=ORIENTED_EDGE('',*,*,#8691,.F.);
#12047=ORIENTED_EDGE('',*,*,#8441,.F.);
#12048=ORIENTED_EDGE('',*,*,#8692,.F.);
#12049=ORIENTED_EDGE('',*,*,#8443,.F.);
#12050=ORIENTED_EDGE('',*,*,#8693,.T.);
#12051=ORIENTED_EDGE('',*,*,#8694,.F.);
#12052=ORIENTED_EDGE('',*,*,#8691,.T.);
#12053=ORIENTED_EDGE('',*,*,#8695,.F.);
#12054=ORIENTED_EDGE('',*,*,#8693,.F.);
#12055=ORIENTED_EDGE('',*,*,#8442,.F.);
#12056=ORIENTED_EDGE('',*,*,#8692,.T.);
#12057=ORIENTED_EDGE('',*,*,#8696,.F.);
#12058=ORIENTED_EDGE('',*,*,#8697,.T.);
#12059=ORIENTED_EDGE('',*,*,#8444,.F.);
#12060=ORIENTED_EDGE('',*,*,#8697,.F.);
#12061=ORIENTED_EDGE('',*,*,#8698,.F.);
#12062=ORIENTED_EDGE('',*,*,#8699,.F.);
#12063=ORIENTED_EDGE('',*,*,#8445,.F.);
#12064=ORIENTED_EDGE('',*,*,#8700,.F.);
#12065=ORIENTED_EDGE('',*,*,#8447,.F.);
#12066=ORIENTED_EDGE('',*,*,#8701,.T.);
#12067=ORIENTED_EDGE('',*,*,#8702,.F.);
#12068=ORIENTED_EDGE('',*,*,#8699,.T.);
#12069=ORIENTED_EDGE('',*,*,#8703,.F.);
#12070=ORIENTED_EDGE('',*,*,#8701,.F.);
#12071=ORIENTED_EDGE('',*,*,#8446,.F.);
#12072=ORIENTED_EDGE('',*,*,#8700,.T.);
#12073=ORIENTED_EDGE('',*,*,#8704,.F.);
#12074=ORIENTED_EDGE('',*,*,#8705,.T.);
#12075=ORIENTED_EDGE('',*,*,#8448,.F.);
#12076=ORIENTED_EDGE('',*,*,#8705,.F.);
#12077=ORIENTED_EDGE('',*,*,#8706,.F.);
#12078=ORIENTED_EDGE('',*,*,#8707,.F.);
#12079=ORIENTED_EDGE('',*,*,#8449,.F.);
#12080=ORIENTED_EDGE('',*,*,#8708,.F.);
#12081=ORIENTED_EDGE('',*,*,#8451,.F.);
#12082=ORIENTED_EDGE('',*,*,#8709,.T.);
#12083=ORIENTED_EDGE('',*,*,#8710,.F.);
#12084=ORIENTED_EDGE('',*,*,#8707,.T.);
#12085=ORIENTED_EDGE('',*,*,#8711,.F.);
#12086=ORIENTED_EDGE('',*,*,#8709,.F.);
#12087=ORIENTED_EDGE('',*,*,#8450,.F.);
#12088=ORIENTED_EDGE('',*,*,#8708,.T.);
#12089=ORIENTED_EDGE('',*,*,#8712,.F.);
#12090=ORIENTED_EDGE('',*,*,#8713,.T.);
#12091=ORIENTED_EDGE('',*,*,#8452,.F.);
#12092=ORIENTED_EDGE('',*,*,#8713,.F.);
#12093=ORIENTED_EDGE('',*,*,#8714,.F.);
#12094=ORIENTED_EDGE('',*,*,#8715,.F.);
#12095=ORIENTED_EDGE('',*,*,#8453,.F.);
#12096=ORIENTED_EDGE('',*,*,#8716,.F.);
#12097=ORIENTED_EDGE('',*,*,#8455,.F.);
#12098=ORIENTED_EDGE('',*,*,#8717,.T.);
#12099=ORIENTED_EDGE('',*,*,#8718,.F.);
#12100=ORIENTED_EDGE('',*,*,#8715,.T.);
#12101=ORIENTED_EDGE('',*,*,#8719,.F.);
#12102=ORIENTED_EDGE('',*,*,#8717,.F.);
#12103=ORIENTED_EDGE('',*,*,#8454,.F.);
#12104=ORIENTED_EDGE('',*,*,#8716,.T.);
#12105=ORIENTED_EDGE('',*,*,#8720,.F.);
#12106=ORIENTED_EDGE('',*,*,#8721,.T.);
#12107=ORIENTED_EDGE('',*,*,#8456,.F.);
#12108=ORIENTED_EDGE('',*,*,#8721,.F.);
#12109=ORIENTED_EDGE('',*,*,#8722,.F.);
#12110=ORIENTED_EDGE('',*,*,#8723,.F.);
#12111=ORIENTED_EDGE('',*,*,#8457,.F.);
#12112=ORIENTED_EDGE('',*,*,#8724,.F.);
#12113=ORIENTED_EDGE('',*,*,#8459,.F.);
#12114=ORIENTED_EDGE('',*,*,#8725,.T.);
#12115=ORIENTED_EDGE('',*,*,#8726,.F.);
#12116=ORIENTED_EDGE('',*,*,#8723,.T.);
#12117=ORIENTED_EDGE('',*,*,#8727,.F.);
#12118=ORIENTED_EDGE('',*,*,#8725,.F.);
#12119=ORIENTED_EDGE('',*,*,#8458,.F.);
#12120=ORIENTED_EDGE('',*,*,#8724,.T.);
#12121=ORIENTED_EDGE('',*,*,#8728,.F.);
#12122=ORIENTED_EDGE('',*,*,#8729,.T.);
#12123=ORIENTED_EDGE('',*,*,#8460,.F.);
#12124=ORIENTED_EDGE('',*,*,#8729,.F.);
#12125=ORIENTED_EDGE('',*,*,#8730,.F.);
#12126=ORIENTED_EDGE('',*,*,#8731,.F.);
#12127=ORIENTED_EDGE('',*,*,#8461,.F.);
#12128=ORIENTED_EDGE('',*,*,#8732,.F.);
#12129=ORIENTED_EDGE('',*,*,#8463,.F.);
#12130=ORIENTED_EDGE('',*,*,#8733,.T.);
#12131=ORIENTED_EDGE('',*,*,#8734,.F.);
#12132=ORIENTED_EDGE('',*,*,#8731,.T.);
#12133=ORIENTED_EDGE('',*,*,#8735,.F.);
#12134=ORIENTED_EDGE('',*,*,#8733,.F.);
#12135=ORIENTED_EDGE('',*,*,#8462,.F.);
#12136=ORIENTED_EDGE('',*,*,#8732,.T.);
#12137=ORIENTED_EDGE('',*,*,#8736,.F.);
#12138=ORIENTED_EDGE('',*,*,#8737,.T.);
#12139=ORIENTED_EDGE('',*,*,#8464,.F.);
#12140=ORIENTED_EDGE('',*,*,#8737,.F.);
#12141=ORIENTED_EDGE('',*,*,#8738,.F.);
#12142=ORIENTED_EDGE('',*,*,#8739,.F.);
#12143=ORIENTED_EDGE('',*,*,#8465,.F.);
#12144=ORIENTED_EDGE('',*,*,#8740,.F.);
#12145=ORIENTED_EDGE('',*,*,#8467,.F.);
#12146=ORIENTED_EDGE('',*,*,#8741,.T.);
#12147=ORIENTED_EDGE('',*,*,#8742,.F.);
#12148=ORIENTED_EDGE('',*,*,#8739,.T.);
#12149=ORIENTED_EDGE('',*,*,#8743,.F.);
#12150=ORIENTED_EDGE('',*,*,#8741,.F.);
#12151=ORIENTED_EDGE('',*,*,#8466,.F.);
#12152=ORIENTED_EDGE('',*,*,#8740,.T.);
#12153=ORIENTED_EDGE('',*,*,#8744,.F.);
#12154=ORIENTED_EDGE('',*,*,#8745,.T.);
#12155=ORIENTED_EDGE('',*,*,#8468,.F.);
#12156=ORIENTED_EDGE('',*,*,#8745,.F.);
#12157=ORIENTED_EDGE('',*,*,#8746,.F.);
#12158=ORIENTED_EDGE('',*,*,#8747,.F.);
#12159=ORIENTED_EDGE('',*,*,#8469,.F.);
#12160=ORIENTED_EDGE('',*,*,#8748,.F.);
#12161=ORIENTED_EDGE('',*,*,#8471,.F.);
#12162=ORIENTED_EDGE('',*,*,#8749,.T.);
#12163=ORIENTED_EDGE('',*,*,#8750,.F.);
#12164=ORIENTED_EDGE('',*,*,#8747,.T.);
#12165=ORIENTED_EDGE('',*,*,#8751,.F.);
#12166=ORIENTED_EDGE('',*,*,#8749,.F.);
#12167=ORIENTED_EDGE('',*,*,#8470,.F.);
#12168=ORIENTED_EDGE('',*,*,#8748,.T.);
#12169=ORIENTED_EDGE('',*,*,#8752,.F.);
#12170=ORIENTED_EDGE('',*,*,#8753,.T.);
#12171=ORIENTED_EDGE('',*,*,#8472,.F.);
#12172=ORIENTED_EDGE('',*,*,#8753,.F.);
#12173=ORIENTED_EDGE('',*,*,#8754,.F.);
#12174=ORIENTED_EDGE('',*,*,#8755,.F.);
#12175=ORIENTED_EDGE('',*,*,#8473,.F.);
#12176=ORIENTED_EDGE('',*,*,#8756,.F.);
#12177=ORIENTED_EDGE('',*,*,#8475,.F.);
#12178=ORIENTED_EDGE('',*,*,#8757,.T.);
#12179=ORIENTED_EDGE('',*,*,#8758,.F.);
#12180=ORIENTED_EDGE('',*,*,#8755,.T.);
#12181=ORIENTED_EDGE('',*,*,#8759,.F.);
#12182=ORIENTED_EDGE('',*,*,#8757,.F.);
#12183=ORIENTED_EDGE('',*,*,#8474,.F.);
#12184=ORIENTED_EDGE('',*,*,#8756,.T.);
#12185=ORIENTED_EDGE('',*,*,#8760,.F.);
#12186=ORIENTED_EDGE('',*,*,#8761,.T.);
#12187=ORIENTED_EDGE('',*,*,#8476,.F.);
#12188=ORIENTED_EDGE('',*,*,#8761,.F.);
#12189=ORIENTED_EDGE('',*,*,#8762,.F.);
#12190=ORIENTED_EDGE('',*,*,#8763,.F.);
#12191=ORIENTED_EDGE('',*,*,#8477,.F.);
#12192=ORIENTED_EDGE('',*,*,#8764,.F.);
#12193=ORIENTED_EDGE('',*,*,#8479,.F.);
#12194=ORIENTED_EDGE('',*,*,#8765,.T.);
#12195=ORIENTED_EDGE('',*,*,#8766,.F.);
#12196=ORIENTED_EDGE('',*,*,#8763,.T.);
#12197=ORIENTED_EDGE('',*,*,#8767,.F.);
#12198=ORIENTED_EDGE('',*,*,#8765,.F.);
#12199=ORIENTED_EDGE('',*,*,#8478,.F.);
#12200=ORIENTED_EDGE('',*,*,#8764,.T.);
#12201=ORIENTED_EDGE('',*,*,#8768,.F.);
#12202=ORIENTED_EDGE('',*,*,#8769,.T.);
#12203=ORIENTED_EDGE('',*,*,#8480,.F.);
#12204=ORIENTED_EDGE('',*,*,#8769,.F.);
#12205=ORIENTED_EDGE('',*,*,#8770,.F.);
#12206=ORIENTED_EDGE('',*,*,#8771,.F.);
#12207=ORIENTED_EDGE('',*,*,#8481,.F.);
#12208=ORIENTED_EDGE('',*,*,#8772,.F.);
#12209=ORIENTED_EDGE('',*,*,#8483,.F.);
#12210=ORIENTED_EDGE('',*,*,#8773,.T.);
#12211=ORIENTED_EDGE('',*,*,#8774,.F.);
#12212=ORIENTED_EDGE('',*,*,#8771,.T.);
#12213=ORIENTED_EDGE('',*,*,#8775,.F.);
#12214=ORIENTED_EDGE('',*,*,#8773,.F.);
#12215=ORIENTED_EDGE('',*,*,#8482,.F.);
#12216=ORIENTED_EDGE('',*,*,#8772,.T.);
#12217=ORIENTED_EDGE('',*,*,#8776,.F.);
#12218=ORIENTED_EDGE('',*,*,#8777,.T.);
#12219=ORIENTED_EDGE('',*,*,#8484,.F.);
#12220=ORIENTED_EDGE('',*,*,#8777,.F.);
#12221=ORIENTED_EDGE('',*,*,#8778,.F.);
#12222=ORIENTED_EDGE('',*,*,#8779,.F.);
#12223=ORIENTED_EDGE('',*,*,#8485,.F.);
#12224=ORIENTED_EDGE('',*,*,#8780,.F.);
#12225=ORIENTED_EDGE('',*,*,#8487,.F.);
#12226=ORIENTED_EDGE('',*,*,#8781,.T.);
#12227=ORIENTED_EDGE('',*,*,#8782,.F.);
#12228=ORIENTED_EDGE('',*,*,#8779,.T.);
#12229=ORIENTED_EDGE('',*,*,#8783,.F.);
#12230=ORIENTED_EDGE('',*,*,#8781,.F.);
#12231=ORIENTED_EDGE('',*,*,#8486,.F.);
#12232=ORIENTED_EDGE('',*,*,#8780,.T.);
#12233=ORIENTED_EDGE('',*,*,#8784,.F.);
#12234=ORIENTED_EDGE('',*,*,#8785,.T.);
#12235=ORIENTED_EDGE('',*,*,#8488,.F.);
#12236=ORIENTED_EDGE('',*,*,#8785,.F.);
#12237=ORIENTED_EDGE('',*,*,#8786,.F.);
#12238=ORIENTED_EDGE('',*,*,#8787,.F.);
#12239=ORIENTED_EDGE('',*,*,#8489,.F.);
#12240=ORIENTED_EDGE('',*,*,#8788,.F.);
#12241=ORIENTED_EDGE('',*,*,#8491,.F.);
#12242=ORIENTED_EDGE('',*,*,#8789,.T.);
#12243=ORIENTED_EDGE('',*,*,#8790,.F.);
#12244=ORIENTED_EDGE('',*,*,#8787,.T.);
#12245=ORIENTED_EDGE('',*,*,#8791,.F.);
#12246=ORIENTED_EDGE('',*,*,#8789,.F.);
#12247=ORIENTED_EDGE('',*,*,#8490,.F.);
#12248=ORIENTED_EDGE('',*,*,#8788,.T.);
#12249=ORIENTED_EDGE('',*,*,#8792,.F.);
#12250=ORIENTED_EDGE('',*,*,#8793,.T.);
#12251=ORIENTED_EDGE('',*,*,#8492,.F.);
#12252=ORIENTED_EDGE('',*,*,#8793,.F.);
#12253=ORIENTED_EDGE('',*,*,#8794,.F.);
#12254=ORIENTED_EDGE('',*,*,#8795,.F.);
#12255=ORIENTED_EDGE('',*,*,#8493,.F.);
#12256=ORIENTED_EDGE('',*,*,#8796,.F.);
#12257=ORIENTED_EDGE('',*,*,#8495,.F.);
#12258=ORIENTED_EDGE('',*,*,#8797,.T.);
#12259=ORIENTED_EDGE('',*,*,#8798,.F.);
#12260=ORIENTED_EDGE('',*,*,#8795,.T.);
#12261=ORIENTED_EDGE('',*,*,#8799,.F.);
#12262=ORIENTED_EDGE('',*,*,#8797,.F.);
#12263=ORIENTED_EDGE('',*,*,#8494,.F.);
#12264=ORIENTED_EDGE('',*,*,#8796,.T.);
#12265=ORIENTED_EDGE('',*,*,#8800,.F.);
#12266=ORIENTED_EDGE('',*,*,#8801,.T.);
#12267=ORIENTED_EDGE('',*,*,#8496,.F.);
#12268=ORIENTED_EDGE('',*,*,#8801,.F.);
#12269=ORIENTED_EDGE('',*,*,#8802,.F.);
#12270=ORIENTED_EDGE('',*,*,#8803,.F.);
#12271=ORIENTED_EDGE('',*,*,#8497,.F.);
#12272=ORIENTED_EDGE('',*,*,#8804,.F.);
#12273=ORIENTED_EDGE('',*,*,#8499,.F.);
#12274=ORIENTED_EDGE('',*,*,#8805,.T.);
#12275=ORIENTED_EDGE('',*,*,#8806,.F.);
#12276=ORIENTED_EDGE('',*,*,#8803,.T.);
#12277=ORIENTED_EDGE('',*,*,#8807,.F.);
#12278=ORIENTED_EDGE('',*,*,#8805,.F.);
#12279=ORIENTED_EDGE('',*,*,#8498,.F.);
#12280=ORIENTED_EDGE('',*,*,#8804,.T.);
#12281=ORIENTED_EDGE('',*,*,#8808,.F.);
#12282=ORIENTED_EDGE('',*,*,#8809,.T.);
#12283=ORIENTED_EDGE('',*,*,#8500,.F.);
#12284=ORIENTED_EDGE('',*,*,#8809,.F.);
#12285=ORIENTED_EDGE('',*,*,#8810,.F.);
#12286=ORIENTED_EDGE('',*,*,#8811,.F.);
#12287=ORIENTED_EDGE('',*,*,#8501,.F.);
#12288=ORIENTED_EDGE('',*,*,#8812,.F.);
#12289=ORIENTED_EDGE('',*,*,#8503,.F.);
#12290=ORIENTED_EDGE('',*,*,#8813,.T.);
#12291=ORIENTED_EDGE('',*,*,#8814,.F.);
#12292=ORIENTED_EDGE('',*,*,#8811,.T.);
#12293=ORIENTED_EDGE('',*,*,#8815,.F.);
#12294=ORIENTED_EDGE('',*,*,#8813,.F.);
#12295=ORIENTED_EDGE('',*,*,#8502,.F.);
#12296=ORIENTED_EDGE('',*,*,#8812,.T.);
#12297=ORIENTED_EDGE('',*,*,#8816,.F.);
#12298=ORIENTED_EDGE('',*,*,#8817,.T.);
#12299=ORIENTED_EDGE('',*,*,#8504,.F.);
#12300=ORIENTED_EDGE('',*,*,#8817,.F.);
#12301=ORIENTED_EDGE('',*,*,#8818,.F.);
#12302=ORIENTED_EDGE('',*,*,#8819,.F.);
#12303=ORIENTED_EDGE('',*,*,#8505,.F.);
#12304=ORIENTED_EDGE('',*,*,#8820,.F.);
#12305=ORIENTED_EDGE('',*,*,#8507,.F.);
#12306=ORIENTED_EDGE('',*,*,#8821,.T.);
#12307=ORIENTED_EDGE('',*,*,#8822,.F.);
#12308=ORIENTED_EDGE('',*,*,#8819,.T.);
#12309=ORIENTED_EDGE('',*,*,#8823,.F.);
#12310=ORIENTED_EDGE('',*,*,#8821,.F.);
#12311=ORIENTED_EDGE('',*,*,#8506,.F.);
#12312=ORIENTED_EDGE('',*,*,#8820,.T.);
#12313=ORIENTED_EDGE('',*,*,#8824,.F.);
#12314=ORIENTED_EDGE('',*,*,#8825,.T.);
#12315=ORIENTED_EDGE('',*,*,#8508,.F.);
#12316=ORIENTED_EDGE('',*,*,#8825,.F.);
#12317=ORIENTED_EDGE('',*,*,#8826,.F.);
#12318=ORIENTED_EDGE('',*,*,#8827,.F.);
#12319=ORIENTED_EDGE('',*,*,#8509,.F.);
#12320=ORIENTED_EDGE('',*,*,#8828,.F.);
#12321=ORIENTED_EDGE('',*,*,#8511,.F.);
#12322=ORIENTED_EDGE('',*,*,#8829,.T.);
#12323=ORIENTED_EDGE('',*,*,#8830,.F.);
#12324=ORIENTED_EDGE('',*,*,#8827,.T.);
#12325=ORIENTED_EDGE('',*,*,#8831,.F.);
#12326=ORIENTED_EDGE('',*,*,#8829,.F.);
#12327=ORIENTED_EDGE('',*,*,#8510,.F.);
#12328=ORIENTED_EDGE('',*,*,#8828,.T.);
#12329=ORIENTED_EDGE('',*,*,#8832,.F.);
#12330=ORIENTED_EDGE('',*,*,#8833,.T.);
#12331=ORIENTED_EDGE('',*,*,#8512,.F.);
#12332=ORIENTED_EDGE('',*,*,#8833,.F.);
#12333=ORIENTED_EDGE('',*,*,#8834,.F.);
#12334=ORIENTED_EDGE('',*,*,#8835,.F.);
#12335=ORIENTED_EDGE('',*,*,#8513,.F.);
#12336=ORIENTED_EDGE('',*,*,#8835,.T.);
#12337=ORIENTED_EDGE('',*,*,#8836,.F.);
#12338=ORIENTED_EDGE('',*,*,#8837,.F.);
#12339=ORIENTED_EDGE('',*,*,#8514,.F.);
#12340=ORIENTED_EDGE('',*,*,#8838,.F.);
#12341=ORIENTED_EDGE('',*,*,#8515,.F.);
#12342=ORIENTED_EDGE('',*,*,#8837,.T.);
#12343=ORIENTED_EDGE('',*,*,#8839,.F.);
#12344=ORIENTED_EDGE('',*,*,#8838,.T.);
#12345=ORIENTED_EDGE('',*,*,#8840,.F.);
#12346=ORIENTED_EDGE('',*,*,#8841,.T.);
#12347=ORIENTED_EDGE('',*,*,#8516,.F.);
#12348=ORIENTED_EDGE('',*,*,#8842,.F.);
#12349=ORIENTED_EDGE('',*,*,#8519,.F.);
#12350=ORIENTED_EDGE('',*,*,#8843,.T.);
#12351=ORIENTED_EDGE('',*,*,#8844,.F.);
#12352=ORIENTED_EDGE('',*,*,#8841,.F.);
#12353=ORIENTED_EDGE('',*,*,#8845,.F.);
#12354=ORIENTED_EDGE('',*,*,#8846,.F.);
#12355=ORIENTED_EDGE('',*,*,#8517,.F.);
#12356=ORIENTED_EDGE('',*,*,#8846,.T.);
#12357=ORIENTED_EDGE('',*,*,#8847,.F.);
#12358=ORIENTED_EDGE('',*,*,#8843,.F.);
#12359=ORIENTED_EDGE('',*,*,#8518,.F.);
#12360=ORIENTED_EDGE('',*,*,#8534,.T.);
#12361=ORIENTED_EDGE('',*,*,#8535,.T.);
#12362=ORIENTED_EDGE('',*,*,#8530,.T.);
#12363=ORIENTED_EDGE('',*,*,#8848,.T.);
#12364=ORIENTED_EDGE('',*,*,#8844,.T.);
#12365=ORIENTED_EDGE('',*,*,#8847,.T.);
#12366=ORIENTED_EDGE('',*,*,#8845,.T.);
#12367=ORIENTED_EDGE('',*,*,#8840,.T.);
#12368=ORIENTED_EDGE('',*,*,#8839,.T.);
#12369=ORIENTED_EDGE('',*,*,#8836,.T.);
#12370=ORIENTED_EDGE('',*,*,#8834,.T.);
#12371=ORIENTED_EDGE('',*,*,#8832,.T.);
#12372=ORIENTED_EDGE('',*,*,#8830,.T.);
#12373=ORIENTED_EDGE('',*,*,#8831,.T.);
#12374=ORIENTED_EDGE('',*,*,#8826,.T.);
#12375=ORIENTED_EDGE('',*,*,#8824,.T.);
#12376=ORIENTED_EDGE('',*,*,#8822,.T.);
#12377=ORIENTED_EDGE('',*,*,#8823,.T.);
#12378=ORIENTED_EDGE('',*,*,#8818,.T.);
#12379=ORIENTED_EDGE('',*,*,#8816,.T.);
#12380=ORIENTED_EDGE('',*,*,#8814,.T.);
#12381=ORIENTED_EDGE('',*,*,#8815,.T.);
#12382=ORIENTED_EDGE('',*,*,#8810,.T.);
#12383=ORIENTED_EDGE('',*,*,#8808,.T.);
#12384=ORIENTED_EDGE('',*,*,#8806,.T.);
#12385=ORIENTED_EDGE('',*,*,#8807,.T.);
#12386=ORIENTED_EDGE('',*,*,#8802,.T.);
#12387=ORIENTED_EDGE('',*,*,#8800,.T.);
#12388=ORIENTED_EDGE('',*,*,#8798,.T.);
#12389=ORIENTED_EDGE('',*,*,#8799,.T.);
#12390=ORIENTED_EDGE('',*,*,#8794,.T.);
#12391=ORIENTED_EDGE('',*,*,#8792,.T.);
#12392=ORIENTED_EDGE('',*,*,#8790,.T.);
#12393=ORIENTED_EDGE('',*,*,#8791,.T.);
#12394=ORIENTED_EDGE('',*,*,#8786,.T.);
#12395=ORIENTED_EDGE('',*,*,#8784,.T.);
#12396=ORIENTED_EDGE('',*,*,#8782,.T.);
#12397=ORIENTED_EDGE('',*,*,#8783,.T.);
#12398=ORIENTED_EDGE('',*,*,#8778,.T.);
#12399=ORIENTED_EDGE('',*,*,#8776,.T.);
#12400=ORIENTED_EDGE('',*,*,#8774,.T.);
#12401=ORIENTED_EDGE('',*,*,#8775,.T.);
#12402=ORIENTED_EDGE('',*,*,#8770,.T.);
#12403=ORIENTED_EDGE('',*,*,#8768,.T.);
#12404=ORIENTED_EDGE('',*,*,#8766,.T.);
#12405=ORIENTED_EDGE('',*,*,#8767,.T.);
#12406=ORIENTED_EDGE('',*,*,#8762,.T.);
#12407=ORIENTED_EDGE('',*,*,#8760,.T.);
#12408=ORIENTED_EDGE('',*,*,#8758,.T.);
#12409=ORIENTED_EDGE('',*,*,#8759,.T.);
#12410=ORIENTED_EDGE('',*,*,#8754,.T.);
#12411=ORIENTED_EDGE('',*,*,#8752,.T.);
#12412=ORIENTED_EDGE('',*,*,#8750,.T.);
#12413=ORIENTED_EDGE('',*,*,#8751,.T.);
#12414=ORIENTED_EDGE('',*,*,#8746,.T.);
#12415=ORIENTED_EDGE('',*,*,#8744,.T.);
#12416=ORIENTED_EDGE('',*,*,#8742,.T.);
#12417=ORIENTED_EDGE('',*,*,#8743,.T.);
#12418=ORIENTED_EDGE('',*,*,#8738,.T.);
#12419=ORIENTED_EDGE('',*,*,#8736,.T.);
#12420=ORIENTED_EDGE('',*,*,#8734,.T.);
#12421=ORIENTED_EDGE('',*,*,#8735,.T.);
#12422=ORIENTED_EDGE('',*,*,#8730,.T.);
#12423=ORIENTED_EDGE('',*,*,#8728,.T.);
#12424=ORIENTED_EDGE('',*,*,#8726,.T.);
#12425=ORIENTED_EDGE('',*,*,#8727,.T.);
#12426=ORIENTED_EDGE('',*,*,#8722,.T.);
#12427=ORIENTED_EDGE('',*,*,#8720,.T.);
#12428=ORIENTED_EDGE('',*,*,#8718,.T.);
#12429=ORIENTED_EDGE('',*,*,#8719,.T.);
#12430=ORIENTED_EDGE('',*,*,#8714,.T.);
#12431=ORIENTED_EDGE('',*,*,#8712,.T.);
#12432=ORIENTED_EDGE('',*,*,#8710,.T.);
#12433=ORIENTED_EDGE('',*,*,#8711,.T.);
#12434=ORIENTED_EDGE('',*,*,#8706,.T.);
#12435=ORIENTED_EDGE('',*,*,#8704,.T.);
#12436=ORIENTED_EDGE('',*,*,#8702,.T.);
#12437=ORIENTED_EDGE('',*,*,#8703,.T.);
#12438=ORIENTED_EDGE('',*,*,#8698,.T.);
#12439=ORIENTED_EDGE('',*,*,#8696,.T.);
#12440=ORIENTED_EDGE('',*,*,#8694,.T.);
#12441=ORIENTED_EDGE('',*,*,#8695,.T.);
#12442=ORIENTED_EDGE('',*,*,#8690,.T.);
#12443=ORIENTED_EDGE('',*,*,#8688,.T.);
#12444=ORIENTED_EDGE('',*,*,#8686,.T.);
#12445=ORIENTED_EDGE('',*,*,#8687,.T.);
#12446=ORIENTED_EDGE('',*,*,#8682,.T.);
#12447=ORIENTED_EDGE('',*,*,#8680,.T.);
#12448=ORIENTED_EDGE('',*,*,#8678,.T.);
#12449=ORIENTED_EDGE('',*,*,#8679,.T.);
#12450=ORIENTED_EDGE('',*,*,#8674,.T.);
#12451=ORIENTED_EDGE('',*,*,#8672,.T.);
#12452=ORIENTED_EDGE('',*,*,#8670,.T.);
#12453=ORIENTED_EDGE('',*,*,#8671,.T.);
#12454=ORIENTED_EDGE('',*,*,#8666,.T.);
#12455=ORIENTED_EDGE('',*,*,#8664,.T.);
#12456=ORIENTED_EDGE('',*,*,#8662,.T.);
#12457=ORIENTED_EDGE('',*,*,#8663,.T.);
#12458=ORIENTED_EDGE('',*,*,#8658,.T.);
#12459=ORIENTED_EDGE('',*,*,#8656,.T.);
#12460=ORIENTED_EDGE('',*,*,#8654,.T.);
#12461=ORIENTED_EDGE('',*,*,#8655,.T.);
#12462=ORIENTED_EDGE('',*,*,#8650,.T.);
#12463=ORIENTED_EDGE('',*,*,#8648,.T.);
#12464=ORIENTED_EDGE('',*,*,#8646,.T.);
#12465=ORIENTED_EDGE('',*,*,#8647,.T.);
#12466=ORIENTED_EDGE('',*,*,#8642,.T.);
#12467=ORIENTED_EDGE('',*,*,#8640,.T.);
#12468=ORIENTED_EDGE('',*,*,#8638,.T.);
#12469=ORIENTED_EDGE('',*,*,#8639,.T.);
#12470=ORIENTED_EDGE('',*,*,#8634,.T.);
#12471=ORIENTED_EDGE('',*,*,#8632,.T.);
#12472=ORIENTED_EDGE('',*,*,#8630,.T.);
#12473=ORIENTED_EDGE('',*,*,#8631,.T.);
#12474=ORIENTED_EDGE('',*,*,#8626,.T.);
#12475=ORIENTED_EDGE('',*,*,#8624,.T.);
#12476=ORIENTED_EDGE('',*,*,#8622,.T.);
#12477=ORIENTED_EDGE('',*,*,#8623,.T.);
#12478=ORIENTED_EDGE('',*,*,#8618,.T.);
#12479=ORIENTED_EDGE('',*,*,#8616,.T.);
#12480=ORIENTED_EDGE('',*,*,#8614,.T.);
#12481=ORIENTED_EDGE('',*,*,#8615,.T.);
#12482=ORIENTED_EDGE('',*,*,#8610,.T.);
#12483=ORIENTED_EDGE('',*,*,#8608,.T.);
#12484=ORIENTED_EDGE('',*,*,#8606,.T.);
#12485=ORIENTED_EDGE('',*,*,#8607,.T.);
#12486=ORIENTED_EDGE('',*,*,#8602,.T.);
#12487=ORIENTED_EDGE('',*,*,#8600,.T.);
#12488=ORIENTED_EDGE('',*,*,#8598,.T.);
#12489=ORIENTED_EDGE('',*,*,#8599,.T.);
#12490=ORIENTED_EDGE('',*,*,#8594,.T.);
#12491=ORIENTED_EDGE('',*,*,#8592,.T.);
#12492=ORIENTED_EDGE('',*,*,#8590,.T.);
#12493=ORIENTED_EDGE('',*,*,#8591,.T.);
#12494=ORIENTED_EDGE('',*,*,#8586,.T.);
#12495=ORIENTED_EDGE('',*,*,#8584,.T.);
#12496=ORIENTED_EDGE('',*,*,#8582,.T.);
#12497=ORIENTED_EDGE('',*,*,#8583,.T.);
#12498=ORIENTED_EDGE('',*,*,#8578,.T.);
#12499=ORIENTED_EDGE('',*,*,#8576,.T.);
#12500=ORIENTED_EDGE('',*,*,#8574,.T.);
#12501=ORIENTED_EDGE('',*,*,#8575,.T.);
#12502=ORIENTED_EDGE('',*,*,#8570,.T.);
#12503=ORIENTED_EDGE('',*,*,#8568,.T.);
#12504=ORIENTED_EDGE('',*,*,#8566,.T.);
#12505=ORIENTED_EDGE('',*,*,#8567,.T.);
#12506=ORIENTED_EDGE('',*,*,#8562,.T.);
#12507=ORIENTED_EDGE('',*,*,#8560,.T.);
#12508=ORIENTED_EDGE('',*,*,#8558,.T.);
#12509=ORIENTED_EDGE('',*,*,#8559,.T.);
#12510=ORIENTED_EDGE('',*,*,#8554,.T.);
#12511=ORIENTED_EDGE('',*,*,#8552,.T.);
#12512=ORIENTED_EDGE('',*,*,#8550,.T.);
#12513=ORIENTED_EDGE('',*,*,#8551,.T.);
#12514=ORIENTED_EDGE('',*,*,#8546,.T.);
#12515=ORIENTED_EDGE('',*,*,#8544,.T.);
#12516=ORIENTED_EDGE('',*,*,#8542,.T.);
#12517=ORIENTED_EDGE('',*,*,#8543,.T.);
#12518=ORIENTED_EDGE('',*,*,#8538,.T.);
#12519=ORIENTED_EDGE('',*,*,#8536,.T.);
#12520=ORIENTED_EDGE('',*,*,#8528,.T.);
#12521=ORIENTED_EDGE('',*,*,#8529,.T.);
#12522=ORIENTED_EDGE('',*,*,#8520,.F.);
#12523=ORIENTED_EDGE('',*,*,#8842,.T.);
#12524=ORIENTED_EDGE('',*,*,#8848,.F.);
#12767=CYLINDRICAL_SURFACE('',#15352,1.);
#12768=CYLINDRICAL_SURFACE('',#15354,2.);
#12769=CYLINDRICAL_SURFACE('',#15359,3.75);
#12770=CYLINDRICAL_SURFACE('',#15362,3.75);
#12771=CYLINDRICAL_SURFACE('',#15365,3.75);
#12772=CYLINDRICAL_SURFACE('',#15368,3.75);
#12773=CYLINDRICAL_SURFACE('',#15371,3.75);
#12774=CYLINDRICAL_SURFACE('',#15374,3.75);
#12775=CYLINDRICAL_SURFACE('',#15377,3.75);
#12776=CYLINDRICAL_SURFACE('',#15380,3.75);
#12777=CYLINDRICAL_SURFACE('',#15383,3.75);
#12778=CYLINDRICAL_SURFACE('',#15386,3.75);
#12779=CYLINDRICAL_SURFACE('',#15389,3.75);
#12780=CYLINDRICAL_SURFACE('',#15392,3.75);
#12781=CYLINDRICAL_SURFACE('',#15395,3.75);
#12782=CYLINDRICAL_SURFACE('',#15398,3.75);
#12783=CYLINDRICAL_SURFACE('',#15401,3.75);
#12784=CYLINDRICAL_SURFACE('',#15404,3.75);
#12785=CYLINDRICAL_SURFACE('',#15407,3.75);
#12786=CYLINDRICAL_SURFACE('',#15410,3.75);
#12787=CYLINDRICAL_SURFACE('',#15413,3.75);
#12788=CYLINDRICAL_SURFACE('',#15416,3.75);
#12789=CYLINDRICAL_SURFACE('',#15419,3.75);
#12790=CYLINDRICAL_SURFACE('',#15422,3.75);
#12791=CYLINDRICAL_SURFACE('',#15425,3.75);
#12792=CYLINDRICAL_SURFACE('',#15428,3.75);
#12793=CYLINDRICAL_SURFACE('',#15431,3.75);
#12794=CYLINDRICAL_SURFACE('',#15434,3.75);
#12795=CYLINDRICAL_SURFACE('',#15437,3.75);
#12796=CYLINDRICAL_SURFACE('',#15440,3.75);
#12797=CYLINDRICAL_SURFACE('',#15443,3.75);
#12798=CYLINDRICAL_SURFACE('',#15446,3.75);
#12799=CYLINDRICAL_SURFACE('',#15449,3.75);
#12800=CYLINDRICAL_SURFACE('',#15452,3.75);
#12801=CYLINDRICAL_SURFACE('',#15455,3.75);
#12802=CYLINDRICAL_SURFACE('',#15458,3.75);
#12803=CYLINDRICAL_SURFACE('',#15461,3.75);
#12804=CYLINDRICAL_SURFACE('',#15464,3.75);
#12805=CYLINDRICAL_SURFACE('',#15467,3.75);
#12806=CYLINDRICAL_SURFACE('',#15470,3.75);
#12807=CYLINDRICAL_SURFACE('',#15473,3.75);
#12808=CYLINDRICAL_SURFACE('',#15478,3.75);
#13392=ADVANCED_FACE('',(#2275),#1637,.F.);
#13393=ADVANCED_FACE('',(#2276),#1638,.F.);
#13394=ADVANCED_FACE('',(#2277),#1639,.F.);
#13395=ADVANCED_FACE('',(#2278,#1326),#1640,.F.);
#13396=ADVANCED_FACE('',(#2279),#12767,.F.);
#13397=ADVANCED_FACE('',(#2280),#12768,.T.);
#13398=ADVANCED_FACE('',(#2281,#1327),#1641,.T.);
#13399=ADVANCED_FACE('',(#2282),#51,.T.);
#13400=ADVANCED_FACE('',(#2283),#52,.T.);
#13401=ADVANCED_FACE('',(#2284),#1642,.T.);
#13402=ADVANCED_FACE('',(#2285),#12769,.T.);
#13403=ADVANCED_FACE('',(#2286),#53,.T.);
#13404=ADVANCED_FACE('',(#2287),#54,.T.);
#13405=ADVANCED_FACE('',(#2288),#1643,.T.);
#13406=ADVANCED_FACE('',(#2289),#12770,.T.);
#13407=ADVANCED_FACE('',(#2290),#55,.T.);
#13408=ADVANCED_FACE('',(#2291),#56,.T.);
#13409=ADVANCED_FACE('',(#2292),#1644,.T.);
#13410=ADVANCED_FACE('',(#2293),#12771,.T.);
#13411=ADVANCED_FACE('',(#2294),#57,.T.);
#13412=ADVANCED_FACE('',(#2295),#58,.T.);
#13413=ADVANCED_FACE('',(#2296),#1645,.T.);
#13414=ADVANCED_FACE('',(#2297),#12772,.T.);
#13415=ADVANCED_FACE('',(#2298),#59,.T.);
#13416=ADVANCED_FACE('',(#2299),#60,.T.);
#13417=ADVANCED_FACE('',(#2300),#1646,.T.);
#13418=ADVANCED_FACE('',(#2301),#12773,.T.);
#13419=ADVANCED_FACE('',(#2302),#61,.T.);
#13420=ADVANCED_FACE('',(#2303),#62,.T.);
#13421=ADVANCED_FACE('',(#2304),#1647,.T.);
#13422=ADVANCED_FACE('',(#2305),#12774,.T.);
#13423=ADVANCED_FACE('',(#2306),#63,.T.);
#13424=ADVANCED_FACE('',(#2307),#64,.T.);
#13425=ADVANCED_FACE('',(#2308),#1648,.T.);
#13426=ADVANCED_FACE('',(#2309),#12775,.T.);
#13427=ADVANCED_FACE('',(#2310),#65,.T.);
#13428=ADVANCED_FACE('',(#2311),#66,.T.);
#13429=ADVANCED_FACE('',(#2312),#1649,.T.);
#13430=ADVANCED_FACE('',(#2313),#12776,.T.);
#13431=ADVANCED_FACE('',(#2314),#67,.T.);
#13432=ADVANCED_FACE('',(#2315),#68,.T.);
#13433=ADVANCED_FACE('',(#2316),#1650,.T.);
#13434=ADVANCED_FACE('',(#2317),#12777,.T.);
#13435=ADVANCED_FACE('',(#2318),#69,.T.);
#13436=ADVANCED_FACE('',(#2319),#70,.T.);
#13437=ADVANCED_FACE('',(#2320),#1651,.T.);
#13438=ADVANCED_FACE('',(#2321),#12778,.T.);
#13439=ADVANCED_FACE('',(#2322),#71,.T.);
#13440=ADVANCED_FACE('',(#2323),#72,.T.);
#13441=ADVANCED_FACE('',(#2324),#1652,.T.);
#13442=ADVANCED_FACE('',(#2325),#12779,.T.);
#13443=ADVANCED_FACE('',(#2326),#73,.T.);
#13444=ADVANCED_FACE('',(#2327),#74,.T.);
#13445=ADVANCED_FACE('',(#2328),#1653,.T.);
#13446=ADVANCED_FACE('',(#2329),#12780,.T.);
#13447=ADVANCED_FACE('',(#2330),#75,.T.);
#13448=ADVANCED_FACE('',(#2331),#76,.T.);
#13449=ADVANCED_FACE('',(#2332),#1654,.T.);
#13450=ADVANCED_FACE('',(#2333),#12781,.T.);
#13451=ADVANCED_FACE('',(#2334),#77,.T.);
#13452=ADVANCED_FACE('',(#2335),#78,.T.);
#13453=ADVANCED_FACE('',(#2336),#1655,.T.);
#13454=ADVANCED_FACE('',(#2337),#12782,.T.);
#13455=ADVANCED_FACE('',(#2338),#79,.T.);
#13456=ADVANCED_FACE('',(#2339),#80,.T.);
#13457=ADVANCED_FACE('',(#2340),#1656,.T.);
#13458=ADVANCED_FACE('',(#2341),#12783,.T.);
#13459=ADVANCED_FACE('',(#2342),#81,.T.);
#13460=ADVANCED_FACE('',(#2343),#82,.T.);
#13461=ADVANCED_FACE('',(#2344),#1657,.T.);
#13462=ADVANCED_FACE('',(#2345),#12784,.T.);
#13463=ADVANCED_FACE('',(#2346),#83,.T.);
#13464=ADVANCED_FACE('',(#2347),#84,.T.);
#13465=ADVANCED_FACE('',(#2348),#1658,.T.);
#13466=ADVANCED_FACE('',(#2349),#12785,.T.);
#13467=ADVANCED_FACE('',(#2350),#85,.T.);
#13468=ADVANCED_FACE('',(#2351),#86,.T.);
#13469=ADVANCED_FACE('',(#2352),#1659,.T.);
#13470=ADVANCED_FACE('',(#2353),#12786,.T.);
#13471=ADVANCED_FACE('',(#2354),#87,.T.);
#13472=ADVANCED_FACE('',(#2355),#88,.T.);
#13473=ADVANCED_FACE('',(#2356),#1660,.T.);
#13474=ADVANCED_FACE('',(#2357),#12787,.T.);
#13475=ADVANCED_FACE('',(#2358),#89,.T.);
#13476=ADVANCED_FACE('',(#2359),#90,.T.);
#13477=ADVANCED_FACE('',(#2360),#1661,.T.);
#13478=ADVANCED_FACE('',(#2361),#12788,.T.);
#13479=ADVANCED_FACE('',(#2362),#91,.T.);
#13480=ADVANCED_FACE('',(#2363),#92,.T.);
#13481=ADVANCED_FACE('',(#2364),#1662,.T.);
#13482=ADVANCED_FACE('',(#2365),#12789,.T.);
#13483=ADVANCED_FACE('',(#2366),#93,.T.);
#13484=ADVANCED_FACE('',(#2367),#94,.T.);
#13485=ADVANCED_FACE('',(#2368),#1663,.T.);
#13486=ADVANCED_FACE('',(#2369),#12790,.T.);
#13487=ADVANCED_FACE('',(#2370),#95,.T.);
#13488=ADVANCED_FACE('',(#2371),#96,.T.);
#13489=ADVANCED_FACE('',(#2372),#1664,.T.);
#13490=ADVANCED_FACE('',(#2373),#12791,.T.);
#13491=ADVANCED_FACE('',(#2374),#97,.T.);
#13492=ADVANCED_FACE('',(#2375),#98,.T.);
#13493=ADVANCED_FACE('',(#2376),#1665,.T.);
#13494=ADVANCED_FACE('',(#2377),#12792,.T.);
#13495=ADVANCED_FACE('',(#2378),#99,.T.);
#13496=ADVANCED_FACE('',(#2379),#100,.T.);
#13497=ADVANCED_FACE('',(#2380),#1666,.T.);
#13498=ADVANCED_FACE('',(#2381),#12793,.T.);
#13499=ADVANCED_FACE('',(#2382),#101,.T.);
#13500=ADVANCED_FACE('',(#2383),#102,.T.);
#13501=ADVANCED_FACE('',(#2384),#1667,.T.);
#13502=ADVANCED_FACE('',(#2385),#12794,.T.);
#13503=ADVANCED_FACE('',(#2386),#103,.T.);
#13504=ADVANCED_FACE('',(#2387),#104,.T.);
#13505=ADVANCED_FACE('',(#2388),#1668,.T.);
#13506=ADVANCED_FACE('',(#2389),#12795,.T.);
#13507=ADVANCED_FACE('',(#2390),#105,.T.);
#13508=ADVANCED_FACE('',(#2391),#106,.T.);
#13509=ADVANCED_FACE('',(#2392),#1669,.T.);
#13510=ADVANCED_FACE('',(#2393),#12796,.T.);
#13511=ADVANCED_FACE('',(#2394),#107,.T.);
#13512=ADVANCED_FACE('',(#2395),#108,.T.);
#13513=ADVANCED_FACE('',(#2396),#1670,.T.);
#13514=ADVANCED_FACE('',(#2397),#12797,.T.);
#13515=ADVANCED_FACE('',(#2398),#109,.T.);
#13516=ADVANCED_FACE('',(#2399),#110,.T.);
#13517=ADVANCED_FACE('',(#2400),#1671,.T.);
#13518=ADVANCED_FACE('',(#2401),#12798,.T.);
#13519=ADVANCED_FACE('',(#2402),#111,.T.);
#13520=ADVANCED_FACE('',(#2403),#112,.T.);
#13521=ADVANCED_FACE('',(#2404),#1672,.T.);
#13522=ADVANCED_FACE('',(#2405),#12799,.T.);
#13523=ADVANCED_FACE('',(#2406),#113,.T.);
#13524=ADVANCED_FACE('',(#2407),#114,.T.);
#13525=ADVANCED_FACE('',(#2408),#1673,.T.);
#13526=ADVANCED_FACE('',(#2409),#12800,.T.);
#13527=ADVANCED_FACE('',(#2410),#115,.T.);
#13528=ADVANCED_FACE('',(#2411),#116,.T.);
#13529=ADVANCED_FACE('',(#2412),#1674,.T.);
#13530=ADVANCED_FACE('',(#2413),#12801,.T.);
#13531=ADVANCED_FACE('',(#2414),#117,.T.);
#13532=ADVANCED_FACE('',(#2415),#118,.T.);
#13533=ADVANCED_FACE('',(#2416),#1675,.T.);
#13534=ADVANCED_FACE('',(#2417),#12802,.T.);
#13535=ADVANCED_FACE('',(#2418),#119,.T.);
#13536=ADVANCED_FACE('',(#2419),#120,.T.);
#13537=ADVANCED_FACE('',(#2420),#1676,.T.);
#13538=ADVANCED_FACE('',(#2421),#12803,.T.);
#13539=ADVANCED_FACE('',(#2422),#121,.T.);
#13540=ADVANCED_FACE('',(#2423),#122,.T.);
#13541=ADVANCED_FACE('',(#2424),#1677,.T.);
#13542=ADVANCED_FACE('',(#2425),#12804,.T.);
#13543=ADVANCED_FACE('',(#2426),#123,.T.);
#13544=ADVANCED_FACE('',(#2427),#124,.T.);
#13545=ADVANCED_FACE('',(#2428),#1678,.T.);
#13546=ADVANCED_FACE('',(#2429),#12805,.T.);
#13547=ADVANCED_FACE('',(#2430),#125,.T.);
#13548=ADVANCED_FACE('',(#2431),#126,.T.);
#13549=ADVANCED_FACE('',(#2432),#1679,.T.);
#13550=ADVANCED_FACE('',(#2433),#12806,.T.);
#13551=ADVANCED_FACE('',(#2434),#127,.T.);
#13552=ADVANCED_FACE('',(#2435),#1680,.T.);
#13553=ADVANCED_FACE('',(#2436),#128,.T.);
#13554=ADVANCED_FACE('',(#2437),#12807,.T.);
#13555=ADVANCED_FACE('',(#2438),#129,.T.);
#13556=ADVANCED_FACE('',(#2439),#130,.T.);
#13557=ADVANCED_FACE('',(#2440),#1681,.T.);
#13558=ADVANCED_FACE('',(#2441,#1328),#1682,.T.);
#13559=ADVANCED_FACE('',(#2442),#12808,.T.);
#13641=CLOSED_SHELL('',(#13392,#13393,#13394,#13395,#13396,#13397,#13398,
#13399,#13400,#13401,#13402,#13403,#13404,#13405,#13406,#13407,#13408,#13409,
#13410,#13411,#13412,#13413,#13414,#13415,#13416,#13417,#13418,#13419,#13420,
#13421,#13422,#13423,#13424,#13425,#13426,#13427,#13428,#13429,#13430,#13431,
#13432,#13433,#13434,#13435,#13436,#13437,#13438,#13439,#13440,#13441,#13442,
#13443,#13444,#13445,#13446,#13447,#13448,#13449,#13450,#13451,#13452,#13453,
#13454,#13455,#13456,#13457,#13458,#13459,#13460,#13461,#13462,#13463,#13464,
#13465,#13466,#13467,#13468,#13469,#13470,#13471,#13472,#13473,#13474,#13475,
#13476,#13477,#13478,#13479,#13480,#13481,#13482,#13483,#13484,#13485,#13486,
#13487,#13488,#13489,#13490,#13491,#13492,#13493,#13494,#13495,#13496,#13497,
#13498,#13499,#13500,#13501,#13502,#13503,#13504,#13505,#13506,#13507,#13508,
#13509,#13510,#13511,#13512,#13513,#13514,#13515,#13516,#13517,#13518,#13519,
#13520,#13521,#13522,#13523,#13524,#13525,#13526,#13527,#13528,#13529,#13530,
#13531,#13532,#13533,#13534,#13535,#13536,#13537,#13538,#13539,#13540,#13541,
#13542,#13543,#13544,#13545,#13546,#13547,#13548,#13549,#13550,#13551,#13552,
#13553,#13554,#13555,#13556,#13557,#13558,#13559));
#15306=AXIS2_PLACEMENT_3D('',#34088,#18495,#18496);
#15307=AXIS2_PLACEMENT_3D('',#34089,#18497,#18498);
#15308=AXIS2_PLACEMENT_3D('',#34098,#18503,#18504);
#15309=AXIS2_PLACEMENT_3D('',#34104,#18508,#18509);
#15310=AXIS2_PLACEMENT_3D('',#34110,#18513,#18514);
#15311=AXIS2_PLACEMENT_3D('',#34113,#18515,#18516);
#15312=AXIS2_PLACEMENT_3D('',#34259,#18518,#18519);
#15313=AXIS2_PLACEMENT_3D('',#34405,#18521,#18522);
#15314=AXIS2_PLACEMENT_3D('',#34551,#18524,#18525);
#15315=AXIS2_PLACEMENT_3D('',#34697,#18527,#18528);
#15316=AXIS2_PLACEMENT_3D('',#34843,#18530,#18531);
#15317=AXIS2_PLACEMENT_3D('',#34989,#18533,#18534);
#15318=AXIS2_PLACEMENT_3D('',#35135,#18536,#18537);
#15319=AXIS2_PLACEMENT_3D('',#35281,#18539,#18540);
#15320=AXIS2_PLACEMENT_3D('',#35427,#18542,#18543);
#15321=AXIS2_PLACEMENT_3D('',#35573,#18545,#18546);
#15322=AXIS2_PLACEMENT_3D('',#35719,#18548,#18549);
#15323=AXIS2_PLACEMENT_3D('',#35865,#18551,#18552);
#15324=AXIS2_PLACEMENT_3D('',#36011,#18554,#18555);
#15325=AXIS2_PLACEMENT_3D('',#36157,#18557,#18558);
#15326=AXIS2_PLACEMENT_3D('',#36303,#18560,#18561);
#15327=AXIS2_PLACEMENT_3D('',#36449,#18563,#18564);
#15328=AXIS2_PLACEMENT_3D('',#36595,#18566,#18567);
#15329=AXIS2_PLACEMENT_3D('',#36741,#18569,#18570);
#15330=AXIS2_PLACEMENT_3D('',#36887,#18572,#18573);
#15331=AXIS2_PLACEMENT_3D('',#37033,#18575,#18576);
#15332=AXIS2_PLACEMENT_3D('',#37179,#18578,#18579);
#15333=AXIS2_PLACEMENT_3D('',#37325,#18581,#18582);
#15334=AXIS2_PLACEMENT_3D('',#37471,#18584,#18585);
#15335=AXIS2_PLACEMENT_3D('',#37617,#18587,#18588);
#15336=AXIS2_PLACEMENT_3D('',#37763,#18590,#18591);
#15337=AXIS2_PLACEMENT_3D('',#37909,#18593,#18594);
#15338=AXIS2_PLACEMENT_3D('',#38055,#18596,#18597);
#15339=AXIS2_PLACEMENT_3D('',#38201,#18599,#18600);
#15340=AXIS2_PLACEMENT_3D('',#38347,#18602,#18603);
#15341=AXIS2_PLACEMENT_3D('',#38493,#18605,#18606);
#15342=AXIS2_PLACEMENT_3D('',#38639,#18608,#18609);
#15343=AXIS2_PLACEMENT_3D('',#38785,#18611,#18612);
#15344=AXIS2_PLACEMENT_3D('',#38931,#18614,#18615);
#15345=AXIS2_PLACEMENT_3D('',#39077,#18617,#18618);
#15346=AXIS2_PLACEMENT_3D('',#39223,#18620,#18621);
#15347=AXIS2_PLACEMENT_3D('',#39369,#18623,#18624);
#15348=AXIS2_PLACEMENT_3D('',#39515,#18626,#18627);
#15349=AXIS2_PLACEMENT_3D('',#39661,#18629,#18630);
#15350=AXIS2_PLACEMENT_3D('',#39807,#18632,#18633);
#15351=AXIS2_PLACEMENT_3D('',#39951,#18635,#18636);
#15352=AXIS2_PLACEMENT_3D('',#39952,#18637,#18638);
#15353=AXIS2_PLACEMENT_3D('',#39953,#18639,#18640);
#15354=AXIS2_PLACEMENT_3D('',#39954,#18641,#18642);
#15355=AXIS2_PLACEMENT_3D('',#39956,#18643,#18644);
#15356=AXIS2_PLACEMENT_3D('',#39959,#18646,#18647);
#15357=AXIS2_PLACEMENT_3D('',#39960,#18648,#18649);
#15358=AXIS2_PLACEMENT_3D('',#40399,#18652,#18653);
#15359=AXIS2_PLACEMENT_3D('',#40401,#18655,#18656);
#15360=AXIS2_PLACEMENT_3D('',#40403,#18657,#18658);
#15361=AXIS2_PLACEMENT_3D('',#40841,#18661,#18662);
#15362=AXIS2_PLACEMENT_3D('',#40843,#18664,#18665);
#15363=AXIS2_PLACEMENT_3D('',#40845,#18666,#18667);
#15364=AXIS2_PLACEMENT_3D('',#41283,#18670,#18671);
#15365=AXIS2_PLACEMENT_3D('',#41285,#18673,#18674);
#15366=AXIS2_PLACEMENT_3D('',#41287,#18675,#18676);
#15367=AXIS2_PLACEMENT_3D('',#41725,#18679,#18680);
#15368=AXIS2_PLACEMENT_3D('',#41727,#18682,#18683);
#15369=AXIS2_PLACEMENT_3D('',#41729,#18684,#18685);
#15370=AXIS2_PLACEMENT_3D('',#42167,#18688,#18689);
#15371=AXIS2_PLACEMENT_3D('',#42169,#18691,#18692);
#15372=AXIS2_PLACEMENT_3D('',#42171,#18693,#18694);
#15373=AXIS2_PLACEMENT_3D('',#42609,#18697,#18698);
#15374=AXIS2_PLACEMENT_3D('',#42611,#18700,#18701);
#15375=AXIS2_PLACEMENT_3D('',#42613,#18702,#18703);
#15376=AXIS2_PLACEMENT_3D('',#43051,#18706,#18707);
#15377=AXIS2_PLACEMENT_3D('',#43053,#18709,#18710);
#15378=AXIS2_PLACEMENT_3D('',#43055,#18711,#18712);
#15379=AXIS2_PLACEMENT_3D('',#43493,#18715,#18716);
#15380=AXIS2_PLACEMENT_3D('',#43495,#18718,#18719);
#15381=AXIS2_PLACEMENT_3D('',#43497,#18720,#18721);
#15382=AXIS2_PLACEMENT_3D('',#43935,#18724,#18725);
#15383=AXIS2_PLACEMENT_3D('',#43937,#18727,#18728);
#15384=AXIS2_PLACEMENT_3D('',#43939,#18729,#18730);
#15385=AXIS2_PLACEMENT_3D('',#44377,#18733,#18734);
#15386=AXIS2_PLACEMENT_3D('',#44379,#18736,#18737);
#15387=AXIS2_PLACEMENT_3D('',#44381,#18738,#18739);
#15388=AXIS2_PLACEMENT_3D('',#44819,#18742,#18743);
#15389=AXIS2_PLACEMENT_3D('',#44821,#18745,#18746);
#15390=AXIS2_PLACEMENT_3D('',#44823,#18747,#18748);
#15391=AXIS2_PLACEMENT_3D('',#45261,#18751,#18752);
#15392=AXIS2_PLACEMENT_3D('',#45263,#18754,#18755);
#15393=AXIS2_PLACEMENT_3D('',#45265,#18756,#18757);
#15394=AXIS2_PLACEMENT_3D('',#45703,#18760,#18761);
#15395=AXIS2_PLACEMENT_3D('',#45705,#18763,#18764);
#15396=AXIS2_PLACEMENT_3D('',#45707,#18765,#18766);
#15397=AXIS2_PLACEMENT_3D('',#46145,#18769,#18770);
#15398=AXIS2_PLACEMENT_3D('',#46147,#18772,#18773);
#15399=AXIS2_PLACEMENT_3D('',#46149,#18774,#18775);
#15400=AXIS2_PLACEMENT_3D('',#46587,#18778,#18779);
#15401=AXIS2_PLACEMENT_3D('',#46589,#18781,#18782);
#15402=AXIS2_PLACEMENT_3D('',#46591,#18783,#18784);
#15403=AXIS2_PLACEMENT_3D('',#47029,#18787,#18788);
#15404=AXIS2_PLACEMENT_3D('',#47031,#18790,#18791);
#15405=AXIS2_PLACEMENT_3D('',#47033,#18792,#18793);
#15406=AXIS2_PLACEMENT_3D('',#47471,#18796,#18797);
#15407=AXIS2_PLACEMENT_3D('',#47473,#18799,#18800);
#15408=AXIS2_PLACEMENT_3D('',#47475,#18801,#18802);
#15409=AXIS2_PLACEMENT_3D('',#47913,#18805,#18806);
#15410=AXIS2_PLACEMENT_3D('',#47915,#18808,#18809);
#15411=AXIS2_PLACEMENT_3D('',#47917,#18810,#18811);
#15412=AXIS2_PLACEMENT_3D('',#48355,#18814,#18815);
#15413=AXIS2_PLACEMENT_3D('',#48357,#18817,#18818);
#15414=AXIS2_PLACEMENT_3D('',#48359,#18819,#18820);
#15415=AXIS2_PLACEMENT_3D('',#48797,#18823,#18824);
#15416=AXIS2_PLACEMENT_3D('',#48799,#18826,#18827);
#15417=AXIS2_PLACEMENT_3D('',#48801,#18828,#18829);
#15418=AXIS2_PLACEMENT_3D('',#49239,#18832,#18833);
#15419=AXIS2_PLACEMENT_3D('',#49241,#18835,#18836);
#15420=AXIS2_PLACEMENT_3D('',#49243,#18837,#18838);
#15421=AXIS2_PLACEMENT_3D('',#49681,#18841,#18842);
#15422=AXIS2_PLACEMENT_3D('',#49683,#18844,#18845);
#15423=AXIS2_PLACEMENT_3D('',#49685,#18846,#18847);
#15424=AXIS2_PLACEMENT_3D('',#50123,#18850,#18851);
#15425=AXIS2_PLACEMENT_3D('',#50125,#18853,#18854);
#15426=AXIS2_PLACEMENT_3D('',#50127,#18855,#18856);
#15427=AXIS2_PLACEMENT_3D('',#50565,#18859,#18860);
#15428=AXIS2_PLACEMENT_3D('',#50567,#18862,#18863);
#15429=AXIS2_PLACEMENT_3D('',#50569,#18864,#18865);
#15430=AXIS2_PLACEMENT_3D('',#51007,#18868,#18869);
#15431=AXIS2_PLACEMENT_3D('',#51009,#18871,#18872);
#15432=AXIS2_PLACEMENT_3D('',#51011,#18873,#18874);
#15433=AXIS2_PLACEMENT_3D('',#51449,#18877,#18878);
#15434=AXIS2_PLACEMENT_3D('',#51451,#18880,#18881);
#15435=AXIS2_PLACEMENT_3D('',#51453,#18882,#18883);
#15436=AXIS2_PLACEMENT_3D('',#51891,#18886,#18887);
#15437=AXIS2_PLACEMENT_3D('',#51893,#18889,#18890);
#15438=AXIS2_PLACEMENT_3D('',#51895,#18891,#18892);
#15439=AXIS2_PLACEMENT_3D('',#52333,#18895,#18896);
#15440=AXIS2_PLACEMENT_3D('',#52335,#18898,#18899);
#15441=AXIS2_PLACEMENT_3D('',#52337,#18900,#18901);
#15442=AXIS2_PLACEMENT_3D('',#52775,#18904,#18905);
#15443=AXIS2_PLACEMENT_3D('',#52777,#18907,#18908);
#15444=AXIS2_PLACEMENT_3D('',#52779,#18909,#18910);
#15445=AXIS2_PLACEMENT_3D('',#53217,#18913,#18914);
#15446=AXIS2_PLACEMENT_3D('',#53219,#18916,#18917);
#15447=AXIS2_PLACEMENT_3D('',#53221,#18918,#18919);
#15448=AXIS2_PLACEMENT_3D('',#53659,#18922,#18923);
#15449=AXIS2_PLACEMENT_3D('',#53661,#18925,#18926);
#15450=AXIS2_PLACEMENT_3D('',#53663,#18927,#18928);
#15451=AXIS2_PLACEMENT_3D('',#54101,#18931,#18932);
#15452=AXIS2_PLACEMENT_3D('',#54103,#18934,#18935);
#15453=AXIS2_PLACEMENT_3D('',#54105,#18936,#18937);
#15454=AXIS2_PLACEMENT_3D('',#54543,#18940,#18941);
#15455=AXIS2_PLACEMENT_3D('',#54545,#18943,#18944);
#15456=AXIS2_PLACEMENT_3D('',#54547,#18945,#18946);
#15457=AXIS2_PLACEMENT_3D('',#54985,#18949,#18950);
#15458=AXIS2_PLACEMENT_3D('',#54987,#18952,#18953);
#15459=AXIS2_PLACEMENT_3D('',#54989,#18954,#18955);
#15460=AXIS2_PLACEMENT_3D('',#55427,#18958,#18959);
#15461=AXIS2_PLACEMENT_3D('',#55429,#18961,#18962);
#15462=AXIS2_PLACEMENT_3D('',#55431,#18963,#18964);
#15463=AXIS2_PLACEMENT_3D('',#55869,#18967,#18968);
#15464=AXIS2_PLACEMENT_3D('',#55871,#18970,#18971);
#15465=AXIS2_PLACEMENT_3D('',#55873,#18972,#18973);
#15466=AXIS2_PLACEMENT_3D('',#56311,#18976,#18977);
#15467=AXIS2_PLACEMENT_3D('',#56313,#18979,#18980);
#15468=AXIS2_PLACEMENT_3D('',#56315,#18981,#18982);
#15469=AXIS2_PLACEMENT_3D('',#56753,#18985,#18986);
#15470=AXIS2_PLACEMENT_3D('',#56755,#18988,#18989);
#15471=AXIS2_PLACEMENT_3D('',#56757,#18990,#18991);
#15472=AXIS2_PLACEMENT_3D('',#56976,#18993,#18994);
#15473=AXIS2_PLACEMENT_3D('',#57197,#18997,#18998);
#15474=AXIS2_PLACEMENT_3D('',#57199,#18999,#19000);
#15475=AXIS2_PLACEMENT_3D('',#57637,#19003,#19004);
#15476=AXIS2_PLACEMENT_3D('',#57639,#19006,#19007);
#15477=AXIS2_PLACEMENT_3D('',#57640,#19008,#19009);
#15478=AXIS2_PLACEMENT_3D('',#57641,#19010,#19011);
#18495=DIRECTION('axis',(0.,0.,1.));
#18496=DIRECTION('refdir',(1.,0.,0.));
#18497=DIRECTION('center_axis',(0.996917333733128,0.,-0.0784590957278449));
#18498=DIRECTION('ref_axis',(-0.0784590957278449,0.,-0.996917333733128));
#18499=DIRECTION('',(0.0784590957278449,0.,0.996917333733128));
#18500=DIRECTION('',(0.,1.,0.));
#18501=DIRECTION('',(-0.0784590957278449,0.,-0.996917333733128));
#18502=DIRECTION('',(0.,-1.,0.));
#18503=DIRECTION('center_axis',(-0.0784590957278449,0.,-0.996917333733128));
#18504=DIRECTION('ref_axis',(-0.996917333733128,0.,0.0784590957278449));
#18505=DIRECTION('',(0.996917333733128,0.,-0.0784590957278449));
#18506=DIRECTION('',(0.,-1.,0.));
#18507=DIRECTION('',(-0.996917333733128,0.,0.0784590957278449));
#18508=DIRECTION('center_axis',(-0.996917333733128,0.,0.0784590957278449));
#18509=DIRECTION('ref_axis',(0.0784590957278449,0.,0.996917333733128));
#18510=DIRECTION('',(-0.0784590957278449,0.,-0.996917333733128));
#18511=DIRECTION('',(0.,1.,0.));
#18512=DIRECTION('',(0.0784590957278449,0.,0.996917333733128));
#18513=DIRECTION('center_axis',(0.,1.,0.));
#18514=DIRECTION('ref_axis',(0.996917333733128,0.,-0.0784590957278449));
#18515=DIRECTION('center_axis',(0.,-1.,0.));
#18516=DIRECTION('ref_axis',(0.996917333733128,0.,-0.0784590957278449));
#18517=DIRECTION('',(-0.233445363855906,0.,0.972369920397677));
#18518=DIRECTION('center_axis',(0.,-1.,0.));
#18519=DIRECTION('ref_axis',(0.996917333733128,0.,-0.0784590957278449));
#18520=DIRECTION('',(-0.38268343236509,0.,0.923879532511287));
#18521=DIRECTION('center_axis',(0.,-1.,0.));
#18522=DIRECTION('ref_axis',(0.996917333733128,0.,-0.0784590957278449));
#18523=DIRECTION('',(-0.522498564715949,0.,0.852640164354092));
#18524=DIRECTION('center_axis',(0.,-1.,0.));
#18525=DIRECTION('ref_axis',(0.996917333733128,0.,-0.0784590957278449));
#18526=DIRECTION('',(-0.649448048330184,0.,0.760405965600031));
#18527=DIRECTION('center_axis',(0.,-1.,0.));
#18528=DIRECTION('ref_axis',(0.996917333733128,0.,-0.0784590957278449));
#18529=DIRECTION('',(-0.760405965600031,0.,0.649448048330184));
#18530=DIRECTION('center_axis',(0.,-1.,0.));
#18531=DIRECTION('ref_axis',(0.996917333733128,0.,-0.0784590957278449));
#18532=DIRECTION('',(-0.852640164354092,0.,0.522498564715949));
#18533=DIRECTION('center_axis',(0.,-1.,0.));
#18534=DIRECTION('ref_axis',(0.996917333733128,0.,-0.0784590957278449));
#18535=DIRECTION('',(-0.923879532511287,0.,0.38268343236509));
#18536=DIRECTION('center_axis',(0.,-1.,0.));
#18537=DIRECTION('ref_axis',(0.996917333733128,0.,-0.0784590957278449));
#18538=DIRECTION('',(-0.972369920397677,0.,0.233445363855905));
#18539=DIRECTION('center_axis',(0.,-1.,0.));
#18540=DIRECTION('ref_axis',(0.996917333733128,0.,-0.0784590957278449));
#18541=DIRECTION('',(-0.996917333733128,0.,0.0784590957278448));
#18542=DIRECTION('center_axis',(0.,-1.,0.));
#18543=DIRECTION('ref_axis',(0.996917333733128,0.,-0.0784590957278449));
#18544=DIRECTION('',(-0.996917333733128,0.,-0.0784590957278451));
#18545=DIRECTION('center_axis',(0.,-1.,0.));
#18546=DIRECTION('ref_axis',(0.996917333733128,0.,-0.0784590957278449));
#18547=DIRECTION('',(-0.972369920397677,0.,-0.233445363855906));
#18548=DIRECTION('center_axis',(0.,-1.,0.));
#18549=DIRECTION('ref_axis',(0.996917333733128,0.,-0.0784590957278449));
#18550=DIRECTION('',(-0.923879532511287,0.,-0.38268343236509));
#18551=DIRECTION('center_axis',(0.,-1.,0.));
#18552=DIRECTION('ref_axis',(0.996917333733128,0.,-0.0784590957278449));
#18553=DIRECTION('',(-0.852640164354092,0.,-0.522498564715949));
#18554=DIRECTION('center_axis',(0.,-1.,0.));
#18555=DIRECTION('ref_axis',(0.996917333733128,0.,-0.0784590957278449));
#18556=DIRECTION('',(-0.760405965600031,0.,-0.649448048330184));
#18557=DIRECTION('center_axis',(0.,-1.,0.));
#18558=DIRECTION('ref_axis',(0.996917333733128,0.,-0.0784590957278449));
#18559=DIRECTION('',(-0.649448048330184,0.,-0.760405965600031));
#18560=DIRECTION('center_axis',(0.,-1.,0.));
#18561=DIRECTION('ref_axis',(0.996917333733128,0.,-0.0784590957278449));
#18562=DIRECTION('',(-0.522498564715949,0.,-0.852640164354092));
#18563=DIRECTION('center_axis',(0.,-1.,0.));
#18564=DIRECTION('ref_axis',(0.996917333733128,0.,-0.0784590957278449));
#18565=DIRECTION('',(-0.38268343236509,0.,-0.923879532511287));
#18566=DIRECTION('center_axis',(0.,-1.,0.));
#18567=DIRECTION('ref_axis',(0.996917333733128,0.,-0.0784590957278449));
#18568=DIRECTION('',(-0.233445363855905,0.,-0.972369920397677));
#18569=DIRECTION('center_axis',(0.,-1.,0.));
#18570=DIRECTION('ref_axis',(0.996917333733128,0.,-0.0784590957278449));
#18571=DIRECTION('',(-0.0784590957278448,0.,-0.996917333733128));
#18572=DIRECTION('center_axis',(0.,-1.,0.));
#18573=DIRECTION('ref_axis',(0.996917333733128,0.,-0.0784590957278449));
#18574=DIRECTION('',(0.0784590957278451,0.,-0.996917333733128));
#18575=DIRECTION('center_axis',(0.,-1.,0.));
#18576=DIRECTION('ref_axis',(0.996917333733128,0.,-0.0784590957278449));
#18577=DIRECTION('',(0.233445363855906,0.,-0.972369920397677));
#18578=DIRECTION('center_axis',(0.,-1.,0.));
#18579=DIRECTION('ref_axis',(0.996917333733128,0.,-0.0784590957278449));
#18580=DIRECTION('',(0.38268343236509,0.,-0.923879532511287));
#18581=DIRECTION('center_axis',(0.,-1.,0.));
#18582=DIRECTION('ref_axis',(0.996917333733128,0.,-0.0784590957278449));
#18583=DIRECTION('',(0.522498564715949,0.,-0.852640164354092));
#18584=DIRECTION('center_axis',(0.,-1.,0.));
#18585=DIRECTION('ref_axis',(0.996917333733128,0.,-0.0784590957278449));
#18586=DIRECTION('',(0.649448048330184,0.,-0.760405965600031));
#18587=DIRECTION('center_axis',(0.,-1.,0.));
#18588=DIRECTION('ref_axis',(0.996917333733128,0.,-0.0784590957278449));
#18589=DIRECTION('',(0.760405965600031,0.,-0.649448048330184));
#18590=DIRECTION('center_axis',(0.,-1.,0.));
#18591=DIRECTION('ref_axis',(0.996917333733128,0.,-0.0784590957278449));
#18592=DIRECTION('',(0.852640164354092,0.,-0.522498564715949));
#18593=DIRECTION('center_axis',(0.,-1.,0.));
#18594=DIRECTION('ref_axis',(0.996917333733128,0.,-0.0784590957278449));
#18595=DIRECTION('',(0.923879532511287,0.,-0.38268343236509));
#18596=DIRECTION('center_axis',(0.,-1.,0.));
#18597=DIRECTION('ref_axis',(0.996917333733128,0.,-0.0784590957278449));
#18598=DIRECTION('',(0.972369920397677,0.,-0.233445363855905));
#18599=DIRECTION('center_axis',(0.,-1.,0.));
#18600=DIRECTION('ref_axis',(0.996917333733128,0.,-0.0784590957278449));
#18601=DIRECTION('',(0.996917333733128,0.,-0.0784590957278449));
#18602=DIRECTION('center_axis',(0.,-1.,0.));
#18603=DIRECTION('ref_axis',(0.996917333733128,0.,-0.0784590957278449));
#18604=DIRECTION('',(0.996917333733128,0.,0.078459095727845));
#18605=DIRECTION('center_axis',(0.,-1.,0.));
#18606=DIRECTION('ref_axis',(0.996917333733128,0.,-0.0784590957278449));
#18607=DIRECTION('',(0.972369920397677,0.,0.233445363855906));
#18608=DIRECTION('center_axis',(0.,-1.,0.));
#18609=DIRECTION('ref_axis',(0.996917333733128,0.,-0.0784590957278449));
#18610=DIRECTION('',(0.923879532511287,0.,0.38268343236509));
#18611=DIRECTION('center_axis',(0.,-1.,0.));
#18612=DIRECTION('ref_axis',(0.996917333733128,0.,-0.0784590957278449));
#18613=DIRECTION('',(0.852640164354092,0.,0.522498564715949));
#18614=DIRECTION('center_axis',(0.,-1.,0.));
#18615=DIRECTION('ref_axis',(0.996917333733128,0.,-0.0784590957278449));
#18616=DIRECTION('',(0.760405965600031,0.,0.649448048330184));
#18617=DIRECTION('center_axis',(0.,-1.,0.));
#18618=DIRECTION('ref_axis',(0.996917333733128,0.,-0.0784590957278449));
#18619=DIRECTION('',(0.649448048330184,0.,0.760405965600031));
#18620=DIRECTION('center_axis',(0.,-1.,0.));
#18621=DIRECTION('ref_axis',(0.996917333733128,0.,-0.0784590957278449));
#18622=DIRECTION('',(0.522498564715949,0.,0.852640164354092));
#18623=DIRECTION('center_axis',(0.,-1.,0.));
#18624=DIRECTION('ref_axis',(0.996917333733128,0.,-0.0784590957278449));
#18625=DIRECTION('',(0.38268343236509,0.,0.923879532511287));
#18626=DIRECTION('center_axis',(0.,-1.,0.));
#18627=DIRECTION('ref_axis',(0.996917333733128,0.,-0.0784590957278449));
#18628=DIRECTION('',(0.233445363855905,0.,0.972369920397677));
#18629=DIRECTION('center_axis',(0.,-1.,0.));
#18630=DIRECTION('ref_axis',(0.996917333733128,0.,-0.0784590957278449));
#18631=DIRECTION('',(0.0784590957278449,0.,0.996917333733128));
#18632=DIRECTION('center_axis',(0.,-1.,0.));
#18633=DIRECTION('ref_axis',(0.996917333733128,0.,-0.0784590957278449));
#18634=DIRECTION('',(-0.0784590957278452,0.,0.996917333733128));
#18635=DIRECTION('center_axis',(0.,1.,0.));
#18636=DIRECTION('ref_axis',(0.996917333733128,0.,-0.0784590957278449));
#18637=DIRECTION('center_axis',(0.,1.,0.));
#18638=DIRECTION('ref_axis',(0.078459095727845,0.,0.996917333733128));
#18639=DIRECTION('center_axis',(0.,-1.,0.));
#18640=DIRECTION('ref_axis',(0.996917333733128,0.,-0.0784590957278449));
#18641=DIRECTION('center_axis',(0.,1.,0.));
#18642=DIRECTION('ref_axis',(0.996917333733128,0.,-0.0784590957278449));
#18643=DIRECTION('center_axis',(0.,1.,0.));
#18644=DIRECTION('ref_axis',(0.996917333733128,0.,-0.0784590957278449));
#18645=DIRECTION('',(0.,-1.,0.));
#18646=DIRECTION('center_axis',(0.,-1.,0.));
#18647=DIRECTION('ref_axis',(0.996917333733128,0.,-0.0784590957278449));
#18648=DIRECTION('center_axis',(0.,1.,0.));
#18649=DIRECTION('ref_axis',(0.996917333733128,0.,-0.0784590957278449));
#18650=DIRECTION('',(0.,1.,0.));
#18651=DIRECTION('',(0.,1.,0.));
#18652=DIRECTION('center_axis',(0.996917333733128,0.,0.0784590957278452));
#18653=DIRECTION('ref_axis',(0.0784590957278452,0.,-0.996917333733128));
#18654=DIRECTION('',(0.0784590957278452,0.,-0.996917333733128));
#18655=DIRECTION('center_axis',(0.,1.,0.));
#18656=DIRECTION('ref_axis',(0.996917333733128,0.,-0.0784590957278449));
#18657=DIRECTION('center_axis',(0.,1.,0.));
#18658=DIRECTION('ref_axis',(0.996917333733128,0.,-0.0784590957278449));
#18659=DIRECTION('',(0.,1.,0.));
#18660=DIRECTION('',(0.,1.,0.));
#18661=DIRECTION('center_axis',(0.972369920397677,0.,0.233445363855906));
#18662=DIRECTION('ref_axis',(0.233445363855906,0.,-0.972369920397677));
#18663=DIRECTION('',(0.233445363855906,0.,-0.972369920397677));
#18664=DIRECTION('center_axis',(0.,1.,0.));
#18665=DIRECTION('ref_axis',(0.996917333733128,0.,-0.0784590957278449));
#18666=DIRECTION('center_axis',(0.,1.,0.));
#18667=DIRECTION('ref_axis',(0.996917333733128,0.,-0.0784590957278449));
#18668=DIRECTION('',(0.,1.,0.));
#18669=DIRECTION('',(0.,1.,0.));
#18670=DIRECTION('center_axis',(0.923879532511287,0.,0.38268343236509));
#18671=DIRECTION('ref_axis',(0.38268343236509,0.,-0.923879532511287));
#18672=DIRECTION('',(0.38268343236509,0.,-0.923879532511287));
#18673=DIRECTION('center_axis',(0.,1.,0.));
#18674=DIRECTION('ref_axis',(0.996917333733128,0.,-0.0784590957278449));
#18675=DIRECTION('center_axis',(0.,1.,0.));
#18676=DIRECTION('ref_axis',(0.996917333733128,0.,-0.0784590957278449));
#18677=DIRECTION('',(0.,1.,0.));
#18678=DIRECTION('',(0.,1.,0.));
#18679=DIRECTION('center_axis',(0.852640164354092,0.,0.522498564715949));
#18680=DIRECTION('ref_axis',(0.522498564715949,0.,-0.852640164354092));
#18681=DIRECTION('',(0.522498564715949,0.,-0.852640164354092));
#18682=DIRECTION('center_axis',(0.,1.,0.));
#18683=DIRECTION('ref_axis',(0.996917333733128,0.,-0.0784590957278449));
#18684=DIRECTION('center_axis',(0.,1.,0.));
#18685=DIRECTION('ref_axis',(0.996917333733128,0.,-0.0784590957278449));
#18686=DIRECTION('',(0.,1.,0.));
#18687=DIRECTION('',(0.,1.,0.));
#18688=DIRECTION('center_axis',(0.760405965600031,0.,0.649448048330184));
#18689=DIRECTION('ref_axis',(0.649448048330184,0.,-0.760405965600031));
#18690=DIRECTION('',(0.649448048330184,0.,-0.760405965600031));
#18691=DIRECTION('center_axis',(0.,1.,0.));
#18692=DIRECTION('ref_axis',(0.996917333733128,0.,-0.0784590957278449));
#18693=DIRECTION('center_axis',(0.,1.,0.));
#18694=DIRECTION('ref_axis',(0.996917333733128,0.,-0.0784590957278449));
#18695=DIRECTION('',(0.,1.,0.));
#18696=DIRECTION('',(0.,1.,0.));
#18697=DIRECTION('center_axis',(0.649448048330184,0.,0.760405965600031));
#18698=DIRECTION('ref_axis',(0.760405965600031,0.,-0.649448048330184));
#18699=DIRECTION('',(0.760405965600031,0.,-0.649448048330184));
#18700=DIRECTION('center_axis',(0.,1.,0.));
#18701=DIRECTION('ref_axis',(0.996917333733128,0.,-0.0784590957278449));
#18702=DIRECTION('center_axis',(0.,1.,0.));
#18703=DIRECTION('ref_axis',(0.996917333733128,0.,-0.0784590957278449));
#18704=DIRECTION('',(0.,1.,0.));
#18705=DIRECTION('',(0.,1.,0.));
#18706=DIRECTION('center_axis',(0.522498564715949,0.,0.852640164354092));
#18707=DIRECTION('ref_axis',(0.852640164354092,0.,-0.522498564715949));
#18708=DIRECTION('',(0.852640164354092,0.,-0.522498564715949));
#18709=DIRECTION('center_axis',(0.,1.,0.));
#18710=DIRECTION('ref_axis',(0.996917333733128,0.,-0.0784590957278449));
#18711=DIRECTION('center_axis',(0.,1.,0.));
#18712=DIRECTION('ref_axis',(0.996917333733128,0.,-0.0784590957278449));
#18713=DIRECTION('',(0.,1.,0.));
#18714=DIRECTION('',(0.,1.,0.));
#18715=DIRECTION('center_axis',(0.38268343236509,0.,0.923879532511287));
#18716=DIRECTION('ref_axis',(0.923879532511287,0.,-0.38268343236509));
#18717=DIRECTION('',(0.923879532511287,0.,-0.38268343236509));
#18718=DIRECTION('center_axis',(0.,1.,0.));
#18719=DIRECTION('ref_axis',(0.996917333733128,0.,-0.0784590957278449));
#18720=DIRECTION('center_axis',(0.,1.,0.));
#18721=DIRECTION('ref_axis',(0.996917333733128,0.,-0.0784590957278449));
#18722=DIRECTION('',(0.,1.,0.));
#18723=DIRECTION('',(0.,1.,0.));
#18724=DIRECTION('center_axis',(0.233445363855905,0.,0.972369920397677));
#18725=DIRECTION('ref_axis',(0.972369920397677,0.,-0.233445363855905));
#18726=DIRECTION('',(0.972369920397677,0.,-0.233445363855905));
#18727=DIRECTION('center_axis',(0.,1.,0.));
#18728=DIRECTION('ref_axis',(0.996917333733128,0.,-0.0784590957278449));
#18729=DIRECTION('center_axis',(0.,1.,0.));
#18730=DIRECTION('ref_axis',(0.996917333733128,0.,-0.0784590957278449));
#18731=DIRECTION('',(0.,1.,0.));
#18732=DIRECTION('',(0.,1.,0.));
#18733=DIRECTION('center_axis',(0.0784590957278448,0.,0.996917333733128));
#18734=DIRECTION('ref_axis',(0.996917333733128,0.,-0.0784590957278448));
#18735=DIRECTION('',(0.996917333733128,0.,-0.0784590957278448));
#18736=DIRECTION('center_axis',(0.,1.,0.));
#18737=DIRECTION('ref_axis',(0.996917333733128,0.,-0.0784590957278449));
#18738=DIRECTION('center_axis',(0.,1.,0.));
#18739=DIRECTION('ref_axis',(0.996917333733128,0.,-0.0784590957278449));
#18740=DIRECTION('',(0.,1.,0.));
#18741=DIRECTION('',(0.,1.,0.));
#18742=DIRECTION('center_axis',(-0.0784590957278451,0.,0.996917333733128));
#18743=DIRECTION('ref_axis',(0.996917333733128,0.,0.0784590957278451));
#18744=DIRECTION('',(0.996917333733128,0.,0.0784590957278451));
#18745=DIRECTION('center_axis',(0.,1.,0.));
#18746=DIRECTION('ref_axis',(0.996917333733128,0.,-0.0784590957278449));
#18747=DIRECTION('center_axis',(0.,1.,0.));
#18748=DIRECTION('ref_axis',(0.996917333733128,0.,-0.0784590957278449));
#18749=DIRECTION('',(0.,1.,0.));
#18750=DIRECTION('',(0.,1.,0.));
#18751=DIRECTION('center_axis',(-0.233445363855906,0.,0.972369920397677));
#18752=DIRECTION('ref_axis',(0.972369920397677,0.,0.233445363855906));
#18753=DIRECTION('',(0.972369920397677,0.,0.233445363855906));
#18754=DIRECTION('center_axis',(0.,1.,0.));
#18755=DIRECTION('ref_axis',(0.996917333733128,0.,-0.0784590957278449));
#18756=DIRECTION('center_axis',(0.,1.,0.));
#18757=DIRECTION('ref_axis',(0.996917333733128,0.,-0.0784590957278449));
#18758=DIRECTION('',(0.,1.,0.));
#18759=DIRECTION('',(0.,1.,0.));
#18760=DIRECTION('center_axis',(-0.38268343236509,0.,0.923879532511287));
#18761=DIRECTION('ref_axis',(0.923879532511287,0.,0.38268343236509));
#18762=DIRECTION('',(0.923879532511287,0.,0.38268343236509));
#18763=DIRECTION('center_axis',(0.,1.,0.));
#18764=DIRECTION('ref_axis',(0.996917333733128,0.,-0.0784590957278449));
#18765=DIRECTION('center_axis',(0.,1.,0.));
#18766=DIRECTION('ref_axis',(0.996917333733128,0.,-0.0784590957278449));
#18767=DIRECTION('',(0.,1.,0.));
#18768=DIRECTION('',(0.,1.,0.));
#18769=DIRECTION('center_axis',(-0.522498564715949,0.,0.852640164354092));
#18770=DIRECTION('ref_axis',(0.852640164354092,0.,0.522498564715949));
#18771=DIRECTION('',(0.852640164354092,0.,0.522498564715949));
#18772=DIRECTION('center_axis',(0.,1.,0.));
#18773=DIRECTION('ref_axis',(0.996917333733128,0.,-0.0784590957278449));
#18774=DIRECTION('center_axis',(0.,1.,0.));
#18775=DIRECTION('ref_axis',(0.996917333733128,0.,-0.0784590957278449));
#18776=DIRECTION('',(0.,1.,0.));
#18777=DIRECTION('',(0.,1.,0.));
#18778=DIRECTION('center_axis',(-0.649448048330184,0.,0.760405965600031));
#18779=DIRECTION('ref_axis',(0.760405965600031,0.,0.649448048330184));
#18780=DIRECTION('',(0.760405965600031,0.,0.649448048330184));
#18781=DIRECTION('center_axis',(0.,1.,0.));
#18782=DIRECTION('ref_axis',(0.996917333733128,0.,-0.0784590957278449));
#18783=DIRECTION('center_axis',(0.,1.,0.));
#18784=DIRECTION('ref_axis',(0.996917333733128,0.,-0.0784590957278449));
#18785=DIRECTION('',(0.,1.,0.));
#18786=DIRECTION('',(0.,1.,0.));
#18787=DIRECTION('center_axis',(-0.760405965600031,0.,0.649448048330184));
#18788=DIRECTION('ref_axis',(0.649448048330184,0.,0.760405965600031));
#18789=DIRECTION('',(0.649448048330184,0.,0.760405965600031));
#18790=DIRECTION('center_axis',(0.,1.,0.));
#18791=DIRECTION('ref_axis',(0.996917333733128,0.,-0.0784590957278449));
#18792=DIRECTION('center_axis',(0.,1.,0.));
#18793=DIRECTION('ref_axis',(0.996917333733128,0.,-0.0784590957278449));
#18794=DIRECTION('',(0.,1.,0.));
#18795=DIRECTION('',(0.,1.,0.));
#18796=DIRECTION('center_axis',(-0.852640164354092,0.,0.522498564715949));
#18797=DIRECTION('ref_axis',(0.522498564715949,0.,0.852640164354092));
#18798=DIRECTION('',(0.522498564715949,0.,0.852640164354092));
#18799=DIRECTION('center_axis',(0.,1.,0.));
#18800=DIRECTION('ref_axis',(0.996917333733128,0.,-0.0784590957278449));
#18801=DIRECTION('center_axis',(0.,1.,0.));
#18802=DIRECTION('ref_axis',(0.996917333733128,0.,-0.0784590957278449));
#18803=DIRECTION('',(0.,1.,0.));
#18804=DIRECTION('',(0.,1.,0.));
#18805=DIRECTION('center_axis',(-0.923879532511287,0.,0.38268343236509));
#18806=DIRECTION('ref_axis',(0.38268343236509,0.,0.923879532511287));
#18807=DIRECTION('',(0.38268343236509,0.,0.923879532511287));
#18808=DIRECTION('center_axis',(0.,1.,0.));
#18809=DIRECTION('ref_axis',(0.996917333733128,0.,-0.0784590957278449));
#18810=DIRECTION('center_axis',(0.,1.,0.));
#18811=DIRECTION('ref_axis',(0.996917333733128,0.,-0.0784590957278449));
#18812=DIRECTION('',(0.,1.,0.));
#18813=DIRECTION('',(0.,1.,0.));
#18814=DIRECTION('center_axis',(-0.972369920397677,0.,0.233445363855905));
#18815=DIRECTION('ref_axis',(0.233445363855905,0.,0.972369920397677));
#18816=DIRECTION('',(0.233445363855905,0.,0.972369920397677));
#18817=DIRECTION('center_axis',(0.,1.,0.));
#18818=DIRECTION('ref_axis',(0.996917333733128,0.,-0.0784590957278449));
#18819=DIRECTION('center_axis',(0.,1.,0.));
#18820=DIRECTION('ref_axis',(0.996917333733128,0.,-0.0784590957278449));
#18821=DIRECTION('',(0.,1.,0.));
#18822=DIRECTION('',(0.,1.,0.));
#18823=DIRECTION('center_axis',(-0.996917333733128,0.,0.0784590957278448));
#18824=DIRECTION('ref_axis',(0.0784590957278448,0.,0.996917333733128));
#18825=DIRECTION('',(0.0784590957278448,0.,0.996917333733128));
#18826=DIRECTION('center_axis',(0.,1.,0.));
#18827=DIRECTION('ref_axis',(0.996917333733128,0.,-0.0784590957278449));
#18828=DIRECTION('center_axis',(0.,1.,0.));
#18829=DIRECTION('ref_axis',(0.996917333733128,0.,-0.0784590957278449));
#18830=DIRECTION('',(0.,1.,0.));
#18831=DIRECTION('',(0.,1.,0.));
#18832=DIRECTION('center_axis',(-0.996917333733128,0.,-0.0784590957278451));
#18833=DIRECTION('ref_axis',(-0.0784590957278451,0.,0.996917333733128));
#18834=DIRECTION('',(-0.0784590957278451,0.,0.996917333733128));
#18835=DIRECTION('center_axis',(0.,1.,0.));
#18836=DIRECTION('ref_axis',(0.996917333733128,0.,-0.0784590957278449));
#18837=DIRECTION('center_axis',(0.,1.,0.));
#18838=DIRECTION('ref_axis',(0.996917333733128,0.,-0.0784590957278449));
#18839=DIRECTION('',(0.,1.,0.));
#18840=DIRECTION('',(0.,1.,0.));
#18841=DIRECTION('center_axis',(-0.972369920397677,0.,-0.233445363855906));
#18842=DIRECTION('ref_axis',(-0.233445363855906,0.,0.972369920397677));
#18843=DIRECTION('',(-0.233445363855906,0.,0.972369920397677));
#18844=DIRECTION('center_axis',(0.,1.,0.));
#18845=DIRECTION('ref_axis',(0.996917333733128,0.,-0.0784590957278449));
#18846=DIRECTION('center_axis',(0.,1.,0.));
#18847=DIRECTION('ref_axis',(0.996917333733128,0.,-0.0784590957278449));
#18848=DIRECTION('',(0.,1.,0.));
#18849=DIRECTION('',(0.,1.,0.));
#18850=DIRECTION('center_axis',(-0.923879532511287,0.,-0.38268343236509));
#18851=DIRECTION('ref_axis',(-0.38268343236509,0.,0.923879532511287));
#18852=DIRECTION('',(-0.38268343236509,0.,0.923879532511287));
#18853=DIRECTION('center_axis',(0.,1.,0.));
#18854=DIRECTION('ref_axis',(0.996917333733128,0.,-0.0784590957278449));
#18855=DIRECTION('center_axis',(0.,1.,0.));
#18856=DIRECTION('ref_axis',(0.996917333733128,0.,-0.0784590957278449));
#18857=DIRECTION('',(0.,1.,0.));
#18858=DIRECTION('',(0.,1.,0.));
#18859=DIRECTION('center_axis',(-0.852640164354092,0.,-0.522498564715949));
#18860=DIRECTION('ref_axis',(-0.522498564715949,0.,0.852640164354092));
#18861=DIRECTION('',(-0.522498564715949,0.,0.852640164354092));
#18862=DIRECTION('center_axis',(0.,1.,0.));
#18863=DIRECTION('ref_axis',(0.996917333733128,0.,-0.0784590957278449));
#18864=DIRECTION('center_axis',(0.,1.,0.));
#18865=DIRECTION('ref_axis',(0.996917333733128,0.,-0.0784590957278449));
#18866=DIRECTION('',(0.,1.,0.));
#18867=DIRECTION('',(0.,1.,0.));
#18868=DIRECTION('center_axis',(-0.760405965600031,0.,-0.649448048330184));
#18869=DIRECTION('ref_axis',(-0.649448048330184,0.,0.760405965600031));
#18870=DIRECTION('',(-0.649448048330184,0.,0.760405965600031));
#18871=DIRECTION('center_axis',(0.,1.,0.));
#18872=DIRECTION('ref_axis',(0.996917333733128,0.,-0.0784590957278449));
#18873=DIRECTION('center_axis',(0.,1.,0.));
#18874=DIRECTION('ref_axis',(0.996917333733128,0.,-0.0784590957278449));
#18875=DIRECTION('',(0.,1.,0.));
#18876=DIRECTION('',(0.,1.,0.));
#18877=DIRECTION('center_axis',(-0.649448048330184,0.,-0.760405965600031));
#18878=DIRECTION('ref_axis',(-0.760405965600031,0.,0.649448048330184));
#18879=DIRECTION('',(-0.760405965600031,0.,0.649448048330184));
#18880=DIRECTION('center_axis',(0.,1.,0.));
#18881=DIRECTION('ref_axis',(0.996917333733128,0.,-0.0784590957278449));
#18882=DIRECTION('center_axis',(0.,1.,0.));
#18883=DIRECTION('ref_axis',(0.996917333733128,0.,-0.0784590957278449));
#18884=DIRECTION('',(0.,1.,0.));
#18885=DIRECTION('',(0.,1.,0.));
#18886=DIRECTION('center_axis',(-0.522498564715949,0.,-0.852640164354092));
#18887=DIRECTION('ref_axis',(-0.852640164354092,0.,0.522498564715949));
#18888=DIRECTION('',(-0.852640164354092,0.,0.522498564715949));
#18889=DIRECTION('center_axis',(0.,1.,0.));
#18890=DIRECTION('ref_axis',(0.996917333733128,0.,-0.0784590957278449));
#18891=DIRECTION('center_axis',(0.,1.,0.));
#18892=DIRECTION('ref_axis',(0.996917333733128,0.,-0.0784590957278449));
#18893=DIRECTION('',(0.,1.,0.));
#18894=DIRECTION('',(0.,1.,0.));
#18895=DIRECTION('center_axis',(-0.38268343236509,0.,-0.923879532511287));
#18896=DIRECTION('ref_axis',(-0.923879532511287,0.,0.38268343236509));
#18897=DIRECTION('',(-0.923879532511287,0.,0.38268343236509));
#18898=DIRECTION('center_axis',(0.,1.,0.));
#18899=DIRECTION('ref_axis',(0.996917333733128,0.,-0.0784590957278449));
#18900=DIRECTION('center_axis',(0.,1.,0.));
#18901=DIRECTION('ref_axis',(0.996917333733128,0.,-0.0784590957278449));
#18902=DIRECTION('',(0.,1.,0.));
#18903=DIRECTION('',(0.,1.,0.));
#18904=DIRECTION('center_axis',(-0.233445363855905,0.,-0.972369920397677));
#18905=DIRECTION('ref_axis',(-0.972369920397677,0.,0.233445363855905));
#18906=DIRECTION('',(-0.972369920397677,0.,0.233445363855905));
#18907=DIRECTION('center_axis',(0.,1.,0.));
#18908=DIRECTION('ref_axis',(0.996917333733128,0.,-0.0784590957278449));
#18909=DIRECTION('center_axis',(0.,1.,0.));
#18910=DIRECTION('ref_axis',(0.996917333733128,0.,-0.0784590957278449));
#18911=DIRECTION('',(0.,1.,0.));
#18912=DIRECTION('',(0.,1.,0.));
#18913=DIRECTION('center_axis',(-0.0784590957278449,0.,-0.996917333733128));
#18914=DIRECTION('ref_axis',(-0.996917333733128,0.,0.0784590957278449));
#18915=DIRECTION('',(-0.996917333733128,0.,0.0784590957278449));
#18916=DIRECTION('center_axis',(0.,1.,0.));
#18917=DIRECTION('ref_axis',(0.996917333733128,0.,-0.0784590957278449));
#18918=DIRECTION('center_axis',(0.,1.,0.));
#18919=DIRECTION('ref_axis',(0.996917333733128,0.,-0.0784590957278449));
#18920=DIRECTION('',(0.,1.,0.));
#18921=DIRECTION('',(0.,1.,0.));
#18922=DIRECTION('center_axis',(0.078459095727845,0.,-0.996917333733128));
#18923=DIRECTION('ref_axis',(-0.996917333733128,0.,-0.078459095727845));
#18924=DIRECTION('',(-0.996917333733128,0.,-0.078459095727845));
#18925=DIRECTION('center_axis',(0.,1.,0.));
#18926=DIRECTION('ref_axis',(0.996917333733128,0.,-0.0784590957278449));
#18927=DIRECTION('center_axis',(0.,1.,0.));
#18928=DIRECTION('ref_axis',(0.996917333733128,0.,-0.0784590957278449));
#18929=DIRECTION('',(0.,1.,0.));
#18930=DIRECTION('',(0.,1.,0.));
#18931=DIRECTION('center_axis',(0.233445363855906,0.,-0.972369920397677));
#18932=DIRECTION('ref_axis',(-0.972369920397677,0.,-0.233445363855906));
#18933=DIRECTION('',(-0.972369920397677,0.,-0.233445363855906));
#18934=DIRECTION('center_axis',(0.,1.,0.));
#18935=DIRECTION('ref_axis',(0.996917333733128,0.,-0.0784590957278449));
#18936=DIRECTION('center_axis',(0.,1.,0.));
#18937=DIRECTION('ref_axis',(0.996917333733128,0.,-0.0784590957278449));
#18938=DIRECTION('',(0.,1.,0.));
#18939=DIRECTION('',(0.,1.,0.));
#18940=DIRECTION('center_axis',(0.38268343236509,0.,-0.923879532511287));
#18941=DIRECTION('ref_axis',(-0.923879532511287,0.,-0.38268343236509));
#18942=DIRECTION('',(-0.923879532511287,0.,-0.38268343236509));
#18943=DIRECTION('center_axis',(0.,1.,0.));
#18944=DIRECTION('ref_axis',(0.996917333733128,0.,-0.0784590957278449));
#18945=DIRECTION('center_axis',(0.,1.,0.));
#18946=DIRECTION('ref_axis',(0.996917333733128,0.,-0.0784590957278449));
#18947=DIRECTION('',(0.,1.,0.));
#18948=DIRECTION('',(0.,1.,0.));
#18949=DIRECTION('center_axis',(0.522498564715949,0.,-0.852640164354092));
#18950=DIRECTION('ref_axis',(-0.852640164354092,0.,-0.522498564715949));
#18951=DIRECTION('',(-0.852640164354092,0.,-0.522498564715949));
#18952=DIRECTION('center_axis',(0.,1.,0.));
#18953=DIRECTION('ref_axis',(0.996917333733128,0.,-0.0784590957278449));
#18954=DIRECTION('center_axis',(0.,1.,0.));
#18955=DIRECTION('ref_axis',(0.996917333733128,0.,-0.0784590957278449));
#18956=DIRECTION('',(0.,1.,0.));
#18957=DIRECTION('',(0.,1.,0.));
#18958=DIRECTION('center_axis',(0.649448048330184,0.,-0.760405965600031));
#18959=DIRECTION('ref_axis',(-0.760405965600031,0.,-0.649448048330184));
#18960=DIRECTION('',(-0.760405965600031,0.,-0.649448048330184));
#18961=DIRECTION('center_axis',(0.,1.,0.));
#18962=DIRECTION('ref_axis',(0.996917333733128,0.,-0.0784590957278449));
#18963=DIRECTION('center_axis',(0.,1.,0.));
#18964=DIRECTION('ref_axis',(0.996917333733128,0.,-0.0784590957278449));
#18965=DIRECTION('',(0.,1.,0.));
#18966=DIRECTION('',(0.,1.,0.));
#18967=DIRECTION('center_axis',(0.760405965600031,0.,-0.649448048330184));
#18968=DIRECTION('ref_axis',(-0.649448048330184,0.,-0.760405965600031));
#18969=DIRECTION('',(-0.649448048330184,0.,-0.760405965600031));
#18970=DIRECTION('center_axis',(0.,1.,0.));
#18971=DIRECTION('ref_axis',(0.996917333733128,0.,-0.0784590957278449));
#18972=DIRECTION('center_axis',(0.,1.,0.));
#18973=DIRECTION('ref_axis',(0.996917333733128,0.,-0.0784590957278449));
#18974=DIRECTION('',(0.,1.,0.));
#18975=DIRECTION('',(0.,1.,0.));
#18976=DIRECTION('center_axis',(0.852640164354092,0.,-0.522498564715949));
#18977=DIRECTION('ref_axis',(-0.522498564715949,0.,-0.852640164354092));
#18978=DIRECTION('',(-0.522498564715949,0.,-0.852640164354092));
#18979=DIRECTION('center_axis',(0.,1.,0.));
#18980=DIRECTION('ref_axis',(0.996917333733128,0.,-0.0784590957278449));
#18981=DIRECTION('center_axis',(0.,1.,0.));
#18982=DIRECTION('ref_axis',(0.996917333733128,0.,-0.0784590957278449));
#18983=DIRECTION('',(0.,1.,0.));
#18984=DIRECTION('',(0.,1.,0.));
#18985=DIRECTION('center_axis',(0.923879532511287,0.,-0.38268343236509));
#18986=DIRECTION('ref_axis',(-0.38268343236509,0.,-0.923879532511287));
#18987=DIRECTION('',(-0.38268343236509,0.,-0.923879532511287));
#18988=DIRECTION('center_axis',(0.,1.,0.));
#18989=DIRECTION('ref_axis',(0.996917333733128,0.,-0.0784590957278449));
#18990=DIRECTION('center_axis',(0.,1.,0.));
#18991=DIRECTION('ref_axis',(0.996917333733128,0.,-0.0784590957278449));
#18992=DIRECTION('',(0.,1.,0.));
#18993=DIRECTION('center_axis',(0.972369920397677,0.,-0.233445363855905));
#18994=DIRECTION('ref_axis',(-0.233445363855905,0.,-0.972369920397677));
#18995=DIRECTION('',(-0.233445363855905,0.,-0.972369920397677));
#18996=DIRECTION('',(0.,1.,0.));
#18997=DIRECTION('center_axis',(0.,1.,0.));
#18998=DIRECTION('ref_axis',(0.996917333733128,0.,-0.0784590957278449));
#18999=DIRECTION('center_axis',(0.,1.,0.));
#19000=DIRECTION('ref_axis',(0.996917333733128,0.,-0.0784590957278449));
#19001=DIRECTION('',(0.,1.,0.));
#19002=DIRECTION('',(0.,1.,0.));
#19003=DIRECTION('center_axis',(0.996917333733128,0.,-0.0784590957278449));
#19004=DIRECTION('ref_axis',(-0.0784590957278449,0.,-0.996917333733128));
#19005=DIRECTION('',(-0.0784590957278449,0.,-0.996917333733128));
#19006=DIRECTION('center_axis',(0.,1.,0.));
#19007=DIRECTION('ref_axis',(0.996917333733128,0.,-0.0784590957278449));
#19008=DIRECTION('center_axis',(0.,1.,0.));
#19009=DIRECTION('ref_axis',(0.996917333733128,0.,-0.0784590957278449));
#19010=DIRECTION('center_axis',(0.,1.,0.));
#19011=DIRECTION('ref_axis',(0.996917333733128,0.,-0.0784590957278449));
#34088=CARTESIAN_POINT('',(0.,0.,0.));
#34089=CARTESIAN_POINT('Origin',(0.299075200119938,0.,-0.0235377287183535));
#34090=CARTESIAN_POINT('',(0.198647557588297,2.2,-1.29959191589676));
#34091=CARTESIAN_POINT('',(0.224229992997422,2.2,-0.974536253938444));
#34092=CARTESIAN_POINT('',(0.299075200119938,2.2,-0.0235377287183535));
#34093=CARTESIAN_POINT('',(0.198647557588297,-1.,-1.29959191589676));
#34094=CARTESIAN_POINT('',(0.198647557588297,0.,-1.29959191589676));
#34095=CARTESIAN_POINT('',(0.224229992997422,-1.,-0.974536253938444));
#34096=CARTESIAN_POINT('',(0.299075200119938,-1.,-0.0235377287183535));
#34097=CARTESIAN_POINT('',(0.224229992997422,0.,-0.974536253938444));
#34098=CARTESIAN_POINT('Origin',(0.198647557588297,0.,-1.29959191589676));
#34099=CARTESIAN_POINT('',(-0.39950284265158,2.2,-1.25251645846005));
#34100=CARTESIAN_POINT('',(0.0491099575283277,2.2,-1.28782305153758));
#34101=CARTESIAN_POINT('',(-0.39950284265158,-1.,-1.25251645846005));
#34102=CARTESIAN_POINT('',(-0.39950284265158,0.,-1.25251645846005));
#34103=CARTESIAN_POINT('',(0.0491099575283277,-1.,-1.28782305153758));
#34104=CARTESIAN_POINT('Origin',(-0.39950284265158,0.,-1.25251645846005));
#34105=CARTESIAN_POINT('',(-0.373920407242454,2.2,-0.927460796501737));
#34106=CARTESIAN_POINT('',(-0.349289021385759,2.2,-0.614489364870848));
#34107=CARTESIAN_POINT('',(-0.373920407242454,-1.,-0.927460796501737));
#34108=CARTESIAN_POINT('',(-0.373920407242454,0.,-0.927460796501737));
#34109=CARTESIAN_POINT('',(-0.349289021385759,-1.,-0.614489364870848));
#34110=CARTESIAN_POINT('Origin',(0.,-1.,0.));
#34111=CARTESIAN_POINT('',(3.71701050416825,-1.,0.496319364827592));
#34112=CARTESIAN_POINT('',(3.68845817949618,-1.,0.676591647973661));
#34113=CARTESIAN_POINT('Origin',(0.,-1.,0.));
#34114=CARTESIAN_POINT('',(4.10104028313088,-1.,0.906349047628867));
#34115=CARTESIAN_POINT('Ctrl Pts',(3.68845817949618,-1.,0.676591647973661));
#34116=CARTESIAN_POINT('Ctrl Pts',(3.68850172300543,-1.,0.67656928609342));
#34117=CARTESIAN_POINT('Ctrl Pts',(3.68869596426099,-1.,0.676535079520366));
#34118=CARTESIAN_POINT('Ctrl Pts',(3.68934997767391,-1.,0.676580391119535));
#34119=CARTESIAN_POINT('Ctrl Pts',(3.6910107117555,-1.,0.676867042599712));
#34120=CARTESIAN_POINT('Ctrl Pts',(3.69443683573443,-1.,0.677621861865197));
#34121=CARTESIAN_POINT('Ctrl Pts',(3.69959004073192,-1.,0.67887882222639));
#34122=CARTESIAN_POINT('Ctrl Pts',(3.70595722032165,-1.,0.680526909711618));
#34123=CARTESIAN_POINT('Ctrl Pts',(3.71319182790334,-1.,0.68249234510969));
#34124=CARTESIAN_POINT('Ctrl Pts',(3.7209063713952,-1.,0.684691698168356));
#34125=CARTESIAN_POINT('Ctrl Pts',(3.72872973554125,-1.,0.687043475232499));
#34126=CARTESIAN_POINT('Ctrl Pts',(3.73636374474993,-1.,0.689479637354652));
#34127=CARTESIAN_POINT('Ctrl Pts',(3.74365508986548,-1.,0.691960080400503));
#34128=CARTESIAN_POINT('Ctrl Pts',(3.7506028824329,-1.,0.694474562581174));
#34129=CARTESIAN_POINT('Ctrl Pts',(3.75729775766913,-1.,0.69703124565953));
#34130=CARTESIAN_POINT('Ctrl Pts',(3.76387780603725,-1.,0.699648552230851));
#34131=CARTESIAN_POINT('Ctrl Pts',(3.77048141872904,-1.,0.702346356621614));
#34132=CARTESIAN_POINT('Ctrl Pts',(3.77719254217197,-1.,0.70513584799995));
#34133=CARTESIAN_POINT('Ctrl Pts',(3.78402183336678,-1.,0.7080158793756));
#34134=CARTESIAN_POINT('Ctrl Pts',(3.79093694007146,-1.,0.710978231689118));
#34135=CARTESIAN_POINT('Ctrl Pts',(3.79788100314994,-1.,0.714010733006678));
#34136=CARTESIAN_POINT('Ctrl Pts',(3.80479445759296,-1.,0.717100993669091));
#34137=CARTESIAN_POINT('Ctrl Pts',(3.81163885127309,-1.,0.720240466589173));
#34138=CARTESIAN_POINT('Ctrl Pts',(3.81840802610795,-1.,0.72342634601935));
#34139=CARTESIAN_POINT('Ctrl Pts',(3.82511495756682,-1.,0.726659281876608));
#34140=CARTESIAN_POINT('Ctrl Pts',(3.8317839240337,-1.,0.729942010490146));
#34141=CARTESIAN_POINT('Ctrl Pts',(3.83844103658016,-1.,0.733277703756091));
#34142=CARTESIAN_POINT('Ctrl Pts',(3.84510432881231,-1.,0.736668240497151));
#34143=CARTESIAN_POINT('Ctrl Pts',(3.85177770351237,-1.,0.740113146827177));
#34144=CARTESIAN_POINT('Ctrl Pts',(3.85845645217611,-1.,0.743610542737042));
#34145=CARTESIAN_POINT('Ctrl Pts',(3.86513062969896,-1.,0.747157716488884));
#34146=CARTESIAN_POINT('Ctrl Pts',(3.87178914078372,-1.,0.750751822383024));
#34147=CARTESIAN_POINT('Ctrl Pts',(3.87842382520058,-1.,0.754390577396847));
#34148=CARTESIAN_POINT('Ctrl Pts',(3.88503262662684,-1.,0.758072800564799));
#34149=CARTESIAN_POINT('Ctrl Pts',(3.89161738162245,-1.,0.761798028793978));
#34150=CARTESIAN_POINT('Ctrl Pts',(3.89818233104381,-1.,0.765566256401307));
#34151=CARTESIAN_POINT('Ctrl Pts',(3.90473237182634,-1.,0.769377629847877));
#34152=CARTESIAN_POINT('Ctrl Pts',(3.91127138115238,-1.,0.773232154506306));
#34153=CARTESIAN_POINT('Ctrl Pts',(3.91780062334464,-1.,0.777129415664915));
#34154=CARTESIAN_POINT('Ctrl Pts',(3.92431956510418,-1.,0.781068718228395));
#34155=CARTESIAN_POINT('Ctrl Pts',(3.93082655631768,-1.,0.785049202786459));
#34156=CARTESIAN_POINT('Ctrl Pts',(3.93731956885671,-1.,0.789069971469324));
#34157=CARTESIAN_POINT('Ctrl Pts',(3.94379688971307,-1.,0.793130205641017));
#34158=CARTESIAN_POINT('Ctrl Pts',(3.95025788827189,-1.,0.797229296085439));
#34159=CARTESIAN_POINT('Ctrl Pts',(3.95670276375176,-1.,0.801366797727206));
#34160=CARTESIAN_POINT('Ctrl Pts',(3.96313222295874,-1.,0.805542372178496));
#34161=CARTESIAN_POINT('Ctrl Pts',(3.96954717513251,-1.,0.809755732818134));
#34162=CARTESIAN_POINT('Ctrl Pts',(3.97594844078763,-1.,0.814006592328738));
#34163=CARTESIAN_POINT('Ctrl Pts',(3.98233640155287,-1.,0.818294599022034));
#34164=CARTESIAN_POINT('Ctrl Pts',(3.98871104646328,-1.,0.82261934602177));
#34165=CARTESIAN_POINT('Ctrl Pts',(3.99507212784289,-1.,0.826980400320474));
#34166=CARTESIAN_POINT('Ctrl Pts',(4.00141928477447,-1.,0.831377325741487));
#34167=CARTESIAN_POINT('Ctrl Pts',(4.00775216907934,-1.,0.835809705809822));
#34168=CARTESIAN_POINT('Ctrl Pts',(4.01407059766338,-1.,0.840277171976381));
#34169=CARTESIAN_POINT('Ctrl Pts',(4.02037456798787,-1.,0.844779403288517));
#34170=CARTESIAN_POINT('Ctrl Pts',(4.02666418343508,-1.,0.849316107475013));
#34171=CARTESIAN_POINT('Ctrl Pts',(4.03293960436945,-1.,0.853887006632179));
#34172=CARTESIAN_POINT('Ctrl Pts',(4.03920099284658,-1.,0.858491822322572));
#34173=CARTESIAN_POINT('Ctrl Pts',(4.04544845048097,-1.,0.863130256642174));
#34174=CARTESIAN_POINT('Ctrl Pts',(4.05168199437128,-1.,0.867801988858176));
#34175=CARTESIAN_POINT('Ctrl Pts',(4.05790159030495,-1.,0.872506694780564));
#34176=CARTESIAN_POINT('Ctrl Pts',(4.06410717232347,-1.,0.877244060484596));
#34177=CARTESIAN_POINT('Ctrl Pts',(4.07029866694292,-1.,0.882013797525917));
#34178=CARTESIAN_POINT('Ctrl Pts',(4.07647601774639,-1.,0.886815658360739));
#34179=CARTESIAN_POINT('Ctrl Pts',(4.08263920306651,-1.,0.891649447920402));
#34180=CARTESIAN_POINT('Ctrl Pts',(4.08878822249095,-1.,0.896515019236369));
#34181=CARTESIAN_POINT('Ctrl Pts',(4.09369611524319,-1.,0.900432820945976));
#34182=CARTESIAN_POINT('Ctrl Pts',(4.09737067247114,-1.,0.903385402444213));
#34183=CARTESIAN_POINT('Ctrl Pts',(4.09981755067956,-1.,0.905360112216302));
#34184=CARTESIAN_POINT('Ctrl Pts',(4.10104028313088,-1.,0.906349047628867));
#34185=CARTESIAN_POINT('',(4.06552750530042,-1.,1.05427041296137));
#34186=CARTESIAN_POINT('',(4.10104028313088,-1.,0.906349047628867));
#34187=CARTESIAN_POINT('',(3.59360648251073,-1.,1.07167739962028));
#34188=CARTESIAN_POINT('Ctrl Pts',(4.06552750530042,-1.,1.05427041296137));
#34189=CARTESIAN_POINT('Ctrl Pts',(4.06398907542249,-1.,1.05459645194823));
#34190=CARTESIAN_POINT('Ctrl Pts',(4.06091239149123,-1.,1.055245071776));
#34191=CARTESIAN_POINT('Ctrl Pts',(4.05629789307025,-1.,1.05620762707996));
#34192=CARTESIAN_POINT('Ctrl Pts',(4.05014628384869,-1.,1.05747027727959));
#34193=CARTESIAN_POINT('Ctrl Pts',(4.04245854427496,-1.,1.05901393666567));
#34194=CARTESIAN_POINT('Ctrl Pts',(4.03477261141553,-1.,1.06052284711857));
#34195=CARTESIAN_POINT('Ctrl Pts',(4.02708855235633,-1.,1.06199687787462));
#34196=CARTESIAN_POINT('Ctrl Pts',(4.01940647495943,-1.,1.06343586496236));
#34197=CARTESIAN_POINT('Ctrl Pts',(4.01172654187398,-1.,1.0648396134311));
#34198=CARTESIAN_POINT('Ctrl Pts',(4.00404894952579,-1.,1.06620789963606));
#34199=CARTESIAN_POINT('Ctrl Pts',(3.99637389920441,-1.,1.06754047381312));
#34200=CARTESIAN_POINT('Ctrl Pts',(3.98870156857412,-1.,1.06883706263942));
#34201=CARTESIAN_POINT('Ctrl Pts',(3.98103208801101,-1.,1.07009737257767));
#34202=CARTESIAN_POINT('Ctrl Pts',(3.9733655022223,-1.,1.07132109206164));
#34203=CARTESIAN_POINT('Ctrl Pts',(3.96570179322338,-1.,1.07250789943007));
#34204=CARTESIAN_POINT('Ctrl Pts',(3.95804094429373,-1.,1.07365747426491));
#34205=CARTESIAN_POINT('Ctrl Pts',(3.95038299600676,-1.,1.07476950921587));
#34206=CARTESIAN_POINT('Ctrl Pts',(3.94272809633331,-1.,1.07584371946443));
#34207=CARTESIAN_POINT('Ctrl Pts',(3.93507657572883,-1.,1.07687985975384));
#34208=CARTESIAN_POINT('Ctrl Pts',(3.9274289334984,-1.,1.07787771707195));
#34209=CARTESIAN_POINT('Ctrl Pts',(3.91978568924178,-1.,1.07883706663554));
#34210=CARTESIAN_POINT('Ctrl Pts',(3.91214726022143,-1.,1.07975763507473));
#34211=CARTESIAN_POINT('Ctrl Pts',(3.90451384092545,-1.,1.08063906483818));
#34212=CARTESIAN_POINT('Ctrl Pts',(3.8968852509835,-1.,1.08148086931358));
#34213=CARTESIAN_POINT('Ctrl Pts',(3.88926088975114,-1.,1.08228241999346));
#34214=CARTESIAN_POINT('Ctrl Pts',(3.88164007721312,-1.,1.08304304871029));
#34215=CARTESIAN_POINT('Ctrl Pts',(3.8740223372254,-1.,1.08376213307504));
#34216=CARTESIAN_POINT('Ctrl Pts',(3.86640769434274,-1.,1.08443918607927));
#34217=CARTESIAN_POINT('Ctrl Pts',(3.85879698702532,-1.,1.08507395120059));
#34218=CARTESIAN_POINT('Ctrl Pts',(3.85119211322755,-1.,1.08566647671844));
#34219=CARTESIAN_POINT('Ctrl Pts',(3.8435952876495,-1.,1.08621688337604));
#34220=CARTESIAN_POINT('Ctrl Pts',(3.83600837071708,-1.,1.08672515456902));
#34221=CARTESIAN_POINT('Ctrl Pts',(3.82843215316984,-1.,1.08719091307558));
#34222=CARTESIAN_POINT('Ctrl Pts',(3.82086569676319,-1.,1.08761321539442));
#34223=CARTESIAN_POINT('Ctrl Pts',(3.81330554446323,-1.,1.08799030610862));
#34224=CARTESIAN_POINT('Ctrl Pts',(3.8057472665766,-1.,1.0883200925538));
#34225=CARTESIAN_POINT('Ctrl Pts',(3.79818708705259,-1.,1.08860064435778));
#34226=CARTESIAN_POINT('Ctrl Pts',(3.79062357974404,-1.,1.08883071512098));
#34227=CARTESIAN_POINT('Ctrl Pts',(3.78305911299504,-1.,1.08901018614636));
#34228=CARTESIAN_POINT('Ctrl Pts',(3.77550199409424,-1.,1.0891407279127));
#34229=CARTESIAN_POINT('Ctrl Pts',(3.76796340094448,-1.,1.08922484204256));
#34230=CARTESIAN_POINT('Ctrl Pts',(3.76045342580208,-1.,1.08926462734282));
#34231=CARTESIAN_POINT('Ctrl Pts',(3.75297711748132,-1.,1.08926054632925));
#34232=CARTESIAN_POINT('Ctrl Pts',(3.74553121371757,-1.,1.08921040494017));
#34233=CARTESIAN_POINT('Ctrl Pts',(3.73809879348239,-1.,1.08910769013298));
#34234=CARTESIAN_POINT('Ctrl Pts',(3.73065515162988,-1.,1.08894337390937));
#34235=CARTESIAN_POINT('Ctrl Pts',(3.72317741369398,-1.,1.08870887220082));
#34236=CARTESIAN_POINT('Ctrl Pts',(3.71565372339075,-1.,1.0883988733478));
#34237=CARTESIAN_POINT('Ctrl Pts',(3.70809084139457,-1.,1.08801367312185));
#34238=CARTESIAN_POINT('Ctrl Pts',(3.70052690909833,-1.,1.08756311291309));
#34239=CARTESIAN_POINT('Ctrl Pts',(3.69302062410157,-1.,1.08706319540271));
#34240=CARTESIAN_POINT('Ctrl Pts',(3.68562817420797,-1.,1.0865288888259));
#34241=CARTESIAN_POINT('Ctrl Pts',(3.67838211685117,-1.,1.0859675575576));
#34242=CARTESIAN_POINT('Ctrl Pts',(3.67127347729666,-1.,1.0853733414449));
#34243=CARTESIAN_POINT('Ctrl Pts',(3.66422237895365,-1.,1.08471809922901));
#34244=CARTESIAN_POINT('Ctrl Pts',(3.65709649161166,-1.,1.08395671077807));
#34245=CARTESIAN_POINT('Ctrl Pts',(3.64976441208358,-1.,1.08304289898623));
#34246=CARTESIAN_POINT('Ctrl Pts',(3.64214167843677,-1.,1.08194278850996));
#34247=CARTESIAN_POINT('Ctrl Pts',(3.63423373196529,-1.,1.08064765719867));
#34248=CARTESIAN_POINT('Ctrl Pts',(3.62619537902361,-1.,1.07919137290742));
#34249=CARTESIAN_POINT('Ctrl Pts',(3.61832318504574,-1.,1.07764868137619));
#34250=CARTESIAN_POINT('Ctrl Pts',(3.61098481349204,-1.,1.07611545402734));
#34251=CARTESIAN_POINT('Ctrl Pts',(3.60456339887778,-1.,1.07469327168578));
#34252=CARTESIAN_POINT('Ctrl Pts',(3.59940121154535,-1.,1.07347372545714));
#34253=CARTESIAN_POINT('Ctrl Pts',(3.59600583194946,-1.,1.07259084660936));
#34254=CARTESIAN_POINT('Ctrl Pts',(3.59439596999862,-1.,1.07209229745229));
#34255=CARTESIAN_POINT('Ctrl Pts',(3.59379266874567,-1.,1.07183575450617));
#34256=CARTESIAN_POINT('Ctrl Pts',(3.5936351279798,-1.,1.07171709254135));
#34257=CARTESIAN_POINT('Ctrl Pts',(3.59360648251073,-1.,1.07167739962028));
#34258=CARTESIAN_POINT('',(3.5372048861597,-1.,1.24526366418038));
#34259=CARTESIAN_POINT('Origin',(0.,-1.,0.));
#34260=CARTESIAN_POINT('',(3.90876544355381,-1.,1.53673442965256));
#34261=CARTESIAN_POINT('Ctrl Pts',(3.5372048861597,-1.,1.24526366418038));
#34262=CARTESIAN_POINT('Ctrl Pts',(3.53725139174486,-1.,1.24524838931757));
#34263=CARTESIAN_POINT('Ctrl Pts',(3.5374485926552,-1.,1.2452449899111));
#34264=CARTESIAN_POINT('Ctrl Pts',(3.53808746578196,-1.,1.24539205388767));
#34265=CARTESIAN_POINT('Ctrl Pts',(3.53968291130022,-1.,1.24593497226008));
#34266=CARTESIAN_POINT('Ctrl Pts',(3.54294877425964,-1.,1.24721646231966));
#34267=CARTESIAN_POINT('Ctrl Pts',(3.54784190283068,-1.,1.24926408628003));
#34268=CARTESIAN_POINT('Ctrl Pts',(3.55387287418985,-1.,1.2518879294064));
#34269=CARTESIAN_POINT('Ctrl Pts',(3.56071094991199,-1.,1.25496090900009));
#34270=CARTESIAN_POINT('Ctrl Pts',(3.56798645995275,-1.,1.25834000485716));
#34271=CARTESIAN_POINT('Ctrl Pts',(3.5753456065171,-1.,1.2618866714281));
#34272=CARTESIAN_POINT('Ctrl Pts',(3.58250452868618,-1.,1.26548706249862));
#34273=CARTESIAN_POINT('Ctrl Pts',(3.58931807846313,-1.,1.26907758484709));
#34274=CARTESIAN_POINT('Ctrl Pts',(3.59578698050006,-1.,1.27264798379307));
#34275=CARTESIAN_POINT('Ctrl Pts',(3.60199947736298,-1.,1.27622049908625));
#34276=CARTESIAN_POINT('Ctrl Pts',(3.60808907746339,-1.,1.27983492861691));
#34277=CARTESIAN_POINT('Ctrl Pts',(3.61418935913823,-1.,1.28353255117765));
#34278=CARTESIAN_POINT('Ctrl Pts',(3.6203814849236,-1.,1.28733755029384));
#34279=CARTESIAN_POINT('Ctrl Pts',(3.62667616004369,-1.,1.29125046021878));
#34280=CARTESIAN_POINT('Ctrl Pts',(3.63304271631046,-1.,1.29525810207762));
#34281=CARTESIAN_POINT('Ctrl Pts',(3.63942689872808,-1.,1.2993395590647));
#34282=CARTESIAN_POINT('Ctrl Pts',(3.64577181380113,-1.,1.30347327603774));
#34283=CARTESIAN_POINT('Ctrl Pts',(3.65204081987068,-1.,1.30764479590039));
#34284=CARTESIAN_POINT('Ctrl Pts',(3.65822827358617,-1.,1.31185038411218));
#34285=CARTESIAN_POINT('Ctrl Pts',(3.66434688899793,-1.,1.31609271239911));
#34286=CARTESIAN_POINT('Ctrl Pts',(3.67042021752656,-1.,1.32037828137766));
#34287=CARTESIAN_POINT('Ctrl Pts',(3.67647355257912,-1.,1.32471430856415));
#34288=CARTESIAN_POINT('Ctrl Pts',(3.68252441182551,-1.,1.3291054707274));
#34289=CARTESIAN_POINT('Ctrl Pts',(3.68857672413033,-1.,1.33355191034523));
#34290=CARTESIAN_POINT('Ctrl Pts',(3.69462613305708,-1.,1.3380510339822));
#34291=CARTESIAN_POINT('Ctrl Pts',(3.70066324015119,-1.,1.34259860752933));
#34292=CARTESIAN_POINT('Ctrl Pts',(3.70667753188248,-1.,1.34719008463534));
#34293=CARTESIAN_POINT('Ctrl Pts',(3.71266130563054,-1.,1.35182193384424));
#34294=CARTESIAN_POINT('Ctrl Pts',(3.71861271513313,-1.,1.35649266705037));
#34295=CARTESIAN_POINT('Ctrl Pts',(3.72453364678279,-1.,1.36120211416354));
#34296=CARTESIAN_POINT('Ctrl Pts',(3.73042829011295,-1.,1.36595093298676));
#34297=CARTESIAN_POINT('Ctrl Pts',(3.7363014588581,-1.,1.37074003422739));
#34298=CARTESIAN_POINT('Ctrl Pts',(3.74215698162555,-1.,1.37557002971687));
#34299=CARTESIAN_POINT('Ctrl Pts',(3.74799617204729,-1.,1.38044070763295));
#34300=CARTESIAN_POINT('Ctrl Pts',(3.75381861212707,-1.,1.38535129801176));
#34301=CARTESIAN_POINT('Ctrl Pts',(3.75962280650855,-1.,1.39030069388918));
#34302=CARTESIAN_POINT('Ctrl Pts',(3.76540689249074,-1.,1.39528769118052));
#34303=CARTESIAN_POINT('Ctrl Pts',(3.77116930621827,-1.,1.40031121335505));
#34304=CARTESIAN_POINT('Ctrl Pts',(3.77690952014259,-1.,1.40537056004722));
#34305=CARTESIAN_POINT('Ctrl Pts',(3.78262780065471,-1.,1.41046532282593));
#34306=CARTESIAN_POINT('Ctrl Pts',(3.78832489879426,-1.,1.4155952780383));
#34307=CARTESIAN_POINT('Ctrl Pts',(3.79400175744408,-1.,1.42076028482836));
#34308=CARTESIAN_POINT('Ctrl Pts',(3.7996592319632,-1.,1.42596018777283));
#34309=CARTESIAN_POINT('Ctrl Pts',(3.80529775429805,-1.,1.4311946992132));
#34310=CARTESIAN_POINT('Ctrl Pts',(3.81091737726815,-1.,1.43646341556724));
#34311=CARTESIAN_POINT('Ctrl Pts',(3.81651792398414,-1.,1.44176587041347));
#34312=CARTESIAN_POINT('Ctrl Pts',(3.82209910620533,-1.,1.44710157648539));
#34313=CARTESIAN_POINT('Ctrl Pts',(3.82766064519074,-1.,1.45247006796836));
#34314=CARTESIAN_POINT('Ctrl Pts',(3.83320241775423,-1.,1.45787095220852));
#34315=CARTESIAN_POINT('Ctrl Pts',(3.83872447159639,-1.,1.46330391180752));
#34316=CARTESIAN_POINT('Ctrl Pts',(3.84422695454796,-1.,1.46876867426504));
#34317=CARTESIAN_POINT('Ctrl Pts',(3.84971006847277,-1.,1.47426499018538));
#34318=CARTESIAN_POINT('Ctrl Pts',(3.85517401698843,-1.,1.4797926099102));
#34319=CARTESIAN_POINT('Ctrl Pts',(3.86061894706087,-1.,1.48535125509919));
#34320=CARTESIAN_POINT('Ctrl Pts',(3.86604492575189,-1.,1.4909406116431));
#34321=CARTESIAN_POINT('Ctrl Pts',(3.87145196998465,-1.,1.49656035399122));
#34322=CARTESIAN_POINT('Ctrl Pts',(3.87684006372134,-1.,1.50221016176556));
#34323=CARTESIAN_POINT('Ctrl Pts',(3.88220917950538,-1.,1.50788973857757));
#34324=CARTESIAN_POINT('Ctrl Pts',(3.88755930033884,-1.,1.51359883110559));
#34325=CARTESIAN_POINT('Ctrl Pts',(3.89289043533657,-1.,1.51933724329306));
#34326=CARTESIAN_POINT('Ctrl Pts',(3.89820260708225,-1.,1.52510482991635));
#34327=CARTESIAN_POINT('Ctrl Pts',(3.90243719631596,-1.,1.52974216056287));
#34328=CARTESIAN_POINT('Ctrl Pts',(3.90560462813969,-1.,1.53323321827755));
#34329=CARTESIAN_POINT('Ctrl Pts',(3.90771246855019,-1.,1.53556639217905));
#34330=CARTESIAN_POINT('Ctrl Pts',(3.90876544355381,-1.,1.53673442965256));
#34331=CARTESIAN_POINT('',(3.85054988729471,-1.,1.67727921511438));
#34332=CARTESIAN_POINT('',(3.90876544355381,-1.,1.53673442965256));
#34333=CARTESIAN_POINT('',(3.38171594275765,-1.,1.62064718014094));
#34334=CARTESIAN_POINT('Ctrl Pts',(3.85054988729471,-1.,1.67727921511438));
#34335=CARTESIAN_POINT('Ctrl Pts',(3.84897939430696,-1.,1.67736057656533));
#34336=CARTESIAN_POINT('Ctrl Pts',(3.84583912296459,-1.,1.6775199114018));
#34337=CARTESIAN_POINT('Ctrl Pts',(3.84113085985244,-1.,1.67774874946079));
#34338=CARTESIAN_POINT('Ctrl Pts',(3.83485746513989,-1.,1.67803353064351));
#34339=CARTESIAN_POINT('Ctrl Pts',(3.82702289286713,-1.,1.6783555575934));
#34340=CARTESIAN_POINT('Ctrl Pts',(3.81919554099578,-1.,1.67864354605954));
#34341=CARTESIAN_POINT('Ctrl Pts',(3.81137549624178,-1.,1.6788973773827));
#34342=CARTESIAN_POINT('Ctrl Pts',(3.80356289079005,-1.,1.67911690648355));
#34343=CARTESIAN_POINT('Ctrl Pts',(3.79575791578424,-1.,1.67930196625548));
#34344=CARTESIAN_POINT('Ctrl Pts',(3.7879608002176,-1.,1.67945236653493));
#34345=CARTESIAN_POINT('Ctrl Pts',(3.78017178197317,-1.,1.67956789212141));
#34346=CARTESIAN_POINT('Ctrl Pts',(3.77239107928502,-1.,1.67964830084993));
#34347=CARTESIAN_POINT('Ctrl Pts',(3.76461886684344,-1.,1.67969332319245));
#34348=CARTESIAN_POINT('Ctrl Pts',(3.75685523754493,-1.,1.67970265841239));
#34349=CARTESIAN_POINT('Ctrl Pts',(3.7491002239452,-1.,1.67967598599525));
#34350=CARTESIAN_POINT('Ctrl Pts',(3.74135385965401,-1.,1.6796129868522));
#34351=CARTESIAN_POINT('Ctrl Pts',(3.73361623282543,-1.,1.67951336376402));
#34352=CARTESIAN_POINT('Ctrl Pts',(3.72588753416396,-1.,1.67937685856652));
#34353=CARTESIAN_POINT('Ctrl Pts',(3.71816812842322,-1.,1.67920328071708));
#34354=CARTESIAN_POINT('Ctrl Pts',(3.71045854208343,-1.,1.67899249793462));
#34355=CARTESIAN_POINT('Ctrl Pts',(3.70275932351108,-1.,1.67874436948667));
#34356=CARTESIAN_POINT('Ctrl Pts',(3.6950709275959,-1.,1.67845869064323));
#34357=CARTESIAN_POINT('Ctrl Pts',(3.68739360236487,-1.,1.67813513867965));
#34358=CARTESIAN_POINT('Ctrl Pts',(3.67972724579124,-1.,1.67777320475848));
#34359=CARTESIAN_POINT('Ctrl Pts',(3.67207136294575,-1.,1.67737217414874));
#34360=CARTESIAN_POINT('Ctrl Pts',(3.66442538670968,-1.,1.67693128053132));
#34361=CARTESIAN_POINT('Ctrl Pts',(3.6567889441642,-1.,1.6764498346945));
#34362=CARTESIAN_POINT('Ctrl Pts',(3.64916213574667,-1.,1.67592735946692));
#34363=CARTESIAN_POINT('Ctrl Pts',(3.6415458297234,-1.,1.67536373264848));
#34364=CARTESIAN_POINT('Ctrl Pts',(3.63394189312924,-1.,1.67475929882971));
#34365=CARTESIAN_POINT('Ctrl Pts',(3.62635249450923,-1.,1.67411452372271));
#34366=CARTESIAN_POINT('Ctrl Pts',(3.61877947398184,-1.,1.67342968196224));
#34367=CARTESIAN_POINT('Ctrl Pts',(3.61122367156181,-1.,1.67270452466968));
#34368=CARTESIAN_POINT('Ctrl Pts',(3.603684308152,-1.,1.67193797318597));
#34369=CARTESIAN_POINT('Ctrl Pts',(3.59615824388807,-1.,1.67112775290707));
#34370=CARTESIAN_POINT('Ctrl Pts',(3.58864143097834,-1.,1.67027110397604));
#34371=CARTESIAN_POINT('Ctrl Pts',(3.58113044183829,-1.,1.66936552908232));
#34372=CARTESIAN_POINT('Ctrl Pts',(3.57362406285887,-1.,1.668409574073));
#34373=CARTESIAN_POINT('Ctrl Pts',(3.56612465179422,-1.,1.66740349220305));
#34374=CARTESIAN_POINT('Ctrl Pts',(3.55864015233602,-1.,1.66635023293114));
#34375=CARTESIAN_POINT('Ctrl Pts',(3.55118121342861,-1.,1.66525401568994));
#34376=CARTESIAN_POINT('Ctrl Pts',(3.54375747475014,-1.,1.66411849222326));
#34377=CARTESIAN_POINT('Ctrl Pts',(3.5363738506022,-1.,1.66294490916111));
#34378=CARTESIAN_POINT('Ctrl Pts',(3.52902746211093,-1.,1.66173058912371));
#34379=CARTESIAN_POINT('Ctrl Pts',(3.52170261543815,-1.,1.66046645222279));
#34380=CARTESIAN_POINT('Ctrl Pts',(3.5143763218894,-1.,1.65913971687342));
#34381=CARTESIAN_POINT('Ctrl Pts',(3.50702733146542,-1.,1.65773832633632));
#34382=CARTESIAN_POINT('Ctrl Pts',(3.4996447647794,-1.,1.65625517961588));
#34383=CARTESIAN_POINT('Ctrl Pts',(3.49223525300176,-1.,1.65469162644468));
#34384=CARTESIAN_POINT('Ctrl Pts',(3.48483492840894,-1.,1.65306335367739));
#34385=CARTESIAN_POINT('Ctrl Pts',(3.47749926256476,-1.,1.65139534930322));
#34386=CARTESIAN_POINT('Ctrl Pts',(3.47028140995992,-1.,1.64971118698256));
#34387=CARTESIAN_POINT('Ctrl Pts',(3.46321237515,-1.,1.64802323352738));
#34388=CARTESIAN_POINT('Ctrl Pts',(3.45628421062422,-1.,1.64632429697521));
#34389=CARTESIAN_POINT('Ctrl Pts',(3.44942242546795,-1.,1.64457408708107));
#34390=CARTESIAN_POINT('Ctrl Pts',(3.44250337701888,-1.,1.64270733821113));
#34391=CARTESIAN_POINT('Ctrl Pts',(3.43540451921548,-1.,1.64065778702023));
#34392=CARTESIAN_POINT('Ctrl Pts',(3.42804772926291,-1.,1.63837876246926));
#34393=CARTESIAN_POINT('Ctrl Pts',(3.42043974590882,-1.,1.63586250099773));
#34394=CARTESIAN_POINT('Ctrl Pts',(3.41272817148478,-1.,1.63316667054044));
#34395=CARTESIAN_POINT('Ctrl Pts',(3.40519422740235,-1.,1.63041148964828));
#34396=CARTESIAN_POINT('Ctrl Pts',(3.39818605297991,-1.,1.62774916464408));
#34397=CARTESIAN_POINT('Ctrl Pts',(3.39206617496906,-1.,1.62533996116713));
#34398=CARTESIAN_POINT('Ctrl Pts',(3.38715832179072,-1.,1.6233278855625));
#34399=CARTESIAN_POINT('Ctrl Pts',(3.38394285763222,-1.,1.62192472202769));
#34400=CARTESIAN_POINT('Ctrl Pts',(3.38243080602408,-1.,1.62118047294498));
#34401=CARTESIAN_POINT('Ctrl Pts',(3.38187506456922,-1.,1.62083271135947));
#34402=CARTESIAN_POINT('Ctrl Pts',(3.38173802621259,-1.,1.62069086551492));
#34403=CARTESIAN_POINT('Ctrl Pts',(3.38171594275764,-1.,1.62064718014094));
#34404=CARTESIAN_POINT('',(3.29885386921599,-1.,1.78327315618183));
#34405=CARTESIAN_POINT('Origin',(0.,-1.,0.));
#34406=CARTESIAN_POINT('',(3.62024382630768,-1.,2.12928030988903));
#34407=CARTESIAN_POINT('Ctrl Pts',(3.29885386921599,-1.,1.78327315618183));
#34408=CARTESIAN_POINT('Ctrl Pts',(3.29890219175522,-1.,1.78326534445426));
#34409=CARTESIAN_POINT('Ctrl Pts',(3.29909749657945,-1.,1.78329283591903));
#34410=CARTESIAN_POINT('Ctrl Pts',(3.29970549824336,-1.,1.78353803106983));
#34411=CARTESIAN_POINT('Ctrl Pts',(3.30119637003466,-1.,1.7843238478823));
#34412=CARTESIAN_POINT('Ctrl Pts',(3.30422155558973,-1.,1.78610045419769));
#34413=CARTESIAN_POINT('Ctrl Pts',(3.30873412266954,-1.,1.78888832245965));
#34414=CARTESIAN_POINT('Ctrl Pts',(3.31428038326763,-1.,1.79242331350137));
#34415=CARTESIAN_POINT('Ctrl Pts',(3.32055355101168,-1.,1.79652817033444));
#34416=CARTESIAN_POINT('Ctrl Pts',(3.3272108803981,-1.,1.80100380443535));
#34417=CARTESIAN_POINT('Ctrl Pts',(3.33392460276874,-1.,1.80565802981139));
#34418=CARTESIAN_POINT('Ctrl Pts',(3.34043216147532,-1.,1.81033399625311));
#34419=CARTESIAN_POINT('Ctrl Pts',(3.34660014370527,-1.,1.81494618732772));
#34420=CARTESIAN_POINT('Ctrl Pts',(3.35243086937451,-1.,1.81948458796748));
#34421=CARTESIAN_POINT('Ctrl Pts',(3.35800801557326,-1.,1.82398496829247));
#34422=CARTESIAN_POINT('Ctrl Pts',(3.36345722124127,-1.,1.82850752153182));
#34423=CARTESIAN_POINT('Ctrl Pts',(3.36890396271864,-1.,1.83311391452338));
#34424=CARTESIAN_POINT('Ctrl Pts',(3.37442462015914,-1.,1.83784072967111));
#34425=CARTESIAN_POINT('Ctrl Pts',(3.38002968341222,-1.,1.84269016931679));
#34426=CARTESIAN_POINT('Ctrl Pts',(3.38569092349639,-1.,1.84764441927778));
#34427=CARTESIAN_POINT('Ctrl Pts',(3.39135802549415,-1.,1.85267433291778));
#34428=CARTESIAN_POINT('Ctrl Pts',(3.39697816833056,-1.,1.85774972037055));
#34429=CARTESIAN_POINT('Ctrl Pts',(3.40251742305445,-1.,1.86285057051228));
#34430=CARTESIAN_POINT('Ctrl Pts',(3.40797080000513,-1.,1.86797231196635));
#34431=CARTESIAN_POINT('Ctrl Pts',(3.41335043875182,-1.,1.87311957248106));
#34432=CARTESIAN_POINT('Ctrl Pts',(3.4186785838376,-1.,1.87830245689338));
#34433=CARTESIAN_POINT('Ctrl Pts',(3.42397908819741,-1.,1.88353205062063));
#34434=CARTESIAN_POINT('Ctrl Pts',(3.42926852222174,-1.,1.88881571322018));
#34435=CARTESIAN_POINT('Ctrl Pts',(3.43455074411591,-1.,1.89415420002553));
#34436=CARTESIAN_POINT('Ctrl Pts',(3.43982185678105,-1.,1.89954426803392));
#34437=CARTESIAN_POINT('Ctrl Pts',(3.44507323983374,-1.,1.90498026502308));
#34438=CARTESIAN_POINT('Ctrl Pts',(3.45029522038885,-1.,1.91045605593638));
#34439=CARTESIAN_POINT('Ctrl Pts',(3.45548074309943,-1.,1.9159669478406));
#34440=CARTESIAN_POINT('Ctrl Pts',(3.4606282172248,-1.,1.9215111821321));
#34441=CARTESIAN_POINT('Ctrl Pts',(3.46573953254084,-1.,1.92708888591159));
#34442=CARTESIAN_POINT('Ctrl Pts',(3.47081872409783,-1.,1.93270136427083));
#34443=CARTESIAN_POINT('Ctrl Pts',(3.47587040389916,-1.,1.93835026973888));
#34444=CARTESIAN_POINT('Ctrl Pts',(3.48089825770411,-1.,1.94403680554062));
#34445=CARTESIAN_POINT('Ctrl Pts',(3.485903616108,-1.,1.94976096795902));
#34446=CARTESIAN_POINT('Ctrl Pts',(3.49088618670967,-1.,1.95552193112071));
#34447=CARTESIAN_POINT('Ctrl Pts',(3.49584466573045,-1.,1.96131836776489));
#34448=CARTESIAN_POINT('Ctrl Pts',(3.50077740176262,-1.,1.9671487972405));
#34449=CARTESIAN_POINT('Ctrl Pts',(3.505683018611,-1.,1.9730119116298));
#34450=CARTESIAN_POINT('Ctrl Pts',(3.51056110478334,-1.,1.97890693666316));
#34451=CARTESIAN_POINT('Ctrl Pts',(3.51541198728362,-1.,1.98483351061066));
#34452=CARTESIAN_POINT('Ctrl Pts',(3.52023644289195,-1.,1.99079153006143));
#34453=CARTESIAN_POINT('Ctrl Pts',(3.52503542491745,-1.,1.99678100339306));
#34454=CARTESIAN_POINT('Ctrl Pts',(3.52980980250181,-1.,2.00280191090341));
#34455=CARTESIAN_POINT('Ctrl Pts',(3.53456004727321,-1.,2.00885403604685));
#34456=CARTESIAN_POINT('Ctrl Pts',(3.53928627453503,-1.,2.0149369884727));
#34457=CARTESIAN_POINT('Ctrl Pts',(3.54398838254011,-1.,2.0210502798303));
#34458=CARTESIAN_POINT('Ctrl Pts',(3.54866616282173,-1.,2.02719338376144));
#34459=CARTESIAN_POINT('Ctrl Pts',(3.55331941294018,-1.,2.03336579658174));
#34460=CARTESIAN_POINT('Ctrl Pts',(3.55794807265052,-1.,2.03956711120099));
#34461=CARTESIAN_POINT('Ctrl Pts',(3.5625522387181,-1.,2.04579702159056));
#34462=CARTESIAN_POINT('Ctrl Pts',(3.56713209978207,-1.,2.05205528173091));
#34463=CARTESIAN_POINT('Ctrl Pts',(3.57168789423507,-1.,2.05834167687524));
#34464=CARTESIAN_POINT('Ctrl Pts',(3.576219862243,-1.,2.06465599229174));
#34465=CARTESIAN_POINT('Ctrl Pts',(3.58072819250442,-1.,2.07099797605747));
#34466=CARTESIAN_POINT('Ctrl Pts',(3.58521300039299,-1.,2.07736732842117));
#34467=CARTESIAN_POINT('Ctrl Pts',(3.58967435355088,-1.,2.08376373048756));
#34468=CARTESIAN_POINT('Ctrl Pts',(3.59411228625588,-1.,2.09018686331416));
#34469=CARTESIAN_POINT('Ctrl Pts',(3.59852681775485,-1.,2.09663642986631));
#34470=CARTESIAN_POINT('Ctrl Pts',(3.60291797088734,-1.,2.1031121772821));
#34471=CARTESIAN_POINT('Ctrl Pts',(3.60728578532601,-1.,2.10961391334462));
#34472=CARTESIAN_POINT('Ctrl Pts',(3.61163030609447,-1.,2.11614149815106));
#34473=CARTESIAN_POINT('Ctrl Pts',(3.61508732216891,-1.,2.12138417126355));
#34474=CARTESIAN_POINT('Ctrl Pts',(3.61766963590482,-1.,2.12532774376758));
#34475=CARTESIAN_POINT('Ctrl Pts',(3.61938653649098,-1.,2.12796193131368));
#34476=CARTESIAN_POINT('Ctrl Pts',(3.62024382630768,-1.,2.12928030988903));
#34477=CARTESIAN_POINT('',(3.54075895182139,-1.,2.25898783642071));
#34478=CARTESIAN_POINT('',(3.62024382630768,-1.,2.12928030988903));
#34479=CARTESIAN_POINT('',(3.08655633322211,-1.,2.1297112484669));
#34480=CARTESIAN_POINT('Ctrl Pts',(3.54075895182139,-1.,2.25898783642071));
#34481=CARTESIAN_POINT('Ctrl Pts',(3.53919506647335,-1.,2.2588225169468));
#34482=CARTESIAN_POINT('Ctrl Pts',(3.53606853162228,-1.,2.25848864343951));
#34483=CARTESIAN_POINT('Ctrl Pts',(3.53138243688262,-1.,2.25797812950104));
#34484=CARTESIAN_POINT('Ctrl Pts',(3.52514172847711,-1.,2.25727802940898));
#34485=CARTESIAN_POINT('Ctrl Pts',(3.51735323667612,-1.,2.25637049455044));
#34486=CARTESIAN_POINT('Ctrl Pts',(3.50957720117341,-1.,2.255430469798));
#34487=CARTESIAN_POINT('Ctrl Pts',(3.50181372617971,-1.,2.25445785151868));
#34488=CARTESIAN_POINT('Ctrl Pts',(3.49406296494791,-1.,2.2534525170976));
#34489=CARTESIAN_POINT('Ctrl Pts',(3.48632513240961,-1.,2.25241433138695));
#34490=CARTESIAN_POINT('Ctrl Pts',(3.47860048448691,-1.,2.25134314238687));
#34491=CARTESIAN_POINT('Ctrl Pts',(3.47088928979888,-1.,2.25023877475942));
#34492=CARTESIAN_POINT('Ctrl Pts',(3.46319180177573,-1.,2.2491010234604));
#34493=CARTESIAN_POINT('Ctrl Pts',(3.45550823512049,-1.,2.2479296496077));
#34494=CARTESIAN_POINT('Ctrl Pts',(3.44783872863151,-1.,2.2467243706995));
#34495=CARTESIAN_POINT('Ctrl Pts',(3.4401833646032,-1.,2.24548487526022));
#34496=CARTESIAN_POINT('Ctrl Pts',(3.43254222614803,-1.,2.24421085338727));
#34497=CARTESIAN_POINT('Ctrl Pts',(3.42491544683008,-1.,2.24290202531101));
#34498=CARTESIAN_POINT('Ctrl Pts',(3.41730325539172,-1.,2.24155816587844));
#34499=CARTESIAN_POINT('Ctrl Pts',(3.40970604190328,-1.,2.24017914395289));
#34500=CARTESIAN_POINT('Ctrl Pts',(3.40212434705647,-1.,2.23876491124151));
#34501=CARTESIAN_POINT('Ctrl Pts',(3.39455873448189,-1.,2.23731541452791));
#34502=CARTESIAN_POINT('Ctrl Pts',(3.38700968549563,-1.,2.23583052276308));
#34503=CARTESIAN_POINT('Ctrl Pts',(3.37947749555632,-1.,2.23430995599561));
#34504=CARTESIAN_POINT('Ctrl Pts',(3.37196214349304,-1.,2.23275319569221));
#34505=CARTESIAN_POINT('Ctrl Pts',(3.36446325227848,-1.,2.23115945849739));
#34506=CARTESIAN_POINT('Ctrl Pts',(3.35698038165483,-1.,2.22952789880983));
#34507=CARTESIAN_POINT('Ctrl Pts',(3.34951327111096,-1.,2.22785777756576));
#34508=CARTESIAN_POINT('Ctrl Pts',(3.34206209449375,-1.,2.22614863918047));
#34509=CARTESIAN_POINT('Ctrl Pts',(3.33462772849598,-1.,2.22440049878511));
#34510=CARTESIAN_POINT('Ctrl Pts',(3.3272119632604,-1.,2.22261398879635));
#34511=CARTESIAN_POINT('Ctrl Pts',(3.31981686778022,-1.,2.22078990842776));
#34512=CARTESIAN_POINT('Ctrl Pts',(3.31244421655666,-1.,2.21892881679086));
#34513=CARTESIAN_POINT('Ctrl Pts',(3.30509487819569,-1.,2.21703059947836));
#34514=CARTESIAN_POINT('Ctrl Pts',(3.29776825193159,-1.,2.21509406923369));
#34515=CARTESIAN_POINT('Ctrl Pts',(3.29046159238343,-1.,2.21311648827391));
#34516=CARTESIAN_POINT('Ctrl Pts',(3.28317133333131,-1.,2.21109449750641));
#34517=CARTESIAN_POINT('Ctrl Pts',(3.2758944800554,-1.,2.2090250941743));
#34518=CARTESIAN_POINT('Ctrl Pts',(3.26863006136782,-1.,2.20690665217743));
#34519=CARTESIAN_POINT('Ctrl Pts',(3.26138036637705,-1.,2.20473979048678));
#34520=CARTESIAN_POINT('Ctrl Pts',(3.25415277957775,-1.,2.20252866491545));
#34521=CARTESIAN_POINT('Ctrl Pts',(3.24695715874338,-1.,2.20027910880981));
#34522=CARTESIAN_POINT('Ctrl Pts',(3.23980245361308,-1.,2.19799623693253));
#34523=CARTESIAN_POINT('Ctrl Pts',(3.23269332296933,-1.,2.19568204933168));
#34524=CARTESIAN_POINT('Ctrl Pts',(3.22562734221646,-1.,2.19333345123538));
#34525=CARTESIAN_POINT('Ctrl Pts',(3.21859043114095,-1.,2.19093901948667));
#34526=CARTESIAN_POINT('Ctrl Pts',(3.21156188355769,-1.,2.18848253363901));
#34527=CARTESIAN_POINT('Ctrl Pts',(3.20452259717976,-1.,2.18594876115934));
#34528=CARTESIAN_POINT('Ctrl Pts',(3.19746293740411,-1.,2.18332898656602));
#34529=CARTESIAN_POINT('Ctrl Pts',(3.19038924261573,-1.,2.18062558031778));
#34530=CARTESIAN_POINT('Ctrl Pts',(3.18333474627807,-1.,2.17785968847142));
#34531=CARTESIAN_POINT('Ctrl Pts',(3.17635032802523,-1.,2.17506466903694));
#34532=CARTESIAN_POINT('Ctrl Pts',(3.16948480019497,-1.,2.17227212063817));
#34533=CARTESIAN_POINT('Ctrl Pts',(3.16276685102972,-1.,2.16949910801219));
#34534=CARTESIAN_POINT('Ctrl Pts',(3.15618975593656,-1.,2.1667372844769));
#34535=CARTESIAN_POINT('Ctrl Pts',(3.14968624389054,-1.,2.16393520288072));
#34536=CARTESIAN_POINT('Ctrl Pts',(3.14314440427022,-1.,2.16100905914435));
#34537=CARTESIAN_POINT('Ctrl Pts',(3.13645356563038,-1.,2.15787423530676));
#34538=CARTESIAN_POINT('Ctrl Pts',(3.12954386795646,-1.,2.1544724138292));
#34539=CARTESIAN_POINT('Ctrl Pts',(3.12242318151938,-1.,2.15079698090585));
#34540=CARTESIAN_POINT('Ctrl Pts',(3.11522827016855,-1.,2.14692798457532));
#34541=CARTESIAN_POINT('Ctrl Pts',(3.10821808668859,-1.,2.14302815601973));
#34542=CARTESIAN_POINT('Ctrl Pts',(3.10171267391049,-1.,2.13930228863751));
#34543=CARTESIAN_POINT('Ctrl Pts',(3.0960450242104,-1.,2.13596538661048));
#34544=CARTESIAN_POINT('Ctrl Pts',(3.09151235281963,-1.,2.13321032560894));
#34545=CARTESIAN_POINT('Ctrl Pts',(3.08855597949761,-1.,2.13132142793017));
#34546=CARTESIAN_POINT('Ctrl Pts',(3.08717896996098,-1.,2.13034980480424));
#34547=CARTESIAN_POINT('Ctrl Pts',(3.08668447250322,-1.,2.12991938762374));
#34548=CARTESIAN_POINT('Ctrl Pts',(3.08657131089497,-1.,2.1297578506149));
#34549=CARTESIAN_POINT('Ctrl Pts',(3.08655633322211,-1.,2.1297112484669));
#34550=CARTESIAN_POINT('',(2.97927412174388,-1.,2.27737254473378));
#34551=CARTESIAN_POINT('Origin',(0.,-1.,0.));
#34552=CARTESIAN_POINT('',(3.24257979115744,-1.,2.66939624221984));
#34553=CARTESIAN_POINT('Ctrl Pts',(2.97927412174388,-1.,2.27737254473378));
#34554=CARTESIAN_POINT('Ctrl Pts',(2.97932307137589,-1.,2.27737238849212));
#34555=CARTESIAN_POINT('Ctrl Pts',(2.97951167106106,-1.,2.27743009389704));
#34556=CARTESIAN_POINT('Ctrl Pts',(2.98007383024333,-1.,2.27776738270369));
#34557=CARTESIAN_POINT('Ctrl Pts',(2.98142341809623,-1.,2.27877674853833));
#34558=CARTESIAN_POINT('Ctrl Pts',(2.98413343613858,-1.,2.28100472516582));
#34559=CARTESIAN_POINT('Ctrl Pts',(2.98815432734929,-1.,2.28446419116036));
#34560=CARTESIAN_POINT('Ctrl Pts',(2.9930793098434,-1.,2.28882328690601));
#34561=CARTESIAN_POINT('Ctrl Pts',(2.99863310340004,-1.,2.29385894577999));
#34562=CARTESIAN_POINT('Ctrl Pts',(3.00450832658822,-1.,2.29932091315939));
#34563=CARTESIAN_POINT('Ctrl Pts',(3.01041131063882,-1.,2.30496809486529));
#34564=CARTESIAN_POINT('Ctrl Pts',(3.01610726819019,-1.,2.31060449886577));
#34565=CARTESIAN_POINT('Ctrl Pts',(3.02147780668029,-1.,2.31612479121528));
#34566=CARTESIAN_POINT('Ctrl Pts',(3.02652678416478,-1.,2.32151944306299));
#34567=CARTESIAN_POINT('Ctrl Pts',(3.03133125185047,-1.,2.32683687412027));
#34568=CARTESIAN_POINT('Ctrl Pts',(3.03600588555765,-1.,2.33215619079807));
#34569=CARTESIAN_POINT('Ctrl Pts',(3.04066496998569,-1.,2.33755792953726));
#34570=CARTESIAN_POINT('Ctrl Pts',(3.04537822217311,-1.,2.3430901708402));
#34571=CARTESIAN_POINT('Ctrl Pts',(3.05015565829976,-1.,2.34875673090816));
#34572=CARTESIAN_POINT('Ctrl Pts',(3.05497218368188,-1.,2.35453559889506));
#34573=CARTESIAN_POINT('Ctrl Pts',(3.05978266240056,-1.,2.36039011602084));
#34574=CARTESIAN_POINT('Ctrl Pts',(3.06453964643152,-1.,2.36628220107001));
#34575=CARTESIAN_POINT('Ctrl Pts',(3.06921275497472,-1.,2.37218678163157));
#34576=CARTESIAN_POINT('Ctrl Pts',(3.07379777492133,-1.,2.37809856205524));
#34577=CARTESIAN_POINT('Ctrl Pts',(3.07830597244301,-1.,2.38402401216107));
#34578=CARTESIAN_POINT('Ctrl Pts',(3.08275773747083,-1.,2.38997659219192));
#34579=CARTESIAN_POINT('Ctrl Pts',(3.08717489512919,-1.,2.39597098250635));
#34580=CARTESIAN_POINT('Ctrl Pts',(3.09157266051115,-1.,2.40201704423352));
#34581=CARTESIAN_POINT('Ctrl Pts',(3.09595472616093,-1.,2.40811612696382));
#34582=CARTESIAN_POINT('Ctrl Pts',(3.10031775027683,-1.,2.41426441798067));
#34583=CARTESIAN_POINT('Ctrl Pts',(3.10465410280902,-1.,2.42045498612494));
#34584=CARTESIAN_POINT('Ctrl Pts',(3.10895518969592,-1.,2.42668025870013));
#34585=CARTESIAN_POINT('Ctrl Pts',(3.11321477659012,-1.,2.4329344968514));
#34586=CARTESIAN_POINT('Ctrl Pts',(3.11743156744182,-1.,2.43921571477975));
#34587=CARTESIAN_POINT('Ctrl Pts',(3.12160740887768,-1.,2.44552433364716));
#34588=CARTESIAN_POINT('Ctrl Pts',(3.12574608210849,-1.,2.45186227369848));
#34589=CARTESIAN_POINT('Ctrl Pts',(3.12985188384372,-1.,2.45823188859367));
#34590=CARTESIAN_POINT('Ctrl Pts',(3.13392826623902,-1.,2.4646349433237));
#34591=CARTESIAN_POINT('Ctrl Pts',(3.13797654408931,-1.,2.47107164236827));
#34592=CARTESIAN_POINT('Ctrl Pts',(3.14199655778845,-1.,2.47754112428028));
#34593=CARTESIAN_POINT('Ctrl Pts',(3.14598722723879,-1.,2.48404187418376));
#34594=CARTESIAN_POINT('Ctrl Pts',(3.14994715298903,-1.,2.49057217131985));
#34595=CARTESIAN_POINT('Ctrl Pts',(3.15387518039064,-1.,2.49713050858911));
#34596=CARTESIAN_POINT('Ctrl Pts',(3.15777102413998,-1.,2.50371605688287));
#34597=CARTESIAN_POINT('Ctrl Pts',(3.16163506380211,-1.,2.51032851007939));
#34598=CARTESIAN_POINT('Ctrl Pts',(3.16546808277069,-1.,2.51696788755616));
#34599=CARTESIAN_POINT('Ctrl Pts',(3.1692710213075,-1.,2.523634346718));
#34600=CARTESIAN_POINT('Ctrl Pts',(3.17304474093574,-1.,2.5303280040691));
#34601=CARTESIAN_POINT('Ctrl Pts',(3.17678974135225,-1.,2.53704871950871));
#34602=CARTESIAN_POINT('Ctrl Pts',(3.18050619750515,-1.,2.54379612552948));
#34603=CARTESIAN_POINT('Ctrl Pts',(3.18419408529482,-1.,2.55056972387638));
#34604=CARTESIAN_POINT('Ctrl Pts',(3.1878532811617,-1.,2.55736896206016));
#34605=CARTESIAN_POINT('Ctrl Pts',(3.19148366395201,-1.,2.56419331092909));
#34606=CARTESIAN_POINT('Ctrl Pts',(3.19508523784548,-1.,2.57104235898053));
#34607=CARTESIAN_POINT('Ctrl Pts',(3.19865814628955,-1.,2.577915819091));
#34608=CARTESIAN_POINT('Ctrl Pts',(3.20220261408685,-1.,2.58481347777953));
#34609=CARTESIAN_POINT('Ctrl Pts',(3.20571891028879,-1.,2.59173516023605));
#34610=CARTESIAN_POINT('Ctrl Pts',(3.2092073056959,-1.,2.59868069194267));
#34611=CARTESIAN_POINT('Ctrl Pts',(3.21266802609297,-1.,2.60564985359699));
#34612=CARTESIAN_POINT('Ctrl Pts',(3.21610123232465,-1.,2.61264236718662));
#34613=CARTESIAN_POINT('Ctrl Pts',(3.21950704108654,-1.,2.61965792832396));
#34614=CARTESIAN_POINT('Ctrl Pts',(3.222885536128,-1.,2.62669622735548));
#34615=CARTESIAN_POINT('Ctrl Pts',(3.22623678292539,-1.,2.63375697391438));
#34616=CARTESIAN_POINT('Ctrl Pts',(3.2295608435934,-1.,2.64083992182478));
#34617=CARTESIAN_POINT('Ctrl Pts',(3.23285778738558,-1.,2.64794488744246));
#34618=CARTESIAN_POINT('Ctrl Pts',(3.23612768065687,-1.,2.6550717396303));
#34619=CARTESIAN_POINT('Ctrl Pts',(3.23872200036311,-1.,2.6607906631973));
#34620=CARTESIAN_POINT('Ctrl Pts',(3.24065561087681,-1.,2.66508964664767));
#34621=CARTESIAN_POINT('Ctrl Pts',(3.24193929584813,-1.,2.66795998539861));
#34622=CARTESIAN_POINT('Ctrl Pts',(3.24257979115744,-1.,2.66939624221984));
#34623=CARTESIAN_POINT('',(3.14378277984898,-1.,2.78507268004356));
#34624=CARTESIAN_POINT('',(3.24257979115744,-1.,2.66939624221984));
#34625=CARTESIAN_POINT('',(2.71539546306948,-1.,2.58633475774921));
#34626=CARTESIAN_POINT('Ctrl Pts',(3.14378277984898,-1.,2.78507268004356));
#34627=CARTESIAN_POINT('Ctrl Pts',(3.14226401018816,-1.,2.7846647503589));
#34628=CARTESIAN_POINT('Ctrl Pts',(3.13922819749279,-1.,2.78384588958166));
#34629=CARTESIAN_POINT('Ctrl Pts',(3.13467965833037,-1.,2.78260859419319));
#34630=CARTESIAN_POINT('Ctrl Pts',(3.12862530318457,-1.,2.78094085161413));
#34631=CARTESIAN_POINT('Ctrl Pts',(3.12107467037201,-1.,2.77882610146731));
#34632=CARTESIAN_POINT('Ctrl Pts',(3.11354142303921,-1.,2.77668121002545));
#34633=CARTESIAN_POINT('Ctrl Pts',(3.10602568032564,-1.,2.77450609123362));
#34634=CARTESIAN_POINT('Ctrl Pts',(3.0985276127786,-1.,2.77230064796057));
#34635=CARTESIAN_POINT('Ctrl Pts',(3.0910474538253,-1.,2.7700647803451));
#34636=CARTESIAN_POINT('Ctrl Pts',(3.08358548001503,-1.,2.76779837829373));
#34637=CARTESIAN_POINT('Ctrl Pts',(3.07614198408862,-1.,2.76550131064852));
#34638=CARTESIAN_POINT('Ctrl Pts',(3.0687172484321,-1.,2.76317341453493));
#34639=CARTESIAN_POINT('Ctrl Pts',(3.06131152247454,-1.,2.76081448759882));
#34640=CARTESIAN_POINT('Ctrl Pts',(3.05392498749847,-1.,2.75842427252931));
#34641=CARTESIAN_POINT('Ctrl Pts',(3.04655777351067,-1.,2.75600247455925));
#34642=CARTESIAN_POINT('Ctrl Pts',(3.03921001107977,-1.,2.75354880060314));
#34643=CARTESIAN_POINT('Ctrl Pts',(3.03188187589107,-1.,2.75106299522979));
#34644=CARTESIAN_POINT('Ctrl Pts',(3.02457362909245,-1.,2.7485448718414));
#34645=CARTESIAN_POINT('Ctrl Pts',(3.01728567646611,-1.,2.74599436193625));
#34646=CARTESIAN_POINT('Ctrl Pts',(3.01001855960162,-1.,2.74341150239887));
#34647=CARTESIAN_POINT('Ctrl Pts',(3.00277284351521,-1.,2.74079632883931));
#34648=CARTESIAN_POINT('Ctrl Pts',(2.99554902409778,-1.,2.73814878711641));
#34649=CARTESIAN_POINT('Ctrl Pts',(2.9883474369644,-1.,2.73546864694536));
#34650=CARTESIAN_POINT('Ctrl Pts',(2.98116814232129,-1.,2.73275539286497));
#34651=CARTESIAN_POINT('Ctrl Pts',(2.97401089032676,-1.,2.73000819218414));
#34652=CARTESIAN_POINT('Ctrl Pts',(2.96687537842451,-1.,2.72722614084076));
#34653=CARTESIAN_POINT('Ctrl Pts',(2.95976146492576,-1.,2.72440846811729));
#34654=CARTESIAN_POINT('Ctrl Pts',(2.95266939280621,-1.,2.72155475123364));
#34655=CARTESIAN_POINT('Ctrl Pts',(2.94560002559805,-1.,2.71866514227965));
#34656=CARTESIAN_POINT('Ctrl Pts',(2.93855503247266,-1.,2.71574054592591));
#34657=CARTESIAN_POINT('Ctrl Pts',(2.93153633192595,-1.,2.71278207520817));
#34658=CARTESIAN_POINT('Ctrl Pts',(2.92454558914778,-1.,2.70979055994754));
#34659=CARTESIAN_POINT('Ctrl Pts',(2.91758367994737,-1.,2.70676602302518));
#34660=CARTESIAN_POINT('Ctrl Pts',(2.91065019668329,-1.,2.70370719782113));
#34661=CARTESIAN_POINT('Ctrl Pts',(2.90374285605838,-1.,2.70061095078692));
#34662=CARTESIAN_POINT('Ctrl Pts',(2.89685866123671,-1.,2.69747340630625));
#34663=CARTESIAN_POINT('Ctrl Pts',(2.88999512410309,-1.,2.69429113011374));
#34664=CARTESIAN_POINT('Ctrl Pts',(2.88315153980466,-1.,2.69106236420198));
#34665=CARTESIAN_POINT('Ctrl Pts',(2.8763300724388,-1.,2.68778807801686));
#34666=CARTESIAN_POINT('Ctrl Pts',(2.86953736547238,-1.,2.68447353139599));
#34667=CARTESIAN_POINT('Ctrl Pts',(2.86278224277689,-1.,2.68112602796308));
#34668=CARTESIAN_POINT('Ctrl Pts',(2.85607274378017,-1.,2.67775201955724));
#34669=CARTESIAN_POINT('Ctrl Pts',(2.84941315703092,-1.,2.67435421039677));
#34670=CARTESIAN_POINT('Ctrl Pts',(2.84280157191323,-1.,2.67092916452125));
#34671=CARTESIAN_POINT('Ctrl Pts',(2.83622586853982,-1.,2.66746339678107));
#34672=CARTESIAN_POINT('Ctrl Pts',(2.82966813308998,-1.,2.6639376472693));
#34673=CARTESIAN_POINT('Ctrl Pts',(2.82311188135078,-1.,2.66033388273461));
#34674=CARTESIAN_POINT('Ctrl Pts',(2.81654896073883,-1.,2.65664198781344));
#34675=CARTESIAN_POINT('Ctrl Pts',(2.80998526078165,-1.,2.65286529532208));
#34676=CARTESIAN_POINT('Ctrl Pts',(2.80345029781152,-1.,2.64902988983337));
#34677=CARTESIAN_POINT('Ctrl Pts',(2.79698910670736,-1.,2.6451766779932));
#34678=CARTESIAN_POINT('Ctrl Pts',(2.79064495573224,-1.,2.64134450532584));
#34679=CARTESIAN_POINT('Ctrl Pts',(2.78444351041571,-1.,2.637554714303));
#34680=CARTESIAN_POINT('Ctrl Pts',(2.77837943466449,-1.,2.63379800904599));
#34681=CARTESIAN_POINT('Ctrl Pts',(2.77239433377921,-1.,2.63001305229625));
#34682=CARTESIAN_POINT('Ctrl Pts',(2.7663907847902,-1.,2.62609956506355));
#34683=CARTESIAN_POINT('Ctrl Pts',(2.76027271596686,-1.,2.62195665834605));
#34684=CARTESIAN_POINT('Ctrl Pts',(2.7539802502603,-1.,2.61751580407667));
#34685=CARTESIAN_POINT('Ctrl Pts',(2.74752219567252,-1.,2.61277170105813));
#34686=CARTESIAN_POINT('Ctrl Pts',(2.7410211099909,-1.,2.60782480638448));
#34687=CARTESIAN_POINT('Ctrl Pts',(2.73470730109615,-1.,2.60287635688728));
#34688=CARTESIAN_POINT('Ctrl Pts',(2.7288648348152,-1.,2.59817869034746));
#34689=CARTESIAN_POINT('Ctrl Pts',(2.72378896977134,-1.,2.59399625537278));
#34690=CARTESIAN_POINT('Ctrl Pts',(2.71974308958086,-1.,2.59056604771971));
#34691=CARTESIAN_POINT('Ctrl Pts',(2.71711860281815,-1.,2.58823792682672));
#34692=CARTESIAN_POINT('Ctrl Pts',(2.71591054189786,-1.,2.58706285424358));
#34693=CARTESIAN_POINT('Ctrl Pts',(2.71548946460575,-1.,2.58656037976753));
#34694=CARTESIAN_POINT('Ctrl Pts',(2.71540296616024,-1.,2.58638312917167));
#34695=CARTESIAN_POINT('Ctrl Pts',(2.71539546306948,-1.,2.58633475774921));
#34696=CARTESIAN_POINT('',(2.58633475775051,-1.,2.71539546306824));
#34697=CARTESIAN_POINT('Origin',(0.,-1.,0.));
#34698=CARTESIAN_POINT('',(2.78507268004355,-1.,3.14378277984898));
#34699=CARTESIAN_POINT('Ctrl Pts',(2.58633475775051,-1.,2.71539546306824));
#34700=CARTESIAN_POINT('Ctrl Pts',(2.58638312917291,-1.,2.71540296615967));
#34701=CARTESIAN_POINT('Ctrl Pts',(2.58656037976884,-1.,2.71548946460616));
#34702=CARTESIAN_POINT('Ctrl Pts',(2.58706285424469,-1.,2.71591054189884));
#34703=CARTESIAN_POINT('Ctrl Pts',(2.58823792682724,-1.,2.7171186028189));
#34704=CARTESIAN_POINT('Ctrl Pts',(2.59056604771863,-1.,2.7197430895797));
#34705=CARTESIAN_POINT('Ctrl Pts',(2.59399625537407,-1.,2.72378896977273));
#34706=CARTESIAN_POINT('Ctrl Pts',(2.5981786903501,-1.,2.72886483481804));
#34707=CARTESIAN_POINT('Ctrl Pts',(2.60287635689,-1.,2.73470730109906));
#34708=CARTESIAN_POINT('Ctrl Pts',(2.60782480638629,-1.,2.74102110999284));
#34709=CARTESIAN_POINT('Ctrl Pts',(2.61277170105864,-1.,2.74752219567307));
#34710=CARTESIAN_POINT('Ctrl Pts',(2.61751580407608,-1.,2.75398025025967));
#34711=CARTESIAN_POINT('Ctrl Pts',(2.62195665834491,-1.,2.76027271596564));
#34712=CARTESIAN_POINT('Ctrl Pts',(2.6260995650624,-1.,2.76639078478898));
#34713=CARTESIAN_POINT('Ctrl Pts',(2.63001305229548,-1.,2.77239433377839));
#34714=CARTESIAN_POINT('Ctrl Pts',(2.63379800904575,-1.,2.77837943466423));
#34715=CARTESIAN_POINT('Ctrl Pts',(2.63755471430322,-1.,2.78444351041594));
#34716=CARTESIAN_POINT('Ctrl Pts',(2.64134450532632,-1.,2.79064495573275));
#34717=CARTESIAN_POINT('Ctrl Pts',(2.6451766779937,-1.,2.7969891067079));
#34718=CARTESIAN_POINT('Ctrl Pts',(2.64902988983373,-1.,2.80345029781191));
#34719=CARTESIAN_POINT('Ctrl Pts',(2.65286529532221,-1.,2.80998526078179));
#34720=CARTESIAN_POINT('Ctrl Pts',(2.65664198781335,-1.,2.81654896073874));
#34721=CARTESIAN_POINT('Ctrl Pts',(2.66033388273437,-1.,2.82311188135053));
#34722=CARTESIAN_POINT('Ctrl Pts',(2.66393764726902,-1.,2.82966813308969));
#34723=CARTESIAN_POINT('Ctrl Pts',(2.66746339678085,-1.,2.8362258685396));
#34724=CARTESIAN_POINT('Ctrl Pts',(2.67092916452116,-1.,2.84280157191314));
#34725=CARTESIAN_POINT('Ctrl Pts',(2.67435421039682,-1.,2.84941315703096));
#34726=CARTESIAN_POINT('Ctrl Pts',(2.67775201955736,-1.,2.85607274378031));
#34727=CARTESIAN_POINT('Ctrl Pts',(2.68112602796323,-1.,2.86278224277705));
#34728=CARTESIAN_POINT('Ctrl Pts',(2.6844735313961,-1.,2.8695373654725));
#34729=CARTESIAN_POINT('Ctrl Pts',(2.68778807801691,-1.,2.87633007243885));
#34730=CARTESIAN_POINT('Ctrl Pts',(2.69106236420196,-1.,2.88315153980464));
#34731=CARTESIAN_POINT('Ctrl Pts',(2.69429113011369,-1.,2.88999512410304));
#34732=CARTESIAN_POINT('Ctrl Pts',(2.69747340630621,-1.,2.89685866123668));
#34733=CARTESIAN_POINT('Ctrl Pts',(2.70061095078692,-1.,2.90374285605839));
#34734=CARTESIAN_POINT('Ctrl Pts',(2.70370719782114,-1.,2.91065019668331));
#34735=CARTESIAN_POINT('Ctrl Pts',(2.70676602302518,-1.,2.91758367994738));
#34736=CARTESIAN_POINT('Ctrl Pts',(2.70979055994751,-1.,2.92454558914774));
#34737=CARTESIAN_POINT('Ctrl Pts',(2.71278207520807,-1.,2.93153633192583));
#34738=CARTESIAN_POINT('Ctrl Pts',(2.71574054592575,-1.,2.93855503247248));
#34739=CARTESIAN_POINT('Ctrl Pts',(2.71866514227951,-1.,2.94560002559789));
#34740=CARTESIAN_POINT('Ctrl Pts',(2.72155475123361,-1.,2.95266939280617));
#34741=CARTESIAN_POINT('Ctrl Pts',(2.72440846811745,-1.,2.95976146492595));
#34742=CARTESIAN_POINT('Ctrl Pts',(2.72722614084112,-1.,2.96687537842492));
#34743=CARTESIAN_POINT('Ctrl Pts',(2.7300081921846,-1.,2.97401089032729));
#34744=CARTESIAN_POINT('Ctrl Pts',(2.73275539286537,-1.,2.98116814232175));
#34745=CARTESIAN_POINT('Ctrl Pts',(2.73546864694548,-1.,2.98834743696455));
#34746=CARTESIAN_POINT('Ctrl Pts',(2.73814878711609,-1.,2.99554902409741));
#34747=CARTESIAN_POINT('Ctrl Pts',(2.74079632883852,-1.,3.00277284351431));
#34748=CARTESIAN_POINT('Ctrl Pts',(2.7434115023978,-1.,3.01001855960041));
#34749=CARTESIAN_POINT('Ctrl Pts',(2.74599436193528,-1.,3.01728567646502));
#34750=CARTESIAN_POINT('Ctrl Pts',(2.74854487184099,-1.,3.02457362909199));
#34751=CARTESIAN_POINT('Ctrl Pts',(2.75106299523032,-1.,3.03188187589168));
#34752=CARTESIAN_POINT('Ctrl Pts',(2.75354880060473,-1.,3.03921001108158));
#34753=CARTESIAN_POINT('Ctrl Pts',(2.7560024745616,-1.,3.04655777351333));
#34754=CARTESIAN_POINT('Ctrl Pts',(2.75842427253164,-1.,3.05392498750112));
#34755=CARTESIAN_POINT('Ctrl Pts',(2.76081448760011,-1.,3.06131152247599));
#34756=CARTESIAN_POINT('Ctrl Pts',(2.76317341453415,-1.,3.06871724843121));
#34757=CARTESIAN_POINT('Ctrl Pts',(2.76550131064522,-1.,3.07614198408488));
#34758=CARTESIAN_POINT('Ctrl Pts',(2.76779837828843,-1.,3.08358548000904));
#34759=CARTESIAN_POINT('Ctrl Pts',(2.77006478033937,-1.,3.09104745381882));
#34760=CARTESIAN_POINT('Ctrl Pts',(2.77230064795679,-1.,3.09852761277432));
#34761=CARTESIAN_POINT('Ctrl Pts',(2.7745060912343,-1.,3.10602568032641));
#34762=CARTESIAN_POINT('Ctrl Pts',(2.77668121003225,-1.,3.11354142304692));
#34763=CARTESIAN_POINT('Ctrl Pts',(2.77882610147986,-1.,3.12107467038623));
#34764=CARTESIAN_POINT('Ctrl Pts',(2.78094085162947,-1.,3.12862530320194));
#34765=CARTESIAN_POINT('Ctrl Pts',(2.78260859420629,-1.,3.1346796583452));
#34766=CARTESIAN_POINT('Ctrl Pts',(2.78384588958965,-1.,3.13922819750185));
#34767=CARTESIAN_POINT('Ctrl Pts',(2.78466475036183,-1.,3.14226401019149));
#34768=CARTESIAN_POINT('Ctrl Pts',(2.78507268004355,-1.,3.14378277984898));
#34769=CARTESIAN_POINT('',(2.66939624221984,-1.,3.24257979115744));
#34770=CARTESIAN_POINT('',(2.78507268004355,-1.,3.14378277984898));
#34771=CARTESIAN_POINT('',(2.27737254473521,-1.,2.97927412174279));
#34772=CARTESIAN_POINT('Ctrl Pts',(2.66939624221984,-1.,3.24257979115744));
#34773=CARTESIAN_POINT('Ctrl Pts',(2.66795998539579,-1.,3.24193929584471));
#34774=CARTESIAN_POINT('Ctrl Pts',(2.66508964663997,-1.,3.24065561086749));
#34775=CARTESIAN_POINT('Ctrl Pts',(2.6607906631847,-1.,3.23872200034785));
#34776=CARTESIAN_POINT('Ctrl Pts',(2.65507173961555,-1.,3.236127680639));
#34777=CARTESIAN_POINT('Ctrl Pts',(2.64794488743038,-1.,3.23285778737096));
#34778=CARTESIAN_POINT('Ctrl Pts',(2.64083992181823,-1.,3.22956084358547));
#34779=CARTESIAN_POINT('Ctrl Pts',(2.63375697391372,-1.,3.2262367829246));
#34780=CARTESIAN_POINT('Ctrl Pts',(2.62669622735912,-1.,3.2228855361324));
#34781=CARTESIAN_POINT('Ctrl Pts',(2.61965792832947,-1.,3.21950704109321));
#34782=CARTESIAN_POINT('Ctrl Pts',(2.61264236719171,-1.,3.21610123233082));
#34783=CARTESIAN_POINT('Ctrl Pts',(2.60564985360017,-1.,3.21266802609682));
#34784=CARTESIAN_POINT('Ctrl Pts',(2.59868069194341,-1.,3.20920730569681));
#34785=CARTESIAN_POINT('Ctrl Pts',(2.59173516023481,-1.,3.2057189102873));
#34786=CARTESIAN_POINT('Ctrl Pts',(2.58481347777728,-1.,3.20220261408414));
#34787=CARTESIAN_POINT('Ctrl Pts',(2.57791581908874,-1.,3.19865814628682));
#34788=CARTESIAN_POINT('Ctrl Pts',(2.57104235897899,-1.,3.19508523784363));
#34789=CARTESIAN_POINT('Ctrl Pts',(2.56419331092858,-1.,3.19148366395139));
#34790=CARTESIAN_POINT('Ctrl Pts',(2.55736896206056,-1.,3.18785328116218));
#34791=CARTESIAN_POINT('Ctrl Pts',(2.5505697238773,-1.,3.18419408529594));
#34792=CARTESIAN_POINT('Ctrl Pts',(2.5437961255305,-1.,3.1805061975064));
#34793=CARTESIAN_POINT('Ctrl Pts',(2.53704871950948,-1.,3.17678974135318));
#34794=CARTESIAN_POINT('Ctrl Pts',(2.53032800406941,-1.,3.17304474093612));
#34795=CARTESIAN_POINT('Ctrl Pts',(2.52363434671788,-1.,3.16927102130736));
#34796=CARTESIAN_POINT('Ctrl Pts',(2.51696788755577,-1.,3.16546808277023));
#34797=CARTESIAN_POINT('Ctrl Pts',(2.51032851007894,-1.,3.16163506380157));
#34798=CARTESIAN_POINT('Ctrl Pts',(2.50371605688252,-1.,3.15777102413957));
#34799=CARTESIAN_POINT('Ctrl Pts',(2.49713050858896,-1.,3.15387518039046));
#34800=CARTESIAN_POINT('Ctrl Pts',(2.49057217131988,-1.,3.14994715298907));
#34801=CARTESIAN_POINT('Ctrl Pts',(2.4840418741839,-1.,3.14598722723896));
#34802=CARTESIAN_POINT('Ctrl Pts',(2.47754112428043,-1.,3.14199655778863));
#34803=CARTESIAN_POINT('Ctrl Pts',(2.47107164236838,-1.,3.13797654408943));
#34804=CARTESIAN_POINT('Ctrl Pts',(2.46463494332374,-1.,3.13392826623906));
#34805=CARTESIAN_POINT('Ctrl Pts',(2.45823188859366,-1.,3.12985188384371));
#34806=CARTESIAN_POINT('Ctrl Pts',(2.45186227369846,-1.,3.12574608210847));
#34807=CARTESIAN_POINT('Ctrl Pts',(2.44552433364715,-1.,3.12160740887768));
#34808=CARTESIAN_POINT('Ctrl Pts',(2.43921571477977,-1.,3.11743156744186));
#34809=CARTESIAN_POINT('Ctrl Pts',(2.43293449685144,-1.,3.11321477659018));
#34810=CARTESIAN_POINT('Ctrl Pts',(2.42668025870015,-1.,3.10895518969595));
#34811=CARTESIAN_POINT('Ctrl Pts',(2.42045498612489,-1.,3.10465410280896));
#34812=CARTESIAN_POINT('Ctrl Pts',(2.41426441798057,-1.,3.1003177502767));
#34813=CARTESIAN_POINT('Ctrl Pts',(2.40811612696369,-1.,3.09595472616076));
#34814=CARTESIAN_POINT('Ctrl Pts',(2.40201704423341,-1.,3.091572660511));
#34815=CARTESIAN_POINT('Ctrl Pts',(2.39597098250631,-1.,3.08717489512914));
#34816=CARTESIAN_POINT('Ctrl Pts',(2.38997659219199,-1.,3.08275773747093));
#34817=CARTESIAN_POINT('Ctrl Pts',(2.38402401216126,-1.,3.07830597244326));
#34818=CARTESIAN_POINT('Ctrl Pts',(2.37809856205548,-1.,3.07379777492165));
#34819=CARTESIAN_POINT('Ctrl Pts',(2.37218678163178,-1.,3.069212754975));
#34820=CARTESIAN_POINT('Ctrl Pts',(2.36628220107009,-1.,3.06453964643162));
#34821=CARTESIAN_POINT('Ctrl Pts',(2.36039011602072,-1.,3.0597826624004));
#34822=CARTESIAN_POINT('Ctrl Pts',(2.35453559889474,-1.,3.05497218368146));
#34823=CARTESIAN_POINT('Ctrl Pts',(2.3487567309077,-1.,3.05015565829918));
#34824=CARTESIAN_POINT('Ctrl Pts',(2.34309017083976,-1.,3.04537822217256));
#34825=CARTESIAN_POINT('Ctrl Pts',(2.33755792953706,-1.,3.04066496998544));
#34826=CARTESIAN_POINT('Ctrl Pts',(2.33215619079829,-1.,3.03600588555793));
#34827=CARTESIAN_POINT('Ctrl Pts',(2.32683687412096,-1.,3.03133125185136));
#34828=CARTESIAN_POINT('Ctrl Pts',(2.32151944306402,-1.,3.02652678416611));
#34829=CARTESIAN_POINT('Ctrl Pts',(2.31612479121631,-1.,3.02147780668161));
#34830=CARTESIAN_POINT('Ctrl Pts',(2.31060449886629,-1.,3.01610726819086));
#34831=CARTESIAN_POINT('Ctrl Pts',(2.30496809486482,-1.,3.01041131063823));
#34832=CARTESIAN_POINT('Ctrl Pts',(2.29932091315775,-1.,3.00450832658613));
#34833=CARTESIAN_POINT('Ctrl Pts',(2.29385894577754,-1.,2.99863310339691));
#34834=CARTESIAN_POINT('Ctrl Pts',(2.28882328690362,-1.,2.99307930984034));
#34835=CARTESIAN_POINT('Ctrl Pts',(2.28446419115919,-1.,2.9881543273478));
#34836=CARTESIAN_POINT('Ctrl Pts',(2.28100472516679,-1.,2.98413343613983));
#34837=CARTESIAN_POINT('Ctrl Pts',(2.27877674853766,-1.,2.9814234180956));
#34838=CARTESIAN_POINT('Ctrl Pts',(2.27776738270289,-1.,2.98007383024207));
#34839=CARTESIAN_POINT('Ctrl Pts',(2.27743009389684,-1.,2.9795116710597));
#34840=CARTESIAN_POINT('Ctrl Pts',(2.27737238849287,-1.,2.97932307137476));
#34841=CARTESIAN_POINT('Ctrl Pts',(2.27737254473521,-1.,2.97927412174279));
#34842=CARTESIAN_POINT('',(2.12971124846838,-1.,3.08655633322109));
#34843=CARTESIAN_POINT('Origin',(0.,-1.,0.));
#34844=CARTESIAN_POINT('',(2.25898783642071,-1.,3.54075895182139));
#34845=CARTESIAN_POINT('Ctrl Pts',(2.12971124846838,-1.,3.08655633322109));
#34846=CARTESIAN_POINT('Ctrl Pts',(2.1297578506162,-1.,3.0865713108946));
#34847=CARTESIAN_POINT('Ctrl Pts',(2.12991938762497,-1.,3.08668447250383));
#34848=CARTESIAN_POINT('Ctrl Pts',(2.13034980480519,-1.,3.08717896996213));
#34849=CARTESIAN_POINT('Ctrl Pts',(2.13132142793056,-1.,3.08855597949844));
#34850=CARTESIAN_POINT('Ctrl Pts',(2.13321032560805,-1.,3.09151235281832));
#34851=CARTESIAN_POINT('Ctrl Pts',(2.13596538661154,-1.,3.09604502421197));
#34852=CARTESIAN_POINT('Ctrl Pts',(2.13930228863968,-1.,3.1017126739137));
#34853=CARTESIAN_POINT('Ctrl Pts',(2.14302815602195,-1.,3.10821808669189));
#34854=CARTESIAN_POINT('Ctrl Pts',(2.1469279845768,-1.,3.11522827017075));
#34855=CARTESIAN_POINT('Ctrl Pts',(2.15079698090627,-1.,3.12242318152001));
#34856=CARTESIAN_POINT('Ctrl Pts',(2.15447241382872,-1.,3.12954386795575));
#34857=CARTESIAN_POINT('Ctrl Pts',(2.15787423530583,-1.,3.136453565629));
#34858=CARTESIAN_POINT('Ctrl Pts',(2.16100905914341,-1.,3.14314440426882));
#34859=CARTESIAN_POINT('Ctrl Pts',(2.16393520288009,-1.,3.14968624388961));
#34860=CARTESIAN_POINT('Ctrl Pts',(2.1667372844767,-1.,3.15618975593627));
#34861=CARTESIAN_POINT('Ctrl Pts',(2.16949910801237,-1.,3.16276685102999));
#34862=CARTESIAN_POINT('Ctrl Pts',(2.17227212063857,-1.,3.16948480019555));
#34863=CARTESIAN_POINT('Ctrl Pts',(2.17506466903736,-1.,3.17635032802584));
#34864=CARTESIAN_POINT('Ctrl Pts',(2.17785968847172,-1.,3.18333474627851));
#34865=CARTESIAN_POINT('Ctrl Pts',(2.18062558031789,-1.,3.19038924261589));
#34866=CARTESIAN_POINT('Ctrl Pts',(2.18332898656595,-1.,3.197462937404));
#34867=CARTESIAN_POINT('Ctrl Pts',(2.18594876115914,-1.,3.20452259717947));
#34868=CARTESIAN_POINT('Ctrl Pts',(2.18848253363878,-1.,3.21156188355736));
#34869=CARTESIAN_POINT('Ctrl Pts',(2.1909390194865,-1.,3.21859043114069));
#34870=CARTESIAN_POINT('Ctrl Pts',(2.19333345123531,-1.,3.22562734221636));
#34871=CARTESIAN_POINT('Ctrl Pts',(2.19568204933172,-1.,3.23269332296938));
#34872=CARTESIAN_POINT('Ctrl Pts',(2.19799623693263,-1.,3.23980245361323));
#34873=CARTESIAN_POINT('Ctrl Pts',(2.20027910880993,-1.,3.24695715874356));
#34874=CARTESIAN_POINT('Ctrl Pts',(2.20252866491554,-1.,3.25415277957789));
#34875=CARTESIAN_POINT('Ctrl Pts',(2.20473979048682,-1.,3.26138036637711));
#34876=CARTESIAN_POINT('Ctrl Pts',(2.20690665217741,-1.,3.2686300613678));
#34877=CARTESIAN_POINT('Ctrl Pts',(2.20902509417425,-1.,3.27589448005534));
#34878=CARTESIAN_POINT('Ctrl Pts',(2.21109449750638,-1.,3.28317133333127));
#34879=CARTESIAN_POINT('Ctrl Pts',(2.2131164882739,-1.,3.29046159238344));
#34880=CARTESIAN_POINT('Ctrl Pts',(2.21509406923369,-1.,3.29776825193162));
#34881=CARTESIAN_POINT('Ctrl Pts',(2.21703059947837,-1.,3.3050948781957));
#34882=CARTESIAN_POINT('Ctrl Pts',(2.21892881679083,-1.,3.31244421655662));
#34883=CARTESIAN_POINT('Ctrl Pts',(2.22078990842768,-1.,3.31981686778008));
#34884=CARTESIAN_POINT('Ctrl Pts',(2.22261398879623,-1.,3.32721196326019));
#34885=CARTESIAN_POINT('Ctrl Pts',(2.224400498785,-1.,3.3346277284958));
#34886=CARTESIAN_POINT('Ctrl Pts',(2.22614863918044,-1.,3.34206209449371));
#34887=CARTESIAN_POINT('Ctrl Pts',(2.22785777756588,-1.,3.34951327111117));
#34888=CARTESIAN_POINT('Ctrl Pts',(2.22952789881011,-1.,3.35698038165529));
#34889=CARTESIAN_POINT('Ctrl Pts',(2.23115945849777,-1.,3.36446325227908));
#34890=CARTESIAN_POINT('Ctrl Pts',(2.23275319569253,-1.,3.37196214349356));
#34891=CARTESIAN_POINT('Ctrl Pts',(2.23430995599572,-1.,3.37947749555649));
#34892=CARTESIAN_POINT('Ctrl Pts',(2.23583052276281,-1.,3.38700968549522));
#34893=CARTESIAN_POINT('Ctrl Pts',(2.23731541452726,-1.,3.39455873448088));
#34894=CARTESIAN_POINT('Ctrl Pts',(2.23876491124064,-1.,3.40212434705511));
#34895=CARTESIAN_POINT('Ctrl Pts',(2.24017914395211,-1.,3.40970604190205));
#34896=CARTESIAN_POINT('Ctrl Pts',(2.24155816587811,-1.,3.41730325539119));
#34897=CARTESIAN_POINT('Ctrl Pts',(2.24290202531144,-1.,3.42491544683075));
#34898=CARTESIAN_POINT('Ctrl Pts',(2.24421085338856,-1.,3.43254222615007));
#34899=CARTESIAN_POINT('Ctrl Pts',(2.24548487526212,-1.,3.44018336460619));
#34900=CARTESIAN_POINT('Ctrl Pts',(2.24672437070139,-1.,3.44783872863448));
#34901=CARTESIAN_POINT('Ctrl Pts',(2.24792964960874,-1.,3.45550823512213));
#34902=CARTESIAN_POINT('Ctrl Pts',(2.24910102345977,-1.,3.46319180177474));
#34903=CARTESIAN_POINT('Ctrl Pts',(2.25023877475674,-1.,3.47088928979467));
#34904=CARTESIAN_POINT('Ctrl Pts',(2.25134314238258,-1.,3.47860048448015));
#34905=CARTESIAN_POINT('Ctrl Pts',(2.25241433138231,-1.,3.48632513240231));
#34906=CARTESIAN_POINT('Ctrl Pts',(2.25345251709453,-1.,3.49406296494309));
#34907=CARTESIAN_POINT('Ctrl Pts',(2.25445785151923,-1.,3.50181372618058));
#34908=CARTESIAN_POINT('Ctrl Pts',(2.25543046980351,-1.,3.50957720118209));
#34909=CARTESIAN_POINT('Ctrl Pts',(2.25637049456061,-1.,3.51735323669213));
#34910=CARTESIAN_POINT('Ctrl Pts',(2.25727802942141,-1.,3.52514172849666));
#34911=CARTESIAN_POINT('Ctrl Pts',(2.25797812951166,-1.,3.53138243689932));
#34912=CARTESIAN_POINT('Ctrl Pts',(2.25848864344599,-1.,3.53606853163247));
#34913=CARTESIAN_POINT('Ctrl Pts',(2.25882251694918,-1.,3.5391950664771));
#34914=CARTESIAN_POINT('Ctrl Pts',(2.25898783642071,-1.,3.54075895182139));
#34915=CARTESIAN_POINT('',(2.12928030988903,-1.,3.62024382630768));
#34916=CARTESIAN_POINT('',(2.25898783642071,-1.,3.54075895182139));
#34917=CARTESIAN_POINT('',(1.78327315618341,-1.,3.29885386921513));
#34918=CARTESIAN_POINT('Ctrl Pts',(2.12928030988903,-1.,3.62024382630768));
#34919=CARTESIAN_POINT('Ctrl Pts',(2.12796193131142,-1.,3.61938653648716));
#34920=CARTESIAN_POINT('Ctrl Pts',(2.12532774376144,-1.,3.61766963589442));
#34921=CARTESIAN_POINT('Ctrl Pts',(2.12138417125349,-1.,3.61508732215187));
#34922=CARTESIAN_POINT('Ctrl Pts',(2.11614149813928,-1.,3.61163030607452));
#34923=CARTESIAN_POINT('Ctrl Pts',(2.10961391333497,-1.,3.60728578530968));
#34924=CARTESIAN_POINT('Ctrl Pts',(2.10311217727687,-1.,3.60291797087849));
#34925=CARTESIAN_POINT('Ctrl Pts',(2.09663642986579,-1.,3.59852681775396));
#34926=CARTESIAN_POINT('Ctrl Pts',(2.09018686331706,-1.,3.5941122862608));
#34927=CARTESIAN_POINT('Ctrl Pts',(2.08376373049196,-1.,3.58967435355834));
#34928=CARTESIAN_POINT('Ctrl Pts',(2.07736732842524,-1.,3.58521300039988));
#34929=CARTESIAN_POINT('Ctrl Pts',(2.07099797606,-1.,3.58072819250872));
#34930=CARTESIAN_POINT('Ctrl Pts',(2.06465599229234,-1.,3.57621986224402));
#34931=CARTESIAN_POINT('Ctrl Pts',(2.05834167687425,-1.,3.5716878942334));
#34932=CARTESIAN_POINT('Ctrl Pts',(2.05205528172911,-1.,3.56713209977904));
#34933=CARTESIAN_POINT('Ctrl Pts',(2.04579702158876,-1.,3.56255223871505));
#34934=CARTESIAN_POINT('Ctrl Pts',(2.03956711119976,-1.,3.55794807264844));
#34935=CARTESIAN_POINT('Ctrl Pts',(2.03336579658133,-1.,3.55331941293949));
#34936=CARTESIAN_POINT('Ctrl Pts',(2.02719338376175,-1.,3.54866616282227));
#34937=CARTESIAN_POINT('Ctrl Pts',(2.02105027983104,-1.,3.54398838254136));
#34938=CARTESIAN_POINT('Ctrl Pts',(2.01493698847351,-1.,3.53928627453642));
#34939=CARTESIAN_POINT('Ctrl Pts',(2.00885403604746,-1.,3.53456004727424));
#34940=CARTESIAN_POINT('Ctrl Pts',(2.00280191090366,-1.,3.52980980250224));
#34941=CARTESIAN_POINT('Ctrl Pts',(1.99678100339295,-1.,3.52503542491728));
#34942=CARTESIAN_POINT('Ctrl Pts',(1.99079153006112,-1.,3.52023644289142));
#34943=CARTESIAN_POINT('Ctrl Pts',(1.9848335106103,-1.,3.51541198728301));
#34944=CARTESIAN_POINT('Ctrl Pts',(1.97890693666288,-1.,3.51056110478287));
#34945=CARTESIAN_POINT('Ctrl Pts',(1.97301191162968,-1.,3.5056830186108));
#34946=CARTESIAN_POINT('Ctrl Pts',(1.96714879724052,-1.,3.50077740176267));
#34947=CARTESIAN_POINT('Ctrl Pts',(1.961318367765,-1.,3.49584466573064));
#34948=CARTESIAN_POINT('Ctrl Pts',(1.95552193112084,-1.,3.49088618670987));
#34949=CARTESIAN_POINT('Ctrl Pts',(1.94976096795911,-1.,3.48590361610814));
#34950=CARTESIAN_POINT('Ctrl Pts',(1.94403680554065,-1.,3.48089825770416));
#34951=CARTESIAN_POINT('Ctrl Pts',(1.93835026973887,-1.,3.47587040389915));
#34952=CARTESIAN_POINT('Ctrl Pts',(1.93270136427081,-1.,3.47081872409781));
#34953=CARTESIAN_POINT('Ctrl Pts',(1.92708888591158,-1.,3.46573953254084));
#34954=CARTESIAN_POINT('Ctrl Pts',(1.92151118213212,-1.,3.46062821722485));
#34955=CARTESIAN_POINT('Ctrl Pts',(1.91596694784063,-1.,3.4554807430995));
#34956=CARTESIAN_POINT('Ctrl Pts',(1.91045605593639,-1.,3.45029522038888));
#34957=CARTESIAN_POINT('Ctrl Pts',(1.90498026502304,-1.,3.44507323983368));
#34958=CARTESIAN_POINT('Ctrl Pts',(1.89954426803384,-1.,3.4398218567809));
#34959=CARTESIAN_POINT('Ctrl Pts',(1.89415420002542,-1.,3.43455074411571));
#34960=CARTESIAN_POINT('Ctrl Pts',(1.88881571322009,-1.,3.42926852222158));
#34961=CARTESIAN_POINT('Ctrl Pts',(1.8835320506206,-1.,3.42397908819736));
#34962=CARTESIAN_POINT('Ctrl Pts',(1.87830245689344,-1.,3.41867858383771));
#34963=CARTESIAN_POINT('Ctrl Pts',(1.87311957248121,-1.,3.41335043875209));
#34964=CARTESIAN_POINT('Ctrl Pts',(1.86797231196654,-1.,3.40797080000549));
#34965=CARTESIAN_POINT('Ctrl Pts',(1.86285057051245,-1.,3.40251742305476));
#34966=CARTESIAN_POINT('Ctrl Pts',(1.85774972037062,-1.,3.39697816833067));
#34967=CARTESIAN_POINT('Ctrl Pts',(1.85267433291769,-1.,3.39135802549398));
#34968=CARTESIAN_POINT('Ctrl Pts',(1.84764441927753,-1.,3.38569092349592));
#34969=CARTESIAN_POINT('Ctrl Pts',(1.84269016931643,-1.,3.38002968341157));
#34970=CARTESIAN_POINT('Ctrl Pts',(1.83784072967077,-1.,3.37442462015853));
#34971=CARTESIAN_POINT('Ctrl Pts',(1.83311391452322,-1.,3.36890396271836));
#34972=CARTESIAN_POINT('Ctrl Pts',(1.82850752153199,-1.,3.36345722124158));
#34973=CARTESIAN_POINT('Ctrl Pts',(1.82398496829301,-1.,3.35800801557424));
#34974=CARTESIAN_POINT('Ctrl Pts',(1.81948458796829,-1.,3.35243086937598));
#34975=CARTESIAN_POINT('Ctrl Pts',(1.81494618732853,-1.,3.34660014370673));
#34976=CARTESIAN_POINT('Ctrl Pts',(1.81033399625352,-1.,3.34043216147606));
#34977=CARTESIAN_POINT('Ctrl Pts',(1.80565802981102,-1.,3.33392460276808));
#34978=CARTESIAN_POINT('Ctrl Pts',(1.80100380443406,-1.,3.32721088039578));
#34979=CARTESIAN_POINT('Ctrl Pts',(1.79652817033251,-1.,3.3205535510082));
#34980=CARTESIAN_POINT('Ctrl Pts',(1.79242331349949,-1.,3.31428038326424));
#34981=CARTESIAN_POINT('Ctrl Pts',(1.78888832245873,-1.,3.30873412266788));
#34982=CARTESIAN_POINT('Ctrl Pts',(1.78610045419846,-1.,3.30422155559112));
#34983=CARTESIAN_POINT('Ctrl Pts',(1.78432384788174,-1.,3.30119637003393));
#34984=CARTESIAN_POINT('Ctrl Pts',(1.78353803106924,-1.,3.299705498242));
#34985=CARTESIAN_POINT('Ctrl Pts',(1.78329283591905,-1.,3.29909749657808));
#34986=CARTESIAN_POINT('Ctrl Pts',(1.78326534445518,-1.,3.29890219175423));
#34987=CARTESIAN_POINT('Ctrl Pts',(1.78327315618341,-1.,3.29885386921513));
#34988=CARTESIAN_POINT('',(1.62064718014256,-1.,3.38171594275687));
#34989=CARTESIAN_POINT('Origin',(0.,-1.,0.));
#34990=CARTESIAN_POINT('',(1.67727921511438,-1.,3.85054988729471));
#34991=CARTESIAN_POINT('Ctrl Pts',(1.62064718014256,-1.,3.38171594275687));
#34992=CARTESIAN_POINT('Ctrl Pts',(1.62069086551626,-1.,3.38173802621243));
#34993=CARTESIAN_POINT('Ctrl Pts',(1.62083271136059,-1.,3.38187506457001));
#34994=CARTESIAN_POINT('Ctrl Pts',(1.62118047294574,-1.,3.38243080602536));
#34995=CARTESIAN_POINT('Ctrl Pts',(1.62192472202795,-1.,3.3839428576331));
#34996=CARTESIAN_POINT('Ctrl Pts',(1.62332788556183,-1.,3.38715832178929));
#34997=CARTESIAN_POINT('Ctrl Pts',(1.62533996116793,-1.,3.39206617497078));
#34998=CARTESIAN_POINT('Ctrl Pts',(1.62774916464571,-1.,3.39818605298342));
#34999=CARTESIAN_POINT('Ctrl Pts',(1.63041148964996,-1.,3.40519422740596));
#35000=CARTESIAN_POINT('Ctrl Pts',(1.63316667054156,-1.,3.41272817148719));
#35001=CARTESIAN_POINT('Ctrl Pts',(1.63586250099804,-1.,3.4204397459095));
#35002=CARTESIAN_POINT('Ctrl Pts',(1.6383787624689,-1.,3.42804772926214));
#35003=CARTESIAN_POINT('Ctrl Pts',(1.64065778701952,-1.,3.43540451921397));
#35004=CARTESIAN_POINT('Ctrl Pts',(1.64270733821042,-1.,3.44250337701736));
#35005=CARTESIAN_POINT('Ctrl Pts',(1.64457408708059,-1.,3.44942242546693));
#35006=CARTESIAN_POINT('Ctrl Pts',(1.64632429697506,-1.,3.4562842106239));
#35007=CARTESIAN_POINT('Ctrl Pts',(1.64802323352752,-1.,3.46321237515029));
#35008=CARTESIAN_POINT('Ctrl Pts',(1.64971118698285,-1.,3.47028140996055));
#35009=CARTESIAN_POINT('Ctrl Pts',(1.65139534930353,-1.,3.47749926256543));
#35010=CARTESIAN_POINT('Ctrl Pts',(1.65306335367762,-1.,3.48483492840942));
#35011=CARTESIAN_POINT('Ctrl Pts',(1.65469162644476,-1.,3.49223525300194));
#35012=CARTESIAN_POINT('Ctrl Pts',(1.65625517961583,-1.,3.49964476477929));
#35013=CARTESIAN_POINT('Ctrl Pts',(1.65773832633617,-1.,3.5070273314651));
#35014=CARTESIAN_POINT('Ctrl Pts',(1.65913971687324,-1.,3.51437632188903));
#35015=CARTESIAN_POINT('Ctrl Pts',(1.66046645222266,-1.,3.52170261543787));
#35016=CARTESIAN_POINT('Ctrl Pts',(1.66173058912365,-1.,3.52902746211082));
#35017=CARTESIAN_POINT('Ctrl Pts',(1.66294490916113,-1.,3.53637385060225));
#35018=CARTESIAN_POINT('Ctrl Pts',(1.66411849222334,-1.,3.5437574747503));
#35019=CARTESIAN_POINT('Ctrl Pts',(1.66525401569004,-1.,3.5511812134288));
#35020=CARTESIAN_POINT('Ctrl Pts',(1.66635023293121,-1.,3.55864015233617));
#35021=CARTESIAN_POINT('Ctrl Pts',(1.66740349220308,-1.,3.56612465179429));
#35022=CARTESIAN_POINT('Ctrl Pts',(1.66840957407299,-1.,3.57362406285884));
#35023=CARTESIAN_POINT('Ctrl Pts',(1.66936552908228,-1.,3.58113044183823));
#35024=CARTESIAN_POINT('Ctrl Pts',(1.67027110397601,-1.,3.5886414309783));
#35025=CARTESIAN_POINT('Ctrl Pts',(1.67112775290706,-1.,3.59615824388808));
#35026=CARTESIAN_POINT('Ctrl Pts',(1.67193797318598,-1.,3.60368430815203));
#35027=CARTESIAN_POINT('Ctrl Pts',(1.67270452466968,-1.,3.61122367156182));
#35028=CARTESIAN_POINT('Ctrl Pts',(1.67342968196223,-1.,3.61877947398179));
#35029=CARTESIAN_POINT('Ctrl Pts',(1.67411452372265,-1.,3.62635249450908));
#35030=CARTESIAN_POINT('Ctrl Pts',(1.67475929882962,-1.,3.63394189312902));
#35031=CARTESIAN_POINT('Ctrl Pts',(1.67536373264839,-1.,3.6415458297232));
#35032=CARTESIAN_POINT('Ctrl Pts',(1.6759273594669,-1.,3.64916213574663));
#35033=CARTESIAN_POINT('Ctrl Pts',(1.67644983469459,-1.,3.65678894416442));
#35034=CARTESIAN_POINT('Ctrl Pts',(1.67693128053153,-1.,3.66442538671018));
#35035=CARTESIAN_POINT('Ctrl Pts',(1.67737217414901,-1.,3.67207136294639));
#35036=CARTESIAN_POINT('Ctrl Pts',(1.67777320475872,-1.,3.6797272457918));
#35037=CARTESIAN_POINT('Ctrl Pts',(1.67813513867973,-1.,3.68739360236505));
#35038=CARTESIAN_POINT('Ctrl Pts',(1.67845869064304,-1.,3.69507092759545));
#35039=CARTESIAN_POINT('Ctrl Pts',(1.6787443694862,-1.,3.70275932350998));
#35040=CARTESIAN_POINT('Ctrl Pts',(1.67899249793398,-1.,3.71045854208195));
#35041=CARTESIAN_POINT('Ctrl Pts',(1.6792032807165,-1.,3.71816812842188));
#35042=CARTESIAN_POINT('Ctrl Pts',(1.67937685856627,-1.,3.72588753416339));
#35043=CARTESIAN_POINT('Ctrl Pts',(1.67951336376434,-1.,3.73361623282617));
#35044=CARTESIAN_POINT('Ctrl Pts',(1.67961298685316,-1.,3.74135385965622));
#35045=CARTESIAN_POINT('Ctrl Pts',(1.67967598599665,-1.,3.74910022394845));
#35046=CARTESIAN_POINT('Ctrl Pts',(1.67970265841379,-1.,3.75685523754816));
#35047=CARTESIAN_POINT('Ctrl Pts',(1.67969332319322,-1.,3.76461886684523));
#35048=CARTESIAN_POINT('Ctrl Pts',(1.67964830084946,-1.,3.77239107928394));
#35049=CARTESIAN_POINT('Ctrl Pts',(1.67956789211943,-1.,3.78017178196859));
#35050=CARTESIAN_POINT('Ctrl Pts',(1.67945236653175,-1.,3.78796080021026));
#35051=CARTESIAN_POINT('Ctrl Pts',(1.67930196625203,-1.,3.7957579157763));
#35052=CARTESIAN_POINT('Ctrl Pts',(1.67911690648128,-1.,3.80356289078481));
#35053=CARTESIAN_POINT('Ctrl Pts',(1.67889737738311,-1.,3.81137549624273));
#35054=CARTESIAN_POINT('Ctrl Pts',(1.67864354606363,-1.,3.81919554100522));
#35055=CARTESIAN_POINT('Ctrl Pts',(1.67835555760094,-1.,3.82702289288453));
#35056=CARTESIAN_POINT('Ctrl Pts',(1.67803353065273,-1.,3.83485746516115));
#35057=CARTESIAN_POINT('Ctrl Pts',(1.67774874946867,-1.,3.8411308598706));
#35058=CARTESIAN_POINT('Ctrl Pts',(1.67751991140661,-1.,3.84583912297567));
#35059=CARTESIAN_POINT('Ctrl Pts',(1.6773605765671,-1.,3.84897939431104));
#35060=CARTESIAN_POINT('Ctrl Pts',(1.67727921511438,-1.,3.85054988729471));
#35061=CARTESIAN_POINT('',(1.53673442965255,-1.,3.90876544355381));
#35062=CARTESIAN_POINT('',(1.67727921511438,-1.,3.85054988729471));
#35063=CARTESIAN_POINT('',(1.24526366418208,-1.,3.5372048861591));
#35064=CARTESIAN_POINT('Ctrl Pts',(1.53673442965255,-1.,3.90876544355381));
#35065=CARTESIAN_POINT('Ctrl Pts',(1.53556639217742,-1.,3.90771246854607));
#35066=CARTESIAN_POINT('Ctrl Pts',(1.53323321827311,-1.,3.90560462812846));
#35067=CARTESIAN_POINT('Ctrl Pts',(1.5297421605556,-1.,3.90243719629755));
#35068=CARTESIAN_POINT('Ctrl Pts',(1.52510482990784,-1.,3.8982026070607));
#35069=CARTESIAN_POINT('Ctrl Pts',(1.51933724328609,-1.,3.89289043531893));
#35070=CARTESIAN_POINT('Ctrl Pts',(1.51359883110181,-1.,3.88755930032927));
#35071=CARTESIAN_POINT('Ctrl Pts',(1.50788973857719,-1.,3.88220917950443));
#35072=CARTESIAN_POINT('Ctrl Pts',(1.50221016176766,-1.,3.87684006372665));
#35073=CARTESIAN_POINT('Ctrl Pts',(1.4965603539944,-1.,3.8714519699927));
#35074=CARTESIAN_POINT('Ctrl Pts',(1.49094061164604,-1.,3.86604492575933));
#35075=CARTESIAN_POINT('Ctrl Pts',(1.48535125510102,-1.,3.86061894706551));
#35076=CARTESIAN_POINT('Ctrl Pts',(1.47979260991063,-1.,3.85517401698952));
#35077=CARTESIAN_POINT('Ctrl Pts',(1.47426499018467,-1.,3.84971006847096));
#35078=CARTESIAN_POINT('Ctrl Pts',(1.46876867426374,-1.,3.84422695454469));
#35079=CARTESIAN_POINT('Ctrl Pts',(1.46330391180621,-1.,3.83872447159309));
#35080=CARTESIAN_POINT('Ctrl Pts',(1.45787095220763,-1.,3.83320241775199));
#35081=CARTESIAN_POINT('Ctrl Pts',(1.45247006796807,-1.,3.82766064519));
#35082=CARTESIAN_POINT('Ctrl Pts',(1.44710157648562,-1.,3.82209910620591));
#35083=CARTESIAN_POINT('Ctrl Pts',(1.441765870414,-1.,3.8165179239855));
#35084=CARTESIAN_POINT('Ctrl Pts',(1.43646341556783,-1.,3.81091737726965));
#35085=CARTESIAN_POINT('Ctrl Pts',(1.43119469921364,-1.,3.80529775429916));
#35086=CARTESIAN_POINT('Ctrl Pts',(1.42596018777301,-1.,3.79965923196365));
#35087=CARTESIAN_POINT('Ctrl Pts',(1.42076028482828,-1.,3.7940017574439));
#35088=CARTESIAN_POINT('Ctrl Pts',(1.41559527803808,-1.,3.78832489879369));
#35089=CARTESIAN_POINT('Ctrl Pts',(1.41046532282567,-1.,3.78262780065406));
#35090=CARTESIAN_POINT('Ctrl Pts',(1.40537056004702,-1.,3.77690952014209));
#35091=CARTESIAN_POINT('Ctrl Pts',(1.40031121335495,-1.,3.77116930621804));
#35092=CARTESIAN_POINT('Ctrl Pts',(1.39528769118054,-1.,3.76540689249078));
#35093=CARTESIAN_POINT('Ctrl Pts',(1.39030069388926,-1.,3.75962280650875));
#35094=CARTESIAN_POINT('Ctrl Pts',(1.38535129801185,-1.,3.75381861212728));
#35095=CARTESIAN_POINT('Ctrl Pts',(1.38044070763302,-1.,3.74799617204744));
#35096=CARTESIAN_POINT('Ctrl Pts',(1.3755700297169,-1.,3.7421569816256));
#35097=CARTESIAN_POINT('Ctrl Pts',(1.37074003422739,-1.,3.73630145885809));
#35098=CARTESIAN_POINT('Ctrl Pts',(1.36595093298674,-1.,3.73042829011293));
#35099=CARTESIAN_POINT('Ctrl Pts',(1.36120211416353,-1.,3.72453364678279));
#35100=CARTESIAN_POINT('Ctrl Pts',(1.35649266705038,-1.,3.71861271513318));
#35101=CARTESIAN_POINT('Ctrl Pts',(1.35182193384426,-1.,3.71266130563061));
#35102=CARTESIAN_POINT('Ctrl Pts',(1.34719008463535,-1.,3.7066775318825));
#35103=CARTESIAN_POINT('Ctrl Pts',(1.3425986075293,-1.,3.70066324015112));
#35104=CARTESIAN_POINT('Ctrl Pts',(1.33805103398214,-1.,3.69462613305692));
#35105=CARTESIAN_POINT('Ctrl Pts',(1.33355191034515,-1.,3.68857672413013));
#35106=CARTESIAN_POINT('Ctrl Pts',(1.32910547072734,-1.,3.68252441182534));
#35107=CARTESIAN_POINT('Ctrl Pts',(1.32471430856413,-1.,3.67647355257906));
#35108=CARTESIAN_POINT('Ctrl Pts',(1.3203782813777,-1.,3.67042021752668));
#35109=CARTESIAN_POINT('Ctrl Pts',(1.31609271239922,-1.,3.66434688899822));
#35110=CARTESIAN_POINT('Ctrl Pts',(1.31185038411231,-1.,3.65822827358655));
#35111=CARTESIAN_POINT('Ctrl Pts',(1.30764479590051,-1.,3.65204081987101));
#35112=CARTESIAN_POINT('Ctrl Pts',(1.30347327603778,-1.,3.64577181380125));
#35113=CARTESIAN_POINT('Ctrl Pts',(1.29933955906463,-1.,3.6394268987279));
#35114=CARTESIAN_POINT('Ctrl Pts',(1.29525810207744,-1.,3.63304271630995));
#35115=CARTESIAN_POINT('Ctrl Pts',(1.29125046021853,-1.,3.62667616004299));
#35116=CARTESIAN_POINT('Ctrl Pts',(1.2873375502936,-1.,3.62038148492295));
#35117=CARTESIAN_POINT('Ctrl Pts',(1.28353255117754,-1.,3.61418935913793));
#35118=CARTESIAN_POINT('Ctrl Pts',(1.27983492861703,-1.,3.60808907746372));
#35119=CARTESIAN_POINT('Ctrl Pts',(1.27622049908664,-1.,3.60199947736404));
#35120=CARTESIAN_POINT('Ctrl Pts',(1.27264798379365,-1.,3.59578698050164));
#35121=CARTESIAN_POINT('Ctrl Pts',(1.26907758484766,-1.,3.5893180784647));
#35122=CARTESIAN_POINT('Ctrl Pts',(1.26548706249891,-1.,3.58250452868699));
#35123=CARTESIAN_POINT('Ctrl Pts',(1.26188667142784,-1.,3.5753456065164));
#35124=CARTESIAN_POINT('Ctrl Pts',(1.25834000485626,-1.,3.56798645995025));
#35125=CARTESIAN_POINT('Ctrl Pts',(1.25496090899873,-1.,3.56071094990825));
#35126=CARTESIAN_POINT('Ctrl Pts',(1.25188792940508,-1.,3.5538728741862));
#35127=CARTESIAN_POINT('Ctrl Pts',(1.24926408627938,-1.,3.54784190282889));
#35128=CARTESIAN_POINT('Ctrl Pts',(1.2472164623202,-1.,3.54294877426113));
#35129=CARTESIAN_POINT('Ctrl Pts',(1.24593497225964,-1.,3.53968291129942));
#35130=CARTESIAN_POINT('Ctrl Pts',(1.2453920538873,-1.,3.53808746578052));
#35131=CARTESIAN_POINT('Ctrl Pts',(1.24524498991133,-1.,3.53744859265385));
#35132=CARTESIAN_POINT('Ctrl Pts',(1.24524838931864,-1.,3.53725139174402));
#35133=CARTESIAN_POINT('Ctrl Pts',(1.24526366418208,-1.,3.5372048861591));
#35134=CARTESIAN_POINT('',(1.071677399622,-1.,3.59360648251021));
#35135=CARTESIAN_POINT('Origin',(0.,-1.,0.));
#35136=CARTESIAN_POINT('',(1.05427041296137,-1.,4.06552750530042));
#35137=CARTESIAN_POINT('Ctrl Pts',(1.071677399622,-1.,3.59360648251021));
#35138=CARTESIAN_POINT('Ctrl Pts',(1.07171709254271,-1.,3.59363512797985));
#35139=CARTESIAN_POINT('Ctrl Pts',(1.07183575450716,-1.,3.59379266874663));
#35140=CARTESIAN_POINT('Ctrl Pts',(1.07209229745284,-1.,3.59439597));
#35141=CARTESIAN_POINT('Ctrl Pts',(1.07259084660947,-1.,3.59600583195037));
#35142=CARTESIAN_POINT('Ctrl Pts',(1.0734737254567,-1.,3.59940121154383));
#35143=CARTESIAN_POINT('Ctrl Pts',(1.0746932716863,-1.,3.6045633988796));
#35144=CARTESIAN_POINT('Ctrl Pts',(1.07611545402841,-1.,3.61098481349577));
#35145=CARTESIAN_POINT('Ctrl Pts',(1.07764868137729,-1.,3.61832318504957));
#35146=CARTESIAN_POINT('Ctrl Pts',(1.07919137290815,-1.,3.62619537902616));
#35147=CARTESIAN_POINT('Ctrl Pts',(1.08064765719887,-1.,3.63423373196602));
#35148=CARTESIAN_POINT('Ctrl Pts',(1.08194278850972,-1.,3.64214167843595));
#35149=CARTESIAN_POINT('Ctrl Pts',(1.08304289898577,-1.,3.64976441208197));
#35150=CARTESIAN_POINT('Ctrl Pts',(1.08395671077761,-1.,3.65709649161004));
#35151=CARTESIAN_POINT('Ctrl Pts',(1.0847180992287,-1.,3.66422237895256));
#35152=CARTESIAN_POINT('Ctrl Pts',(1.0853733414448,-1.,3.67127347729632));
#35153=CARTESIAN_POINT('Ctrl Pts',(1.08596755755768,-1.,3.67838211685148));
#35154=CARTESIAN_POINT('Ctrl Pts',(1.08652888882609,-1.,3.68562817420864));
#35155=CARTESIAN_POINT('Ctrl Pts',(1.08706319540291,-1.,3.69302062410229));
#35156=CARTESIAN_POINT('Ctrl Pts',(1.08756311291324,-1.,3.70052690909884));
#35157=CARTESIAN_POINT('Ctrl Pts',(1.0880136731219,-1.,3.70809084139476));
#35158=CARTESIAN_POINT('Ctrl Pts',(1.08839887334776,-1.,3.71565372339063));
#35159=CARTESIAN_POINT('Ctrl Pts',(1.08870887220072,-1.,3.72317741369364));
#35160=CARTESIAN_POINT('Ctrl Pts',(1.08894337390925,-1.,3.73065515162949));
#35161=CARTESIAN_POINT('Ctrl Pts',(1.08910769013288,-1.,3.73809879348209));
#35162=CARTESIAN_POINT('Ctrl Pts',(1.08921040494013,-1.,3.74553121371745));
#35163=CARTESIAN_POINT('Ctrl Pts',(1.08926054632927,-1.,3.75297711748138));
#35164=CARTESIAN_POINT('Ctrl Pts',(1.08926462734287,-1.,3.76045342580226));
#35165=CARTESIAN_POINT('Ctrl Pts',(1.08922484204263,-1.,3.76796340094469));
#35166=CARTESIAN_POINT('Ctrl Pts',(1.08914072791275,-1.,3.7755019940944));
#35167=CARTESIAN_POINT('Ctrl Pts',(1.08901018614638,-1.,3.78305911299511));
#35168=CARTESIAN_POINT('Ctrl Pts',(1.08883071512097,-1.,3.79062357974401));
#35169=CARTESIAN_POINT('Ctrl Pts',(1.08860064435775,-1.,3.79818708705252));
#35170=CARTESIAN_POINT('Ctrl Pts',(1.08832009255378,-1.,3.80574726657656));
#35171=CARTESIAN_POINT('Ctrl Pts',(1.08799030610861,-1.,3.81330554446324));
#35172=CARTESIAN_POINT('Ctrl Pts',(1.08761321539442,-1.,3.82086569676321));
#35173=CARTESIAN_POINT('Ctrl Pts',(1.08719091307558,-1.,3.82843215316985));
#35174=CARTESIAN_POINT('Ctrl Pts',(1.08672515456901,-1.,3.83600837071702));
#35175=CARTESIAN_POINT('Ctrl Pts',(1.08621688337601,-1.,3.84359528764934));
#35176=CARTESIAN_POINT('Ctrl Pts',(1.08566647671838,-1.,3.85119211322732));
#35177=CARTESIAN_POINT('Ctrl Pts',(1.08507395120054,-1.,3.85879698702511));
#35178=CARTESIAN_POINT('Ctrl Pts',(1.08443918607926,-1.,3.86640769434269));
#35179=CARTESIAN_POINT('Ctrl Pts',(1.0837621330751,-1.,3.87402233722563));
#35180=CARTESIAN_POINT('Ctrl Pts',(1.08304304871042,-1.,3.88164007721365));
#35181=CARTESIAN_POINT('Ctrl Pts',(1.08228241999363,-1.,3.88926088975182));
#35182=CARTESIAN_POINT('Ctrl Pts',(1.08148086931373,-1.,3.89688525098408));
#35183=CARTESIAN_POINT('Ctrl Pts',(1.08063906483822,-1.,3.90451384092564));
#35184=CARTESIAN_POINT('Ctrl Pts',(1.0797576350746,-1.,3.91214726022096));
#35185=CARTESIAN_POINT('Ctrl Pts',(1.07883706663524,-1.,3.91978568924062));
#35186=CARTESIAN_POINT('Ctrl Pts',(1.07787771707155,-1.,3.92742893349684));
#35187=CARTESIAN_POINT('Ctrl Pts',(1.07687985975348,-1.,3.93507657572743));
#35188=CARTESIAN_POINT('Ctrl Pts',(1.07584371946428,-1.,3.94272809633271));
#35189=CARTESIAN_POINT('Ctrl Pts',(1.07476950921607,-1.,3.95038299600754));
#35190=CARTESIAN_POINT('Ctrl Pts',(1.07365747426551,-1.,3.95804094429606));
#35191=CARTESIAN_POINT('Ctrl Pts',(1.07250789943095,-1.,3.96570179322681));
#35192=CARTESIAN_POINT('Ctrl Pts',(1.07132109206252,-1.,3.97336550222571));
#35193=CARTESIAN_POINT('Ctrl Pts',(1.07009737257815,-1.,3.98103208801289));
#35194=CARTESIAN_POINT('Ctrl Pts',(1.06883706263912,-1.,3.98870156857298));
#35195=CARTESIAN_POINT('Ctrl Pts',(1.06754047381188,-1.,3.99637389919958));
#35196=CARTESIAN_POINT('Ctrl Pts',(1.06620789963406,-1.,4.00404894951804));
#35197=CARTESIAN_POINT('Ctrl Pts',(1.06483961342894,-1.,4.0117265418656));
#35198=CARTESIAN_POINT('Ctrl Pts',(1.06343586496094,-1.,4.0194064749539));
#35199=CARTESIAN_POINT('Ctrl Pts',(1.06199687787488,-1.,4.02708855235732));
#35200=CARTESIAN_POINT('Ctrl Pts',(1.06052284712114,-1.,4.03477261142549));
#35201=CARTESIAN_POINT('Ctrl Pts',(1.05901393667039,-1.,4.04245854429333));
#35202=CARTESIAN_POINT('Ctrl Pts',(1.05747027728537,-1.,4.05014628387112));
#35203=CARTESIAN_POINT('Ctrl Pts',(1.0562076270849,-1.,4.05629789308941));
#35204=CARTESIAN_POINT('Ctrl Pts',(1.05524507177901,-1.,4.06091239150293));
#35205=CARTESIAN_POINT('Ctrl Pts',(1.05459645194934,-1.,4.06398907542679));
#35206=CARTESIAN_POINT('Ctrl Pts',(1.05427041296137,-1.,4.06552750530042));
#35207=CARTESIAN_POINT('',(0.906349047628865,-1.,4.10104028313088));
#35208=CARTESIAN_POINT('',(1.05427041296137,-1.,4.06552750530042));
#35209=CARTESIAN_POINT('',(0.676591647975428,-1.,3.68845817949586));
#35210=CARTESIAN_POINT('Ctrl Pts',(0.906349047628865,-1.,4.10104028313088));
#35211=CARTESIAN_POINT('Ctrl Pts',(0.905360112215337,-1.,4.09981755067523));
#35212=CARTESIAN_POINT('Ctrl Pts',(0.903385402441587,-1.,4.09737067245935));
#35213=CARTESIAN_POINT('Ctrl Pts',(0.900432820941674,-1.,4.09369611522387));
#35214=CARTESIAN_POINT('Ctrl Pts',(0.896515019231333,-1.,4.08878822246833));
#35215=CARTESIAN_POINT('Ctrl Pts',(0.891649447916277,-1.,4.08263920304799));
#35216=CARTESIAN_POINT('Ctrl Pts',(0.886815658358501,-1.,4.07647601773635));
#35217=CARTESIAN_POINT('Ctrl Pts',(0.882013797525691,-1.,4.07029866694192));
#35218=CARTESIAN_POINT('Ctrl Pts',(0.877244060485837,-1.,4.06410717232905));
#35219=CARTESIAN_POINT('Ctrl Pts',(0.872506694782446,-1.,4.0579015903134));
#35220=CARTESIAN_POINT('Ctrl Pts',(0.867801988859917,-1.,4.05168199437909));
#35221=CARTESIAN_POINT('Ctrl Pts',(0.863130256643258,-1.,4.04544845048584));
#35222=CARTESIAN_POINT('Ctrl Pts',(0.858491822322827,-1.,4.03920099284773));
#35223=CARTESIAN_POINT('Ctrl Pts',(0.853887006631755,-1.,4.03293960436756));
#35224=CARTESIAN_POINT('Ctrl Pts',(0.849316107474244,-1.,4.02666418343164));
#35225=CARTESIAN_POINT('Ctrl Pts',(0.844779403287745,-1.,4.02037456798441));
#35226=CARTESIAN_POINT('Ctrl Pts',(0.840277171975854,-1.,4.01407059766103));
#35227=CARTESIAN_POINT('Ctrl Pts',(0.835809705809645,-1.,4.00775216907856));
#35228=CARTESIAN_POINT('Ctrl Pts',(0.831377325741622,-1.,4.00141928477507));
#35229=CARTESIAN_POINT('Ctrl Pts',(0.826980400320789,-1.,3.99507212784431));
#35230=CARTESIAN_POINT('Ctrl Pts',(0.822619346022118,-1.,3.98871104646485));
#35231=CARTESIAN_POINT('Ctrl Pts',(0.818294599022293,-1.,3.98233640155404));
#35232=CARTESIAN_POINT('Ctrl Pts',(0.814006592328843,-1.,3.97594844078811));
#35233=CARTESIAN_POINT('Ctrl Pts',(0.80975573281809,-1.,3.96954717513232));
#35234=CARTESIAN_POINT('Ctrl Pts',(0.805542372178361,-1.,3.96313222295815));
#35235=CARTESIAN_POINT('Ctrl Pts',(0.801366797727049,-1.,3.95670276375108));
#35236=CARTESIAN_POINT('Ctrl Pts',(0.797229296085315,-1.,3.95025788827136));
#35237=CARTESIAN_POINT('Ctrl Pts',(0.79313020564096,-1.,3.94379688971283));
#35238=CARTESIAN_POINT('Ctrl Pts',(0.789069971469332,-1.,3.93731956885676));
#35239=CARTESIAN_POINT('Ctrl Pts',(0.785049202786507,-1.,3.93082655631789));
#35240=CARTESIAN_POINT('Ctrl Pts',(0.781068718228451,-1.,3.92431956510441));
#35241=CARTESIAN_POINT('Ctrl Pts',(0.777129415664956,-1.,3.9178006233448));
#35242=CARTESIAN_POINT('Ctrl Pts',(0.77323215450632,-1.,3.91127138115243));
#35243=CARTESIAN_POINT('Ctrl Pts',(0.769377629847873,-1.,3.90473237182633));
#35244=CARTESIAN_POINT('Ctrl Pts',(0.765566256401295,-1.,3.89818233104378));
#35245=CARTESIAN_POINT('Ctrl Pts',(0.761798028793969,-1.,3.89161738162245));
#35246=CARTESIAN_POINT('Ctrl Pts',(0.758072800564801,-1.,3.88503262662689));
#35247=CARTESIAN_POINT('Ctrl Pts',(0.754390577396856,-1.,3.87842382520065));
#35248=CARTESIAN_POINT('Ctrl Pts',(0.750751822383027,-1.,3.87178914078374));
#35249=CARTESIAN_POINT('Ctrl Pts',(0.747157716488871,-1.,3.86513062969889));
#35250=CARTESIAN_POINT('Ctrl Pts',(0.743610542737012,-1.,3.85845645217594));
#35251=CARTESIAN_POINT('Ctrl Pts',(0.740113146827137,-1.,3.85177770351216));
#35252=CARTESIAN_POINT('Ctrl Pts',(0.736668240497117,-1.,3.84510432881213));
#35253=CARTESIAN_POINT('Ctrl Pts',(0.733277703756078,-1.,3.83844103658009));
#35254=CARTESIAN_POINT('Ctrl Pts',(0.729942010490167,-1.,3.83178392403383));
#35255=CARTESIAN_POINT('Ctrl Pts',(0.726659281876663,-1.,3.82511495756713));
#35256=CARTESIAN_POINT('Ctrl Pts',(0.723426346019422,-1.,3.81840802610835));
#35257=CARTESIAN_POINT('Ctrl Pts',(0.720240466589236,-1.,3.81163885127344));
#35258=CARTESIAN_POINT('Ctrl Pts',(0.717100993669114,-1.,3.80479445759309));
#35259=CARTESIAN_POINT('Ctrl Pts',(0.71401073300664,-1.,3.79788100314975));
#35260=CARTESIAN_POINT('Ctrl Pts',(0.710978231689016,-1.,3.79093694007094));
#35261=CARTESIAN_POINT('Ctrl Pts',(0.708015879375459,-1.,3.78402183336605));
#35262=CARTESIAN_POINT('Ctrl Pts',(0.705135847999816,-1.,3.77719254217129));
#35263=CARTESIAN_POINT('Ctrl Pts',(0.702346356621551,-1.,3.77048141872872));
#35264=CARTESIAN_POINT('Ctrl Pts',(0.699648552230917,-1.,3.76387780603759));
#35265=CARTESIAN_POINT('Ctrl Pts',(0.697031245659743,-1.,3.75729775767023));
#35266=CARTESIAN_POINT('Ctrl Pts',(0.694474562581492,-1.,3.75060288243455));
#35267=CARTESIAN_POINT('Ctrl Pts',(0.69196008040082,-1.,3.74365508986712));
#35268=CARTESIAN_POINT('Ctrl Pts',(0.689479637354813,-1.,3.73636374475077));
#35269=CARTESIAN_POINT('Ctrl Pts',(0.687043475232354,-1.,3.72872973554051));
#35270=CARTESIAN_POINT('Ctrl Pts',(0.684691698167848,-1.,3.7209063713926));
#35271=CARTESIAN_POINT('Ctrl Pts',(0.682492345108929,-1.,3.71319182789943));
#35272=CARTESIAN_POINT('Ctrl Pts',(0.680526909710876,-1.,3.70595722031785));
#35273=CARTESIAN_POINT('Ctrl Pts',(0.678878822226026,-1.,3.69959004073005));
#35274=CARTESIAN_POINT('Ctrl Pts',(0.677621861865497,-1.,3.69443683573598));
#35275=CARTESIAN_POINT('Ctrl Pts',(0.676867042599401,-1.,3.69101071175464));
#35276=CARTESIAN_POINT('Ctrl Pts',(0.676580391119396,-1.,3.68934997767243));
#35277=CARTESIAN_POINT('Ctrl Pts',(0.676535079520806,-1.,3.68869596425969));
#35278=CARTESIAN_POINT('Ctrl Pts',(0.676569286094606,-1.,3.68850172300477));
#35279=CARTESIAN_POINT('Ctrl Pts',(0.676591647975428,-1.,3.68845817949586));
#35280=CARTESIAN_POINT('',(0.496319364829373,-1.,3.71701050416802));
#35281=CARTESIAN_POINT('Origin',(0.,-1.,0.));
#35282=CARTESIAN_POINT('',(0.405301974318349,-1.,4.18039834341342));
#35283=CARTESIAN_POINT('Ctrl Pts',(0.496319364829373,-1.,3.71701050416802));
#35284=CARTESIAN_POINT('Ctrl Pts',(0.496354087925645,-1.,3.71704500630521));
#35285=CARTESIAN_POINT('Ctrl Pts',(0.496446644158827,-1.,3.71721917030465));
#35286=CARTESIAN_POINT('Ctrl Pts',(0.496605651526313,-1.,3.71785517607694));
#35287=CARTESIAN_POINT('Ctrl Pts',(0.496846224822534,-1.,3.7195232082259));
#35288=CARTESIAN_POINT('Ctrl Pts',(0.497187079575794,-1.,3.72301489774241));
#35289=CARTESIAN_POINT('Ctrl Pts',(0.497584067153279,-1.,3.72830430904794));
#35290=CARTESIAN_POINT('Ctrl Pts',(0.497984209510495,-1.,3.73486914372834));
#35291=CARTESIAN_POINT('Ctrl Pts',(0.498350586058176,-1.,3.74235701735109));
#35292=CARTESIAN_POINT('Ctrl Pts',(0.498642802042929,-1.,3.75037362168103));
#35293=CARTESIAN_POINT('Ctrl Pts',(0.498823681615513,-1.,3.75854082221127));
#35294=CARTESIAN_POINT('Ctrl Pts',(0.498865792335185,-1.,3.76655401191144));
#35295=CARTESIAN_POINT('Ctrl Pts',(0.498759900365686,-1.,3.77425499225089));
#35296=CARTESIAN_POINT('Ctrl Pts',(0.498515471679378,-1.,3.78163975337189));
#35297=CARTESIAN_POINT('Ctrl Pts',(0.498152751800819,-1.,3.78879701661152));
#35298=CARTESIAN_POINT('Ctrl Pts',(0.49769689210058,-1.,3.79586380669959));
#35299=CARTESIAN_POINT('Ctrl Pts',(0.49717175620109,-1.,3.80297788298545));
#35300=CARTESIAN_POINT('Ctrl Pts',(0.496592643443789,-1.,3.81022254090909));
#35301=CARTESIAN_POINT('Ctrl Pts',(0.495963937875571,-1.,3.81760756144099));
#35302=CARTESIAN_POINT('Ctrl Pts',(0.495283458893903,-1.,3.82509963594156));
#35303=CARTESIAN_POINT('Ctrl Pts',(0.494545212256425,-1.,3.8326409268245));
#35304=CARTESIAN_POINT('Ctrl Pts',(0.493742574629117,-1.,3.84017095578438));
#35305=CARTESIAN_POINT('Ctrl Pts',(0.492871792414095,-1.,3.84765051147965));
#35306=CARTESIAN_POINT('Ctrl Pts',(0.49193363108376,-1.,3.85507287020223));
#35307=CARTESIAN_POINT('Ctrl Pts',(0.490931482170849,-1.,3.86245057319215));
#35308=CARTESIAN_POINT('Ctrl Pts',(0.489870245704899,-1.,3.86980755613694));
#35309=CARTESIAN_POINT('Ctrl Pts',(0.488754973798281,-1.,3.87716963231115));
#35310=CARTESIAN_POINT('Ctrl Pts',(0.487589452275179,-1.,3.88455453328156));
#35311=CARTESIAN_POINT('Ctrl Pts',(0.486375337854133,-1.,3.89196582437574));
#35312=CARTESIAN_POINT('Ctrl Pts',(0.485112963522245,-1.,3.89939844658529));
#35313=CARTESIAN_POINT('Ctrl Pts',(0.48380183508916,-1.,3.90684210358063));
#35314=CARTESIAN_POINT('Ctrl Pts',(0.482441230340708,-1.,3.91428536373749));
#35315=CARTESIAN_POINT('Ctrl Pts',(0.481030798910735,-1.,3.92171976072334));
#35316=CARTESIAN_POINT('Ctrl Pts',(0.479571028525565,-1.,3.92914297392067));
#35317=CARTESIAN_POINT('Ctrl Pts',(0.478062927140957,-1.,3.93655660689819));
#35318=CARTESIAN_POINT('Ctrl Pts',(0.476507810658534,-1.,3.94396469119385));
#35319=CARTESIAN_POINT('Ctrl Pts',(0.47490705302179,-1.,3.95137192932898));
#35320=CARTESIAN_POINT('Ctrl Pts',(0.473261847236295,-1.,3.95878201038332));
#35321=CARTESIAN_POINT('Ctrl Pts',(0.471572978413493,-1.,3.96619600864626));
#35322=CARTESIAN_POINT('Ctrl Pts',(0.469840942829878,-1.,3.97361320212413));
#35323=CARTESIAN_POINT('Ctrl Pts',(0.468066047920139,-1.,3.98103175589349));
#35324=CARTESIAN_POINT('Ctrl Pts',(0.466248520883034,-1.,3.98844946363258));
#35325=CARTESIAN_POINT('Ctrl Pts',(0.464388610938994,-1.,3.99586444320135));
#35326=CARTESIAN_POINT('Ctrl Pts',(0.462486702616251,-1.,4.00327590659129));
#35327=CARTESIAN_POINT('Ctrl Pts',(0.460543280768577,-1.,4.01068390573469));
#35328=CARTESIAN_POINT('Ctrl Pts',(0.458558885637,-1.,4.01808900827647));
#35329=CARTESIAN_POINT('Ctrl Pts',(0.456534070784968,-1.,4.02549199038414));
#35330=CARTESIAN_POINT('Ctrl Pts',(0.454469363020495,-1.,4.03289354362745));
#35331=CARTESIAN_POINT('Ctrl Pts',(0.452365214748778,-1.,4.0402939222793));
#35332=CARTESIAN_POINT('Ctrl Pts',(0.450222009543773,-1.,4.0476929901797));
#35333=CARTESIAN_POINT('Ctrl Pts',(0.448040082683976,-1.,4.05509037796815));
#35334=CARTESIAN_POINT('Ctrl Pts',(0.445819737468477,-1.,4.06248560760596));
#35335=CARTESIAN_POINT('Ctrl Pts',(0.443561262395407,-1.,4.0698782192577));
#35336=CARTESIAN_POINT('Ctrl Pts',(0.441264951396587,-1.,4.07726792490256));
#35337=CARTESIAN_POINT('Ctrl Pts',(0.438931108931613,-1.,4.08465462294625));
#35338=CARTESIAN_POINT('Ctrl Pts',(0.436560044913814,-1.,4.09203832139439));
#35339=CARTESIAN_POINT('Ctrl Pts',(0.434152073200642,-1.,4.09941908688567));
#35340=CARTESIAN_POINT('Ctrl Pts',(0.431707508679771,-1.,4.10679698750219));
#35341=CARTESIAN_POINT('Ctrl Pts',(0.429226666075372,-1.,4.1141720278277));
#35342=CARTESIAN_POINT('Ctrl Pts',(0.426709855706242,-1.,4.1215441250121));
#35343=CARTESIAN_POINT('Ctrl Pts',(0.424157375323155,-1.,4.1289131463371));
#35344=CARTESIAN_POINT('Ctrl Pts',(0.421569503103971,-1.,4.13627893206433));
#35345=CARTESIAN_POINT('Ctrl Pts',(0.418946490667799,-1.,4.14364132317223));
#35346=CARTESIAN_POINT('Ctrl Pts',(0.416288556008986,-1.,4.15100018950989));
#35347=CARTESIAN_POINT('Ctrl Pts',(0.413595877953268,-1.,4.1583554501909));
#35348=CARTESIAN_POINT('Ctrl Pts',(0.410868596148613,-1.,4.16570705940731));
#35349=CARTESIAN_POINT('Ctrl Pts',(0.408659167570152,-1.,4.17158541009947));
#35350=CARTESIAN_POINT('Ctrl Pts',(0.406986596326602,-1.,4.17599251955585));
#35351=CARTESIAN_POINT('Ctrl Pts',(0.40586466267963,-1.,4.17892985789908));
#35352=CARTESIAN_POINT('Ctrl Pts',(0.405301974318349,-1.,4.18039834341342));
#35353=CARTESIAN_POINT('',(0.253646344052521,-1.,4.1923339003649));
#35354=CARTESIAN_POINT('',(0.405301974318349,-1.,4.18039834341342));
#35355=CARTESIAN_POINT('',(0.091259699916682,-1.,3.74888939116255));
#35356=CARTESIAN_POINT('Ctrl Pts',(0.253646344052521,-1.,4.1923339003649));
#35357=CARTESIAN_POINT('Ctrl Pts',(0.252860861572565,-1.,4.19097151819241));
#35358=CARTESIAN_POINT('Ctrl Pts',(0.251293239837692,-1.,4.18824585244066));
#35359=CARTESIAN_POINT('Ctrl Pts',(0.248951836910963,-1.,4.18415464959491));
#35360=CARTESIAN_POINT('Ctrl Pts',(0.245850033418583,-1.,4.17869430192868));
#35361=CARTESIAN_POINT('Ctrl Pts',(0.242006283923911,-1.,4.17185984409533));
#35362=CARTESIAN_POINT('Ctrl Pts',(0.238196140933976,-1.,4.1650163665385));
#35363=CARTESIAN_POINT('Ctrl Pts',(0.234419749543142,-1.,4.1581638926525));
#35364=CARTESIAN_POINT('Ctrl Pts',(0.230677299028737,-1.,4.15130247435029));
#35365=CARTESIAN_POINT('Ctrl Pts',(0.226969025061243,-1.,4.14443220607733));
#35366=CARTESIAN_POINT('Ctrl Pts',(0.223295201038383,-1.,4.13755320553563));
#35367=CARTESIAN_POINT('Ctrl Pts',(0.219656126701851,-1.,4.13066558698156));
#35368=CARTESIAN_POINT('Ctrl Pts',(0.216052116898424,-1.,4.12376943492249));
#35369=CARTESIAN_POINT('Ctrl Pts',(0.212483491087067,-1.,4.11686478264545));
#35370=CARTESIAN_POINT('Ctrl Pts',(0.208950559400171,-1.,4.10995157639026));
#35371=CARTESIAN_POINT('Ctrl Pts',(0.205453622198233,-1.,4.10302969965374));
#35372=CARTESIAN_POINT('Ctrl Pts',(0.201992979049984,-1.,4.09609903751912));
#35373=CARTESIAN_POINT('Ctrl Pts',(0.19856893480081,-1.,4.08915953359753));
#35374=CARTESIAN_POINT('Ctrl Pts',(0.195181806054714,-1.,4.08221124060385));
#35375=CARTESIAN_POINT('Ctrl Pts',(0.191831928181081,-1.,4.07525439703137));
#35376=CARTESIAN_POINT('Ctrl Pts',(0.188519658060255,-1.,4.06828941192308));
#35377=CARTESIAN_POINT('Ctrl Pts',(0.185245370038947,-1.,4.06131670998589));
#35378=CARTESIAN_POINT('Ctrl Pts',(0.18200945304855,-1.,4.05433660358402));
#35379=CARTESIAN_POINT('Ctrl Pts',(0.178812307240715,-1.,4.04734916719722));
#35380=CARTESIAN_POINT('Ctrl Pts',(0.175654339673757,-1.,4.04035407891161));
#35381=CARTESIAN_POINT('Ctrl Pts',(0.172535962484466,-1.,4.03335057326093));
#35382=CARTESIAN_POINT('Ctrl Pts',(0.169457601001653,-1.,4.0263377970371));
#35383=CARTESIAN_POINT('Ctrl Pts',(0.166419700015847,-1.,4.01931510507143));
#35384=CARTESIAN_POINT('Ctrl Pts',(0.163422730287458,-1.,4.01228237022301));
#35385=CARTESIAN_POINT('Ctrl Pts',(0.160467194882218,-1.,4.00524031064509));
#35386=CARTESIAN_POINT('Ctrl Pts',(0.157553634383809,-1.,3.99819074631874));
#35387=CARTESIAN_POINT('Ctrl Pts',(0.154682618338563,-1.,3.99113582086059));
#35388=CARTESIAN_POINT('Ctrl Pts',(0.151854737441405,-1.,3.9840772985098));
#35389=CARTESIAN_POINT('Ctrl Pts',(0.149070594803543,-1.,3.97701581473643));
#35390=CARTESIAN_POINT('Ctrl Pts',(0.146330797814513,-1.,3.96995018565891));
#35391=CARTESIAN_POINT('Ctrl Pts',(0.143635947692791,-1.,3.96287658098896));
#35392=CARTESIAN_POINT('Ctrl Pts',(0.140986665829936,-1.,3.95579014116899));
#35393=CARTESIAN_POINT('Ctrl Pts',(0.138383621255159,-1.,3.94868667844355));
#35394=CARTESIAN_POINT('Ctrl Pts',(0.135827558661187,-1.,3.94156445130744));
#35395=CARTESIAN_POINT('Ctrl Pts',(0.133319322794189,-1.,3.93442567551035));
#35396=CARTESIAN_POINT('Ctrl Pts',(0.130859892027798,-1.,3.9272787679596));
#35397=CARTESIAN_POINT('Ctrl Pts',(0.128450341339527,-1.,3.92013513251642));
#35398=CARTESIAN_POINT('Ctrl Pts',(0.126091793324136,-1.,3.91300501605392));
#35399=CARTESIAN_POINT('Ctrl Pts',(0.123785368272377,-1.,3.90589336320508));
#35400=CARTESIAN_POINT('Ctrl Pts',(0.121532144765723,-1.,3.89879639336952));
#35401=CARTESIAN_POINT('Ctrl Pts',(0.119333088190417,-1.,3.89169600105201));
#35402=CARTESIAN_POINT('Ctrl Pts',(0.117189150373144,-1.,3.88456590045767));
#35403=CARTESIAN_POINT('Ctrl Pts',(0.115101426649469,-1.,3.87738168405343));
#35404=CARTESIAN_POINT('Ctrl Pts',(0.113071304914561,-1.,3.87013043445014));
#35405=CARTESIAN_POINT('Ctrl Pts',(0.11110059303626,-1.,3.86281867282965));
#35406=CARTESIAN_POINT('Ctrl Pts',(0.109191717634943,-1.,3.855485714969));
#35407=CARTESIAN_POINT('Ctrl Pts',(0.107347597812183,-1.,3.84819233070317));
#35408=CARTESIAN_POINT('Ctrl Pts',(0.105571360916569,-1.,3.84099658324803));
#35409=CARTESIAN_POINT('Ctrl Pts',(0.103866063811622,-1.,3.83393171228002));
#35410=CARTESIAN_POINT('Ctrl Pts',(0.102234506488456,-1.,3.82698737143255));
#35411=CARTESIAN_POINT('Ctrl Pts',(0.100678769650632,-1.,3.82007889742625));
#35412=CARTESIAN_POINT('Ctrl Pts',(0.0992008728096511,-1.,3.81306649386461));
#35413=CARTESIAN_POINT('Ctrl Pts',(0.097804222290664,-1.,3.80581088847809));
#35414=CARTESIAN_POINT('Ctrl Pts',(0.0964949352873128,-1.,3.79822128513845));
#35415=CARTESIAN_POINT('Ctrl Pts',(0.0952829885100798,-1.,3.79030016353111));
#35416=CARTESIAN_POINT('Ctrl Pts',(0.0941840095090811,-1.,3.782205218991));
#35417=CARTESIAN_POINT('Ctrl Pts',(0.0932185546203175,-1.,3.77424159971059));
#35418=CARTESIAN_POINT('Ctrl Pts',(0.0924090589602688,-1.,3.76678860031841));
#35419=CARTESIAN_POINT('Ctrl Pts',(0.0917773084998332,-1.,3.76024199359303));
#35420=CARTESIAN_POINT('Ctrl Pts',(0.0913419622736395,-1.,3.75495560118212));
#35421=CARTESIAN_POINT('Ctrl Pts',(0.0911323999574423,-1.,3.75145357872422));
#35422=CARTESIAN_POINT('Ctrl Pts',(0.0911090736805507,-1.,3.74976844886346));
#35423=CARTESIAN_POINT('Ctrl Pts',(0.0911666301812815,-1.,3.74911539914542));
#35424=CARTESIAN_POINT('Ctrl Pts',(0.0912308016421979,-1.,3.74892890040975));
#35425=CARTESIAN_POINT('Ctrl Pts',(0.091259699916682,-1.,3.74888939116255));
#35426=CARTESIAN_POINT('',(-0.091259699914886,-1.,3.74888939116259));
#35427=CARTESIAN_POINT('Origin',(0.,-1.,0.));
#35428=CARTESIAN_POINT('',(-0.253646344052522,-1.,4.1923339003649));
#35429=CARTESIAN_POINT('Ctrl Pts',(-0.091259699914886,-1.,3.74888939116259));
#35430=CARTESIAN_POINT('Ctrl Pts',(-0.0912308016409234,-1.,3.74892890041021));
#35431=CARTESIAN_POINT('Ctrl Pts',(-0.0911666301806427,-1.,3.74911539914664));
#35432=CARTESIAN_POINT('Ctrl Pts',(-0.0911090736804572,-1.,3.74976844886495));
#35433=CARTESIAN_POINT('Ctrl Pts',(-0.0911323999576145,-1.,3.75145357872511));
#35434=CARTESIAN_POINT('Ctrl Pts',(-0.0913419622735854,-1.,3.75495560118053));
#35435=CARTESIAN_POINT('Ctrl Pts',(-0.091777308499901,-1.,3.76024199359493));
#35436=CARTESIAN_POINT('Ctrl Pts',(-0.0924090589604057,-1.,3.76678860032228));
#35437=CARTESIAN_POINT('Ctrl Pts',(-0.0932185546204576,-1.,3.77424159971456));
#35438=CARTESIAN_POINT('Ctrl Pts',(-0.0941840095091746,-1.,3.78220521899366));
#35439=CARTESIAN_POINT('Ctrl Pts',(-0.095282988510107,-1.,3.79030016353186));
#35440=CARTESIAN_POINT('Ctrl Pts',(-0.0964949352872846,-1.,3.7982212851376));
#35441=CARTESIAN_POINT('Ctrl Pts',(-0.0978042222906077,-1.,3.80581088847642));
#35442=CARTESIAN_POINT('Ctrl Pts',(-0.0992008728095946,-1.,3.81306649386293));
#35443=CARTESIAN_POINT('Ctrl Pts',(-0.100678769650594,-1.,3.82007889742512));
#35444=CARTESIAN_POINT('Ctrl Pts',(-0.102234506488445,-1.,3.8269873714322));
#35445=CARTESIAN_POINT('Ctrl Pts',(-0.103866063811634,-1.,3.83393171228034));
#35446=CARTESIAN_POINT('Ctrl Pts',(-0.105571360916593,-1.,3.84099658324873));
#35447=CARTESIAN_POINT('Ctrl Pts',(-0.107347597812208,-1.,3.84819233070391));
#35448=CARTESIAN_POINT('Ctrl Pts',(-0.109191717634961,-1.,3.85548571496953));
#35449=CARTESIAN_POINT('Ctrl Pts',(-0.111100593036267,-1.,3.86281867282984));
#35450=CARTESIAN_POINT('Ctrl Pts',(-0.113071304914559,-1.,3.87013043445001));
#35451=CARTESIAN_POINT('Ctrl Pts',(-0.115101426649461,-1.,3.87738168405308));
#35452=CARTESIAN_POINT('Ctrl Pts',(-0.117189150373134,-1.,3.88456590045726));
#35453=CARTESIAN_POINT('Ctrl Pts',(-0.11933308819041,-1.,3.8916960010517));
#35454=CARTESIAN_POINT('Ctrl Pts',(-0.121532144765721,-1.,3.89879639336939));
#35455=CARTESIAN_POINT('Ctrl Pts',(-0.12378536827238,-1.,3.90589336320515));
#35456=CARTESIAN_POINT('Ctrl Pts',(-0.126091793324141,-1.,3.91300501605411));
#35457=CARTESIAN_POINT('Ctrl Pts',(-0.128450341339532,-1.,3.92013513251664));
#35458=CARTESIAN_POINT('Ctrl Pts',(-0.130859892027802,-1.,3.92727876795977));
#35459=CARTESIAN_POINT('Ctrl Pts',(-0.133319322794191,-1.,3.93442567551042));
#35460=CARTESIAN_POINT('Ctrl Pts',(-0.135827558661188,-1.,3.94156445130741));
#35461=CARTESIAN_POINT('Ctrl Pts',(-0.138383621255161,-1.,3.94868667844347));
#35462=CARTESIAN_POINT('Ctrl Pts',(-0.140986665829942,-1.,3.95579014116894));
#35463=CARTESIAN_POINT('Ctrl Pts',(-0.143635947692799,-1.,3.96287658098896));
#35464=CARTESIAN_POINT('Ctrl Pts',(-0.14633079781452,-1.,3.96995018565893));
#35465=CARTESIAN_POINT('Ctrl Pts',(-0.149070594803545,-1.,3.97701581473644));
#35466=CARTESIAN_POINT('Ctrl Pts',(-0.151854737441398,-1.,3.98407729850975));
#35467=CARTESIAN_POINT('Ctrl Pts',(-0.154682618338548,-1.,3.99113582086043));
#35468=CARTESIAN_POINT('Ctrl Pts',(-0.15755363438379,-1.,3.9981907463185));
#35469=CARTESIAN_POINT('Ctrl Pts',(-0.160467194882203,-1.,4.00524031064487));
#35470=CARTESIAN_POINT('Ctrl Pts',(-0.163422730287457,-1.,4.01228237022296));
#35471=CARTESIAN_POINT('Ctrl Pts',(-0.166419700015866,-1.,4.01931510507167));
#35472=CARTESIAN_POINT('Ctrl Pts',(-0.169457601001691,-1.,4.02633779703764));
#35473=CARTESIAN_POINT('Ctrl Pts',(-0.172535962484514,-1.,4.03335057326163));
#35474=CARTESIAN_POINT('Ctrl Pts',(-0.175654339673798,-1.,4.04035407891222));
#35475=CARTESIAN_POINT('Ctrl Pts',(-0.178812307240729,-1.,4.04734916719741));
#35476=CARTESIAN_POINT('Ctrl Pts',(-0.18200945304852,-1.,4.05433660358353));
#35477=CARTESIAN_POINT('Ctrl Pts',(-0.185245370038874,-1.,4.06131670998469));
#35478=CARTESIAN_POINT('Ctrl Pts',(-0.188519658060156,-1.,4.06828941192148));
#35479=CARTESIAN_POINT('Ctrl Pts',(-0.191831928180991,-1.,4.07525439702992));
#35480=CARTESIAN_POINT('Ctrl Pts',(-0.195181806054676,-1.,4.08221124060322));
#35481=CARTESIAN_POINT('Ctrl Pts',(-0.198568934800862,-1.,4.08915953359833));
#35482=CARTESIAN_POINT('Ctrl Pts',(-0.201992979050136,-1.,4.09609903752152));
#35483=CARTESIAN_POINT('Ctrl Pts',(-0.205453622198455,-1.,4.10302969965728));
#35484=CARTESIAN_POINT('Ctrl Pts',(-0.208950559400393,-1.,4.10995157639377));
#35485=CARTESIAN_POINT('Ctrl Pts',(-0.21248349108719,-1.,4.11686478264739));
#35486=CARTESIAN_POINT('Ctrl Pts',(-0.216052116898352,-1.,4.12376943492132));
#35487=CARTESIAN_POINT('Ctrl Pts',(-0.219656126701542,-1.,4.13066558697658));
#35488=CARTESIAN_POINT('Ctrl Pts',(-0.223295201037886,-1.,4.13755320552764));
#35489=CARTESIAN_POINT('Ctrl Pts',(-0.226969025060705,-1.,4.14443220606869));
#35490=CARTESIAN_POINT('Ctrl Pts',(-0.230677299028383,-1.,4.15130247434459));
#35491=CARTESIAN_POINT('Ctrl Pts',(-0.234419749543208,-1.,4.15816389265352));
#35492=CARTESIAN_POINT('Ctrl Pts',(-0.238196140934616,-1.,4.16501636654877));
#35493=CARTESIAN_POINT('Ctrl Pts',(-0.242006283925089,-1.,4.17185984411426));
#35494=CARTESIAN_POINT('Ctrl Pts',(-0.245850033420019,-1.,4.1786943019518));
#35495=CARTESIAN_POINT('Ctrl Pts',(-0.248951836912189,-1.,4.18415464961466));
#35496=CARTESIAN_POINT('Ctrl Pts',(-0.251293239838441,-1.,4.18824585245272));
#35497=CARTESIAN_POINT('Ctrl Pts',(-0.252860861572841,-1.,4.19097151819684));
#35498=CARTESIAN_POINT('Ctrl Pts',(-0.253646344052522,-1.,4.1923339003649));
#35499=CARTESIAN_POINT('',(-0.40530197431835,-1.,4.18039834341342));
#35500=CARTESIAN_POINT('',(-0.253646344052522,-1.,4.1923339003649));
#35501=CARTESIAN_POINT('',(-0.496319364827592,-1.,3.71701050416825));
#35502=CARTESIAN_POINT('Ctrl Pts',(-0.40530197431835,-1.,4.18039834341342));
#35503=CARTESIAN_POINT('Ctrl Pts',(-0.40586466267921,-1.,4.17892985789466));
#35504=CARTESIAN_POINT('Ctrl Pts',(-0.406986596325455,-1.,4.17599251954382));
#35505=CARTESIAN_POINT('Ctrl Pts',(-0.408659167568273,-1.,4.17158541007977));
#35506=CARTESIAN_POINT('Ctrl Pts',(-0.410868596146414,-1.,4.16570705938425));
#35507=CARTESIAN_POINT('Ctrl Pts',(-0.41359587795147,-1.,4.15835545017202));
#35508=CARTESIAN_POINT('Ctrl Pts',(-0.416288556008012,-1.,4.15100018949965));
#35509=CARTESIAN_POINT('Ctrl Pts',(-0.418946490667703,-1.,4.14364132317121));
#35510=CARTESIAN_POINT('Ctrl Pts',(-0.421569503104513,-1.,4.13627893207002));
#35511=CARTESIAN_POINT('Ctrl Pts',(-0.424157375323975,-1.,4.12891314634572));
#35512=CARTESIAN_POINT('Ctrl Pts',(-0.426709855707001,-1.,4.12154412502007));
#35513=CARTESIAN_POINT('Ctrl Pts',(-0.429226666075845,-1.,4.11417202783267));
#35514=CARTESIAN_POINT('Ctrl Pts',(-0.431707508679884,-1.,4.10679698750336));
#35515=CARTESIAN_POINT('Ctrl Pts',(-0.43415207320046,-1.,4.09941908688373));
#35516=CARTESIAN_POINT('Ctrl Pts',(-0.436560044913482,-1.,4.09203832139089));
#35517=CARTESIAN_POINT('Ctrl Pts',(-0.43893110893128,-1.,4.08465462294273));
#35518=CARTESIAN_POINT('Ctrl Pts',(-0.441264951396361,-1.,4.07726792490016));
#35519=CARTESIAN_POINT('Ctrl Pts',(-0.443561262395333,-1.,4.0698782192569));
#35520=CARTESIAN_POINT('Ctrl Pts',(-0.445819737468538,-1.,4.06248560760659));
#35521=CARTESIAN_POINT('Ctrl Pts',(-0.448040082684115,-1.,4.0550903779696));
#35522=CARTESIAN_POINT('Ctrl Pts',(-0.450222009543927,-1.,4.0476929901813));
#35523=CARTESIAN_POINT('Ctrl Pts',(-0.452365214748893,-1.,4.04029392228049));
#35524=CARTESIAN_POINT('Ctrl Pts',(-0.454469363020542,-1.,4.03289354362794));
#35525=CARTESIAN_POINT('Ctrl Pts',(-0.456534070784951,-1.,4.02549199038394));
#35526=CARTESIAN_POINT('Ctrl Pts',(-0.458558885636946,-1.,4.01808900827587));
#35527=CARTESIAN_POINT('Ctrl Pts',(-0.460543280768515,-1.,4.01068390573399));
#35528=CARTESIAN_POINT('Ctrl Pts',(-0.462486702616205,-1.,4.00327590659075));
#35529=CARTESIAN_POINT('Ctrl Pts',(-0.464388610938975,-1.,3.9958644432011));
#35530=CARTESIAN_POINT('Ctrl Pts',(-0.46624852088304,-1.,3.98844946363262));
#35531=CARTESIAN_POINT('Ctrl Pts',(-0.468066047920157,-1.,3.98103175589371));
#35532=CARTESIAN_POINT('Ctrl Pts',(-0.469840942829896,-1.,3.97361320212436));
#35533=CARTESIAN_POINT('Ctrl Pts',(-0.471572978413504,-1.,3.96619600864643));
#35534=CARTESIAN_POINT('Ctrl Pts',(-0.473261847236297,-1.,3.95878201038338));
#35535=CARTESIAN_POINT('Ctrl Pts',(-0.47490705302179,-1.,3.95137192932897));
#35536=CARTESIAN_POINT('Ctrl Pts',(-0.476507810658537,-1.,3.94396469119383));
#35537=CARTESIAN_POINT('Ctrl Pts',(-0.478062927140965,-1.,3.93655660689819));
#35538=CARTESIAN_POINT('Ctrl Pts',(-0.479571028525579,-1.,3.92914297392071));
#35539=CARTESIAN_POINT('Ctrl Pts',(-0.481030798910748,-1.,3.92171976072341));
#35540=CARTESIAN_POINT('Ctrl Pts',(-0.482441230340713,-1.,3.91428536373751));
#35541=CARTESIAN_POINT('Ctrl Pts',(-0.48380183508915,-1.,3.90684210358056));
#35542=CARTESIAN_POINT('Ctrl Pts',(-0.485112963522222,-1.,3.89939844658513));
#35543=CARTESIAN_POINT('Ctrl Pts',(-0.486375337854103,-1.,3.89196582437552));
#35544=CARTESIAN_POINT('Ctrl Pts',(-0.487589452275155,-1.,3.88455453328138));
#35545=CARTESIAN_POINT('Ctrl Pts',(-0.488754973798274,-1.,3.87716963231109));
#35546=CARTESIAN_POINT('Ctrl Pts',(-0.489870245704918,-1.,3.86980755613707));
#35547=CARTESIAN_POINT('Ctrl Pts',(-0.490931482170891,-1.,3.86245057319246));
#35548=CARTESIAN_POINT('Ctrl Pts',(-0.491933631083813,-1.,3.85507287020263));
#35549=CARTESIAN_POINT('Ctrl Pts',(-0.492871792414141,-1.,3.84765051147999));
#35550=CARTESIAN_POINT('Ctrl Pts',(-0.493742574629135,-1.,3.84017095578451));
#35551=CARTESIAN_POINT('Ctrl Pts',(-0.494545212256401,-1.,3.83264092682431));
#35552=CARTESIAN_POINT('Ctrl Pts',(-0.495283458893837,-1.,3.82509963594103));
#35553=CARTESIAN_POINT('Ctrl Pts',(-0.49596393787548,-1.,3.81760756144025));
#35554=CARTESIAN_POINT('Ctrl Pts',(-0.496592643443704,-1.,3.81022254090839));
#35555=CARTESIAN_POINT('Ctrl Pts',(-0.497171756201052,-1.,3.80297788298514));
#35556=CARTESIAN_POINT('Ctrl Pts',(-0.497696892100625,-1.,3.79586380669994));
#35557=CARTESIAN_POINT('Ctrl Pts',(-0.498152751800958,-1.,3.78879701661264));
#35558=CARTESIAN_POINT('Ctrl Pts',(-0.498515471679585,-1.,3.78163975337356));
#35559=CARTESIAN_POINT('Ctrl Pts',(-0.498759900365892,-1.,3.77425499225255));
#35560=CARTESIAN_POINT('Ctrl Pts',(-0.498865792335291,-1.,3.76655401191229));
#35561=CARTESIAN_POINT('Ctrl Pts',(-0.498823681615422,-1.,3.75854082221053));
#35562=CARTESIAN_POINT('Ctrl Pts',(-0.498642802042606,-1.,3.75037362167839));
#35563=CARTESIAN_POINT('Ctrl Pts',(-0.498350586057692,-1.,3.74235701734714));
#35564=CARTESIAN_POINT('Ctrl Pts',(-0.497984209510024,-1.,3.73486914372449));
#35565=CARTESIAN_POINT('Ctrl Pts',(-0.497584067153049,-1.,3.72830430904606));
#35566=CARTESIAN_POINT('Ctrl Pts',(-0.497187079575988,-1.,3.72301489774398));
#35567=CARTESIAN_POINT('Ctrl Pts',(-0.496846224822564,-1.,3.71952320822499));
#35568=CARTESIAN_POINT('Ctrl Pts',(-0.496605651525989,-1.,3.71785517607549));
#35569=CARTESIAN_POINT('Ctrl Pts',(-0.496446644158005,-1.,3.71721917030355));
#35570=CARTESIAN_POINT('Ctrl Pts',(-0.496354087924313,-1.,3.71704500630495));
#35571=CARTESIAN_POINT('Ctrl Pts',(-0.496319364827592,-1.,3.71701050416825));
#35572=CARTESIAN_POINT('',(-0.676591647973661,-1.,3.68845817949618));
#35573=CARTESIAN_POINT('Origin',(0.,-1.,0.));
#35574=CARTESIAN_POINT('',(-0.906349047628866,-1.,4.10104028313088));
#35575=CARTESIAN_POINT('Ctrl Pts',(-0.676591647973661,-1.,3.68845817949618));
#35576=CARTESIAN_POINT('Ctrl Pts',(-0.67656928609342,-1.,3.68850172300543));
#35577=CARTESIAN_POINT('Ctrl Pts',(-0.676535079520365,-1.,3.68869596426099));
#35578=CARTESIAN_POINT('Ctrl Pts',(-0.676580391119535,-1.,3.68934997767391));
#35579=CARTESIAN_POINT('Ctrl Pts',(-0.676867042599712,-1.,3.6910107117555));
#35580=CARTESIAN_POINT('Ctrl Pts',(-0.677621861865196,-1.,3.69443683573443));
#35581=CARTESIAN_POINT('Ctrl Pts',(-0.67887882222639,-1.,3.69959004073192));
#35582=CARTESIAN_POINT('Ctrl Pts',(-0.680526909711618,-1.,3.70595722032165));
#35583=CARTESIAN_POINT('Ctrl Pts',(-0.682492345109689,-1.,3.71319182790334));
#35584=CARTESIAN_POINT('Ctrl Pts',(-0.684691698168355,-1.,3.7209063713952));
#35585=CARTESIAN_POINT('Ctrl Pts',(-0.687043475232499,-1.,3.72872973554125));
#35586=CARTESIAN_POINT('Ctrl Pts',(-0.689479637354651,-1.,3.73636374474993));
#35587=CARTESIAN_POINT('Ctrl Pts',(-0.691960080400503,-1.,3.74365508986548));
#35588=CARTESIAN_POINT('Ctrl Pts',(-0.694474562581173,-1.,3.7506028824329));
#35589=CARTESIAN_POINT('Ctrl Pts',(-0.69703124565953,-1.,3.75729775766913));
#35590=CARTESIAN_POINT('Ctrl Pts',(-0.699648552230851,-1.,3.76387780603725));
#35591=CARTESIAN_POINT('Ctrl Pts',(-0.702346356621613,-1.,3.77048141872904));
#35592=CARTESIAN_POINT('Ctrl Pts',(-0.70513584799995,-1.,3.77719254217197));
#35593=CARTESIAN_POINT('Ctrl Pts',(-0.7080158793756,-1.,3.78402183336678));
#35594=CARTESIAN_POINT('Ctrl Pts',(-0.710978231689117,-1.,3.79093694007146));
#35595=CARTESIAN_POINT('Ctrl Pts',(-0.714010733006677,-1.,3.79788100314994));
#35596=CARTESIAN_POINT('Ctrl Pts',(-0.717100993669091,-1.,3.80479445759296));
#35597=CARTESIAN_POINT('Ctrl Pts',(-0.720240466589172,-1.,3.81163885127309));
#35598=CARTESIAN_POINT('Ctrl Pts',(-0.723426346019349,-1.,3.81840802610795));
#35599=CARTESIAN_POINT('Ctrl Pts',(-0.726659281876608,-1.,3.82511495756682));
#35600=CARTESIAN_POINT('Ctrl Pts',(-0.729942010490146,-1.,3.8317839240337));
#35601=CARTESIAN_POINT('Ctrl Pts',(-0.73327770375609,-1.,3.83844103658016));
#35602=CARTESIAN_POINT('Ctrl Pts',(-0.736668240497151,-1.,3.84510432881231));
#35603=CARTESIAN_POINT('Ctrl Pts',(-0.740113146827176,-1.,3.85177770351237));
#35604=CARTESIAN_POINT('Ctrl Pts',(-0.743610542737042,-1.,3.85845645217611));
#35605=CARTESIAN_POINT('Ctrl Pts',(-0.747157716488884,-1.,3.86513062969896));
#35606=CARTESIAN_POINT('Ctrl Pts',(-0.750751822383024,-1.,3.87178914078372));
#35607=CARTESIAN_POINT('Ctrl Pts',(-0.754390577396847,-1.,3.87842382520058));
#35608=CARTESIAN_POINT('Ctrl Pts',(-0.758072800564799,-1.,3.88503262662684));
#35609=CARTESIAN_POINT('Ctrl Pts',(-0.761798028793978,-1.,3.89161738162245));
#35610=CARTESIAN_POINT('Ctrl Pts',(-0.765566256401306,-1.,3.89818233104381));
#35611=CARTESIAN_POINT('Ctrl Pts',(-0.769377629847877,-1.,3.90473237182634));
#35612=CARTESIAN_POINT('Ctrl Pts',(-0.773232154506305,-1.,3.91127138115238));
#35613=CARTESIAN_POINT('Ctrl Pts',(-0.777129415664915,-1.,3.91780062334464));
#35614=CARTESIAN_POINT('Ctrl Pts',(-0.781068718228395,-1.,3.92431956510418));
#35615=CARTESIAN_POINT('Ctrl Pts',(-0.785049202786458,-1.,3.93082655631768));
#35616=CARTESIAN_POINT('Ctrl Pts',(-0.789069971469323,-1.,3.93731956885671));
#35617=CARTESIAN_POINT('Ctrl Pts',(-0.793130205641017,-1.,3.94379688971307));
#35618=CARTESIAN_POINT('Ctrl Pts',(-0.797229296085438,-1.,3.95025788827189));
#35619=CARTESIAN_POINT('Ctrl Pts',(-0.801366797727206,-1.,3.95670276375176));
#35620=CARTESIAN_POINT('Ctrl Pts',(-0.805542372178496,-1.,3.96313222295874));
#35621=CARTESIAN_POINT('Ctrl Pts',(-0.809755732818134,-1.,3.96954717513251));
#35622=CARTESIAN_POINT('Ctrl Pts',(-0.814006592328737,-1.,3.97594844078763));
#35623=CARTESIAN_POINT('Ctrl Pts',(-0.818294599022033,-1.,3.98233640155287));
#35624=CARTESIAN_POINT('Ctrl Pts',(-0.822619346021769,-1.,3.98871104646328));
#35625=CARTESIAN_POINT('Ctrl Pts',(-0.826980400320473,-1.,3.99507212784289));
#35626=CARTESIAN_POINT('Ctrl Pts',(-0.831377325741487,-1.,4.00141928477447));
#35627=CARTESIAN_POINT('Ctrl Pts',(-0.835809705809822,-1.,4.00775216907934));
#35628=CARTESIAN_POINT('Ctrl Pts',(-0.84027717197638,-1.,4.01407059766338));
#35629=CARTESIAN_POINT('Ctrl Pts',(-0.844779403288517,-1.,4.02037456798787));
#35630=CARTESIAN_POINT('Ctrl Pts',(-0.849316107475012,-1.,4.02666418343508));
#35631=CARTESIAN_POINT('Ctrl Pts',(-0.853887006632178,-1.,4.03293960436945));
#35632=CARTESIAN_POINT('Ctrl Pts',(-0.858491822322571,-1.,4.03920099284658));
#35633=CARTESIAN_POINT('Ctrl Pts',(-0.863130256642173,-1.,4.04544845048097));
#35634=CARTESIAN_POINT('Ctrl Pts',(-0.867801988858176,-1.,4.05168199437128));
#35635=CARTESIAN_POINT('Ctrl Pts',(-0.872506694780563,-1.,4.05790159030495));
#35636=CARTESIAN_POINT('Ctrl Pts',(-0.877244060484595,-1.,4.06410717232347));
#35637=CARTESIAN_POINT('Ctrl Pts',(-0.882013797525916,-1.,4.07029866694292));
#35638=CARTESIAN_POINT('Ctrl Pts',(-0.886815658360739,-1.,4.07647601774639));
#35639=CARTESIAN_POINT('Ctrl Pts',(-0.891649447920401,-1.,4.08263920306651));
#35640=CARTESIAN_POINT('Ctrl Pts',(-0.896515019236368,-1.,4.08878822249095));
#35641=CARTESIAN_POINT('Ctrl Pts',(-0.900432820945975,-1.,4.09369611524319));
#35642=CARTESIAN_POINT('Ctrl Pts',(-0.903385402444213,-1.,4.09737067247114));
#35643=CARTESIAN_POINT('Ctrl Pts',(-0.905360112216302,-1.,4.09981755067956));
#35644=CARTESIAN_POINT('Ctrl Pts',(-0.906349047628866,-1.,4.10104028313088));
#35645=CARTESIAN_POINT('',(-1.05427041296137,-1.,4.06552750530042));
#35646=CARTESIAN_POINT('',(-0.906349047628866,-1.,4.10104028313088));
#35647=CARTESIAN_POINT('',(-1.07167739962028,-1.,3.59360648251073));
#35648=CARTESIAN_POINT('Ctrl Pts',(-1.05427041296137,-1.,4.06552750530042));
#35649=CARTESIAN_POINT('Ctrl Pts',(-1.05459645194823,-1.,4.06398907542249));
#35650=CARTESIAN_POINT('Ctrl Pts',(-1.055245071776,-1.,4.06091239149123));
#35651=CARTESIAN_POINT('Ctrl Pts',(-1.05620762707996,-1.,4.05629789307025));
#35652=CARTESIAN_POINT('Ctrl Pts',(-1.05747027727959,-1.,4.05014628384869));
#35653=CARTESIAN_POINT('Ctrl Pts',(-1.05901393666566,-1.,4.04245854427496));
#35654=CARTESIAN_POINT('Ctrl Pts',(-1.06052284711857,-1.,4.03477261141553));
#35655=CARTESIAN_POINT('Ctrl Pts',(-1.06199687787462,-1.,4.02708855235633));
#35656=CARTESIAN_POINT('Ctrl Pts',(-1.06343586496236,-1.,4.01940647495943));
#35657=CARTESIAN_POINT('Ctrl Pts',(-1.06483961343109,-1.,4.01172654187398));
#35658=CARTESIAN_POINT('Ctrl Pts',(-1.06620789963606,-1.,4.00404894952579));
#35659=CARTESIAN_POINT('Ctrl Pts',(-1.06754047381312,-1.,3.99637389920441));
#35660=CARTESIAN_POINT('Ctrl Pts',(-1.06883706263942,-1.,3.98870156857412));
#35661=CARTESIAN_POINT('Ctrl Pts',(-1.07009737257767,-1.,3.98103208801101));
#35662=CARTESIAN_POINT('Ctrl Pts',(-1.07132109206164,-1.,3.9733655022223));
#35663=CARTESIAN_POINT('Ctrl Pts',(-1.07250789943007,-1.,3.96570179322338));
#35664=CARTESIAN_POINT('Ctrl Pts',(-1.07365747426491,-1.,3.95804094429373));
#35665=CARTESIAN_POINT('Ctrl Pts',(-1.07476950921587,-1.,3.95038299600676));
#35666=CARTESIAN_POINT('Ctrl Pts',(-1.07584371946443,-1.,3.94272809633331));
#35667=CARTESIAN_POINT('Ctrl Pts',(-1.07687985975384,-1.,3.93507657572883));
#35668=CARTESIAN_POINT('Ctrl Pts',(-1.07787771707195,-1.,3.9274289334984));
#35669=CARTESIAN_POINT('Ctrl Pts',(-1.07883706663554,-1.,3.91978568924178));
#35670=CARTESIAN_POINT('Ctrl Pts',(-1.07975763507473,-1.,3.91214726022143));
#35671=CARTESIAN_POINT('Ctrl Pts',(-1.08063906483818,-1.,3.90451384092545));
#35672=CARTESIAN_POINT('Ctrl Pts',(-1.08148086931358,-1.,3.8968852509835));
#35673=CARTESIAN_POINT('Ctrl Pts',(-1.08228241999346,-1.,3.88926088975114));
#35674=CARTESIAN_POINT('Ctrl Pts',(-1.08304304871028,-1.,3.88164007721312));
#35675=CARTESIAN_POINT('Ctrl Pts',(-1.08376213307504,-1.,3.8740223372254));
#35676=CARTESIAN_POINT('Ctrl Pts',(-1.08443918607927,-1.,3.86640769434274));
#35677=CARTESIAN_POINT('Ctrl Pts',(-1.08507395120059,-1.,3.85879698702532));
#35678=CARTESIAN_POINT('Ctrl Pts',(-1.08566647671844,-1.,3.85119211322755));
#35679=CARTESIAN_POINT('Ctrl Pts',(-1.08621688337604,-1.,3.8435952876495));
#35680=CARTESIAN_POINT('Ctrl Pts',(-1.08672515456902,-1.,3.83600837071708));
#35681=CARTESIAN_POINT('Ctrl Pts',(-1.08719091307558,-1.,3.82843215316984));
#35682=CARTESIAN_POINT('Ctrl Pts',(-1.08761321539442,-1.,3.82086569676319));
#35683=CARTESIAN_POINT('Ctrl Pts',(-1.08799030610862,-1.,3.81330554446323));
#35684=CARTESIAN_POINT('Ctrl Pts',(-1.0883200925538,-1.,3.8057472665766));
#35685=CARTESIAN_POINT('Ctrl Pts',(-1.08860064435778,-1.,3.79818708705259));
#35686=CARTESIAN_POINT('Ctrl Pts',(-1.08883071512098,-1.,3.79062357974404));
#35687=CARTESIAN_POINT('Ctrl Pts',(-1.08901018614636,-1.,3.78305911299504));
#35688=CARTESIAN_POINT('Ctrl Pts',(-1.0891407279127,-1.,3.77550199409424));
#35689=CARTESIAN_POINT('Ctrl Pts',(-1.08922484204256,-1.,3.76796340094448));
#35690=CARTESIAN_POINT('Ctrl Pts',(-1.08926462734282,-1.,3.76045342580208));
#35691=CARTESIAN_POINT('Ctrl Pts',(-1.08926054632925,-1.,3.75297711748132));
#35692=CARTESIAN_POINT('Ctrl Pts',(-1.08921040494017,-1.,3.74553121371757));
#35693=CARTESIAN_POINT('Ctrl Pts',(-1.08910769013297,-1.,3.73809879348239));
#35694=CARTESIAN_POINT('Ctrl Pts',(-1.08894337390937,-1.,3.73065515162988));
#35695=CARTESIAN_POINT('Ctrl Pts',(-1.08870887220082,-1.,3.72317741369398));
#35696=CARTESIAN_POINT('Ctrl Pts',(-1.0883988733478,-1.,3.71565372339075));
#35697=CARTESIAN_POINT('Ctrl Pts',(-1.08801367312185,-1.,3.70809084139457));
#35698=CARTESIAN_POINT('Ctrl Pts',(-1.08756311291309,-1.,3.70052690909833));
#35699=CARTESIAN_POINT('Ctrl Pts',(-1.08706319540271,-1.,3.69302062410157));
#35700=CARTESIAN_POINT('Ctrl Pts',(-1.0865288888259,-1.,3.68562817420797));
#35701=CARTESIAN_POINT('Ctrl Pts',(-1.0859675575576,-1.,3.67838211685117));
#35702=CARTESIAN_POINT('Ctrl Pts',(-1.0853733414449,-1.,3.67127347729666));
#35703=CARTESIAN_POINT('Ctrl Pts',(-1.08471809922901,-1.,3.66422237895365));
#35704=CARTESIAN_POINT('Ctrl Pts',(-1.08395671077807,-1.,3.65709649161166));
#35705=CARTESIAN_POINT('Ctrl Pts',(-1.08304289898623,-1.,3.64976441208358));
#35706=CARTESIAN_POINT('Ctrl Pts',(-1.08194278850996,-1.,3.64214167843677));
#35707=CARTESIAN_POINT('Ctrl Pts',(-1.08064765719867,-1.,3.63423373196529));
#35708=CARTESIAN_POINT('Ctrl Pts',(-1.07919137290742,-1.,3.62619537902361));
#35709=CARTESIAN_POINT('Ctrl Pts',(-1.07764868137619,-1.,3.61832318504574));
#35710=CARTESIAN_POINT('Ctrl Pts',(-1.07611545402734,-1.,3.61098481349204));
#35711=CARTESIAN_POINT('Ctrl Pts',(-1.07469327168578,-1.,3.60456339887778));
#35712=CARTESIAN_POINT('Ctrl Pts',(-1.07347372545714,-1.,3.59940121154535));
#35713=CARTESIAN_POINT('Ctrl Pts',(-1.07259084660936,-1.,3.59600583194946));
#35714=CARTESIAN_POINT('Ctrl Pts',(-1.07209229745229,-1.,3.59439596999862));
#35715=CARTESIAN_POINT('Ctrl Pts',(-1.07183575450617,-1.,3.59379266874567));
#35716=CARTESIAN_POINT('Ctrl Pts',(-1.07171709254135,-1.,3.5936351279798));
#35717=CARTESIAN_POINT('Ctrl Pts',(-1.07167739962028,-1.,3.59360648251073));
#35718=CARTESIAN_POINT('',(-1.24526366418038,-1.,3.5372048861597));
#35719=CARTESIAN_POINT('Origin',(0.,-1.,0.));
#35720=CARTESIAN_POINT('',(-1.53673442965256,-1.,3.90876544355381));
#35721=CARTESIAN_POINT('Ctrl Pts',(-1.24526366418038,-1.,3.5372048861597));
#35722=CARTESIAN_POINT('Ctrl Pts',(-1.24524838931757,-1.,3.53725139174486));
#35723=CARTESIAN_POINT('Ctrl Pts',(-1.2452449899111,-1.,3.5374485926552));
#35724=CARTESIAN_POINT('Ctrl Pts',(-1.24539205388767,-1.,3.53808746578196));
#35725=CARTESIAN_POINT('Ctrl Pts',(-1.24593497226008,-1.,3.53968291130022));
#35726=CARTESIAN_POINT('Ctrl Pts',(-1.24721646231966,-1.,3.54294877425964));
#35727=CARTESIAN_POINT('Ctrl Pts',(-1.24926408628003,-1.,3.54784190283068));
#35728=CARTESIAN_POINT('Ctrl Pts',(-1.2518879294064,-1.,3.55387287418985));
#35729=CARTESIAN_POINT('Ctrl Pts',(-1.25496090900009,-1.,3.56071094991199));
#35730=CARTESIAN_POINT('Ctrl Pts',(-1.25834000485716,-1.,3.56798645995275));
#35731=CARTESIAN_POINT('Ctrl Pts',(-1.2618866714281,-1.,3.5753456065171));
#35732=CARTESIAN_POINT('Ctrl Pts',(-1.26548706249862,-1.,3.58250452868618));
#35733=CARTESIAN_POINT('Ctrl Pts',(-1.26907758484709,-1.,3.58931807846313));
#35734=CARTESIAN_POINT('Ctrl Pts',(-1.27264798379307,-1.,3.59578698050006));
#35735=CARTESIAN_POINT('Ctrl Pts',(-1.27622049908625,-1.,3.60199947736298));
#35736=CARTESIAN_POINT('Ctrl Pts',(-1.27983492861691,-1.,3.60808907746339));
#35737=CARTESIAN_POINT('Ctrl Pts',(-1.28353255117765,-1.,3.61418935913823));
#35738=CARTESIAN_POINT('Ctrl Pts',(-1.28733755029384,-1.,3.6203814849236));
#35739=CARTESIAN_POINT('Ctrl Pts',(-1.29125046021878,-1.,3.62667616004369));
#35740=CARTESIAN_POINT('Ctrl Pts',(-1.29525810207762,-1.,3.63304271631046));
#35741=CARTESIAN_POINT('Ctrl Pts',(-1.2993395590647,-1.,3.63942689872808));
#35742=CARTESIAN_POINT('Ctrl Pts',(-1.30347327603774,-1.,3.64577181380113));
#35743=CARTESIAN_POINT('Ctrl Pts',(-1.30764479590039,-1.,3.65204081987068));
#35744=CARTESIAN_POINT('Ctrl Pts',(-1.31185038411218,-1.,3.65822827358617));
#35745=CARTESIAN_POINT('Ctrl Pts',(-1.31609271239911,-1.,3.66434688899793));
#35746=CARTESIAN_POINT('Ctrl Pts',(-1.32037828137766,-1.,3.67042021752656));
#35747=CARTESIAN_POINT('Ctrl Pts',(-1.32471430856415,-1.,3.67647355257912));
#35748=CARTESIAN_POINT('Ctrl Pts',(-1.3291054707274,-1.,3.68252441182551));
#35749=CARTESIAN_POINT('Ctrl Pts',(-1.33355191034523,-1.,3.68857672413033));
#35750=CARTESIAN_POINT('Ctrl Pts',(-1.3380510339822,-1.,3.69462613305708));
#35751=CARTESIAN_POINT('Ctrl Pts',(-1.34259860752933,-1.,3.70066324015119));
#35752=CARTESIAN_POINT('Ctrl Pts',(-1.34719008463534,-1.,3.70667753188248));
#35753=CARTESIAN_POINT('Ctrl Pts',(-1.35182193384424,-1.,3.71266130563054));
#35754=CARTESIAN_POINT('Ctrl Pts',(-1.35649266705037,-1.,3.71861271513313));
#35755=CARTESIAN_POINT('Ctrl Pts',(-1.36120211416354,-1.,3.72453364678279));
#35756=CARTESIAN_POINT('Ctrl Pts',(-1.36595093298676,-1.,3.73042829011295));
#35757=CARTESIAN_POINT('Ctrl Pts',(-1.37074003422739,-1.,3.7363014588581));
#35758=CARTESIAN_POINT('Ctrl Pts',(-1.37557002971687,-1.,3.74215698162555));
#35759=CARTESIAN_POINT('Ctrl Pts',(-1.38044070763295,-1.,3.74799617204729));
#35760=CARTESIAN_POINT('Ctrl Pts',(-1.38535129801176,-1.,3.75381861212707));
#35761=CARTESIAN_POINT('Ctrl Pts',(-1.39030069388918,-1.,3.75962280650855));
#35762=CARTESIAN_POINT('Ctrl Pts',(-1.39528769118052,-1.,3.76540689249074));
#35763=CARTESIAN_POINT('Ctrl Pts',(-1.40031121335505,-1.,3.77116930621827));
#35764=CARTESIAN_POINT('Ctrl Pts',(-1.40537056004722,-1.,3.77690952014259));
#35765=CARTESIAN_POINT('Ctrl Pts',(-1.41046532282593,-1.,3.78262780065471));
#35766=CARTESIAN_POINT('Ctrl Pts',(-1.4155952780383,-1.,3.78832489879426));
#35767=CARTESIAN_POINT('Ctrl Pts',(-1.42076028482836,-1.,3.79400175744408));
#35768=CARTESIAN_POINT('Ctrl Pts',(-1.42596018777283,-1.,3.7996592319632));
#35769=CARTESIAN_POINT('Ctrl Pts',(-1.4311946992132,-1.,3.80529775429805));
#35770=CARTESIAN_POINT('Ctrl Pts',(-1.43646341556724,-1.,3.81091737726815));
#35771=CARTESIAN_POINT('Ctrl Pts',(-1.44176587041347,-1.,3.81651792398414));
#35772=CARTESIAN_POINT('Ctrl Pts',(-1.44710157648539,-1.,3.82209910620533));
#35773=CARTESIAN_POINT('Ctrl Pts',(-1.45247006796836,-1.,3.82766064519074));
#35774=CARTESIAN_POINT('Ctrl Pts',(-1.45787095220852,-1.,3.83320241775423));
#35775=CARTESIAN_POINT('Ctrl Pts',(-1.46330391180752,-1.,3.83872447159639));
#35776=CARTESIAN_POINT('Ctrl Pts',(-1.46876867426504,-1.,3.84422695454796));
#35777=CARTESIAN_POINT('Ctrl Pts',(-1.47426499018538,-1.,3.84971006847277));
#35778=CARTESIAN_POINT('Ctrl Pts',(-1.4797926099102,-1.,3.85517401698843));
#35779=CARTESIAN_POINT('Ctrl Pts',(-1.48535125509919,-1.,3.86061894706087));
#35780=CARTESIAN_POINT('Ctrl Pts',(-1.4909406116431,-1.,3.86604492575189));
#35781=CARTESIAN_POINT('Ctrl Pts',(-1.49656035399122,-1.,3.87145196998465));
#35782=CARTESIAN_POINT('Ctrl Pts',(-1.50221016176556,-1.,3.87684006372134));
#35783=CARTESIAN_POINT('Ctrl Pts',(-1.50788973857757,-1.,3.88220917950538));
#35784=CARTESIAN_POINT('Ctrl Pts',(-1.51359883110559,-1.,3.88755930033884));
#35785=CARTESIAN_POINT('Ctrl Pts',(-1.51933724329306,-1.,3.89289043533657));
#35786=CARTESIAN_POINT('Ctrl Pts',(-1.52510482991635,-1.,3.89820260708225));
#35787=CARTESIAN_POINT('Ctrl Pts',(-1.52974216056287,-1.,3.90243719631596));
#35788=CARTESIAN_POINT('Ctrl Pts',(-1.53323321827755,-1.,3.90560462813969));
#35789=CARTESIAN_POINT('Ctrl Pts',(-1.53556639217905,-1.,3.90771246855019));
#35790=CARTESIAN_POINT('Ctrl Pts',(-1.53673442965256,-1.,3.90876544355381));
#35791=CARTESIAN_POINT('',(-1.67727921511438,-1.,3.85054988729471));
#35792=CARTESIAN_POINT('',(-1.53673442965256,-1.,3.90876544355381));
#35793=CARTESIAN_POINT('',(-1.62064718014094,-1.,3.38171594275765));
#35794=CARTESIAN_POINT('Ctrl Pts',(-1.67727921511438,-1.,3.85054988729471));
#35795=CARTESIAN_POINT('Ctrl Pts',(-1.67736057656533,-1.,3.84897939430696));
#35796=CARTESIAN_POINT('Ctrl Pts',(-1.6775199114018,-1.,3.84583912296459));
#35797=CARTESIAN_POINT('Ctrl Pts',(-1.67774874946079,-1.,3.84113085985244));
#35798=CARTESIAN_POINT('Ctrl Pts',(-1.67803353064351,-1.,3.83485746513989));
#35799=CARTESIAN_POINT('Ctrl Pts',(-1.6783555575934,-1.,3.82702289286713));
#35800=CARTESIAN_POINT('Ctrl Pts',(-1.67864354605954,-1.,3.81919554099578));
#35801=CARTESIAN_POINT('Ctrl Pts',(-1.6788973773827,-1.,3.81137549624178));
#35802=CARTESIAN_POINT('Ctrl Pts',(-1.67911690648355,-1.,3.80356289079005));
#35803=CARTESIAN_POINT('Ctrl Pts',(-1.67930196625548,-1.,3.79575791578424));
#35804=CARTESIAN_POINT('Ctrl Pts',(-1.67945236653493,-1.,3.7879608002176));
#35805=CARTESIAN_POINT('Ctrl Pts',(-1.67956789212141,-1.,3.78017178197317));
#35806=CARTESIAN_POINT('Ctrl Pts',(-1.67964830084993,-1.,3.77239107928502));
#35807=CARTESIAN_POINT('Ctrl Pts',(-1.67969332319245,-1.,3.76461886684344));
#35808=CARTESIAN_POINT('Ctrl Pts',(-1.67970265841239,-1.,3.75685523754493));
#35809=CARTESIAN_POINT('Ctrl Pts',(-1.67967598599525,-1.,3.7491002239452));
#35810=CARTESIAN_POINT('Ctrl Pts',(-1.6796129868522,-1.,3.74135385965401));
#35811=CARTESIAN_POINT('Ctrl Pts',(-1.67951336376402,-1.,3.73361623282543));
#35812=CARTESIAN_POINT('Ctrl Pts',(-1.67937685856652,-1.,3.72588753416396));
#35813=CARTESIAN_POINT('Ctrl Pts',(-1.67920328071708,-1.,3.71816812842322));
#35814=CARTESIAN_POINT('Ctrl Pts',(-1.67899249793462,-1.,3.71045854208343));
#35815=CARTESIAN_POINT('Ctrl Pts',(-1.67874436948667,-1.,3.70275932351108));
#35816=CARTESIAN_POINT('Ctrl Pts',(-1.67845869064323,-1.,3.6950709275959));
#35817=CARTESIAN_POINT('Ctrl Pts',(-1.67813513867965,-1.,3.68739360236487));
#35818=CARTESIAN_POINT('Ctrl Pts',(-1.67777320475848,-1.,3.67972724579124));
#35819=CARTESIAN_POINT('Ctrl Pts',(-1.67737217414874,-1.,3.67207136294575));
#35820=CARTESIAN_POINT('Ctrl Pts',(-1.67693128053132,-1.,3.66442538670968));
#35821=CARTESIAN_POINT('Ctrl Pts',(-1.6764498346945,-1.,3.6567889441642));
#35822=CARTESIAN_POINT('Ctrl Pts',(-1.67592735946692,-1.,3.64916213574667));
#35823=CARTESIAN_POINT('Ctrl Pts',(-1.67536373264848,-1.,3.6415458297234));
#35824=CARTESIAN_POINT('Ctrl Pts',(-1.67475929882971,-1.,3.63394189312924));
#35825=CARTESIAN_POINT('Ctrl Pts',(-1.67411452372271,-1.,3.62635249450923));
#35826=CARTESIAN_POINT('Ctrl Pts',(-1.67342968196224,-1.,3.61877947398184));
#35827=CARTESIAN_POINT('Ctrl Pts',(-1.67270452466968,-1.,3.61122367156181));
#35828=CARTESIAN_POINT('Ctrl Pts',(-1.67193797318597,-1.,3.603684308152));
#35829=CARTESIAN_POINT('Ctrl Pts',(-1.67112775290707,-1.,3.59615824388807));
#35830=CARTESIAN_POINT('Ctrl Pts',(-1.67027110397604,-1.,3.58864143097834));
#35831=CARTESIAN_POINT('Ctrl Pts',(-1.66936552908232,-1.,3.58113044183829));
#35832=CARTESIAN_POINT('Ctrl Pts',(-1.668409574073,-1.,3.57362406285887));
#35833=CARTESIAN_POINT('Ctrl Pts',(-1.66740349220305,-1.,3.56612465179422));
#35834=CARTESIAN_POINT('Ctrl Pts',(-1.66635023293114,-1.,3.55864015233602));
#35835=CARTESIAN_POINT('Ctrl Pts',(-1.66525401568994,-1.,3.55118121342861));
#35836=CARTESIAN_POINT('Ctrl Pts',(-1.66411849222326,-1.,3.54375747475014));
#35837=CARTESIAN_POINT('Ctrl Pts',(-1.66294490916111,-1.,3.5363738506022));
#35838=CARTESIAN_POINT('Ctrl Pts',(-1.66173058912371,-1.,3.52902746211093));
#35839=CARTESIAN_POINT('Ctrl Pts',(-1.66046645222279,-1.,3.52170261543815));
#35840=CARTESIAN_POINT('Ctrl Pts',(-1.65913971687342,-1.,3.5143763218894));
#35841=CARTESIAN_POINT('Ctrl Pts',(-1.65773832633632,-1.,3.50702733146542));
#35842=CARTESIAN_POINT('Ctrl Pts',(-1.65625517961588,-1.,3.4996447647794));
#35843=CARTESIAN_POINT('Ctrl Pts',(-1.65469162644468,-1.,3.49223525300176));
#35844=CARTESIAN_POINT('Ctrl Pts',(-1.65306335367739,-1.,3.48483492840894));
#35845=CARTESIAN_POINT('Ctrl Pts',(-1.65139534930322,-1.,3.47749926256476));
#35846=CARTESIAN_POINT('Ctrl Pts',(-1.64971118698256,-1.,3.47028140995992));
#35847=CARTESIAN_POINT('Ctrl Pts',(-1.64802323352738,-1.,3.46321237515));
#35848=CARTESIAN_POINT('Ctrl Pts',(-1.64632429697521,-1.,3.45628421062422));
#35849=CARTESIAN_POINT('Ctrl Pts',(-1.64457408708107,-1.,3.44942242546795));
#35850=CARTESIAN_POINT('Ctrl Pts',(-1.64270733821113,-1.,3.44250337701888));
#35851=CARTESIAN_POINT('Ctrl Pts',(-1.64065778702023,-1.,3.43540451921548));
#35852=CARTESIAN_POINT('Ctrl Pts',(-1.63837876246926,-1.,3.42804772926291));
#35853=CARTESIAN_POINT('Ctrl Pts',(-1.63586250099773,-1.,3.42043974590882));
#35854=CARTESIAN_POINT('Ctrl Pts',(-1.63316667054044,-1.,3.41272817148478));
#35855=CARTESIAN_POINT('Ctrl Pts',(-1.63041148964828,-1.,3.40519422740235));
#35856=CARTESIAN_POINT('Ctrl Pts',(-1.62774916464408,-1.,3.39818605297991));
#35857=CARTESIAN_POINT('Ctrl Pts',(-1.62533996116713,-1.,3.39206617496906));
#35858=CARTESIAN_POINT('Ctrl Pts',(-1.6233278855625,-1.,3.38715832179072));
#35859=CARTESIAN_POINT('Ctrl Pts',(-1.62192472202769,-1.,3.38394285763222));
#35860=CARTESIAN_POINT('Ctrl Pts',(-1.62118047294498,-1.,3.38243080602408));
#35861=CARTESIAN_POINT('Ctrl Pts',(-1.62083271135947,-1.,3.38187506456922));
#35862=CARTESIAN_POINT('Ctrl Pts',(-1.62069086551492,-1.,3.38173802621259));
#35863=CARTESIAN_POINT('Ctrl Pts',(-1.62064718014094,-1.,3.38171594275764));
#35864=CARTESIAN_POINT('',(-1.78327315618183,-1.,3.29885386921599));
#35865=CARTESIAN_POINT('Origin',(0.,-1.,0.));
#35866=CARTESIAN_POINT('',(-2.12928030988903,-1.,3.62024382630768));
#35867=CARTESIAN_POINT('Ctrl Pts',(-1.78327315618183,-1.,3.29885386921599));
#35868=CARTESIAN_POINT('Ctrl Pts',(-1.78326534445426,-1.,3.29890219175522));
#35869=CARTESIAN_POINT('Ctrl Pts',(-1.78329283591903,-1.,3.29909749657945));
#35870=CARTESIAN_POINT('Ctrl Pts',(-1.78353803106983,-1.,3.29970549824337));
#35871=CARTESIAN_POINT('Ctrl Pts',(-1.7843238478823,-1.,3.30119637003466));
#35872=CARTESIAN_POINT('Ctrl Pts',(-1.78610045419769,-1.,3.30422155558973));
#35873=CARTESIAN_POINT('Ctrl Pts',(-1.78888832245965,-1.,3.30873412266954));
#35874=CARTESIAN_POINT('Ctrl Pts',(-1.79242331350137,-1.,3.31428038326763));
#35875=CARTESIAN_POINT('Ctrl Pts',(-1.79652817033444,-1.,3.32055355101168));
#35876=CARTESIAN_POINT('Ctrl Pts',(-1.80100380443535,-1.,3.3272108803981));
#35877=CARTESIAN_POINT('Ctrl Pts',(-1.80565802981138,-1.,3.33392460276874));
#35878=CARTESIAN_POINT('Ctrl Pts',(-1.81033399625311,-1.,3.34043216147532));
#35879=CARTESIAN_POINT('Ctrl Pts',(-1.81494618732772,-1.,3.34660014370527));
#35880=CARTESIAN_POINT('Ctrl Pts',(-1.81948458796748,-1.,3.35243086937451));
#35881=CARTESIAN_POINT('Ctrl Pts',(-1.82398496829247,-1.,3.35800801557326));
#35882=CARTESIAN_POINT('Ctrl Pts',(-1.82850752153182,-1.,3.36345722124127));
#35883=CARTESIAN_POINT('Ctrl Pts',(-1.83311391452338,-1.,3.36890396271864));
#35884=CARTESIAN_POINT('Ctrl Pts',(-1.83784072967111,-1.,3.37442462015914));
#35885=CARTESIAN_POINT('Ctrl Pts',(-1.84269016931679,-1.,3.38002968341222));
#35886=CARTESIAN_POINT('Ctrl Pts',(-1.84764441927778,-1.,3.38569092349639));
#35887=CARTESIAN_POINT('Ctrl Pts',(-1.85267433291778,-1.,3.39135802549415));
#35888=CARTESIAN_POINT('Ctrl Pts',(-1.85774972037055,-1.,3.39697816833056));
#35889=CARTESIAN_POINT('Ctrl Pts',(-1.86285057051228,-1.,3.40251742305445));
#35890=CARTESIAN_POINT('Ctrl Pts',(-1.86797231196635,-1.,3.40797080000513));
#35891=CARTESIAN_POINT('Ctrl Pts',(-1.87311957248106,-1.,3.41335043875182));
#35892=CARTESIAN_POINT('Ctrl Pts',(-1.87830245689338,-1.,3.4186785838376));
#35893=CARTESIAN_POINT('Ctrl Pts',(-1.88353205062063,-1.,3.42397908819741));
#35894=CARTESIAN_POINT('Ctrl Pts',(-1.88881571322018,-1.,3.42926852222174));
#35895=CARTESIAN_POINT('Ctrl Pts',(-1.89415420002553,-1.,3.43455074411591));
#35896=CARTESIAN_POINT('Ctrl Pts',(-1.89954426803392,-1.,3.43982185678105));
#35897=CARTESIAN_POINT('Ctrl Pts',(-1.90498026502308,-1.,3.44507323983374));
#35898=CARTESIAN_POINT('Ctrl Pts',(-1.91045605593638,-1.,3.45029522038885));
#35899=CARTESIAN_POINT('Ctrl Pts',(-1.9159669478406,-1.,3.45548074309943));
#35900=CARTESIAN_POINT('Ctrl Pts',(-1.9215111821321,-1.,3.4606282172248));
#35901=CARTESIAN_POINT('Ctrl Pts',(-1.92708888591159,-1.,3.46573953254084));
#35902=CARTESIAN_POINT('Ctrl Pts',(-1.93270136427083,-1.,3.47081872409783));
#35903=CARTESIAN_POINT('Ctrl Pts',(-1.93835026973888,-1.,3.47587040389916));
#35904=CARTESIAN_POINT('Ctrl Pts',(-1.94403680554062,-1.,3.48089825770411));
#35905=CARTESIAN_POINT('Ctrl Pts',(-1.94976096795902,-1.,3.485903616108));
#35906=CARTESIAN_POINT('Ctrl Pts',(-1.95552193112071,-1.,3.49088618670967));
#35907=CARTESIAN_POINT('Ctrl Pts',(-1.96131836776489,-1.,3.49584466573045));
#35908=CARTESIAN_POINT('Ctrl Pts',(-1.9671487972405,-1.,3.50077740176262));
#35909=CARTESIAN_POINT('Ctrl Pts',(-1.9730119116298,-1.,3.505683018611));
#35910=CARTESIAN_POINT('Ctrl Pts',(-1.97890693666316,-1.,3.51056110478334));
#35911=CARTESIAN_POINT('Ctrl Pts',(-1.98483351061066,-1.,3.51541198728362));
#35912=CARTESIAN_POINT('Ctrl Pts',(-1.99079153006143,-1.,3.52023644289195));
#35913=CARTESIAN_POINT('Ctrl Pts',(-1.99678100339305,-1.,3.52503542491745));
#35914=CARTESIAN_POINT('Ctrl Pts',(-2.00280191090341,-1.,3.52980980250181));
#35915=CARTESIAN_POINT('Ctrl Pts',(-2.00885403604685,-1.,3.53456004727321));
#35916=CARTESIAN_POINT('Ctrl Pts',(-2.0149369884727,-1.,3.53928627453503));
#35917=CARTESIAN_POINT('Ctrl Pts',(-2.0210502798303,-1.,3.54398838254011));
#35918=CARTESIAN_POINT('Ctrl Pts',(-2.02719338376144,-1.,3.54866616282173));
#35919=CARTESIAN_POINT('Ctrl Pts',(-2.03336579658174,-1.,3.55331941294018));
#35920=CARTESIAN_POINT('Ctrl Pts',(-2.03956711120099,-1.,3.55794807265052));
#35921=CARTESIAN_POINT('Ctrl Pts',(-2.04579702159056,-1.,3.5625522387181));
#35922=CARTESIAN_POINT('Ctrl Pts',(-2.0520552817309,-1.,3.56713209978207));
#35923=CARTESIAN_POINT('Ctrl Pts',(-2.05834167687523,-1.,3.57168789423507));
#35924=CARTESIAN_POINT('Ctrl Pts',(-2.06465599229174,-1.,3.576219862243));
#35925=CARTESIAN_POINT('Ctrl Pts',(-2.07099797605747,-1.,3.58072819250442));
#35926=CARTESIAN_POINT('Ctrl Pts',(-2.07736732842117,-1.,3.58521300039299));
#35927=CARTESIAN_POINT('Ctrl Pts',(-2.08376373048756,-1.,3.58967435355088));
#35928=CARTESIAN_POINT('Ctrl Pts',(-2.09018686331416,-1.,3.59411228625588));
#35929=CARTESIAN_POINT('Ctrl Pts',(-2.09663642986631,-1.,3.59852681775485));
#35930=CARTESIAN_POINT('Ctrl Pts',(-2.1031121772821,-1.,3.60291797088734));
#35931=CARTESIAN_POINT('Ctrl Pts',(-2.10961391334462,-1.,3.60728578532601));
#35932=CARTESIAN_POINT('Ctrl Pts',(-2.11614149815106,-1.,3.61163030609447));
#35933=CARTESIAN_POINT('Ctrl Pts',(-2.12138417126355,-1.,3.61508732216891));
#35934=CARTESIAN_POINT('Ctrl Pts',(-2.12532774376758,-1.,3.61766963590482));
#35935=CARTESIAN_POINT('Ctrl Pts',(-2.12796193131368,-1.,3.61938653649098));
#35936=CARTESIAN_POINT('Ctrl Pts',(-2.12928030988903,-1.,3.62024382630768));
#35937=CARTESIAN_POINT('',(-2.25898783642071,-1.,3.54075895182139));
#35938=CARTESIAN_POINT('',(-2.12928030988903,-1.,3.62024382630768));
#35939=CARTESIAN_POINT('',(-2.1297112484669,-1.,3.08655633322212));
#35940=CARTESIAN_POINT('Ctrl Pts',(-2.25898783642071,-1.,3.54075895182139));
#35941=CARTESIAN_POINT('Ctrl Pts',(-2.2588225169468,-1.,3.53919506647335));
#35942=CARTESIAN_POINT('Ctrl Pts',(-2.25848864343951,-1.,3.53606853162228));
#35943=CARTESIAN_POINT('Ctrl Pts',(-2.25797812950104,-1.,3.53138243688262));
#35944=CARTESIAN_POINT('Ctrl Pts',(-2.25727802940898,-1.,3.52514172847711));
#35945=CARTESIAN_POINT('Ctrl Pts',(-2.25637049455044,-1.,3.51735323667612));
#35946=CARTESIAN_POINT('Ctrl Pts',(-2.25543046979799,-1.,3.50957720117341));
#35947=CARTESIAN_POINT('Ctrl Pts',(-2.25445785151868,-1.,3.50181372617971));
#35948=CARTESIAN_POINT('Ctrl Pts',(-2.2534525170976,-1.,3.49406296494791));
#35949=CARTESIAN_POINT('Ctrl Pts',(-2.25241433138695,-1.,3.48632513240961));
#35950=CARTESIAN_POINT('Ctrl Pts',(-2.25134314238687,-1.,3.47860048448691));
#35951=CARTESIAN_POINT('Ctrl Pts',(-2.25023877475942,-1.,3.47088928979888));
#35952=CARTESIAN_POINT('Ctrl Pts',(-2.2491010234604,-1.,3.46319180177573));
#35953=CARTESIAN_POINT('Ctrl Pts',(-2.2479296496077,-1.,3.45550823512049));
#35954=CARTESIAN_POINT('Ctrl Pts',(-2.2467243706995,-1.,3.44783872863151));
#35955=CARTESIAN_POINT('Ctrl Pts',(-2.24548487526022,-1.,3.4401833646032));
#35956=CARTESIAN_POINT('Ctrl Pts',(-2.24421085338727,-1.,3.43254222614803));
#35957=CARTESIAN_POINT('Ctrl Pts',(-2.24290202531101,-1.,3.42491544683008));
#35958=CARTESIAN_POINT('Ctrl Pts',(-2.24155816587844,-1.,3.41730325539172));
#35959=CARTESIAN_POINT('Ctrl Pts',(-2.24017914395289,-1.,3.40970604190328));
#35960=CARTESIAN_POINT('Ctrl Pts',(-2.2387649112415,-1.,3.40212434705647));
#35961=CARTESIAN_POINT('Ctrl Pts',(-2.23731541452791,-1.,3.39455873448189));
#35962=CARTESIAN_POINT('Ctrl Pts',(-2.23583052276308,-1.,3.38700968549563));
#35963=CARTESIAN_POINT('Ctrl Pts',(-2.23430995599561,-1.,3.37947749555632));
#35964=CARTESIAN_POINT('Ctrl Pts',(-2.23275319569221,-1.,3.37196214349304));
#35965=CARTESIAN_POINT('Ctrl Pts',(-2.23115945849739,-1.,3.36446325227848));
#35966=CARTESIAN_POINT('Ctrl Pts',(-2.22952789880982,-1.,3.35698038165483));
#35967=CARTESIAN_POINT('Ctrl Pts',(-2.22785777756576,-1.,3.34951327111096));
#35968=CARTESIAN_POINT('Ctrl Pts',(-2.22614863918047,-1.,3.34206209449375));
#35969=CARTESIAN_POINT('Ctrl Pts',(-2.22440049878511,-1.,3.33462772849598));
#35970=CARTESIAN_POINT('Ctrl Pts',(-2.22261398879635,-1.,3.3272119632604));
#35971=CARTESIAN_POINT('Ctrl Pts',(-2.22078990842776,-1.,3.31981686778022));
#35972=CARTESIAN_POINT('Ctrl Pts',(-2.21892881679086,-1.,3.31244421655666));
#35973=CARTESIAN_POINT('Ctrl Pts',(-2.21703059947836,-1.,3.30509487819569));
#35974=CARTESIAN_POINT('Ctrl Pts',(-2.21509406923368,-1.,3.29776825193159));
#35975=CARTESIAN_POINT('Ctrl Pts',(-2.21311648827391,-1.,3.29046159238343));
#35976=CARTESIAN_POINT('Ctrl Pts',(-2.21109449750641,-1.,3.28317133333131));
#35977=CARTESIAN_POINT('Ctrl Pts',(-2.2090250941743,-1.,3.2758944800554));
#35978=CARTESIAN_POINT('Ctrl Pts',(-2.20690665217743,-1.,3.26863006136782));
#35979=CARTESIAN_POINT('Ctrl Pts',(-2.20473979048678,-1.,3.26138036637705));
#35980=CARTESIAN_POINT('Ctrl Pts',(-2.20252866491545,-1.,3.25415277957775));
#35981=CARTESIAN_POINT('Ctrl Pts',(-2.20027910880981,-1.,3.24695715874338));
#35982=CARTESIAN_POINT('Ctrl Pts',(-2.19799623693253,-1.,3.23980245361308));
#35983=CARTESIAN_POINT('Ctrl Pts',(-2.19568204933168,-1.,3.23269332296933));
#35984=CARTESIAN_POINT('Ctrl Pts',(-2.19333345123538,-1.,3.22562734221646));
#35985=CARTESIAN_POINT('Ctrl Pts',(-2.19093901948667,-1.,3.21859043114095));
#35986=CARTESIAN_POINT('Ctrl Pts',(-2.18848253363901,-1.,3.21156188355769));
#35987=CARTESIAN_POINT('Ctrl Pts',(-2.18594876115934,-1.,3.20452259717976));
#35988=CARTESIAN_POINT('Ctrl Pts',(-2.18332898656602,-1.,3.19746293740411));
#35989=CARTESIAN_POINT('Ctrl Pts',(-2.18062558031778,-1.,3.19038924261573));
#35990=CARTESIAN_POINT('Ctrl Pts',(-2.17785968847142,-1.,3.18333474627807));
#35991=CARTESIAN_POINT('Ctrl Pts',(-2.17506466903694,-1.,3.17635032802523));
#35992=CARTESIAN_POINT('Ctrl Pts',(-2.17227212063817,-1.,3.16948480019497));
#35993=CARTESIAN_POINT('Ctrl Pts',(-2.16949910801219,-1.,3.16276685102972));
#35994=CARTESIAN_POINT('Ctrl Pts',(-2.1667372844769,-1.,3.15618975593656));
#35995=CARTESIAN_POINT('Ctrl Pts',(-2.16393520288072,-1.,3.14968624389054));
#35996=CARTESIAN_POINT('Ctrl Pts',(-2.16100905914435,-1.,3.14314440427022));
#35997=CARTESIAN_POINT('Ctrl Pts',(-2.15787423530676,-1.,3.13645356563038));
#35998=CARTESIAN_POINT('Ctrl Pts',(-2.1544724138292,-1.,3.12954386795646));
#35999=CARTESIAN_POINT('Ctrl Pts',(-2.15079698090585,-1.,3.12242318151938));
#36000=CARTESIAN_POINT('Ctrl Pts',(-2.14692798457532,-1.,3.11522827016855));
#36001=CARTESIAN_POINT('Ctrl Pts',(-2.14302815601973,-1.,3.10821808668859));
#36002=CARTESIAN_POINT('Ctrl Pts',(-2.13930228863751,-1.,3.10171267391049));
#36003=CARTESIAN_POINT('Ctrl Pts',(-2.13596538661048,-1.,3.0960450242104));
#36004=CARTESIAN_POINT('Ctrl Pts',(-2.13321032560893,-1.,3.09151235281963));
#36005=CARTESIAN_POINT('Ctrl Pts',(-2.13132142793017,-1.,3.08855597949761));
#36006=CARTESIAN_POINT('Ctrl Pts',(-2.13034980480424,-1.,3.08717896996099));
#36007=CARTESIAN_POINT('Ctrl Pts',(-2.12991938762374,-1.,3.08668447250322));
#36008=CARTESIAN_POINT('Ctrl Pts',(-2.1297578506149,-1.,3.08657131089497));
#36009=CARTESIAN_POINT('Ctrl Pts',(-2.1297112484669,-1.,3.08655633322212));
#36010=CARTESIAN_POINT('',(-2.27737254473378,-1.,2.97927412174388));
#36011=CARTESIAN_POINT('Origin',(0.,-1.,0.));
#36012=CARTESIAN_POINT('',(-2.66939624221984,-1.,3.24257979115744));
#36013=CARTESIAN_POINT('Ctrl Pts',(-2.27737254473378,-1.,2.97927412174388));
#36014=CARTESIAN_POINT('Ctrl Pts',(-2.27737238849212,-1.,2.97932307137589));
#36015=CARTESIAN_POINT('Ctrl Pts',(-2.27743009389704,-1.,2.97951167106106));
#36016=CARTESIAN_POINT('Ctrl Pts',(-2.27776738270369,-1.,2.98007383024333));
#36017=CARTESIAN_POINT('Ctrl Pts',(-2.27877674853833,-1.,2.98142341809623));
#36018=CARTESIAN_POINT('Ctrl Pts',(-2.28100472516582,-1.,2.98413343613858));
#36019=CARTESIAN_POINT('Ctrl Pts',(-2.28446419116036,-1.,2.98815432734929));
#36020=CARTESIAN_POINT('Ctrl Pts',(-2.28882328690601,-1.,2.9930793098434));
#36021=CARTESIAN_POINT('Ctrl Pts',(-2.29385894577999,-1.,2.99863310340004));
#36022=CARTESIAN_POINT('Ctrl Pts',(-2.29932091315939,-1.,3.00450832658822));
#36023=CARTESIAN_POINT('Ctrl Pts',(-2.30496809486529,-1.,3.01041131063882));
#36024=CARTESIAN_POINT('Ctrl Pts',(-2.31060449886577,-1.,3.01610726819019));
#36025=CARTESIAN_POINT('Ctrl Pts',(-2.31612479121528,-1.,3.02147780668029));
#36026=CARTESIAN_POINT('Ctrl Pts',(-2.32151944306299,-1.,3.02652678416478));
#36027=CARTESIAN_POINT('Ctrl Pts',(-2.32683687412027,-1.,3.03133125185047));
#36028=CARTESIAN_POINT('Ctrl Pts',(-2.33215619079807,-1.,3.03600588555765));
#36029=CARTESIAN_POINT('Ctrl Pts',(-2.33755792953726,-1.,3.04066496998569));
#36030=CARTESIAN_POINT('Ctrl Pts',(-2.3430901708402,-1.,3.04537822217311));
#36031=CARTESIAN_POINT('Ctrl Pts',(-2.34875673090816,-1.,3.05015565829976));
#36032=CARTESIAN_POINT('Ctrl Pts',(-2.35453559889506,-1.,3.05497218368188));
#36033=CARTESIAN_POINT('Ctrl Pts',(-2.36039011602084,-1.,3.05978266240056));
#36034=CARTESIAN_POINT('Ctrl Pts',(-2.36628220107001,-1.,3.06453964643152));
#36035=CARTESIAN_POINT('Ctrl Pts',(-2.37218678163157,-1.,3.06921275497472));
#36036=CARTESIAN_POINT('Ctrl Pts',(-2.37809856205524,-1.,3.07379777492133));
#36037=CARTESIAN_POINT('Ctrl Pts',(-2.38402401216107,-1.,3.07830597244301));
#36038=CARTESIAN_POINT('Ctrl Pts',(-2.38997659219192,-1.,3.08275773747083));
#36039=CARTESIAN_POINT('Ctrl Pts',(-2.39597098250635,-1.,3.08717489512919));
#36040=CARTESIAN_POINT('Ctrl Pts',(-2.40201704423352,-1.,3.09157266051115));
#36041=CARTESIAN_POINT('Ctrl Pts',(-2.40811612696382,-1.,3.09595472616093));
#36042=CARTESIAN_POINT('Ctrl Pts',(-2.41426441798067,-1.,3.10031775027683));
#36043=CARTESIAN_POINT('Ctrl Pts',(-2.42045498612494,-1.,3.10465410280902));
#36044=CARTESIAN_POINT('Ctrl Pts',(-2.42668025870013,-1.,3.10895518969592));
#36045=CARTESIAN_POINT('Ctrl Pts',(-2.4329344968514,-1.,3.11321477659012));
#36046=CARTESIAN_POINT('Ctrl Pts',(-2.43921571477975,-1.,3.11743156744182));
#36047=CARTESIAN_POINT('Ctrl Pts',(-2.44552433364716,-1.,3.12160740887768));
#36048=CARTESIAN_POINT('Ctrl Pts',(-2.45186227369848,-1.,3.12574608210849));
#36049=CARTESIAN_POINT('Ctrl Pts',(-2.45823188859367,-1.,3.12985188384372));
#36050=CARTESIAN_POINT('Ctrl Pts',(-2.4646349433237,-1.,3.13392826623902));
#36051=CARTESIAN_POINT('Ctrl Pts',(-2.47107164236827,-1.,3.13797654408931));
#36052=CARTESIAN_POINT('Ctrl Pts',(-2.47754112428028,-1.,3.14199655778845));
#36053=CARTESIAN_POINT('Ctrl Pts',(-2.48404187418376,-1.,3.1459872272388));
#36054=CARTESIAN_POINT('Ctrl Pts',(-2.49057217131985,-1.,3.14994715298903));
#36055=CARTESIAN_POINT('Ctrl Pts',(-2.49713050858911,-1.,3.15387518039064));
#36056=CARTESIAN_POINT('Ctrl Pts',(-2.50371605688287,-1.,3.15777102413998));
#36057=CARTESIAN_POINT('Ctrl Pts',(-2.51032851007939,-1.,3.16163506380211));
#36058=CARTESIAN_POINT('Ctrl Pts',(-2.51696788755616,-1.,3.16546808277069));
#36059=CARTESIAN_POINT('Ctrl Pts',(-2.523634346718,-1.,3.16927102130751));
#36060=CARTESIAN_POINT('Ctrl Pts',(-2.5303280040691,-1.,3.17304474093574));
#36061=CARTESIAN_POINT('Ctrl Pts',(-2.53704871950871,-1.,3.17678974135225));
#36062=CARTESIAN_POINT('Ctrl Pts',(-2.54379612552948,-1.,3.18050619750515));
#36063=CARTESIAN_POINT('Ctrl Pts',(-2.55056972387638,-1.,3.18419408529482));
#36064=CARTESIAN_POINT('Ctrl Pts',(-2.55736896206016,-1.,3.1878532811617));
#36065=CARTESIAN_POINT('Ctrl Pts',(-2.56419331092909,-1.,3.19148366395201));
#36066=CARTESIAN_POINT('Ctrl Pts',(-2.57104235898053,-1.,3.19508523784548));
#36067=CARTESIAN_POINT('Ctrl Pts',(-2.577915819091,-1.,3.19865814628955));
#36068=CARTESIAN_POINT('Ctrl Pts',(-2.58481347777953,-1.,3.20220261408685));
#36069=CARTESIAN_POINT('Ctrl Pts',(-2.59173516023605,-1.,3.20571891028879));
#36070=CARTESIAN_POINT('Ctrl Pts',(-2.59868069194267,-1.,3.2092073056959));
#36071=CARTESIAN_POINT('Ctrl Pts',(-2.60564985359699,-1.,3.21266802609297));
#36072=CARTESIAN_POINT('Ctrl Pts',(-2.61264236718662,-1.,3.21610123232465));
#36073=CARTESIAN_POINT('Ctrl Pts',(-2.61965792832396,-1.,3.21950704108654));
#36074=CARTESIAN_POINT('Ctrl Pts',(-2.62669622735548,-1.,3.222885536128));
#36075=CARTESIAN_POINT('Ctrl Pts',(-2.63375697391438,-1.,3.22623678292539));
#36076=CARTESIAN_POINT('Ctrl Pts',(-2.64083992182478,-1.,3.2295608435934));
#36077=CARTESIAN_POINT('Ctrl Pts',(-2.64794488744246,-1.,3.23285778738558));
#36078=CARTESIAN_POINT('Ctrl Pts',(-2.6550717396303,-1.,3.23612768065687));
#36079=CARTESIAN_POINT('Ctrl Pts',(-2.6607906631973,-1.,3.23872200036311));
#36080=CARTESIAN_POINT('Ctrl Pts',(-2.66508964664767,-1.,3.24065561087681));
#36081=CARTESIAN_POINT('Ctrl Pts',(-2.66795998539861,-1.,3.24193929584813));
#36082=CARTESIAN_POINT('Ctrl Pts',(-2.66939624221984,-1.,3.24257979115744));
#36083=CARTESIAN_POINT('',(-2.78507268004356,-1.,3.14378277984898));
#36084=CARTESIAN_POINT('',(-2.66939624221984,-1.,3.24257979115744));
#36085=CARTESIAN_POINT('',(-2.58633475774921,-1.,2.71539546306948));
#36086=CARTESIAN_POINT('Ctrl Pts',(-2.78507268004356,-1.,3.14378277984898));
#36087=CARTESIAN_POINT('Ctrl Pts',(-2.7846647503589,-1.,3.14226401018816));
#36088=CARTESIAN_POINT('Ctrl Pts',(-2.78384588958166,-1.,3.13922819749279));
#36089=CARTESIAN_POINT('Ctrl Pts',(-2.78260859419319,-1.,3.13467965833037));
#36090=CARTESIAN_POINT('Ctrl Pts',(-2.78094085161413,-1.,3.12862530318457));
#36091=CARTESIAN_POINT('Ctrl Pts',(-2.77882610146731,-1.,3.12107467037201));
#36092=CARTESIAN_POINT('Ctrl Pts',(-2.77668121002545,-1.,3.11354142303921));
#36093=CARTESIAN_POINT('Ctrl Pts',(-2.77450609123362,-1.,3.10602568032564));
#36094=CARTESIAN_POINT('Ctrl Pts',(-2.77230064796057,-1.,3.0985276127786));
#36095=CARTESIAN_POINT('Ctrl Pts',(-2.7700647803451,-1.,3.09104745382531));
#36096=CARTESIAN_POINT('Ctrl Pts',(-2.76779837829373,-1.,3.08358548001504));
#36097=CARTESIAN_POINT('Ctrl Pts',(-2.76550131064852,-1.,3.07614198408862));
#36098=CARTESIAN_POINT('Ctrl Pts',(-2.76317341453493,-1.,3.0687172484321));
#36099=CARTESIAN_POINT('Ctrl Pts',(-2.76081448759882,-1.,3.06131152247454));
#36100=CARTESIAN_POINT('Ctrl Pts',(-2.75842427252931,-1.,3.05392498749847));
#36101=CARTESIAN_POINT('Ctrl Pts',(-2.75600247455925,-1.,3.04655777351067));
#36102=CARTESIAN_POINT('Ctrl Pts',(-2.75354880060314,-1.,3.03921001107977));
#36103=CARTESIAN_POINT('Ctrl Pts',(-2.75106299522979,-1.,3.03188187589107));
#36104=CARTESIAN_POINT('Ctrl Pts',(-2.7485448718414,-1.,3.02457362909245));
#36105=CARTESIAN_POINT('Ctrl Pts',(-2.74599436193625,-1.,3.01728567646611));
#36106=CARTESIAN_POINT('Ctrl Pts',(-2.74341150239887,-1.,3.01001855960162));
#36107=CARTESIAN_POINT('Ctrl Pts',(-2.74079632883931,-1.,3.00277284351521));
#36108=CARTESIAN_POINT('Ctrl Pts',(-2.73814878711641,-1.,2.99554902409778));
#36109=CARTESIAN_POINT('Ctrl Pts',(-2.73546864694536,-1.,2.9883474369644));
#36110=CARTESIAN_POINT('Ctrl Pts',(-2.73275539286497,-1.,2.98116814232129));
#36111=CARTESIAN_POINT('Ctrl Pts',(-2.73000819218414,-1.,2.97401089032677));
#36112=CARTESIAN_POINT('Ctrl Pts',(-2.72722614084076,-1.,2.96687537842451));
#36113=CARTESIAN_POINT('Ctrl Pts',(-2.72440846811729,-1.,2.95976146492576));
#36114=CARTESIAN_POINT('Ctrl Pts',(-2.72155475123364,-1.,2.95266939280621));
#36115=CARTESIAN_POINT('Ctrl Pts',(-2.71866514227965,-1.,2.94560002559806));
#36116=CARTESIAN_POINT('Ctrl Pts',(-2.71574054592591,-1.,2.93855503247266));
#36117=CARTESIAN_POINT('Ctrl Pts',(-2.71278207520817,-1.,2.93153633192595));
#36118=CARTESIAN_POINT('Ctrl Pts',(-2.70979055994754,-1.,2.92454558914778));
#36119=CARTESIAN_POINT('Ctrl Pts',(-2.70676602302518,-1.,2.91758367994737));
#36120=CARTESIAN_POINT('Ctrl Pts',(-2.70370719782113,-1.,2.91065019668329));
#36121=CARTESIAN_POINT('Ctrl Pts',(-2.70061095078692,-1.,2.90374285605838));
#36122=CARTESIAN_POINT('Ctrl Pts',(-2.69747340630625,-1.,2.89685866123671));
#36123=CARTESIAN_POINT('Ctrl Pts',(-2.69429113011374,-1.,2.88999512410309));
#36124=CARTESIAN_POINT('Ctrl Pts',(-2.69106236420198,-1.,2.88315153980466));
#36125=CARTESIAN_POINT('Ctrl Pts',(-2.68778807801686,-1.,2.8763300724388));
#36126=CARTESIAN_POINT('Ctrl Pts',(-2.68447353139599,-1.,2.86953736547238));
#36127=CARTESIAN_POINT('Ctrl Pts',(-2.68112602796308,-1.,2.86278224277689));
#36128=CARTESIAN_POINT('Ctrl Pts',(-2.67775201955724,-1.,2.85607274378018));
#36129=CARTESIAN_POINT('Ctrl Pts',(-2.67435421039677,-1.,2.84941315703092));
#36130=CARTESIAN_POINT('Ctrl Pts',(-2.67092916452125,-1.,2.84280157191323));
#36131=CARTESIAN_POINT('Ctrl Pts',(-2.66746339678107,-1.,2.83622586853982));
#36132=CARTESIAN_POINT('Ctrl Pts',(-2.6639376472693,-1.,2.82966813308998));
#36133=CARTESIAN_POINT('Ctrl Pts',(-2.66033388273461,-1.,2.82311188135078));
#36134=CARTESIAN_POINT('Ctrl Pts',(-2.65664198781344,-1.,2.81654896073883));
#36135=CARTESIAN_POINT('Ctrl Pts',(-2.65286529532208,-1.,2.80998526078165));
#36136=CARTESIAN_POINT('Ctrl Pts',(-2.64902988983337,-1.,2.80345029781152));
#36137=CARTESIAN_POINT('Ctrl Pts',(-2.6451766779932,-1.,2.79698910670736));
#36138=CARTESIAN_POINT('Ctrl Pts',(-2.64134450532584,-1.,2.79064495573224));
#36139=CARTESIAN_POINT('Ctrl Pts',(-2.637554714303,-1.,2.78444351041571));
#36140=CARTESIAN_POINT('Ctrl Pts',(-2.63379800904599,-1.,2.77837943466449));
#36141=CARTESIAN_POINT('Ctrl Pts',(-2.63001305229625,-1.,2.77239433377921));
#36142=CARTESIAN_POINT('Ctrl Pts',(-2.62609956506355,-1.,2.76639078479021));
#36143=CARTESIAN_POINT('Ctrl Pts',(-2.62195665834605,-1.,2.76027271596686));
#36144=CARTESIAN_POINT('Ctrl Pts',(-2.61751580407667,-1.,2.7539802502603));
#36145=CARTESIAN_POINT('Ctrl Pts',(-2.61277170105813,-1.,2.74752219567252));
#36146=CARTESIAN_POINT('Ctrl Pts',(-2.60782480638448,-1.,2.7410211099909));
#36147=CARTESIAN_POINT('Ctrl Pts',(-2.60287635688728,-1.,2.73470730109615));
#36148=CARTESIAN_POINT('Ctrl Pts',(-2.59817869034746,-1.,2.7288648348152));
#36149=CARTESIAN_POINT('Ctrl Pts',(-2.59399625537278,-1.,2.72378896977134));
#36150=CARTESIAN_POINT('Ctrl Pts',(-2.59056604771971,-1.,2.71974308958086));
#36151=CARTESIAN_POINT('Ctrl Pts',(-2.58823792682672,-1.,2.71711860281815));
#36152=CARTESIAN_POINT('Ctrl Pts',(-2.58706285424358,-1.,2.71591054189786));
#36153=CARTESIAN_POINT('Ctrl Pts',(-2.58656037976753,-1.,2.71548946460575));
#36154=CARTESIAN_POINT('Ctrl Pts',(-2.58638312917168,-1.,2.71540296616024));
#36155=CARTESIAN_POINT('Ctrl Pts',(-2.58633475774921,-1.,2.71539546306948));
#36156=CARTESIAN_POINT('',(-2.71539546306824,-1.,2.58633475775051));
#36157=CARTESIAN_POINT('Origin',(0.,-1.,0.));
#36158=CARTESIAN_POINT('',(-3.14378277984898,-1.,2.78507268004356));
#36159=CARTESIAN_POINT('Ctrl Pts',(-2.71539546306824,-1.,2.58633475775051));
#36160=CARTESIAN_POINT('Ctrl Pts',(-2.71540296615967,-1.,2.58638312917291));
#36161=CARTESIAN_POINT('Ctrl Pts',(-2.71548946460616,-1.,2.58656037976884));
#36162=CARTESIAN_POINT('Ctrl Pts',(-2.71591054189884,-1.,2.58706285424469));
#36163=CARTESIAN_POINT('Ctrl Pts',(-2.7171186028189,-1.,2.58823792682724));
#36164=CARTESIAN_POINT('Ctrl Pts',(-2.7197430895797,-1.,2.59056604771863));
#36165=CARTESIAN_POINT('Ctrl Pts',(-2.72378896977273,-1.,2.59399625537407));
#36166=CARTESIAN_POINT('Ctrl Pts',(-2.72886483481804,-1.,2.5981786903501));
#36167=CARTESIAN_POINT('Ctrl Pts',(-2.73470730109906,-1.,2.60287635689));
#36168=CARTESIAN_POINT('Ctrl Pts',(-2.74102110999284,-1.,2.60782480638629));
#36169=CARTESIAN_POINT('Ctrl Pts',(-2.74752219567307,-1.,2.61277170105864));
#36170=CARTESIAN_POINT('Ctrl Pts',(-2.75398025025967,-1.,2.61751580407608));
#36171=CARTESIAN_POINT('Ctrl Pts',(-2.76027271596564,-1.,2.62195665834491));
#36172=CARTESIAN_POINT('Ctrl Pts',(-2.76639078478898,-1.,2.6260995650624));
#36173=CARTESIAN_POINT('Ctrl Pts',(-2.77239433377839,-1.,2.63001305229548));
#36174=CARTESIAN_POINT('Ctrl Pts',(-2.77837943466423,-1.,2.63379800904575));
#36175=CARTESIAN_POINT('Ctrl Pts',(-2.78444351041594,-1.,2.63755471430322));
#36176=CARTESIAN_POINT('Ctrl Pts',(-2.79064495573275,-1.,2.64134450532632));
#36177=CARTESIAN_POINT('Ctrl Pts',(-2.7969891067079,-1.,2.6451766779937));
#36178=CARTESIAN_POINT('Ctrl Pts',(-2.80345029781191,-1.,2.64902988983373));
#36179=CARTESIAN_POINT('Ctrl Pts',(-2.80998526078179,-1.,2.65286529532221));
#36180=CARTESIAN_POINT('Ctrl Pts',(-2.81654896073874,-1.,2.65664198781335));
#36181=CARTESIAN_POINT('Ctrl Pts',(-2.82311188135053,-1.,2.66033388273437));
#36182=CARTESIAN_POINT('Ctrl Pts',(-2.82966813308969,-1.,2.66393764726902));
#36183=CARTESIAN_POINT('Ctrl Pts',(-2.8362258685396,-1.,2.66746339678085));
#36184=CARTESIAN_POINT('Ctrl Pts',(-2.84280157191314,-1.,2.67092916452117));
#36185=CARTESIAN_POINT('Ctrl Pts',(-2.84941315703096,-1.,2.67435421039682));
#36186=CARTESIAN_POINT('Ctrl Pts',(-2.85607274378031,-1.,2.67775201955736));
#36187=CARTESIAN_POINT('Ctrl Pts',(-2.86278224277705,-1.,2.68112602796323));
#36188=CARTESIAN_POINT('Ctrl Pts',(-2.8695373654725,-1.,2.68447353139611));
#36189=CARTESIAN_POINT('Ctrl Pts',(-2.87633007243885,-1.,2.68778807801691));
#36190=CARTESIAN_POINT('Ctrl Pts',(-2.88315153980464,-1.,2.69106236420197));
#36191=CARTESIAN_POINT('Ctrl Pts',(-2.88999512410304,-1.,2.69429113011369));
#36192=CARTESIAN_POINT('Ctrl Pts',(-2.89685866123668,-1.,2.69747340630621));
#36193=CARTESIAN_POINT('Ctrl Pts',(-2.90374285605839,-1.,2.70061095078692));
#36194=CARTESIAN_POINT('Ctrl Pts',(-2.91065019668331,-1.,2.70370719782114));
#36195=CARTESIAN_POINT('Ctrl Pts',(-2.91758367994738,-1.,2.70676602302518));
#36196=CARTESIAN_POINT('Ctrl Pts',(-2.92454558914774,-1.,2.70979055994751));
#36197=CARTESIAN_POINT('Ctrl Pts',(-2.93153633192583,-1.,2.71278207520807));
#36198=CARTESIAN_POINT('Ctrl Pts',(-2.93855503247248,-1.,2.71574054592575));
#36199=CARTESIAN_POINT('Ctrl Pts',(-2.94560002559789,-1.,2.71866514227952));
#36200=CARTESIAN_POINT('Ctrl Pts',(-2.95266939280617,-1.,2.72155475123361));
#36201=CARTESIAN_POINT('Ctrl Pts',(-2.95976146492595,-1.,2.72440846811745));
#36202=CARTESIAN_POINT('Ctrl Pts',(-2.96687537842492,-1.,2.72722614084112));
#36203=CARTESIAN_POINT('Ctrl Pts',(-2.97401089032729,-1.,2.7300081921846));
#36204=CARTESIAN_POINT('Ctrl Pts',(-2.98116814232175,-1.,2.73275539286537));
#36205=CARTESIAN_POINT('Ctrl Pts',(-2.98834743696455,-1.,2.73546864694548));
#36206=CARTESIAN_POINT('Ctrl Pts',(-2.99554902409741,-1.,2.73814878711609));
#36207=CARTESIAN_POINT('Ctrl Pts',(-3.00277284351431,-1.,2.74079632883852));
#36208=CARTESIAN_POINT('Ctrl Pts',(-3.01001855960041,-1.,2.7434115023978));
#36209=CARTESIAN_POINT('Ctrl Pts',(-3.01728567646502,-1.,2.74599436193528));
#36210=CARTESIAN_POINT('Ctrl Pts',(-3.02457362909199,-1.,2.74854487184099));
#36211=CARTESIAN_POINT('Ctrl Pts',(-3.03188187589168,-1.,2.75106299523032));
#36212=CARTESIAN_POINT('Ctrl Pts',(-3.03921001108158,-1.,2.75354880060473));
#36213=CARTESIAN_POINT('Ctrl Pts',(-3.04655777351333,-1.,2.7560024745616));
#36214=CARTESIAN_POINT('Ctrl Pts',(-3.05392498750112,-1.,2.75842427253164));
#36215=CARTESIAN_POINT('Ctrl Pts',(-3.06131152247599,-1.,2.76081448760011));
#36216=CARTESIAN_POINT('Ctrl Pts',(-3.06871724843121,-1.,2.76317341453415));
#36217=CARTESIAN_POINT('Ctrl Pts',(-3.07614198408488,-1.,2.76550131064522));
#36218=CARTESIAN_POINT('Ctrl Pts',(-3.08358548000904,-1.,2.76779837828843));
#36219=CARTESIAN_POINT('Ctrl Pts',(-3.09104745381882,-1.,2.77006478033937));
#36220=CARTESIAN_POINT('Ctrl Pts',(-3.09852761277432,-1.,2.77230064795679));
#36221=CARTESIAN_POINT('Ctrl Pts',(-3.10602568032641,-1.,2.7745060912343));
#36222=CARTESIAN_POINT('Ctrl Pts',(-3.11354142304692,-1.,2.77668121003225));
#36223=CARTESIAN_POINT('Ctrl Pts',(-3.12107467038623,-1.,2.77882610147986));
#36224=CARTESIAN_POINT('Ctrl Pts',(-3.12862530320194,-1.,2.78094085162947));
#36225=CARTESIAN_POINT('Ctrl Pts',(-3.1346796583452,-1.,2.78260859420629));
#36226=CARTESIAN_POINT('Ctrl Pts',(-3.13922819750185,-1.,2.78384588958965));
#36227=CARTESIAN_POINT('Ctrl Pts',(-3.14226401019149,-1.,2.78466475036183));
#36228=CARTESIAN_POINT('Ctrl Pts',(-3.14378277984898,-1.,2.78507268004356));
#36229=CARTESIAN_POINT('',(-3.24257979115744,-1.,2.66939624221984));
#36230=CARTESIAN_POINT('',(-3.14378277984898,-1.,2.78507268004356));
#36231=CARTESIAN_POINT('',(-2.97927412174279,-1.,2.27737254473521));
#36232=CARTESIAN_POINT('Ctrl Pts',(-3.24257979115744,-1.,2.66939624221984));
#36233=CARTESIAN_POINT('Ctrl Pts',(-3.24193929584471,-1.,2.66795998539579));
#36234=CARTESIAN_POINT('Ctrl Pts',(-3.24065561086749,-1.,2.66508964663997));
#36235=CARTESIAN_POINT('Ctrl Pts',(-3.23872200034785,-1.,2.6607906631847));
#36236=CARTESIAN_POINT('Ctrl Pts',(-3.236127680639,-1.,2.65507173961555));
#36237=CARTESIAN_POINT('Ctrl Pts',(-3.23285778737096,-1.,2.64794488743038));
#36238=CARTESIAN_POINT('Ctrl Pts',(-3.22956084358547,-1.,2.64083992181823));
#36239=CARTESIAN_POINT('Ctrl Pts',(-3.2262367829246,-1.,2.63375697391372));
#36240=CARTESIAN_POINT('Ctrl Pts',(-3.2228855361324,-1.,2.62669622735912));
#36241=CARTESIAN_POINT('Ctrl Pts',(-3.21950704109321,-1.,2.61965792832947));
#36242=CARTESIAN_POINT('Ctrl Pts',(-3.21610123233082,-1.,2.61264236719171));
#36243=CARTESIAN_POINT('Ctrl Pts',(-3.21266802609682,-1.,2.60564985360017));
#36244=CARTESIAN_POINT('Ctrl Pts',(-3.20920730569681,-1.,2.59868069194342));
#36245=CARTESIAN_POINT('Ctrl Pts',(-3.2057189102873,-1.,2.59173516023481));
#36246=CARTESIAN_POINT('Ctrl Pts',(-3.20220261408414,-1.,2.58481347777729));
#36247=CARTESIAN_POINT('Ctrl Pts',(-3.19865814628682,-1.,2.57791581908875));
#36248=CARTESIAN_POINT('Ctrl Pts',(-3.19508523784363,-1.,2.57104235897899));
#36249=CARTESIAN_POINT('Ctrl Pts',(-3.19148366395139,-1.,2.56419331092858));
#36250=CARTESIAN_POINT('Ctrl Pts',(-3.18785328116218,-1.,2.55736896206056));
#36251=CARTESIAN_POINT('Ctrl Pts',(-3.18419408529594,-1.,2.55056972387731));
#36252=CARTESIAN_POINT('Ctrl Pts',(-3.1805061975064,-1.,2.54379612553051));
#36253=CARTESIAN_POINT('Ctrl Pts',(-3.17678974135318,-1.,2.53704871950948));
#36254=CARTESIAN_POINT('Ctrl Pts',(-3.17304474093612,-1.,2.53032800406941));
#36255=CARTESIAN_POINT('Ctrl Pts',(-3.16927102130736,-1.,2.52363434671788));
#36256=CARTESIAN_POINT('Ctrl Pts',(-3.16546808277023,-1.,2.51696788755577));
#36257=CARTESIAN_POINT('Ctrl Pts',(-3.16163506380157,-1.,2.51032851007894));
#36258=CARTESIAN_POINT('Ctrl Pts',(-3.15777102413957,-1.,2.50371605688252));
#36259=CARTESIAN_POINT('Ctrl Pts',(-3.15387518039046,-1.,2.49713050858896));
#36260=CARTESIAN_POINT('Ctrl Pts',(-3.14994715298907,-1.,2.49057217131988));
#36261=CARTESIAN_POINT('Ctrl Pts',(-3.14598722723896,-1.,2.4840418741839));
#36262=CARTESIAN_POINT('Ctrl Pts',(-3.14199655778863,-1.,2.47754112428043));
#36263=CARTESIAN_POINT('Ctrl Pts',(-3.13797654408943,-1.,2.47107164236838));
#36264=CARTESIAN_POINT('Ctrl Pts',(-3.13392826623906,-1.,2.46463494332374));
#36265=CARTESIAN_POINT('Ctrl Pts',(-3.12985188384371,-1.,2.45823188859366));
#36266=CARTESIAN_POINT('Ctrl Pts',(-3.12574608210847,-1.,2.45186227369846));
#36267=CARTESIAN_POINT('Ctrl Pts',(-3.12160740887768,-1.,2.44552433364715));
#36268=CARTESIAN_POINT('Ctrl Pts',(-3.11743156744186,-1.,2.43921571477977));
#36269=CARTESIAN_POINT('Ctrl Pts',(-3.11321477659018,-1.,2.43293449685144));
#36270=CARTESIAN_POINT('Ctrl Pts',(-3.10895518969595,-1.,2.42668025870015));
#36271=CARTESIAN_POINT('Ctrl Pts',(-3.10465410280896,-1.,2.42045498612489));
#36272=CARTESIAN_POINT('Ctrl Pts',(-3.1003177502767,-1.,2.41426441798057));
#36273=CARTESIAN_POINT('Ctrl Pts',(-3.09595472616076,-1.,2.40811612696369));
#36274=CARTESIAN_POINT('Ctrl Pts',(-3.091572660511,-1.,2.40201704423341));
#36275=CARTESIAN_POINT('Ctrl Pts',(-3.08717489512914,-1.,2.39597098250631));
#36276=CARTESIAN_POINT('Ctrl Pts',(-3.08275773747093,-1.,2.38997659219199));
#36277=CARTESIAN_POINT('Ctrl Pts',(-3.07830597244326,-1.,2.38402401216126));
#36278=CARTESIAN_POINT('Ctrl Pts',(-3.07379777492165,-1.,2.37809856205548));
#36279=CARTESIAN_POINT('Ctrl Pts',(-3.069212754975,-1.,2.37218678163178));
#36280=CARTESIAN_POINT('Ctrl Pts',(-3.06453964643162,-1.,2.36628220107009));
#36281=CARTESIAN_POINT('Ctrl Pts',(-3.0597826624004,-1.,2.36039011602072));
#36282=CARTESIAN_POINT('Ctrl Pts',(-3.05497218368146,-1.,2.35453559889474));
#36283=CARTESIAN_POINT('Ctrl Pts',(-3.05015565829918,-1.,2.34875673090771));
#36284=CARTESIAN_POINT('Ctrl Pts',(-3.04537822217256,-1.,2.34309017083977));
#36285=CARTESIAN_POINT('Ctrl Pts',(-3.04066496998544,-1.,2.33755792953706));
#36286=CARTESIAN_POINT('Ctrl Pts',(-3.03600588555793,-1.,2.33215619079829));
#36287=CARTESIAN_POINT('Ctrl Pts',(-3.03133125185136,-1.,2.32683687412097));
#36288=CARTESIAN_POINT('Ctrl Pts',(-3.02652678416611,-1.,2.32151944306402));
#36289=CARTESIAN_POINT('Ctrl Pts',(-3.02147780668161,-1.,2.31612479121631));
#36290=CARTESIAN_POINT('Ctrl Pts',(-3.01610726819086,-1.,2.31060449886629));
#36291=CARTESIAN_POINT('Ctrl Pts',(-3.01041131063823,-1.,2.30496809486482));
#36292=CARTESIAN_POINT('Ctrl Pts',(-3.00450832658613,-1.,2.29932091315775));
#36293=CARTESIAN_POINT('Ctrl Pts',(-2.99863310339691,-1.,2.29385894577754));
#36294=CARTESIAN_POINT('Ctrl Pts',(-2.99307930984034,-1.,2.28882328690362));
#36295=CARTESIAN_POINT('Ctrl Pts',(-2.9881543273478,-1.,2.28446419115919));
#36296=CARTESIAN_POINT('Ctrl Pts',(-2.98413343613983,-1.,2.28100472516679));
#36297=CARTESIAN_POINT('Ctrl Pts',(-2.9814234180956,-1.,2.27877674853766));
#36298=CARTESIAN_POINT('Ctrl Pts',(-2.98007383024207,-1.,2.27776738270289));
#36299=CARTESIAN_POINT('Ctrl Pts',(-2.9795116710597,-1.,2.27743009389684));
#36300=CARTESIAN_POINT('Ctrl Pts',(-2.97932307137477,-1.,2.27737238849287));
#36301=CARTESIAN_POINT('Ctrl Pts',(-2.97927412174279,-1.,2.27737254473521));
#36302=CARTESIAN_POINT('',(-3.08655633322109,-1.,2.12971124846838));
#36303=CARTESIAN_POINT('Origin',(0.,-1.,0.));
#36304=CARTESIAN_POINT('',(-3.54075895182139,-1.,2.25898783642071));
#36305=CARTESIAN_POINT('Ctrl Pts',(-3.08655633322109,-1.,2.12971124846838));
#36306=CARTESIAN_POINT('Ctrl Pts',(-3.0865713108946,-1.,2.1297578506162));
#36307=CARTESIAN_POINT('Ctrl Pts',(-3.08668447250383,-1.,2.12991938762497));
#36308=CARTESIAN_POINT('Ctrl Pts',(-3.08717896996213,-1.,2.13034980480519));
#36309=CARTESIAN_POINT('Ctrl Pts',(-3.08855597949844,-1.,2.13132142793056));
#36310=CARTESIAN_POINT('Ctrl Pts',(-3.09151235281832,-1.,2.13321032560805));
#36311=CARTESIAN_POINT('Ctrl Pts',(-3.09604502421197,-1.,2.13596538661154));
#36312=CARTESIAN_POINT('Ctrl Pts',(-3.1017126739137,-1.,2.13930228863968));
#36313=CARTESIAN_POINT('Ctrl Pts',(-3.10821808669189,-1.,2.14302815602195));
#36314=CARTESIAN_POINT('Ctrl Pts',(-3.11522827017075,-1.,2.1469279845768));
#36315=CARTESIAN_POINT('Ctrl Pts',(-3.12242318152001,-1.,2.15079698090627));
#36316=CARTESIAN_POINT('Ctrl Pts',(-3.12954386795575,-1.,2.15447241382872));
#36317=CARTESIAN_POINT('Ctrl Pts',(-3.136453565629,-1.,2.15787423530583));
#36318=CARTESIAN_POINT('Ctrl Pts',(-3.14314440426882,-1.,2.16100905914341));
#36319=CARTESIAN_POINT('Ctrl Pts',(-3.14968624388961,-1.,2.16393520288009));
#36320=CARTESIAN_POINT('Ctrl Pts',(-3.15618975593627,-1.,2.1667372844767));
#36321=CARTESIAN_POINT('Ctrl Pts',(-3.16276685102999,-1.,2.16949910801237));
#36322=CARTESIAN_POINT('Ctrl Pts',(-3.16948480019555,-1.,2.17227212063857));
#36323=CARTESIAN_POINT('Ctrl Pts',(-3.17635032802584,-1.,2.17506466903736));
#36324=CARTESIAN_POINT('Ctrl Pts',(-3.18333474627851,-1.,2.17785968847172));
#36325=CARTESIAN_POINT('Ctrl Pts',(-3.19038924261589,-1.,2.18062558031789));
#36326=CARTESIAN_POINT('Ctrl Pts',(-3.197462937404,-1.,2.18332898656595));
#36327=CARTESIAN_POINT('Ctrl Pts',(-3.20452259717947,-1.,2.18594876115914));
#36328=CARTESIAN_POINT('Ctrl Pts',(-3.21156188355736,-1.,2.18848253363878));
#36329=CARTESIAN_POINT('Ctrl Pts',(-3.21859043114069,-1.,2.1909390194865));
#36330=CARTESIAN_POINT('Ctrl Pts',(-3.22562734221636,-1.,2.19333345123531));
#36331=CARTESIAN_POINT('Ctrl Pts',(-3.23269332296938,-1.,2.19568204933172));
#36332=CARTESIAN_POINT('Ctrl Pts',(-3.23980245361323,-1.,2.19799623693263));
#36333=CARTESIAN_POINT('Ctrl Pts',(-3.24695715874356,-1.,2.20027910880993));
#36334=CARTESIAN_POINT('Ctrl Pts',(-3.25415277957789,-1.,2.20252866491554));
#36335=CARTESIAN_POINT('Ctrl Pts',(-3.26138036637711,-1.,2.20473979048682));
#36336=CARTESIAN_POINT('Ctrl Pts',(-3.2686300613678,-1.,2.20690665217741));
#36337=CARTESIAN_POINT('Ctrl Pts',(-3.27589448005534,-1.,2.20902509417425));
#36338=CARTESIAN_POINT('Ctrl Pts',(-3.28317133333127,-1.,2.21109449750638));
#36339=CARTESIAN_POINT('Ctrl Pts',(-3.29046159238344,-1.,2.21311648827391));
#36340=CARTESIAN_POINT('Ctrl Pts',(-3.29776825193162,-1.,2.21509406923369));
#36341=CARTESIAN_POINT('Ctrl Pts',(-3.3050948781957,-1.,2.21703059947837));
#36342=CARTESIAN_POINT('Ctrl Pts',(-3.31244421655662,-1.,2.21892881679083));
#36343=CARTESIAN_POINT('Ctrl Pts',(-3.31981686778008,-1.,2.22078990842768));
#36344=CARTESIAN_POINT('Ctrl Pts',(-3.32721196326019,-1.,2.22261398879623));
#36345=CARTESIAN_POINT('Ctrl Pts',(-3.3346277284958,-1.,2.224400498785));
#36346=CARTESIAN_POINT('Ctrl Pts',(-3.34206209449371,-1.,2.22614863918044));
#36347=CARTESIAN_POINT('Ctrl Pts',(-3.34951327111117,-1.,2.22785777756588));
#36348=CARTESIAN_POINT('Ctrl Pts',(-3.35698038165529,-1.,2.22952789881011));
#36349=CARTESIAN_POINT('Ctrl Pts',(-3.36446325227908,-1.,2.23115945849777));
#36350=CARTESIAN_POINT('Ctrl Pts',(-3.37196214349356,-1.,2.23275319569253));
#36351=CARTESIAN_POINT('Ctrl Pts',(-3.37947749555649,-1.,2.23430995599572));
#36352=CARTESIAN_POINT('Ctrl Pts',(-3.38700968549522,-1.,2.23583052276281));
#36353=CARTESIAN_POINT('Ctrl Pts',(-3.39455873448088,-1.,2.23731541452727));
#36354=CARTESIAN_POINT('Ctrl Pts',(-3.40212434705511,-1.,2.23876491124064));
#36355=CARTESIAN_POINT('Ctrl Pts',(-3.40970604190205,-1.,2.24017914395211));
#36356=CARTESIAN_POINT('Ctrl Pts',(-3.41730325539119,-1.,2.24155816587811));
#36357=CARTESIAN_POINT('Ctrl Pts',(-3.42491544683075,-1.,2.24290202531144));
#36358=CARTESIAN_POINT('Ctrl Pts',(-3.43254222615007,-1.,2.24421085338856));
#36359=CARTESIAN_POINT('Ctrl Pts',(-3.44018336460619,-1.,2.24548487526212));
#36360=CARTESIAN_POINT('Ctrl Pts',(-3.44783872863448,-1.,2.24672437070139));
#36361=CARTESIAN_POINT('Ctrl Pts',(-3.45550823512213,-1.,2.24792964960874));
#36362=CARTESIAN_POINT('Ctrl Pts',(-3.46319180177474,-1.,2.24910102345977));
#36363=CARTESIAN_POINT('Ctrl Pts',(-3.47088928979467,-1.,2.25023877475674));
#36364=CARTESIAN_POINT('Ctrl Pts',(-3.47860048448015,-1.,2.25134314238258));
#36365=CARTESIAN_POINT('Ctrl Pts',(-3.48632513240231,-1.,2.25241433138231));
#36366=CARTESIAN_POINT('Ctrl Pts',(-3.49406296494309,-1.,2.25345251709453));
#36367=CARTESIAN_POINT('Ctrl Pts',(-3.50181372618058,-1.,2.25445785151923));
#36368=CARTESIAN_POINT('Ctrl Pts',(-3.50957720118209,-1.,2.25543046980351));
#36369=CARTESIAN_POINT('Ctrl Pts',(-3.51735323669213,-1.,2.25637049456061));
#36370=CARTESIAN_POINT('Ctrl Pts',(-3.52514172849666,-1.,2.25727802942141));
#36371=CARTESIAN_POINT('Ctrl Pts',(-3.53138243689932,-1.,2.25797812951166));
#36372=CARTESIAN_POINT('Ctrl Pts',(-3.53606853163247,-1.,2.25848864344599));
#36373=CARTESIAN_POINT('Ctrl Pts',(-3.5391950664771,-1.,2.25882251694918));
#36374=CARTESIAN_POINT('Ctrl Pts',(-3.54075895182139,-1.,2.25898783642071));
#36375=CARTESIAN_POINT('',(-3.62024382630768,-1.,2.12928030988903));
#36376=CARTESIAN_POINT('',(-3.54075895182139,-1.,2.25898783642071));
#36377=CARTESIAN_POINT('',(-3.29885386921513,-1.,1.78327315618341));
#36378=CARTESIAN_POINT('Ctrl Pts',(-3.62024382630768,-1.,2.12928030988903));
#36379=CARTESIAN_POINT('Ctrl Pts',(-3.61938653648716,-1.,2.12796193131142));
#36380=CARTESIAN_POINT('Ctrl Pts',(-3.61766963589442,-1.,2.12532774376144));
#36381=CARTESIAN_POINT('Ctrl Pts',(-3.61508732215187,-1.,2.12138417125349));
#36382=CARTESIAN_POINT('Ctrl Pts',(-3.61163030607452,-1.,2.11614149813928));
#36383=CARTESIAN_POINT('Ctrl Pts',(-3.60728578530968,-1.,2.10961391333497));
#36384=CARTESIAN_POINT('Ctrl Pts',(-3.60291797087849,-1.,2.10311217727687));
#36385=CARTESIAN_POINT('Ctrl Pts',(-3.59852681775396,-1.,2.09663642986579));
#36386=CARTESIAN_POINT('Ctrl Pts',(-3.5941122862608,-1.,2.09018686331706));
#36387=CARTESIAN_POINT('Ctrl Pts',(-3.58967435355834,-1.,2.08376373049196));
#36388=CARTESIAN_POINT('Ctrl Pts',(-3.58521300039988,-1.,2.07736732842524));
#36389=CARTESIAN_POINT('Ctrl Pts',(-3.58072819250872,-1.,2.07099797606));
#36390=CARTESIAN_POINT('Ctrl Pts',(-3.57621986224402,-1.,2.06465599229234));
#36391=CARTESIAN_POINT('Ctrl Pts',(-3.5716878942334,-1.,2.05834167687425));
#36392=CARTESIAN_POINT('Ctrl Pts',(-3.56713209977904,-1.,2.05205528172911));
#36393=CARTESIAN_POINT('Ctrl Pts',(-3.56255223871505,-1.,2.04579702158876));
#36394=CARTESIAN_POINT('Ctrl Pts',(-3.55794807264844,-1.,2.03956711119976));
#36395=CARTESIAN_POINT('Ctrl Pts',(-3.55331941293949,-1.,2.03336579658133));
#36396=CARTESIAN_POINT('Ctrl Pts',(-3.54866616282227,-1.,2.02719338376175));
#36397=CARTESIAN_POINT('Ctrl Pts',(-3.54398838254136,-1.,2.02105027983104));
#36398=CARTESIAN_POINT('Ctrl Pts',(-3.53928627453642,-1.,2.01493698847351));
#36399=CARTESIAN_POINT('Ctrl Pts',(-3.53456004727424,-1.,2.00885403604746));
#36400=CARTESIAN_POINT('Ctrl Pts',(-3.52980980250224,-1.,2.00280191090366));
#36401=CARTESIAN_POINT('Ctrl Pts',(-3.52503542491728,-1.,1.99678100339295));
#36402=CARTESIAN_POINT('Ctrl Pts',(-3.52023644289142,-1.,1.99079153006112));
#36403=CARTESIAN_POINT('Ctrl Pts',(-3.51541198728301,-1.,1.9848335106103));
#36404=CARTESIAN_POINT('Ctrl Pts',(-3.51056110478287,-1.,1.97890693666288));
#36405=CARTESIAN_POINT('Ctrl Pts',(-3.5056830186108,-1.,1.97301191162968));
#36406=CARTESIAN_POINT('Ctrl Pts',(-3.50077740176267,-1.,1.96714879724052));
#36407=CARTESIAN_POINT('Ctrl Pts',(-3.49584466573064,-1.,1.961318367765));
#36408=CARTESIAN_POINT('Ctrl Pts',(-3.49088618670987,-1.,1.95552193112084));
#36409=CARTESIAN_POINT('Ctrl Pts',(-3.48590361610814,-1.,1.94976096795911));
#36410=CARTESIAN_POINT('Ctrl Pts',(-3.48089825770416,-1.,1.94403680554065));
#36411=CARTESIAN_POINT('Ctrl Pts',(-3.47587040389915,-1.,1.93835026973887));
#36412=CARTESIAN_POINT('Ctrl Pts',(-3.47081872409781,-1.,1.93270136427081));
#36413=CARTESIAN_POINT('Ctrl Pts',(-3.46573953254084,-1.,1.92708888591158));
#36414=CARTESIAN_POINT('Ctrl Pts',(-3.46062821722485,-1.,1.92151118213212));
#36415=CARTESIAN_POINT('Ctrl Pts',(-3.4554807430995,-1.,1.91596694784063));
#36416=CARTESIAN_POINT('Ctrl Pts',(-3.45029522038888,-1.,1.91045605593639));
#36417=CARTESIAN_POINT('Ctrl Pts',(-3.44507323983367,-1.,1.90498026502304));
#36418=CARTESIAN_POINT('Ctrl Pts',(-3.4398218567809,-1.,1.89954426803384));
#36419=CARTESIAN_POINT('Ctrl Pts',(-3.43455074411571,-1.,1.89415420002542));
#36420=CARTESIAN_POINT('Ctrl Pts',(-3.42926852222158,-1.,1.88881571322009));
#36421=CARTESIAN_POINT('Ctrl Pts',(-3.42397908819736,-1.,1.8835320506206));
#36422=CARTESIAN_POINT('Ctrl Pts',(-3.41867858383771,-1.,1.87830245689344));
#36423=CARTESIAN_POINT('Ctrl Pts',(-3.41335043875209,-1.,1.87311957248121));
#36424=CARTESIAN_POINT('Ctrl Pts',(-3.40797080000549,-1.,1.86797231196654));
#36425=CARTESIAN_POINT('Ctrl Pts',(-3.40251742305476,-1.,1.86285057051245));
#36426=CARTESIAN_POINT('Ctrl Pts',(-3.39697816833067,-1.,1.85774972037062));
#36427=CARTESIAN_POINT('Ctrl Pts',(-3.39135802549398,-1.,1.85267433291769));
#36428=CARTESIAN_POINT('Ctrl Pts',(-3.38569092349592,-1.,1.84764441927753));
#36429=CARTESIAN_POINT('Ctrl Pts',(-3.38002968341157,-1.,1.84269016931643));
#36430=CARTESIAN_POINT('Ctrl Pts',(-3.37442462015853,-1.,1.83784072967077));
#36431=CARTESIAN_POINT('Ctrl Pts',(-3.36890396271836,-1.,1.83311391452322));
#36432=CARTESIAN_POINT('Ctrl Pts',(-3.36345722124158,-1.,1.82850752153199));
#36433=CARTESIAN_POINT('Ctrl Pts',(-3.35800801557424,-1.,1.82398496829301));
#36434=CARTESIAN_POINT('Ctrl Pts',(-3.35243086937598,-1.,1.81948458796829));
#36435=CARTESIAN_POINT('Ctrl Pts',(-3.34660014370673,-1.,1.81494618732853));
#36436=CARTESIAN_POINT('Ctrl Pts',(-3.34043216147606,-1.,1.81033399625352));
#36437=CARTESIAN_POINT('Ctrl Pts',(-3.33392460276808,-1.,1.80565802981102));
#36438=CARTESIAN_POINT('Ctrl Pts',(-3.32721088039578,-1.,1.80100380443406));
#36439=CARTESIAN_POINT('Ctrl Pts',(-3.3205535510082,-1.,1.79652817033251));
#36440=CARTESIAN_POINT('Ctrl Pts',(-3.31428038326424,-1.,1.79242331349949));
#36441=CARTESIAN_POINT('Ctrl Pts',(-3.30873412266788,-1.,1.78888832245873));
#36442=CARTESIAN_POINT('Ctrl Pts',(-3.30422155559112,-1.,1.78610045419846));
#36443=CARTESIAN_POINT('Ctrl Pts',(-3.30119637003393,-1.,1.78432384788174));
#36444=CARTESIAN_POINT('Ctrl Pts',(-3.299705498242,-1.,1.78353803106924));
#36445=CARTESIAN_POINT('Ctrl Pts',(-3.29909749657808,-1.,1.78329283591905));
#36446=CARTESIAN_POINT('Ctrl Pts',(-3.29890219175423,-1.,1.78326534445518));
#36447=CARTESIAN_POINT('Ctrl Pts',(-3.29885386921513,-1.,1.78327315618341));
#36448=CARTESIAN_POINT('',(-3.38171594275687,-1.,1.62064718014256));
#36449=CARTESIAN_POINT('Origin',(0.,-1.,0.));
#36450=CARTESIAN_POINT('',(-3.85054988729471,-1.,1.67727921511438));
#36451=CARTESIAN_POINT('Ctrl Pts',(-3.38171594275687,-1.,1.62064718014256));
#36452=CARTESIAN_POINT('Ctrl Pts',(-3.38173802621243,-1.,1.62069086551626));
#36453=CARTESIAN_POINT('Ctrl Pts',(-3.38187506457001,-1.,1.62083271136059));
#36454=CARTESIAN_POINT('Ctrl Pts',(-3.38243080602536,-1.,1.62118047294574));
#36455=CARTESIAN_POINT('Ctrl Pts',(-3.3839428576331,-1.,1.62192472202795));
#36456=CARTESIAN_POINT('Ctrl Pts',(-3.38715832178929,-1.,1.62332788556183));
#36457=CARTESIAN_POINT('Ctrl Pts',(-3.39206617497078,-1.,1.62533996116793));
#36458=CARTESIAN_POINT('Ctrl Pts',(-3.39818605298342,-1.,1.62774916464571));
#36459=CARTESIAN_POINT('Ctrl Pts',(-3.40519422740596,-1.,1.63041148964996));
#36460=CARTESIAN_POINT('Ctrl Pts',(-3.41272817148719,-1.,1.63316667054156));
#36461=CARTESIAN_POINT('Ctrl Pts',(-3.4204397459095,-1.,1.63586250099804));
#36462=CARTESIAN_POINT('Ctrl Pts',(-3.42804772926213,-1.,1.6383787624689));
#36463=CARTESIAN_POINT('Ctrl Pts',(-3.43540451921397,-1.,1.64065778701952));
#36464=CARTESIAN_POINT('Ctrl Pts',(-3.44250337701736,-1.,1.64270733821042));
#36465=CARTESIAN_POINT('Ctrl Pts',(-3.44942242546693,-1.,1.64457408708059));
#36466=CARTESIAN_POINT('Ctrl Pts',(-3.4562842106239,-1.,1.64632429697506));
#36467=CARTESIAN_POINT('Ctrl Pts',(-3.46321237515029,-1.,1.64802323352752));
#36468=CARTESIAN_POINT('Ctrl Pts',(-3.47028140996055,-1.,1.64971118698285));
#36469=CARTESIAN_POINT('Ctrl Pts',(-3.47749926256543,-1.,1.65139534930353));
#36470=CARTESIAN_POINT('Ctrl Pts',(-3.48483492840942,-1.,1.65306335367762));
#36471=CARTESIAN_POINT('Ctrl Pts',(-3.49223525300194,-1.,1.65469162644476));
#36472=CARTESIAN_POINT('Ctrl Pts',(-3.49964476477929,-1.,1.65625517961583));
#36473=CARTESIAN_POINT('Ctrl Pts',(-3.5070273314651,-1.,1.65773832633617));
#36474=CARTESIAN_POINT('Ctrl Pts',(-3.51437632188903,-1.,1.65913971687324));
#36475=CARTESIAN_POINT('Ctrl Pts',(-3.52170261543787,-1.,1.66046645222266));
#36476=CARTESIAN_POINT('Ctrl Pts',(-3.52902746211081,-1.,1.66173058912365));
#36477=CARTESIAN_POINT('Ctrl Pts',(-3.53637385060225,-1.,1.66294490916113));
#36478=CARTESIAN_POINT('Ctrl Pts',(-3.5437574747503,-1.,1.66411849222334));
#36479=CARTESIAN_POINT('Ctrl Pts',(-3.5511812134288,-1.,1.66525401569004));
#36480=CARTESIAN_POINT('Ctrl Pts',(-3.55864015233617,-1.,1.66635023293121));
#36481=CARTESIAN_POINT('Ctrl Pts',(-3.56612465179429,-1.,1.66740349220308));
#36482=CARTESIAN_POINT('Ctrl Pts',(-3.57362406285884,-1.,1.66840957407299));
#36483=CARTESIAN_POINT('Ctrl Pts',(-3.58113044183823,-1.,1.66936552908228));
#36484=CARTESIAN_POINT('Ctrl Pts',(-3.5886414309783,-1.,1.67027110397601));
#36485=CARTESIAN_POINT('Ctrl Pts',(-3.59615824388808,-1.,1.67112775290706));
#36486=CARTESIAN_POINT('Ctrl Pts',(-3.60368430815203,-1.,1.67193797318598));
#36487=CARTESIAN_POINT('Ctrl Pts',(-3.61122367156182,-1.,1.67270452466968));
#36488=CARTESIAN_POINT('Ctrl Pts',(-3.61877947398179,-1.,1.67342968196223));
#36489=CARTESIAN_POINT('Ctrl Pts',(-3.62635249450908,-1.,1.67411452372265));
#36490=CARTESIAN_POINT('Ctrl Pts',(-3.63394189312902,-1.,1.67475929882962));
#36491=CARTESIAN_POINT('Ctrl Pts',(-3.6415458297232,-1.,1.67536373264839));
#36492=CARTESIAN_POINT('Ctrl Pts',(-3.64916213574663,-1.,1.6759273594669));
#36493=CARTESIAN_POINT('Ctrl Pts',(-3.65678894416442,-1.,1.67644983469459));
#36494=CARTESIAN_POINT('Ctrl Pts',(-3.66442538671018,-1.,1.67693128053153));
#36495=CARTESIAN_POINT('Ctrl Pts',(-3.67207136294639,-1.,1.67737217414901));
#36496=CARTESIAN_POINT('Ctrl Pts',(-3.6797272457918,-1.,1.67777320475872));
#36497=CARTESIAN_POINT('Ctrl Pts',(-3.68739360236505,-1.,1.67813513867973));
#36498=CARTESIAN_POINT('Ctrl Pts',(-3.69507092759545,-1.,1.67845869064304));
#36499=CARTESIAN_POINT('Ctrl Pts',(-3.70275932350998,-1.,1.6787443694862));
#36500=CARTESIAN_POINT('Ctrl Pts',(-3.71045854208195,-1.,1.67899249793398));
#36501=CARTESIAN_POINT('Ctrl Pts',(-3.71816812842188,-1.,1.6792032807165));
#36502=CARTESIAN_POINT('Ctrl Pts',(-3.72588753416339,-1.,1.67937685856627));
#36503=CARTESIAN_POINT('Ctrl Pts',(-3.73361623282617,-1.,1.67951336376434));
#36504=CARTESIAN_POINT('Ctrl Pts',(-3.74135385965622,-1.,1.67961298685316));
#36505=CARTESIAN_POINT('Ctrl Pts',(-3.74910022394845,-1.,1.67967598599665));
#36506=CARTESIAN_POINT('Ctrl Pts',(-3.75685523754816,-1.,1.67970265841379));
#36507=CARTESIAN_POINT('Ctrl Pts',(-3.76461886684523,-1.,1.67969332319322));
#36508=CARTESIAN_POINT('Ctrl Pts',(-3.77239107928394,-1.,1.67964830084946));
#36509=CARTESIAN_POINT('Ctrl Pts',(-3.78017178196859,-1.,1.67956789211943));
#36510=CARTESIAN_POINT('Ctrl Pts',(-3.78796080021026,-1.,1.67945236653175));
#36511=CARTESIAN_POINT('Ctrl Pts',(-3.7957579157763,-1.,1.67930196625203));
#36512=CARTESIAN_POINT('Ctrl Pts',(-3.80356289078481,-1.,1.67911690648128));
#36513=CARTESIAN_POINT('Ctrl Pts',(-3.81137549624273,-1.,1.67889737738311));
#36514=CARTESIAN_POINT('Ctrl Pts',(-3.81919554100522,-1.,1.67864354606363));
#36515=CARTESIAN_POINT('Ctrl Pts',(-3.82702289288453,-1.,1.67835555760094));
#36516=CARTESIAN_POINT('Ctrl Pts',(-3.83485746516115,-1.,1.67803353065273));
#36517=CARTESIAN_POINT('Ctrl Pts',(-3.8411308598706,-1.,1.67774874946867));
#36518=CARTESIAN_POINT('Ctrl Pts',(-3.84583912297567,-1.,1.67751991140661));
#36519=CARTESIAN_POINT('Ctrl Pts',(-3.84897939431104,-1.,1.6773605765671));
#36520=CARTESIAN_POINT('Ctrl Pts',(-3.85054988729471,-1.,1.67727921511438));
#36521=CARTESIAN_POINT('',(-3.90876544355381,-1.,1.53673442965255));
#36522=CARTESIAN_POINT('',(-3.85054988729471,-1.,1.67727921511438));
#36523=CARTESIAN_POINT('',(-3.5372048861591,-1.,1.24526366418208));
#36524=CARTESIAN_POINT('Ctrl Pts',(-3.90876544355381,-1.,1.53673442965255));
#36525=CARTESIAN_POINT('Ctrl Pts',(-3.90771246854607,-1.,1.53556639217742));
#36526=CARTESIAN_POINT('Ctrl Pts',(-3.90560462812846,-1.,1.53323321827311));
#36527=CARTESIAN_POINT('Ctrl Pts',(-3.90243719629755,-1.,1.5297421605556));
#36528=CARTESIAN_POINT('Ctrl Pts',(-3.8982026070607,-1.,1.52510482990784));
#36529=CARTESIAN_POINT('Ctrl Pts',(-3.89289043531893,-1.,1.51933724328609));
#36530=CARTESIAN_POINT('Ctrl Pts',(-3.88755930032927,-1.,1.51359883110181));
#36531=CARTESIAN_POINT('Ctrl Pts',(-3.88220917950443,-1.,1.50788973857719));
#36532=CARTESIAN_POINT('Ctrl Pts',(-3.87684006372665,-1.,1.50221016176766));
#36533=CARTESIAN_POINT('Ctrl Pts',(-3.8714519699927,-1.,1.4965603539944));
#36534=CARTESIAN_POINT('Ctrl Pts',(-3.86604492575933,-1.,1.49094061164604));
#36535=CARTESIAN_POINT('Ctrl Pts',(-3.86061894706551,-1.,1.48535125510102));
#36536=CARTESIAN_POINT('Ctrl Pts',(-3.85517401698952,-1.,1.47979260991063));
#36537=CARTESIAN_POINT('Ctrl Pts',(-3.84971006847096,-1.,1.47426499018467));
#36538=CARTESIAN_POINT('Ctrl Pts',(-3.84422695454469,-1.,1.46876867426374));
#36539=CARTESIAN_POINT('Ctrl Pts',(-3.83872447159309,-1.,1.46330391180621));
#36540=CARTESIAN_POINT('Ctrl Pts',(-3.83320241775199,-1.,1.45787095220763));
#36541=CARTESIAN_POINT('Ctrl Pts',(-3.82766064519,-1.,1.45247006796807));
#36542=CARTESIAN_POINT('Ctrl Pts',(-3.82209910620591,-1.,1.44710157648562));
#36543=CARTESIAN_POINT('Ctrl Pts',(-3.8165179239855,-1.,1.441765870414));
#36544=CARTESIAN_POINT('Ctrl Pts',(-3.81091737726965,-1.,1.43646341556783));
#36545=CARTESIAN_POINT('Ctrl Pts',(-3.80529775429916,-1.,1.43119469921364));
#36546=CARTESIAN_POINT('Ctrl Pts',(-3.79965923196365,-1.,1.42596018777301));
#36547=CARTESIAN_POINT('Ctrl Pts',(-3.7940017574439,-1.,1.42076028482828));
#36548=CARTESIAN_POINT('Ctrl Pts',(-3.78832489879369,-1.,1.41559527803808));
#36549=CARTESIAN_POINT('Ctrl Pts',(-3.78262780065406,-1.,1.41046532282567));
#36550=CARTESIAN_POINT('Ctrl Pts',(-3.77690952014209,-1.,1.40537056004702));
#36551=CARTESIAN_POINT('Ctrl Pts',(-3.77116930621804,-1.,1.40031121335495));
#36552=CARTESIAN_POINT('Ctrl Pts',(-3.76540689249078,-1.,1.39528769118054));
#36553=CARTESIAN_POINT('Ctrl Pts',(-3.75962280650875,-1.,1.39030069388926));
#36554=CARTESIAN_POINT('Ctrl Pts',(-3.75381861212728,-1.,1.38535129801185));
#36555=CARTESIAN_POINT('Ctrl Pts',(-3.74799617204744,-1.,1.38044070763302));
#36556=CARTESIAN_POINT('Ctrl Pts',(-3.7421569816256,-1.,1.3755700297169));
#36557=CARTESIAN_POINT('Ctrl Pts',(-3.73630145885809,-1.,1.37074003422739));
#36558=CARTESIAN_POINT('Ctrl Pts',(-3.73042829011293,-1.,1.36595093298674));
#36559=CARTESIAN_POINT('Ctrl Pts',(-3.72453364678279,-1.,1.36120211416353));
#36560=CARTESIAN_POINT('Ctrl Pts',(-3.71861271513318,-1.,1.35649266705038));
#36561=CARTESIAN_POINT('Ctrl Pts',(-3.71266130563061,-1.,1.35182193384426));
#36562=CARTESIAN_POINT('Ctrl Pts',(-3.7066775318825,-1.,1.34719008463535));
#36563=CARTESIAN_POINT('Ctrl Pts',(-3.70066324015112,-1.,1.3425986075293));
#36564=CARTESIAN_POINT('Ctrl Pts',(-3.69462613305692,-1.,1.33805103398214));
#36565=CARTESIAN_POINT('Ctrl Pts',(-3.68857672413013,-1.,1.33355191034515));
#36566=CARTESIAN_POINT('Ctrl Pts',(-3.68252441182534,-1.,1.32910547072734));
#36567=CARTESIAN_POINT('Ctrl Pts',(-3.67647355257906,-1.,1.32471430856413));
#36568=CARTESIAN_POINT('Ctrl Pts',(-3.67042021752668,-1.,1.3203782813777));
#36569=CARTESIAN_POINT('Ctrl Pts',(-3.66434688899822,-1.,1.31609271239922));
#36570=CARTESIAN_POINT('Ctrl Pts',(-3.65822827358655,-1.,1.31185038411231));
#36571=CARTESIAN_POINT('Ctrl Pts',(-3.65204081987101,-1.,1.30764479590051));
#36572=CARTESIAN_POINT('Ctrl Pts',(-3.64577181380125,-1.,1.30347327603778));
#36573=CARTESIAN_POINT('Ctrl Pts',(-3.6394268987279,-1.,1.29933955906463));
#36574=CARTESIAN_POINT('Ctrl Pts',(-3.63304271630995,-1.,1.29525810207744));
#36575=CARTESIAN_POINT('Ctrl Pts',(-3.62667616004299,-1.,1.29125046021853));
#36576=CARTESIAN_POINT('Ctrl Pts',(-3.62038148492295,-1.,1.2873375502936));
#36577=CARTESIAN_POINT('Ctrl Pts',(-3.61418935913793,-1.,1.28353255117754));
#36578=CARTESIAN_POINT('Ctrl Pts',(-3.60808907746372,-1.,1.27983492861703));
#36579=CARTESIAN_POINT('Ctrl Pts',(-3.60199947736404,-1.,1.27622049908664));
#36580=CARTESIAN_POINT('Ctrl Pts',(-3.59578698050164,-1.,1.27264798379365));
#36581=CARTESIAN_POINT('Ctrl Pts',(-3.5893180784647,-1.,1.26907758484766));
#36582=CARTESIAN_POINT('Ctrl Pts',(-3.58250452868699,-1.,1.26548706249891));
#36583=CARTESIAN_POINT('Ctrl Pts',(-3.5753456065164,-1.,1.26188667142784));
#36584=CARTESIAN_POINT('Ctrl Pts',(-3.56798645995025,-1.,1.25834000485626));
#36585=CARTESIAN_POINT('Ctrl Pts',(-3.56071094990825,-1.,1.25496090899873));
#36586=CARTESIAN_POINT('Ctrl Pts',(-3.5538728741862,-1.,1.25188792940508));
#36587=CARTESIAN_POINT('Ctrl Pts',(-3.54784190282889,-1.,1.24926408627938));
#36588=CARTESIAN_POINT('Ctrl Pts',(-3.54294877426113,-1.,1.2472164623202));
#36589=CARTESIAN_POINT('Ctrl Pts',(-3.53968291129942,-1.,1.24593497225964));
#36590=CARTESIAN_POINT('Ctrl Pts',(-3.53808746578052,-1.,1.2453920538873));
#36591=CARTESIAN_POINT('Ctrl Pts',(-3.53744859265385,-1.,1.24524498991133));
#36592=CARTESIAN_POINT('Ctrl Pts',(-3.53725139174402,-1.,1.24524838931864));
#36593=CARTESIAN_POINT('Ctrl Pts',(-3.5372048861591,-1.,1.24526366418208));
#36594=CARTESIAN_POINT('',(-3.59360648251021,-1.,1.071677399622));
#36595=CARTESIAN_POINT('Origin',(0.,-1.,0.));
#36596=CARTESIAN_POINT('',(-4.06552750530042,-1.,1.05427041296137));
#36597=CARTESIAN_POINT('Ctrl Pts',(-3.59360648251021,-1.,1.071677399622));
#36598=CARTESIAN_POINT('Ctrl Pts',(-3.59363512797985,-1.,1.07171709254271));
#36599=CARTESIAN_POINT('Ctrl Pts',(-3.59379266874663,-1.,1.07183575450716));
#36600=CARTESIAN_POINT('Ctrl Pts',(-3.59439597,-1.,1.07209229745284));
#36601=CARTESIAN_POINT('Ctrl Pts',(-3.59600583195037,-1.,1.07259084660947));
#36602=CARTESIAN_POINT('Ctrl Pts',(-3.59940121154383,-1.,1.0734737254567));
#36603=CARTESIAN_POINT('Ctrl Pts',(-3.6045633988796,-1.,1.0746932716863));
#36604=CARTESIAN_POINT('Ctrl Pts',(-3.61098481349577,-1.,1.07611545402841));
#36605=CARTESIAN_POINT('Ctrl Pts',(-3.61832318504957,-1.,1.07764868137729));
#36606=CARTESIAN_POINT('Ctrl Pts',(-3.62619537902616,-1.,1.07919137290815));
#36607=CARTESIAN_POINT('Ctrl Pts',(-3.63423373196602,-1.,1.08064765719887));
#36608=CARTESIAN_POINT('Ctrl Pts',(-3.64214167843595,-1.,1.08194278850972));
#36609=CARTESIAN_POINT('Ctrl Pts',(-3.64976441208197,-1.,1.08304289898577));
#36610=CARTESIAN_POINT('Ctrl Pts',(-3.65709649161004,-1.,1.08395671077761));
#36611=CARTESIAN_POINT('Ctrl Pts',(-3.66422237895256,-1.,1.0847180992287));
#36612=CARTESIAN_POINT('Ctrl Pts',(-3.67127347729632,-1.,1.0853733414448));
#36613=CARTESIAN_POINT('Ctrl Pts',(-3.67838211685148,-1.,1.08596755755768));
#36614=CARTESIAN_POINT('Ctrl Pts',(-3.68562817420864,-1.,1.08652888882609));
#36615=CARTESIAN_POINT('Ctrl Pts',(-3.69302062410229,-1.,1.08706319540291));
#36616=CARTESIAN_POINT('Ctrl Pts',(-3.70052690909884,-1.,1.08756311291324));
#36617=CARTESIAN_POINT('Ctrl Pts',(-3.70809084139476,-1.,1.0880136731219));
#36618=CARTESIAN_POINT('Ctrl Pts',(-3.71565372339063,-1.,1.08839887334776));
#36619=CARTESIAN_POINT('Ctrl Pts',(-3.72317741369364,-1.,1.08870887220072));
#36620=CARTESIAN_POINT('Ctrl Pts',(-3.73065515162949,-1.,1.08894337390925));
#36621=CARTESIAN_POINT('Ctrl Pts',(-3.73809879348209,-1.,1.08910769013288));
#36622=CARTESIAN_POINT('Ctrl Pts',(-3.74553121371745,-1.,1.08921040494013));
#36623=CARTESIAN_POINT('Ctrl Pts',(-3.75297711748138,-1.,1.08926054632927));
#36624=CARTESIAN_POINT('Ctrl Pts',(-3.76045342580226,-1.,1.08926462734287));
#36625=CARTESIAN_POINT('Ctrl Pts',(-3.76796340094469,-1.,1.08922484204263));
#36626=CARTESIAN_POINT('Ctrl Pts',(-3.7755019940944,-1.,1.08914072791275));
#36627=CARTESIAN_POINT('Ctrl Pts',(-3.78305911299511,-1.,1.08901018614638));
#36628=CARTESIAN_POINT('Ctrl Pts',(-3.79062357974401,-1.,1.08883071512097));
#36629=CARTESIAN_POINT('Ctrl Pts',(-3.79818708705252,-1.,1.08860064435776));
#36630=CARTESIAN_POINT('Ctrl Pts',(-3.80574726657656,-1.,1.08832009255378));
#36631=CARTESIAN_POINT('Ctrl Pts',(-3.81330554446324,-1.,1.08799030610861));
#36632=CARTESIAN_POINT('Ctrl Pts',(-3.82086569676321,-1.,1.08761321539442));
#36633=CARTESIAN_POINT('Ctrl Pts',(-3.82843215316985,-1.,1.08719091307558));
#36634=CARTESIAN_POINT('Ctrl Pts',(-3.83600837071702,-1.,1.08672515456901));
#36635=CARTESIAN_POINT('Ctrl Pts',(-3.84359528764934,-1.,1.08621688337601));
#36636=CARTESIAN_POINT('Ctrl Pts',(-3.85119211322732,-1.,1.08566647671838));
#36637=CARTESIAN_POINT('Ctrl Pts',(-3.85879698702511,-1.,1.08507395120054));
#36638=CARTESIAN_POINT('Ctrl Pts',(-3.86640769434269,-1.,1.08443918607926));
#36639=CARTESIAN_POINT('Ctrl Pts',(-3.87402233722563,-1.,1.0837621330751));
#36640=CARTESIAN_POINT('Ctrl Pts',(-3.88164007721365,-1.,1.08304304871042));
#36641=CARTESIAN_POINT('Ctrl Pts',(-3.88926088975182,-1.,1.08228241999363));
#36642=CARTESIAN_POINT('Ctrl Pts',(-3.89688525098408,-1.,1.08148086931373));
#36643=CARTESIAN_POINT('Ctrl Pts',(-3.90451384092564,-1.,1.08063906483822));
#36644=CARTESIAN_POINT('Ctrl Pts',(-3.91214726022096,-1.,1.0797576350746));
#36645=CARTESIAN_POINT('Ctrl Pts',(-3.91978568924062,-1.,1.07883706663524));
#36646=CARTESIAN_POINT('Ctrl Pts',(-3.92742893349684,-1.,1.07787771707155));
#36647=CARTESIAN_POINT('Ctrl Pts',(-3.93507657572743,-1.,1.07687985975348));
#36648=CARTESIAN_POINT('Ctrl Pts',(-3.94272809633271,-1.,1.07584371946428));
#36649=CARTESIAN_POINT('Ctrl Pts',(-3.95038299600754,-1.,1.07476950921607));
#36650=CARTESIAN_POINT('Ctrl Pts',(-3.95804094429606,-1.,1.07365747426551));
#36651=CARTESIAN_POINT('Ctrl Pts',(-3.96570179322681,-1.,1.07250789943095));
#36652=CARTESIAN_POINT('Ctrl Pts',(-3.97336550222571,-1.,1.07132109206252));
#36653=CARTESIAN_POINT('Ctrl Pts',(-3.98103208801289,-1.,1.07009737257815));
#36654=CARTESIAN_POINT('Ctrl Pts',(-3.98870156857298,-1.,1.06883706263912));
#36655=CARTESIAN_POINT('Ctrl Pts',(-3.99637389919958,-1.,1.06754047381188));
#36656=CARTESIAN_POINT('Ctrl Pts',(-4.00404894951804,-1.,1.06620789963406));
#36657=CARTESIAN_POINT('Ctrl Pts',(-4.0117265418656,-1.,1.06483961342894));
#36658=CARTESIAN_POINT('Ctrl Pts',(-4.0194064749539,-1.,1.06343586496094));
#36659=CARTESIAN_POINT('Ctrl Pts',(-4.02708855235732,-1.,1.06199687787488));
#36660=CARTESIAN_POINT('Ctrl Pts',(-4.03477261142549,-1.,1.06052284712114));
#36661=CARTESIAN_POINT('Ctrl Pts',(-4.04245854429333,-1.,1.05901393667039));
#36662=CARTESIAN_POINT('Ctrl Pts',(-4.05014628387112,-1.,1.05747027728537));
#36663=CARTESIAN_POINT('Ctrl Pts',(-4.05629789308941,-1.,1.0562076270849));
#36664=CARTESIAN_POINT('Ctrl Pts',(-4.06091239150293,-1.,1.05524507177901));
#36665=CARTESIAN_POINT('Ctrl Pts',(-4.06398907542679,-1.,1.05459645194934));
#36666=CARTESIAN_POINT('Ctrl Pts',(-4.06552750530042,-1.,1.05427041296137));
#36667=CARTESIAN_POINT('',(-4.10104028313088,-1.,0.906349047628866));
#36668=CARTESIAN_POINT('',(-4.06552750530042,-1.,1.05427041296137));
#36669=CARTESIAN_POINT('',(-3.68845817949586,-1.,0.676591647975428));
#36670=CARTESIAN_POINT('Ctrl Pts',(-4.10104028313088,-1.,0.906349047628866));
#36671=CARTESIAN_POINT('Ctrl Pts',(-4.09981755067523,-1.,0.905360112215337));
#36672=CARTESIAN_POINT('Ctrl Pts',(-4.09737067245935,-1.,0.903385402441587));
#36673=CARTESIAN_POINT('Ctrl Pts',(-4.09369611522387,-1.,0.900432820941674));
#36674=CARTESIAN_POINT('Ctrl Pts',(-4.08878822246833,-1.,0.896515019231333));
#36675=CARTESIAN_POINT('Ctrl Pts',(-4.08263920304799,-1.,0.891649447916277));
#36676=CARTESIAN_POINT('Ctrl Pts',(-4.07647601773635,-1.,0.886815658358501));
#36677=CARTESIAN_POINT('Ctrl Pts',(-4.07029866694192,-1.,0.882013797525692));
#36678=CARTESIAN_POINT('Ctrl Pts',(-4.06410717232905,-1.,0.877244060485837));
#36679=CARTESIAN_POINT('Ctrl Pts',(-4.0579015903134,-1.,0.872506694782446));
#36680=CARTESIAN_POINT('Ctrl Pts',(-4.05168199437909,-1.,0.867801988859917));
#36681=CARTESIAN_POINT('Ctrl Pts',(-4.04544845048584,-1.,0.863130256643259));
#36682=CARTESIAN_POINT('Ctrl Pts',(-4.03920099284773,-1.,0.858491822322827));
#36683=CARTESIAN_POINT('Ctrl Pts',(-4.03293960436756,-1.,0.853887006631755));
#36684=CARTESIAN_POINT('Ctrl Pts',(-4.02666418343164,-1.,0.849316107474245));
#36685=CARTESIAN_POINT('Ctrl Pts',(-4.02037456798441,-1.,0.844779403287745));
#36686=CARTESIAN_POINT('Ctrl Pts',(-4.01407059766103,-1.,0.840277171975855));
#36687=CARTESIAN_POINT('Ctrl Pts',(-4.00775216907856,-1.,0.835809705809646));
#36688=CARTESIAN_POINT('Ctrl Pts',(-4.00141928477507,-1.,0.831377325741622));
#36689=CARTESIAN_POINT('Ctrl Pts',(-3.99507212784431,-1.,0.826980400320789));
#36690=CARTESIAN_POINT('Ctrl Pts',(-3.98871104646485,-1.,0.822619346022119));
#36691=CARTESIAN_POINT('Ctrl Pts',(-3.98233640155404,-1.,0.818294599022293));
#36692=CARTESIAN_POINT('Ctrl Pts',(-3.97594844078811,-1.,0.814006592328843));
#36693=CARTESIAN_POINT('Ctrl Pts',(-3.96954717513232,-1.,0.80975573281809));
#36694=CARTESIAN_POINT('Ctrl Pts',(-3.96313222295815,-1.,0.805542372178361));
#36695=CARTESIAN_POINT('Ctrl Pts',(-3.95670276375108,-1.,0.801366797727049));
#36696=CARTESIAN_POINT('Ctrl Pts',(-3.95025788827136,-1.,0.797229296085315));
#36697=CARTESIAN_POINT('Ctrl Pts',(-3.94379688971283,-1.,0.793130205640961));
#36698=CARTESIAN_POINT('Ctrl Pts',(-3.93731956885676,-1.,0.789069971469333));
#36699=CARTESIAN_POINT('Ctrl Pts',(-3.93082655631789,-1.,0.785049202786507));
#36700=CARTESIAN_POINT('Ctrl Pts',(-3.92431956510441,-1.,0.781068718228451));
#36701=CARTESIAN_POINT('Ctrl Pts',(-3.9178006233448,-1.,0.777129415664956));
#36702=CARTESIAN_POINT('Ctrl Pts',(-3.91127138115243,-1.,0.773232154506321));
#36703=CARTESIAN_POINT('Ctrl Pts',(-3.90473237182633,-1.,0.769377629847874));
#36704=CARTESIAN_POINT('Ctrl Pts',(-3.89818233104378,-1.,0.765566256401295));
#36705=CARTESIAN_POINT('Ctrl Pts',(-3.89161738162245,-1.,0.761798028793969));
#36706=CARTESIAN_POINT('Ctrl Pts',(-3.88503262662689,-1.,0.758072800564801));
#36707=CARTESIAN_POINT('Ctrl Pts',(-3.87842382520065,-1.,0.754390577396856));
#36708=CARTESIAN_POINT('Ctrl Pts',(-3.87178914078374,-1.,0.750751822383027));
#36709=CARTESIAN_POINT('Ctrl Pts',(-3.86513062969889,-1.,0.747157716488871));
#36710=CARTESIAN_POINT('Ctrl Pts',(-3.85845645217594,-1.,0.743610542737012));
#36711=CARTESIAN_POINT('Ctrl Pts',(-3.85177770351216,-1.,0.740113146827137));
#36712=CARTESIAN_POINT('Ctrl Pts',(-3.84510432881213,-1.,0.736668240497117));
#36713=CARTESIAN_POINT('Ctrl Pts',(-3.83844103658009,-1.,0.733277703756078));
#36714=CARTESIAN_POINT('Ctrl Pts',(-3.83178392403383,-1.,0.729942010490167));
#36715=CARTESIAN_POINT('Ctrl Pts',(-3.82511495756713,-1.,0.726659281876664));
#36716=CARTESIAN_POINT('Ctrl Pts',(-3.81840802610835,-1.,0.723426346019422));
#36717=CARTESIAN_POINT('Ctrl Pts',(-3.81163885127344,-1.,0.720240466589236));
#36718=CARTESIAN_POINT('Ctrl Pts',(-3.80479445759309,-1.,0.717100993669114));
#36719=CARTESIAN_POINT('Ctrl Pts',(-3.79788100314975,-1.,0.71401073300664));
#36720=CARTESIAN_POINT('Ctrl Pts',(-3.79093694007094,-1.,0.710978231689017));
#36721=CARTESIAN_POINT('Ctrl Pts',(-3.78402183336605,-1.,0.708015879375459));
#36722=CARTESIAN_POINT('Ctrl Pts',(-3.77719254217129,-1.,0.705135847999816));
#36723=CARTESIAN_POINT('Ctrl Pts',(-3.77048141872872,-1.,0.702346356621551));
#36724=CARTESIAN_POINT('Ctrl Pts',(-3.76387780603759,-1.,0.699648552230917));
#36725=CARTESIAN_POINT('Ctrl Pts',(-3.75729775767023,-1.,0.697031245659743));
#36726=CARTESIAN_POINT('Ctrl Pts',(-3.75060288243455,-1.,0.694474562581492));
#36727=CARTESIAN_POINT('Ctrl Pts',(-3.74365508986712,-1.,0.69196008040082));
#36728=CARTESIAN_POINT('Ctrl Pts',(-3.73636374475077,-1.,0.689479637354813));
#36729=CARTESIAN_POINT('Ctrl Pts',(-3.72872973554051,-1.,0.687043475232354));
#36730=CARTESIAN_POINT('Ctrl Pts',(-3.7209063713926,-1.,0.684691698167848));
#36731=CARTESIAN_POINT('Ctrl Pts',(-3.71319182789943,-1.,0.68249234510893));
#36732=CARTESIAN_POINT('Ctrl Pts',(-3.70595722031785,-1.,0.680526909710877));
#36733=CARTESIAN_POINT('Ctrl Pts',(-3.69959004073005,-1.,0.678878822226026));
#36734=CARTESIAN_POINT('Ctrl Pts',(-3.69443683573598,-1.,0.677621861865498));
#36735=CARTESIAN_POINT('Ctrl Pts',(-3.69101071175464,-1.,0.676867042599401));
#36736=CARTESIAN_POINT('Ctrl Pts',(-3.68934997767243,-1.,0.676580391119396));
#36737=CARTESIAN_POINT('Ctrl Pts',(-3.68869596425969,-1.,0.676535079520806));
#36738=CARTESIAN_POINT('Ctrl Pts',(-3.68850172300477,-1.,0.676569286094606));
#36739=CARTESIAN_POINT('Ctrl Pts',(-3.68845817949586,-1.,0.676591647975428));
#36740=CARTESIAN_POINT('',(-3.71701050416802,-1.,0.496319364829374));
#36741=CARTESIAN_POINT('Origin',(0.,-1.,0.));
#36742=CARTESIAN_POINT('',(-4.18039834341342,-1.,0.405301974318349));
#36743=CARTESIAN_POINT('Ctrl Pts',(-3.71701050416802,-1.,0.496319364829374));
#36744=CARTESIAN_POINT('Ctrl Pts',(-3.71704500630521,-1.,0.496354087925645));
#36745=CARTESIAN_POINT('Ctrl Pts',(-3.71721917030465,-1.,0.496446644158827));
#36746=CARTESIAN_POINT('Ctrl Pts',(-3.71785517607694,-1.,0.496605651526313));
#36747=CARTESIAN_POINT('Ctrl Pts',(-3.7195232082259,-1.,0.496846224822534));
#36748=CARTESIAN_POINT('Ctrl Pts',(-3.72301489774241,-1.,0.497187079575794));
#36749=CARTESIAN_POINT('Ctrl Pts',(-3.72830430904794,-1.,0.497584067153279));
#36750=CARTESIAN_POINT('Ctrl Pts',(-3.73486914372834,-1.,0.497984209510495));
#36751=CARTESIAN_POINT('Ctrl Pts',(-3.74235701735109,-1.,0.498350586058176));
#36752=CARTESIAN_POINT('Ctrl Pts',(-3.75037362168103,-1.,0.498642802042929));
#36753=CARTESIAN_POINT('Ctrl Pts',(-3.75854082221127,-1.,0.498823681615513));
#36754=CARTESIAN_POINT('Ctrl Pts',(-3.76655401191144,-1.,0.498865792335185));
#36755=CARTESIAN_POINT('Ctrl Pts',(-3.77425499225089,-1.,0.498759900365687));
#36756=CARTESIAN_POINT('Ctrl Pts',(-3.78163975337189,-1.,0.498515471679378));
#36757=CARTESIAN_POINT('Ctrl Pts',(-3.78879701661152,-1.,0.498152751800819));
#36758=CARTESIAN_POINT('Ctrl Pts',(-3.79586380669959,-1.,0.49769689210058));
#36759=CARTESIAN_POINT('Ctrl Pts',(-3.80297788298545,-1.,0.49717175620109));
#36760=CARTESIAN_POINT('Ctrl Pts',(-3.81022254090909,-1.,0.496592643443789));
#36761=CARTESIAN_POINT('Ctrl Pts',(-3.81760756144099,-1.,0.495963937875572));
#36762=CARTESIAN_POINT('Ctrl Pts',(-3.82509963594156,-1.,0.495283458893903));
#36763=CARTESIAN_POINT('Ctrl Pts',(-3.8326409268245,-1.,0.494545212256425));
#36764=CARTESIAN_POINT('Ctrl Pts',(-3.84017095578438,-1.,0.493742574629117));
#36765=CARTESIAN_POINT('Ctrl Pts',(-3.84765051147965,-1.,0.492871792414095));
#36766=CARTESIAN_POINT('Ctrl Pts',(-3.85507287020223,-1.,0.49193363108376));
#36767=CARTESIAN_POINT('Ctrl Pts',(-3.86245057319215,-1.,0.490931482170849));
#36768=CARTESIAN_POINT('Ctrl Pts',(-3.86980755613694,-1.,0.489870245704899));
#36769=CARTESIAN_POINT('Ctrl Pts',(-3.87716963231115,-1.,0.488754973798281));
#36770=CARTESIAN_POINT('Ctrl Pts',(-3.88455453328156,-1.,0.487589452275179));
#36771=CARTESIAN_POINT('Ctrl Pts',(-3.89196582437574,-1.,0.486375337854133));
#36772=CARTESIAN_POINT('Ctrl Pts',(-3.89939844658529,-1.,0.485112963522246));
#36773=CARTESIAN_POINT('Ctrl Pts',(-3.90684210358063,-1.,0.48380183508916));
#36774=CARTESIAN_POINT('Ctrl Pts',(-3.91428536373749,-1.,0.482441230340708));
#36775=CARTESIAN_POINT('Ctrl Pts',(-3.92171976072334,-1.,0.481030798910735));
#36776=CARTESIAN_POINT('Ctrl Pts',(-3.92914297392067,-1.,0.479571028525566));
#36777=CARTESIAN_POINT('Ctrl Pts',(-3.93655660689819,-1.,0.478062927140957));
#36778=CARTESIAN_POINT('Ctrl Pts',(-3.94396469119385,-1.,0.476507810658534));
#36779=CARTESIAN_POINT('Ctrl Pts',(-3.95137192932898,-1.,0.47490705302179));
#36780=CARTESIAN_POINT('Ctrl Pts',(-3.95878201038332,-1.,0.473261847236296));
#36781=CARTESIAN_POINT('Ctrl Pts',(-3.96619600864626,-1.,0.471572978413493));
#36782=CARTESIAN_POINT('Ctrl Pts',(-3.97361320212413,-1.,0.469840942829878));
#36783=CARTESIAN_POINT('Ctrl Pts',(-3.98103175589349,-1.,0.468066047920139));
#36784=CARTESIAN_POINT('Ctrl Pts',(-3.98844946363258,-1.,0.466248520883034));
#36785=CARTESIAN_POINT('Ctrl Pts',(-3.99586444320135,-1.,0.464388610938995));
#36786=CARTESIAN_POINT('Ctrl Pts',(-4.00327590659129,-1.,0.462486702616252));
#36787=CARTESIAN_POINT('Ctrl Pts',(-4.01068390573469,-1.,0.460543280768577));
#36788=CARTESIAN_POINT('Ctrl Pts',(-4.01808900827647,-1.,0.458558885637001));
#36789=CARTESIAN_POINT('Ctrl Pts',(-4.02549199038414,-1.,0.456534070784968));
#36790=CARTESIAN_POINT('Ctrl Pts',(-4.03289354362745,-1.,0.454469363020495));
#36791=CARTESIAN_POINT('Ctrl Pts',(-4.0402939222793,-1.,0.452365214748779));
#36792=CARTESIAN_POINT('Ctrl Pts',(-4.0476929901797,-1.,0.450222009543774));
#36793=CARTESIAN_POINT('Ctrl Pts',(-4.05509037796815,-1.,0.448040082683976));
#36794=CARTESIAN_POINT('Ctrl Pts',(-4.06248560760596,-1.,0.445819737468478));
#36795=CARTESIAN_POINT('Ctrl Pts',(-4.0698782192577,-1.,0.443561262395408));
#36796=CARTESIAN_POINT('Ctrl Pts',(-4.07726792490256,-1.,0.441264951396587));
#36797=CARTESIAN_POINT('Ctrl Pts',(-4.08465462294625,-1.,0.438931108931613));
#36798=CARTESIAN_POINT('Ctrl Pts',(-4.09203832139439,-1.,0.436560044913814));
#36799=CARTESIAN_POINT('Ctrl Pts',(-4.09941908688567,-1.,0.434152073200642));
#36800=CARTESIAN_POINT('Ctrl Pts',(-4.10679698750219,-1.,0.431707508679772));
#36801=CARTESIAN_POINT('Ctrl Pts',(-4.1141720278277,-1.,0.429226666075372));
#36802=CARTESIAN_POINT('Ctrl Pts',(-4.1215441250121,-1.,0.426709855706243));
#36803=CARTESIAN_POINT('Ctrl Pts',(-4.1289131463371,-1.,0.424157375323155));
#36804=CARTESIAN_POINT('Ctrl Pts',(-4.13627893206433,-1.,0.421569503103971));
#36805=CARTESIAN_POINT('Ctrl Pts',(-4.14364132317223,-1.,0.418946490667799));
#36806=CARTESIAN_POINT('Ctrl Pts',(-4.15100018950989,-1.,0.416288556008986));
#36807=CARTESIAN_POINT('Ctrl Pts',(-4.1583554501909,-1.,0.413595877953269));
#36808=CARTESIAN_POINT('Ctrl Pts',(-4.16570705940731,-1.,0.410868596148613));
#36809=CARTESIAN_POINT('Ctrl Pts',(-4.17158541009947,-1.,0.408659167570153));
#36810=CARTESIAN_POINT('Ctrl Pts',(-4.17599251955585,-1.,0.406986596326602));
#36811=CARTESIAN_POINT('Ctrl Pts',(-4.17892985789908,-1.,0.40586466267963));
#36812=CARTESIAN_POINT('Ctrl Pts',(-4.18039834341342,-1.,0.405301974318349));
#36813=CARTESIAN_POINT('',(-4.1923339003649,-1.,0.253646344052521));
#36814=CARTESIAN_POINT('',(-4.18039834341342,-1.,0.405301974318349));
#36815=CARTESIAN_POINT('',(-3.74888939116255,-1.,0.0912596999166822));
#36816=CARTESIAN_POINT('Ctrl Pts',(-4.1923339003649,-1.,0.253646344052521));
#36817=CARTESIAN_POINT('Ctrl Pts',(-4.19097151819241,-1.,0.252860861572565));
#36818=CARTESIAN_POINT('Ctrl Pts',(-4.18824585244066,-1.,0.251293239837692));
#36819=CARTESIAN_POINT('Ctrl Pts',(-4.18415464959491,-1.,0.248951836910963));
#36820=CARTESIAN_POINT('Ctrl Pts',(-4.17869430192868,-1.,0.245850033418583));
#36821=CARTESIAN_POINT('Ctrl Pts',(-4.17185984409533,-1.,0.242006283923911));
#36822=CARTESIAN_POINT('Ctrl Pts',(-4.1650163665385,-1.,0.238196140933976));
#36823=CARTESIAN_POINT('Ctrl Pts',(-4.1581638926525,-1.,0.234419749543143));
#36824=CARTESIAN_POINT('Ctrl Pts',(-4.15130247435029,-1.,0.230677299028738));
#36825=CARTESIAN_POINT('Ctrl Pts',(-4.14443220607733,-1.,0.226969025061243));
#36826=CARTESIAN_POINT('Ctrl Pts',(-4.13755320553563,-1.,0.223295201038383));
#36827=CARTESIAN_POINT('Ctrl Pts',(-4.13066558698156,-1.,0.219656126701851));
#36828=CARTESIAN_POINT('Ctrl Pts',(-4.12376943492249,-1.,0.216052116898425));
#36829=CARTESIAN_POINT('Ctrl Pts',(-4.11686478264545,-1.,0.212483491087068));
#36830=CARTESIAN_POINT('Ctrl Pts',(-4.10995157639026,-1.,0.208950559400172));
#36831=CARTESIAN_POINT('Ctrl Pts',(-4.10302969965374,-1.,0.205453622198233));
#36832=CARTESIAN_POINT('Ctrl Pts',(-4.09609903751912,-1.,0.201992979049984));
#36833=CARTESIAN_POINT('Ctrl Pts',(-4.08915953359753,-1.,0.19856893480081));
#36834=CARTESIAN_POINT('Ctrl Pts',(-4.08221124060385,-1.,0.195181806054714));
#36835=CARTESIAN_POINT('Ctrl Pts',(-4.07525439703137,-1.,0.191831928181081));
#36836=CARTESIAN_POINT('Ctrl Pts',(-4.06828941192308,-1.,0.188519658060255));
#36837=CARTESIAN_POINT('Ctrl Pts',(-4.06131670998589,-1.,0.185245370038948));
#36838=CARTESIAN_POINT('Ctrl Pts',(-4.05433660358402,-1.,0.18200945304855));
#36839=CARTESIAN_POINT('Ctrl Pts',(-4.04734916719722,-1.,0.178812307240715));
#36840=CARTESIAN_POINT('Ctrl Pts',(-4.04035407891161,-1.,0.175654339673757));
#36841=CARTESIAN_POINT('Ctrl Pts',(-4.03335057326093,-1.,0.172535962484466));
#36842=CARTESIAN_POINT('Ctrl Pts',(-4.0263377970371,-1.,0.169457601001653));
#36843=CARTESIAN_POINT('Ctrl Pts',(-4.01931510507143,-1.,0.166419700015847));
#36844=CARTESIAN_POINT('Ctrl Pts',(-4.01228237022301,-1.,0.163422730287458));
#36845=CARTESIAN_POINT('Ctrl Pts',(-4.00524031064509,-1.,0.160467194882219));
#36846=CARTESIAN_POINT('Ctrl Pts',(-3.99819074631874,-1.,0.157553634383809));
#36847=CARTESIAN_POINT('Ctrl Pts',(-3.99113582086059,-1.,0.154682618338563));
#36848=CARTESIAN_POINT('Ctrl Pts',(-3.9840772985098,-1.,0.151854737441405));
#36849=CARTESIAN_POINT('Ctrl Pts',(-3.97701581473643,-1.,0.149070594803543));
#36850=CARTESIAN_POINT('Ctrl Pts',(-3.96995018565891,-1.,0.146330797814513));
#36851=CARTESIAN_POINT('Ctrl Pts',(-3.96287658098896,-1.,0.143635947692791));
#36852=CARTESIAN_POINT('Ctrl Pts',(-3.95579014116899,-1.,0.140986665829937));
#36853=CARTESIAN_POINT('Ctrl Pts',(-3.94868667844355,-1.,0.138383621255159));
#36854=CARTESIAN_POINT('Ctrl Pts',(-3.94156445130744,-1.,0.135827558661188));
#36855=CARTESIAN_POINT('Ctrl Pts',(-3.93442567551035,-1.,0.133319322794189));
#36856=CARTESIAN_POINT('Ctrl Pts',(-3.9272787679596,-1.,0.130859892027798));
#36857=CARTESIAN_POINT('Ctrl Pts',(-3.92013513251642,-1.,0.128450341339528));
#36858=CARTESIAN_POINT('Ctrl Pts',(-3.91300501605392,-1.,0.126091793324136));
#36859=CARTESIAN_POINT('Ctrl Pts',(-3.90589336320508,-1.,0.123785368272377));
#36860=CARTESIAN_POINT('Ctrl Pts',(-3.89879639336952,-1.,0.121532144765723));
#36861=CARTESIAN_POINT('Ctrl Pts',(-3.89169600105201,-1.,0.119333088190417));
#36862=CARTESIAN_POINT('Ctrl Pts',(-3.88456590045767,-1.,0.117189150373144));
#36863=CARTESIAN_POINT('Ctrl Pts',(-3.87738168405343,-1.,0.11510142664947));
#36864=CARTESIAN_POINT('Ctrl Pts',(-3.87013043445014,-1.,0.113071304914561));
#36865=CARTESIAN_POINT('Ctrl Pts',(-3.86281867282965,-1.,0.11110059303626));
#36866=CARTESIAN_POINT('Ctrl Pts',(-3.855485714969,-1.,0.109191717634943));
#36867=CARTESIAN_POINT('Ctrl Pts',(-3.84819233070317,-1.,0.107347597812183));
#36868=CARTESIAN_POINT('Ctrl Pts',(-3.84099658324803,-1.,0.105571360916569));
#36869=CARTESIAN_POINT('Ctrl Pts',(-3.83393171228002,-1.,0.103866063811622));
#36870=CARTESIAN_POINT('Ctrl Pts',(-3.82698737143255,-1.,0.102234506488456));
#36871=CARTESIAN_POINT('Ctrl Pts',(-3.82007889742625,-1.,0.100678769650632));
#36872=CARTESIAN_POINT('Ctrl Pts',(-3.81306649386461,-1.,0.0992008728096513));
#36873=CARTESIAN_POINT('Ctrl Pts',(-3.80581088847809,-1.,0.0978042222906642));
#36874=CARTESIAN_POINT('Ctrl Pts',(-3.79822128513845,-1.,0.0964949352873131));
#36875=CARTESIAN_POINT('Ctrl Pts',(-3.79030016353111,-1.,0.09528298851008));
#36876=CARTESIAN_POINT('Ctrl Pts',(-3.782205218991,-1.,0.0941840095090813));
#36877=CARTESIAN_POINT('Ctrl Pts',(-3.77424159971059,-1.,0.0932185546203178));
#36878=CARTESIAN_POINT('Ctrl Pts',(-3.76678860031841,-1.,0.092409058960269));
#36879=CARTESIAN_POINT('Ctrl Pts',(-3.76024199359303,-1.,0.0917773084998334));
#36880=CARTESIAN_POINT('Ctrl Pts',(-3.75495560118212,-1.,0.0913419622736397));
#36881=CARTESIAN_POINT('Ctrl Pts',(-3.75145357872422,-1.,0.0911323999574425));
#36882=CARTESIAN_POINT('Ctrl Pts',(-3.74976844886346,-1.,0.0911090736805509));
#36883=CARTESIAN_POINT('Ctrl Pts',(-3.74911539914542,-1.,0.0911666301812817));
#36884=CARTESIAN_POINT('Ctrl Pts',(-3.74892890040975,-1.,0.0912308016421982));
#36885=CARTESIAN_POINT('Ctrl Pts',(-3.74888939116255,-1.,0.0912596999166822));
#36886=CARTESIAN_POINT('',(-3.74888939116259,-1.,-0.0912596999148858));
#36887=CARTESIAN_POINT('Origin',(0.,-1.,0.));
#36888=CARTESIAN_POINT('',(-4.1923339003649,-1.,-0.253646344052522));
#36889=CARTESIAN_POINT('Ctrl Pts',(-3.74888939116259,-1.,-0.0912596999148858));
#36890=CARTESIAN_POINT('Ctrl Pts',(-3.74892890041021,-1.,-0.0912308016409232));
#36891=CARTESIAN_POINT('Ctrl Pts',(-3.74911539914664,-1.,-0.0911666301806425));
#36892=CARTESIAN_POINT('Ctrl Pts',(-3.74976844886495,-1.,-0.0911090736804571));
#36893=CARTESIAN_POINT('Ctrl Pts',(-3.75145357872511,-1.,-0.0911323999576144));
#36894=CARTESIAN_POINT('Ctrl Pts',(-3.75495560118053,-1.,-0.0913419622735852));
#36895=CARTESIAN_POINT('Ctrl Pts',(-3.76024199359493,-1.,-0.0917773084999007));
#36896=CARTESIAN_POINT('Ctrl Pts',(-3.76678860032228,-1.,-0.0924090589604056));
#36897=CARTESIAN_POINT('Ctrl Pts',(-3.77424159971456,-1.,-0.0932185546204574));
#36898=CARTESIAN_POINT('Ctrl Pts',(-3.78220521899366,-1.,-0.0941840095091744));
#36899=CARTESIAN_POINT('Ctrl Pts',(-3.79030016353186,-1.,-0.0952829885101068));
#36900=CARTESIAN_POINT('Ctrl Pts',(-3.7982212851376,-1.,-0.0964949352872844));
#36901=CARTESIAN_POINT('Ctrl Pts',(-3.80581088847642,-1.,-0.0978042222906075));
#36902=CARTESIAN_POINT('Ctrl Pts',(-3.81306649386293,-1.,-0.0992008728095943));
#36903=CARTESIAN_POINT('Ctrl Pts',(-3.82007889742512,-1.,-0.100678769650594));
#36904=CARTESIAN_POINT('Ctrl Pts',(-3.8269873714322,-1.,-0.102234506488445));
#36905=CARTESIAN_POINT('Ctrl Pts',(-3.83393171228034,-1.,-0.103866063811634));
#36906=CARTESIAN_POINT('Ctrl Pts',(-3.84099658324873,-1.,-0.105571360916593));
#36907=CARTESIAN_POINT('Ctrl Pts',(-3.84819233070391,-1.,-0.107347597812208));
#36908=CARTESIAN_POINT('Ctrl Pts',(-3.85548571496953,-1.,-0.109191717634961));
#36909=CARTESIAN_POINT('Ctrl Pts',(-3.86281867282984,-1.,-0.111100593036267));
#36910=CARTESIAN_POINT('Ctrl Pts',(-3.87013043445001,-1.,-0.113071304914559));
#36911=CARTESIAN_POINT('Ctrl Pts',(-3.87738168405308,-1.,-0.115101426649461));
#36912=CARTESIAN_POINT('Ctrl Pts',(-3.88456590045726,-1.,-0.117189150373134));
#36913=CARTESIAN_POINT('Ctrl Pts',(-3.8916960010517,-1.,-0.11933308819041));
#36914=CARTESIAN_POINT('Ctrl Pts',(-3.89879639336939,-1.,-0.121532144765721));
#36915=CARTESIAN_POINT('Ctrl Pts',(-3.90589336320515,-1.,-0.12378536827238));
#36916=CARTESIAN_POINT('Ctrl Pts',(-3.91300501605411,-1.,-0.126091793324141));
#36917=CARTESIAN_POINT('Ctrl Pts',(-3.92013513251664,-1.,-0.128450341339532));
#36918=CARTESIAN_POINT('Ctrl Pts',(-3.92727876795977,-1.,-0.130859892027801));
#36919=CARTESIAN_POINT('Ctrl Pts',(-3.93442567551042,-1.,-0.133319322794191));
#36920=CARTESIAN_POINT('Ctrl Pts',(-3.94156445130741,-1.,-0.135827558661188));
#36921=CARTESIAN_POINT('Ctrl Pts',(-3.94868667844347,-1.,-0.138383621255161));
#36922=CARTESIAN_POINT('Ctrl Pts',(-3.95579014116894,-1.,-0.140986665829942));
#36923=CARTESIAN_POINT('Ctrl Pts',(-3.96287658098896,-1.,-0.143635947692799));
#36924=CARTESIAN_POINT('Ctrl Pts',(-3.96995018565893,-1.,-0.14633079781452));
#36925=CARTESIAN_POINT('Ctrl Pts',(-3.97701581473644,-1.,-0.149070594803545));
#36926=CARTESIAN_POINT('Ctrl Pts',(-3.98407729850975,-1.,-0.151854737441398));
#36927=CARTESIAN_POINT('Ctrl Pts',(-3.99113582086043,-1.,-0.154682618338547));
#36928=CARTESIAN_POINT('Ctrl Pts',(-3.9981907463185,-1.,-0.15755363438379));
#36929=CARTESIAN_POINT('Ctrl Pts',(-4.00524031064487,-1.,-0.160467194882203));
#36930=CARTESIAN_POINT('Ctrl Pts',(-4.01228237022296,-1.,-0.163422730287456));
#36931=CARTESIAN_POINT('Ctrl Pts',(-4.01931510507167,-1.,-0.166419700015866));
#36932=CARTESIAN_POINT('Ctrl Pts',(-4.02633779703764,-1.,-0.169457601001691));
#36933=CARTESIAN_POINT('Ctrl Pts',(-4.03335057326163,-1.,-0.172535962484514));
#36934=CARTESIAN_POINT('Ctrl Pts',(-4.04035407891222,-1.,-0.175654339673797));
#36935=CARTESIAN_POINT('Ctrl Pts',(-4.04734916719741,-1.,-0.178812307240728));
#36936=CARTESIAN_POINT('Ctrl Pts',(-4.05433660358353,-1.,-0.18200945304852));
#36937=CARTESIAN_POINT('Ctrl Pts',(-4.06131670998469,-1.,-0.185245370038874));
#36938=CARTESIAN_POINT('Ctrl Pts',(-4.06828941192148,-1.,-0.188519658060155));
#36939=CARTESIAN_POINT('Ctrl Pts',(-4.07525439702992,-1.,-0.191831928180991));
#36940=CARTESIAN_POINT('Ctrl Pts',(-4.08221124060322,-1.,-0.195181806054676));
#36941=CARTESIAN_POINT('Ctrl Pts',(-4.08915953359833,-1.,-0.198568934800862));
#36942=CARTESIAN_POINT('Ctrl Pts',(-4.09609903752152,-1.,-0.201992979050136));
#36943=CARTESIAN_POINT('Ctrl Pts',(-4.10302969965728,-1.,-0.205453622198455));
#36944=CARTESIAN_POINT('Ctrl Pts',(-4.10995157639377,-1.,-0.208950559400392));
#36945=CARTESIAN_POINT('Ctrl Pts',(-4.11686478264739,-1.,-0.21248349108719));
#36946=CARTESIAN_POINT('Ctrl Pts',(-4.12376943492132,-1.,-0.216052116898352));
#36947=CARTESIAN_POINT('Ctrl Pts',(-4.13066558697658,-1.,-0.219656126701541));
#36948=CARTESIAN_POINT('Ctrl Pts',(-4.13755320552764,-1.,-0.223295201037886));
#36949=CARTESIAN_POINT('Ctrl Pts',(-4.14443220606869,-1.,-0.226969025060705));
#36950=CARTESIAN_POINT('Ctrl Pts',(-4.15130247434459,-1.,-0.230677299028383));
#36951=CARTESIAN_POINT('Ctrl Pts',(-4.15816389265352,-1.,-0.234419749543208));
#36952=CARTESIAN_POINT('Ctrl Pts',(-4.16501636654877,-1.,-0.238196140934616));
#36953=CARTESIAN_POINT('Ctrl Pts',(-4.17185984411426,-1.,-0.242006283925088));
#36954=CARTESIAN_POINT('Ctrl Pts',(-4.1786943019518,-1.,-0.245850033420019));
#36955=CARTESIAN_POINT('Ctrl Pts',(-4.18415464961466,-1.,-0.248951836912189));
#36956=CARTESIAN_POINT('Ctrl Pts',(-4.18824585245272,-1.,-0.251293239838441));
#36957=CARTESIAN_POINT('Ctrl Pts',(-4.19097151819684,-1.,-0.25286086157284));
#36958=CARTESIAN_POINT('Ctrl Pts',(-4.1923339003649,-1.,-0.253646344052522));
#36959=CARTESIAN_POINT('',(-4.18039834341342,-1.,-0.40530197431835));
#36960=CARTESIAN_POINT('',(-4.1923339003649,-1.,-0.253646344052522));
#36961=CARTESIAN_POINT('',(-3.71701050416825,-1.,-0.496319364827592));
#36962=CARTESIAN_POINT('Ctrl Pts',(-4.18039834341342,-1.,-0.40530197431835));
#36963=CARTESIAN_POINT('Ctrl Pts',(-4.17892985789466,-1.,-0.40586466267921));
#36964=CARTESIAN_POINT('Ctrl Pts',(-4.17599251954382,-1.,-0.406986596325455));
#36965=CARTESIAN_POINT('Ctrl Pts',(-4.17158541007977,-1.,-0.408659167568273));
#36966=CARTESIAN_POINT('Ctrl Pts',(-4.16570705938425,-1.,-0.410868596146414));
#36967=CARTESIAN_POINT('Ctrl Pts',(-4.15835545017202,-1.,-0.41359587795147));
#36968=CARTESIAN_POINT('Ctrl Pts',(-4.15100018949965,-1.,-0.416288556008012));
#36969=CARTESIAN_POINT('Ctrl Pts',(-4.14364132317121,-1.,-0.418946490667703));
#36970=CARTESIAN_POINT('Ctrl Pts',(-4.13627893207002,-1.,-0.421569503104513));
#36971=CARTESIAN_POINT('Ctrl Pts',(-4.12891314634572,-1.,-0.424157375323975));
#36972=CARTESIAN_POINT('Ctrl Pts',(-4.12154412502007,-1.,-0.426709855707));
#36973=CARTESIAN_POINT('Ctrl Pts',(-4.11417202783267,-1.,-0.429226666075845));
#36974=CARTESIAN_POINT('Ctrl Pts',(-4.10679698750336,-1.,-0.431707508679884));
#36975=CARTESIAN_POINT('Ctrl Pts',(-4.09941908688373,-1.,-0.43415207320046));
#36976=CARTESIAN_POINT('Ctrl Pts',(-4.09203832139089,-1.,-0.436560044913482));
#36977=CARTESIAN_POINT('Ctrl Pts',(-4.08465462294273,-1.,-0.438931108931279));
#36978=CARTESIAN_POINT('Ctrl Pts',(-4.07726792490016,-1.,-0.44126495139636));
#36979=CARTESIAN_POINT('Ctrl Pts',(-4.0698782192569,-1.,-0.443561262395333));
#36980=CARTESIAN_POINT('Ctrl Pts',(-4.06248560760659,-1.,-0.445819737468538));
#36981=CARTESIAN_POINT('Ctrl Pts',(-4.0550903779696,-1.,-0.448040082684114));
#36982=CARTESIAN_POINT('Ctrl Pts',(-4.0476929901813,-1.,-0.450222009543926));
#36983=CARTESIAN_POINT('Ctrl Pts',(-4.04029392228049,-1.,-0.452365214748892));
#36984=CARTESIAN_POINT('Ctrl Pts',(-4.03289354362794,-1.,-0.454469363020542));
#36985=CARTESIAN_POINT('Ctrl Pts',(-4.02549199038394,-1.,-0.456534070784951));
#36986=CARTESIAN_POINT('Ctrl Pts',(-4.01808900827587,-1.,-0.458558885636945));
#36987=CARTESIAN_POINT('Ctrl Pts',(-4.01068390573399,-1.,-0.460543280768515));
#36988=CARTESIAN_POINT('Ctrl Pts',(-4.00327590659075,-1.,-0.462486702616205));
#36989=CARTESIAN_POINT('Ctrl Pts',(-3.9958644432011,-1.,-0.464388610938975));
#36990=CARTESIAN_POINT('Ctrl Pts',(-3.98844946363262,-1.,-0.46624852088304));
#36991=CARTESIAN_POINT('Ctrl Pts',(-3.98103175589371,-1.,-0.468066047920157));
#36992=CARTESIAN_POINT('Ctrl Pts',(-3.97361320212436,-1.,-0.469840942829895));
#36993=CARTESIAN_POINT('Ctrl Pts',(-3.96619600864643,-1.,-0.471572978413503));
#36994=CARTESIAN_POINT('Ctrl Pts',(-3.95878201038338,-1.,-0.473261847236297));
#36995=CARTESIAN_POINT('Ctrl Pts',(-3.95137192932897,-1.,-0.47490705302179));
#36996=CARTESIAN_POINT('Ctrl Pts',(-3.94396469119383,-1.,-0.476507810658537));
#36997=CARTESIAN_POINT('Ctrl Pts',(-3.93655660689819,-1.,-0.478062927140964));
#36998=CARTESIAN_POINT('Ctrl Pts',(-3.92914297392071,-1.,-0.479571028525579));
#36999=CARTESIAN_POINT('Ctrl Pts',(-3.92171976072341,-1.,-0.481030798910748));
#37000=CARTESIAN_POINT('Ctrl Pts',(-3.91428536373751,-1.,-0.482441230340713));
#37001=CARTESIAN_POINT('Ctrl Pts',(-3.90684210358056,-1.,-0.48380183508915));
#37002=CARTESIAN_POINT('Ctrl Pts',(-3.89939844658513,-1.,-0.485112963522222));
#37003=CARTESIAN_POINT('Ctrl Pts',(-3.89196582437552,-1.,-0.486375337854103));
#37004=CARTESIAN_POINT('Ctrl Pts',(-3.88455453328138,-1.,-0.487589452275154));
#37005=CARTESIAN_POINT('Ctrl Pts',(-3.87716963231109,-1.,-0.488754973798274));
#37006=CARTESIAN_POINT('Ctrl Pts',(-3.86980755613707,-1.,-0.489870245704918));
#37007=CARTESIAN_POINT('Ctrl Pts',(-3.86245057319246,-1.,-0.490931482170891));
#37008=CARTESIAN_POINT('Ctrl Pts',(-3.85507287020263,-1.,-0.491933631083813));
#37009=CARTESIAN_POINT('Ctrl Pts',(-3.84765051147999,-1.,-0.492871792414141));
#37010=CARTESIAN_POINT('Ctrl Pts',(-3.84017095578451,-1.,-0.493742574629134));
#37011=CARTESIAN_POINT('Ctrl Pts',(-3.83264092682431,-1.,-0.494545212256401));
#37012=CARTESIAN_POINT('Ctrl Pts',(-3.82509963594103,-1.,-0.495283458893837));
#37013=CARTESIAN_POINT('Ctrl Pts',(-3.81760756144025,-1.,-0.49596393787548));
#37014=CARTESIAN_POINT('Ctrl Pts',(-3.81022254090839,-1.,-0.496592643443704));
#37015=CARTESIAN_POINT('Ctrl Pts',(-3.80297788298514,-1.,-0.497171756201052));
#37016=CARTESIAN_POINT('Ctrl Pts',(-3.79586380669994,-1.,-0.497696892100625));
#37017=CARTESIAN_POINT('Ctrl Pts',(-3.78879701661264,-1.,-0.498152751800958));
#37018=CARTESIAN_POINT('Ctrl Pts',(-3.78163975337356,-1.,-0.498515471679585));
#37019=CARTESIAN_POINT('Ctrl Pts',(-3.77425499225255,-1.,-0.498759900365892));
#37020=CARTESIAN_POINT('Ctrl Pts',(-3.76655401191229,-1.,-0.49886579233529));
#37021=CARTESIAN_POINT('Ctrl Pts',(-3.75854082221053,-1.,-0.498823681615422));
#37022=CARTESIAN_POINT('Ctrl Pts',(-3.75037362167839,-1.,-0.498642802042606));
#37023=CARTESIAN_POINT('Ctrl Pts',(-3.74235701734714,-1.,-0.498350586057692));
#37024=CARTESIAN_POINT('Ctrl Pts',(-3.73486914372449,-1.,-0.497984209510024));
#37025=CARTESIAN_POINT('Ctrl Pts',(-3.72830430904606,-1.,-0.497584067153049));
#37026=CARTESIAN_POINT('Ctrl Pts',(-3.72301489774398,-1.,-0.497187079575988));
#37027=CARTESIAN_POINT('Ctrl Pts',(-3.71952320822499,-1.,-0.496846224822563));
#37028=CARTESIAN_POINT('Ctrl Pts',(-3.71785517607549,-1.,-0.496605651525989));
#37029=CARTESIAN_POINT('Ctrl Pts',(-3.71721917030355,-1.,-0.496446644158005));
#37030=CARTESIAN_POINT('Ctrl Pts',(-3.71704500630495,-1.,-0.496354087924313));
#37031=CARTESIAN_POINT('Ctrl Pts',(-3.71701050416825,-1.,-0.496319364827592));
#37032=CARTESIAN_POINT('',(-3.68845817949618,-1.,-0.676591647973661));
#37033=CARTESIAN_POINT('Origin',(0.,-1.,0.));
#37034=CARTESIAN_POINT('',(-4.10104028313088,-1.,-0.906349047628866));
#37035=CARTESIAN_POINT('Ctrl Pts',(-3.68845817949618,-1.,-0.676591647973661));
#37036=CARTESIAN_POINT('Ctrl Pts',(-3.68850172300543,-1.,-0.67656928609342));
#37037=CARTESIAN_POINT('Ctrl Pts',(-3.68869596426099,-1.,-0.676535079520365));
#37038=CARTESIAN_POINT('Ctrl Pts',(-3.68934997767391,-1.,-0.676580391119535));
#37039=CARTESIAN_POINT('Ctrl Pts',(-3.6910107117555,-1.,-0.676867042599711));
#37040=CARTESIAN_POINT('Ctrl Pts',(-3.69443683573443,-1.,-0.677621861865196));
#37041=CARTESIAN_POINT('Ctrl Pts',(-3.69959004073192,-1.,-0.678878822226389));
#37042=CARTESIAN_POINT('Ctrl Pts',(-3.70595722032165,-1.,-0.680526909711617));
#37043=CARTESIAN_POINT('Ctrl Pts',(-3.71319182790334,-1.,-0.682492345109689));
#37044=CARTESIAN_POINT('Ctrl Pts',(-3.7209063713952,-1.,-0.684691698168355));
#37045=CARTESIAN_POINT('Ctrl Pts',(-3.72872973554125,-1.,-0.687043475232499));
#37046=CARTESIAN_POINT('Ctrl Pts',(-3.73636374474993,-1.,-0.689479637354651));
#37047=CARTESIAN_POINT('Ctrl Pts',(-3.74365508986548,-1.,-0.691960080400503));
#37048=CARTESIAN_POINT('Ctrl Pts',(-3.7506028824329,-1.,-0.694474562581173));
#37049=CARTESIAN_POINT('Ctrl Pts',(-3.75729775766913,-1.,-0.69703124565953));
#37050=CARTESIAN_POINT('Ctrl Pts',(-3.76387780603725,-1.,-0.699648552230851));
#37051=CARTESIAN_POINT('Ctrl Pts',(-3.77048141872904,-1.,-0.702346356621613));
#37052=CARTESIAN_POINT('Ctrl Pts',(-3.77719254217197,-1.,-0.705135847999949));
#37053=CARTESIAN_POINT('Ctrl Pts',(-3.78402183336678,-1.,-0.7080158793756));
#37054=CARTESIAN_POINT('Ctrl Pts',(-3.79093694007146,-1.,-0.710978231689117));
#37055=CARTESIAN_POINT('Ctrl Pts',(-3.79788100314994,-1.,-0.714010733006677));
#37056=CARTESIAN_POINT('Ctrl Pts',(-3.80479445759296,-1.,-0.717100993669091));
#37057=CARTESIAN_POINT('Ctrl Pts',(-3.81163885127309,-1.,-0.720240466589172));
#37058=CARTESIAN_POINT('Ctrl Pts',(-3.81840802610795,-1.,-0.723426346019349));
#37059=CARTESIAN_POINT('Ctrl Pts',(-3.82511495756682,-1.,-0.726659281876608));
#37060=CARTESIAN_POINT('Ctrl Pts',(-3.8317839240337,-1.,-0.729942010490145));
#37061=CARTESIAN_POINT('Ctrl Pts',(-3.83844103658016,-1.,-0.73327770375609));
#37062=CARTESIAN_POINT('Ctrl Pts',(-3.84510432881231,-1.,-0.736668240497151));
#37063=CARTESIAN_POINT('Ctrl Pts',(-3.85177770351237,-1.,-0.740113146827176));
#37064=CARTESIAN_POINT('Ctrl Pts',(-3.85845645217611,-1.,-0.743610542737042));
#37065=CARTESIAN_POINT('Ctrl Pts',(-3.86513062969896,-1.,-0.747157716488884));
#37066=CARTESIAN_POINT('Ctrl Pts',(-3.87178914078372,-1.,-0.750751822383023));
#37067=CARTESIAN_POINT('Ctrl Pts',(-3.87842382520058,-1.,-0.754390577396846));
#37068=CARTESIAN_POINT('Ctrl Pts',(-3.88503262662684,-1.,-0.758072800564798));
#37069=CARTESIAN_POINT('Ctrl Pts',(-3.89161738162245,-1.,-0.761798028793978));
#37070=CARTESIAN_POINT('Ctrl Pts',(-3.89818233104381,-1.,-0.765566256401306));
#37071=CARTESIAN_POINT('Ctrl Pts',(-3.90473237182634,-1.,-0.769377629847876));
#37072=CARTESIAN_POINT('Ctrl Pts',(-3.91127138115238,-1.,-0.773232154506305));
#37073=CARTESIAN_POINT('Ctrl Pts',(-3.91780062334464,-1.,-0.777129415664915));
#37074=CARTESIAN_POINT('Ctrl Pts',(-3.92431956510418,-1.,-0.781068718228395));
#37075=CARTESIAN_POINT('Ctrl Pts',(-3.93082655631768,-1.,-0.785049202786458));
#37076=CARTESIAN_POINT('Ctrl Pts',(-3.93731956885671,-1.,-0.789069971469323));
#37077=CARTESIAN_POINT('Ctrl Pts',(-3.94379688971307,-1.,-0.793130205641017));
#37078=CARTESIAN_POINT('Ctrl Pts',(-3.95025788827189,-1.,-0.797229296085438));
#37079=CARTESIAN_POINT('Ctrl Pts',(-3.95670276375176,-1.,-0.801366797727206));
#37080=CARTESIAN_POINT('Ctrl Pts',(-3.96313222295874,-1.,-0.805542372178496));
#37081=CARTESIAN_POINT('Ctrl Pts',(-3.96954717513251,-1.,-0.809755732818134));
#37082=CARTESIAN_POINT('Ctrl Pts',(-3.97594844078763,-1.,-0.814006592328737));
#37083=CARTESIAN_POINT('Ctrl Pts',(-3.98233640155287,-1.,-0.818294599022033));
#37084=CARTESIAN_POINT('Ctrl Pts',(-3.98871104646328,-1.,-0.822619346021769));
#37085=CARTESIAN_POINT('Ctrl Pts',(-3.99507212784289,-1.,-0.826980400320473));
#37086=CARTESIAN_POINT('Ctrl Pts',(-4.00141928477447,-1.,-0.831377325741487));
#37087=CARTESIAN_POINT('Ctrl Pts',(-4.00775216907934,-1.,-0.835809705809821));
#37088=CARTESIAN_POINT('Ctrl Pts',(-4.01407059766338,-1.,-0.84027717197638));
#37089=CARTESIAN_POINT('Ctrl Pts',(-4.02037456798787,-1.,-0.844779403288517));
#37090=CARTESIAN_POINT('Ctrl Pts',(-4.02666418343508,-1.,-0.849316107475012));
#37091=CARTESIAN_POINT('Ctrl Pts',(-4.03293960436945,-1.,-0.853887006632178));
#37092=CARTESIAN_POINT('Ctrl Pts',(-4.03920099284658,-1.,-0.858491822322571));
#37093=CARTESIAN_POINT('Ctrl Pts',(-4.04544845048097,-1.,-0.863130256642173));
#37094=CARTESIAN_POINT('Ctrl Pts',(-4.05168199437128,-1.,-0.867801988858176));
#37095=CARTESIAN_POINT('Ctrl Pts',(-4.05790159030495,-1.,-0.872506694780563));
#37096=CARTESIAN_POINT('Ctrl Pts',(-4.06410717232347,-1.,-0.877244060484595));
#37097=CARTESIAN_POINT('Ctrl Pts',(-4.07029866694292,-1.,-0.882013797525916));
#37098=CARTESIAN_POINT('Ctrl Pts',(-4.07647601774639,-1.,-0.886815658360739));
#37099=CARTESIAN_POINT('Ctrl Pts',(-4.08263920306651,-1.,-0.891649447920401));
#37100=CARTESIAN_POINT('Ctrl Pts',(-4.08878822249095,-1.,-0.896515019236368));
#37101=CARTESIAN_POINT('Ctrl Pts',(-4.09369611524319,-1.,-0.900432820945975));
#37102=CARTESIAN_POINT('Ctrl Pts',(-4.09737067247114,-1.,-0.903385402444212));
#37103=CARTESIAN_POINT('Ctrl Pts',(-4.09981755067956,-1.,-0.905360112216302));
#37104=CARTESIAN_POINT('Ctrl Pts',(-4.10104028313088,-1.,-0.906349047628866));
#37105=CARTESIAN_POINT('',(-4.06552750530042,-1.,-1.05427041296137));
#37106=CARTESIAN_POINT('',(-4.10104028313088,-1.,-0.906349047628866));
#37107=CARTESIAN_POINT('',(-3.59360648251073,-1.,-1.07167739962028));
#37108=CARTESIAN_POINT('Ctrl Pts',(-4.06552750530042,-1.,-1.05427041296137));
#37109=CARTESIAN_POINT('Ctrl Pts',(-4.06398907542249,-1.,-1.05459645194823));
#37110=CARTESIAN_POINT('Ctrl Pts',(-4.06091239149123,-1.,-1.05524507177599));
#37111=CARTESIAN_POINT('Ctrl Pts',(-4.05629789307025,-1.,-1.05620762707996));
#37112=CARTESIAN_POINT('Ctrl Pts',(-4.05014628384869,-1.,-1.05747027727959));
#37113=CARTESIAN_POINT('Ctrl Pts',(-4.04245854427496,-1.,-1.05901393666566));
#37114=CARTESIAN_POINT('Ctrl Pts',(-4.03477261141553,-1.,-1.06052284711857));
#37115=CARTESIAN_POINT('Ctrl Pts',(-4.02708855235633,-1.,-1.06199687787462));
#37116=CARTESIAN_POINT('Ctrl Pts',(-4.01940647495943,-1.,-1.06343586496236));
#37117=CARTESIAN_POINT('Ctrl Pts',(-4.01172654187398,-1.,-1.06483961343109));
#37118=CARTESIAN_POINT('Ctrl Pts',(-4.00404894952579,-1.,-1.06620789963606));
#37119=CARTESIAN_POINT('Ctrl Pts',(-3.99637389920441,-1.,-1.06754047381312));
#37120=CARTESIAN_POINT('Ctrl Pts',(-3.98870156857412,-1.,-1.06883706263941));
#37121=CARTESIAN_POINT('Ctrl Pts',(-3.98103208801101,-1.,-1.07009737257767));
#37122=CARTESIAN_POINT('Ctrl Pts',(-3.9733655022223,-1.,-1.07132109206164));
#37123=CARTESIAN_POINT('Ctrl Pts',(-3.96570179322338,-1.,-1.07250789943007));
#37124=CARTESIAN_POINT('Ctrl Pts',(-3.95804094429373,-1.,-1.07365747426491));
#37125=CARTESIAN_POINT('Ctrl Pts',(-3.95038299600676,-1.,-1.07476950921587));
#37126=CARTESIAN_POINT('Ctrl Pts',(-3.94272809633331,-1.,-1.07584371946443));
#37127=CARTESIAN_POINT('Ctrl Pts',(-3.93507657572883,-1.,-1.07687985975384));
#37128=CARTESIAN_POINT('Ctrl Pts',(-3.9274289334984,-1.,-1.07787771707195));
#37129=CARTESIAN_POINT('Ctrl Pts',(-3.91978568924178,-1.,-1.07883706663554));
#37130=CARTESIAN_POINT('Ctrl Pts',(-3.91214726022143,-1.,-1.07975763507473));
#37131=CARTESIAN_POINT('Ctrl Pts',(-3.90451384092545,-1.,-1.08063906483818));
#37132=CARTESIAN_POINT('Ctrl Pts',(-3.8968852509835,-1.,-1.08148086931358));
#37133=CARTESIAN_POINT('Ctrl Pts',(-3.88926088975114,-1.,-1.08228241999346));
#37134=CARTESIAN_POINT('Ctrl Pts',(-3.88164007721312,-1.,-1.08304304871028));
#37135=CARTESIAN_POINT('Ctrl Pts',(-3.8740223372254,-1.,-1.08376213307504));
#37136=CARTESIAN_POINT('Ctrl Pts',(-3.86640769434274,-1.,-1.08443918607927));
#37137=CARTESIAN_POINT('Ctrl Pts',(-3.85879698702532,-1.,-1.08507395120059));
#37138=CARTESIAN_POINT('Ctrl Pts',(-3.85119211322755,-1.,-1.08566647671844));
#37139=CARTESIAN_POINT('Ctrl Pts',(-3.8435952876495,-1.,-1.08621688337604));
#37140=CARTESIAN_POINT('Ctrl Pts',(-3.83600837071708,-1.,-1.08672515456902));
#37141=CARTESIAN_POINT('Ctrl Pts',(-3.82843215316984,-1.,-1.08719091307558));
#37142=CARTESIAN_POINT('Ctrl Pts',(-3.82086569676319,-1.,-1.08761321539442));
#37143=CARTESIAN_POINT('Ctrl Pts',(-3.81330554446323,-1.,-1.08799030610862));
#37144=CARTESIAN_POINT('Ctrl Pts',(-3.8057472665766,-1.,-1.0883200925538));
#37145=CARTESIAN_POINT('Ctrl Pts',(-3.79818708705259,-1.,-1.08860064435778));
#37146=CARTESIAN_POINT('Ctrl Pts',(-3.79062357974404,-1.,-1.08883071512098));
#37147=CARTESIAN_POINT('Ctrl Pts',(-3.78305911299504,-1.,-1.08901018614636));
#37148=CARTESIAN_POINT('Ctrl Pts',(-3.77550199409424,-1.,-1.0891407279127));
#37149=CARTESIAN_POINT('Ctrl Pts',(-3.76796340094448,-1.,-1.08922484204256));
#37150=CARTESIAN_POINT('Ctrl Pts',(-3.76045342580208,-1.,-1.08926462734281));
#37151=CARTESIAN_POINT('Ctrl Pts',(-3.75297711748132,-1.,-1.08926054632925));
#37152=CARTESIAN_POINT('Ctrl Pts',(-3.74553121371757,-1.,-1.08921040494017));
#37153=CARTESIAN_POINT('Ctrl Pts',(-3.73809879348239,-1.,-1.08910769013297));
#37154=CARTESIAN_POINT('Ctrl Pts',(-3.73065515162988,-1.,-1.08894337390937));
#37155=CARTESIAN_POINT('Ctrl Pts',(-3.72317741369398,-1.,-1.08870887220082));
#37156=CARTESIAN_POINT('Ctrl Pts',(-3.71565372339075,-1.,-1.0883988733478));
#37157=CARTESIAN_POINT('Ctrl Pts',(-3.70809084139457,-1.,-1.08801367312185));
#37158=CARTESIAN_POINT('Ctrl Pts',(-3.70052690909833,-1.,-1.08756311291309));
#37159=CARTESIAN_POINT('Ctrl Pts',(-3.69302062410157,-1.,-1.08706319540271));
#37160=CARTESIAN_POINT('Ctrl Pts',(-3.68562817420797,-1.,-1.0865288888259));
#37161=CARTESIAN_POINT('Ctrl Pts',(-3.67838211685117,-1.,-1.0859675575576));
#37162=CARTESIAN_POINT('Ctrl Pts',(-3.67127347729666,-1.,-1.0853733414449));
#37163=CARTESIAN_POINT('Ctrl Pts',(-3.66422237895365,-1.,-1.08471809922901));
#37164=CARTESIAN_POINT('Ctrl Pts',(-3.65709649161166,-1.,-1.08395671077807));
#37165=CARTESIAN_POINT('Ctrl Pts',(-3.64976441208358,-1.,-1.08304289898623));
#37166=CARTESIAN_POINT('Ctrl Pts',(-3.64214167843677,-1.,-1.08194278850996));
#37167=CARTESIAN_POINT('Ctrl Pts',(-3.63423373196529,-1.,-1.08064765719867));
#37168=CARTESIAN_POINT('Ctrl Pts',(-3.62619537902361,-1.,-1.07919137290742));
#37169=CARTESIAN_POINT('Ctrl Pts',(-3.61832318504574,-1.,-1.07764868137619));
#37170=CARTESIAN_POINT('Ctrl Pts',(-3.61098481349204,-1.,-1.07611545402734));
#37171=CARTESIAN_POINT('Ctrl Pts',(-3.60456339887778,-1.,-1.07469327168578));
#37172=CARTESIAN_POINT('Ctrl Pts',(-3.59940121154535,-1.,-1.07347372545714));
#37173=CARTESIAN_POINT('Ctrl Pts',(-3.59600583194946,-1.,-1.07259084660936));
#37174=CARTESIAN_POINT('Ctrl Pts',(-3.59439596999862,-1.,-1.07209229745229));
#37175=CARTESIAN_POINT('Ctrl Pts',(-3.59379266874567,-1.,-1.07183575450617));
#37176=CARTESIAN_POINT('Ctrl Pts',(-3.5936351279798,-1.,-1.07171709254135));
#37177=CARTESIAN_POINT('Ctrl Pts',(-3.59360648251073,-1.,-1.07167739962028));
#37178=CARTESIAN_POINT('',(-3.5372048861597,-1.,-1.24526366418038));
#37179=CARTESIAN_POINT('Origin',(0.,-1.,0.));
#37180=CARTESIAN_POINT('',(-3.90876544355381,-1.,-1.53673442965256));
#37181=CARTESIAN_POINT('Ctrl Pts',(-3.5372048861597,-1.,-1.24526366418038));
#37182=CARTESIAN_POINT('Ctrl Pts',(-3.53725139174486,-1.,-1.24524838931757));
#37183=CARTESIAN_POINT('Ctrl Pts',(-3.5374485926552,-1.,-1.2452449899111));
#37184=CARTESIAN_POINT('Ctrl Pts',(-3.53808746578196,-1.,-1.24539205388767));
#37185=CARTESIAN_POINT('Ctrl Pts',(-3.53968291130022,-1.,-1.24593497226008));
#37186=CARTESIAN_POINT('Ctrl Pts',(-3.54294877425964,-1.,-1.24721646231966));
#37187=CARTESIAN_POINT('Ctrl Pts',(-3.54784190283068,-1.,-1.24926408628003));
#37188=CARTESIAN_POINT('Ctrl Pts',(-3.55387287418985,-1.,-1.2518879294064));
#37189=CARTESIAN_POINT('Ctrl Pts',(-3.56071094991199,-1.,-1.25496090900009));
#37190=CARTESIAN_POINT('Ctrl Pts',(-3.56798645995275,-1.,-1.25834000485716));
#37191=CARTESIAN_POINT('Ctrl Pts',(-3.5753456065171,-1.,-1.2618866714281));
#37192=CARTESIAN_POINT('Ctrl Pts',(-3.58250452868618,-1.,-1.26548706249862));
#37193=CARTESIAN_POINT('Ctrl Pts',(-3.58931807846313,-1.,-1.26907758484709));
#37194=CARTESIAN_POINT('Ctrl Pts',(-3.59578698050006,-1.,-1.27264798379307));
#37195=CARTESIAN_POINT('Ctrl Pts',(-3.60199947736298,-1.,-1.27622049908625));
#37196=CARTESIAN_POINT('Ctrl Pts',(-3.60808907746339,-1.,-1.27983492861691));
#37197=CARTESIAN_POINT('Ctrl Pts',(-3.61418935913823,-1.,-1.28353255117765));
#37198=CARTESIAN_POINT('Ctrl Pts',(-3.6203814849236,-1.,-1.28733755029384));
#37199=CARTESIAN_POINT('Ctrl Pts',(-3.62667616004369,-1.,-1.29125046021878));
#37200=CARTESIAN_POINT('Ctrl Pts',(-3.63304271631046,-1.,-1.29525810207762));
#37201=CARTESIAN_POINT('Ctrl Pts',(-3.63942689872808,-1.,-1.2993395590647));
#37202=CARTESIAN_POINT('Ctrl Pts',(-3.64577181380113,-1.,-1.30347327603774));
#37203=CARTESIAN_POINT('Ctrl Pts',(-3.65204081987068,-1.,-1.30764479590039));
#37204=CARTESIAN_POINT('Ctrl Pts',(-3.65822827358617,-1.,-1.31185038411218));
#37205=CARTESIAN_POINT('Ctrl Pts',(-3.66434688899793,-1.,-1.31609271239911));
#37206=CARTESIAN_POINT('Ctrl Pts',(-3.67042021752656,-1.,-1.32037828137766));
#37207=CARTESIAN_POINT('Ctrl Pts',(-3.67647355257912,-1.,-1.32471430856415));
#37208=CARTESIAN_POINT('Ctrl Pts',(-3.68252441182551,-1.,-1.3291054707274));
#37209=CARTESIAN_POINT('Ctrl Pts',(-3.68857672413033,-1.,-1.33355191034523));
#37210=CARTESIAN_POINT('Ctrl Pts',(-3.69462613305708,-1.,-1.33805103398219));
#37211=CARTESIAN_POINT('Ctrl Pts',(-3.70066324015119,-1.,-1.34259860752933));
#37212=CARTESIAN_POINT('Ctrl Pts',(-3.70667753188248,-1.,-1.34719008463534));
#37213=CARTESIAN_POINT('Ctrl Pts',(-3.71266130563054,-1.,-1.35182193384424));
#37214=CARTESIAN_POINT('Ctrl Pts',(-3.71861271513313,-1.,-1.35649266705037));
#37215=CARTESIAN_POINT('Ctrl Pts',(-3.72453364678279,-1.,-1.36120211416354));
#37216=CARTESIAN_POINT('Ctrl Pts',(-3.73042829011295,-1.,-1.36595093298676));
#37217=CARTESIAN_POINT('Ctrl Pts',(-3.7363014588581,-1.,-1.37074003422739));
#37218=CARTESIAN_POINT('Ctrl Pts',(-3.74215698162555,-1.,-1.37557002971687));
#37219=CARTESIAN_POINT('Ctrl Pts',(-3.74799617204729,-1.,-1.38044070763295));
#37220=CARTESIAN_POINT('Ctrl Pts',(-3.75381861212707,-1.,-1.38535129801176));
#37221=CARTESIAN_POINT('Ctrl Pts',(-3.75962280650855,-1.,-1.39030069388918));
#37222=CARTESIAN_POINT('Ctrl Pts',(-3.76540689249074,-1.,-1.39528769118052));
#37223=CARTESIAN_POINT('Ctrl Pts',(-3.77116930621827,-1.,-1.40031121335505));
#37224=CARTESIAN_POINT('Ctrl Pts',(-3.77690952014259,-1.,-1.40537056004722));
#37225=CARTESIAN_POINT('Ctrl Pts',(-3.78262780065471,-1.,-1.41046532282593));
#37226=CARTESIAN_POINT('Ctrl Pts',(-3.78832489879426,-1.,-1.4155952780383));
#37227=CARTESIAN_POINT('Ctrl Pts',(-3.79400175744408,-1.,-1.42076028482836));
#37228=CARTESIAN_POINT('Ctrl Pts',(-3.7996592319632,-1.,-1.42596018777283));
#37229=CARTESIAN_POINT('Ctrl Pts',(-3.80529775429805,-1.,-1.4311946992132));
#37230=CARTESIAN_POINT('Ctrl Pts',(-3.81091737726815,-1.,-1.43646341556724));
#37231=CARTESIAN_POINT('Ctrl Pts',(-3.81651792398414,-1.,-1.44176587041347));
#37232=CARTESIAN_POINT('Ctrl Pts',(-3.82209910620533,-1.,-1.44710157648539));
#37233=CARTESIAN_POINT('Ctrl Pts',(-3.82766064519074,-1.,-1.45247006796836));
#37234=CARTESIAN_POINT('Ctrl Pts',(-3.83320241775423,-1.,-1.45787095220852));
#37235=CARTESIAN_POINT('Ctrl Pts',(-3.83872447159639,-1.,-1.46330391180752));
#37236=CARTESIAN_POINT('Ctrl Pts',(-3.84422695454796,-1.,-1.46876867426504));
#37237=CARTESIAN_POINT('Ctrl Pts',(-3.84971006847277,-1.,-1.47426499018538));
#37238=CARTESIAN_POINT('Ctrl Pts',(-3.85517401698843,-1.,-1.4797926099102));
#37239=CARTESIAN_POINT('Ctrl Pts',(-3.86061894706087,-1.,-1.48535125509919));
#37240=CARTESIAN_POINT('Ctrl Pts',(-3.86604492575189,-1.,-1.4909406116431));
#37241=CARTESIAN_POINT('Ctrl Pts',(-3.87145196998465,-1.,-1.49656035399122));
#37242=CARTESIAN_POINT('Ctrl Pts',(-3.87684006372134,-1.,-1.50221016176556));
#37243=CARTESIAN_POINT('Ctrl Pts',(-3.88220917950538,-1.,-1.50788973857757));
#37244=CARTESIAN_POINT('Ctrl Pts',(-3.88755930033884,-1.,-1.51359883110559));
#37245=CARTESIAN_POINT('Ctrl Pts',(-3.89289043533657,-1.,-1.51933724329305));
#37246=CARTESIAN_POINT('Ctrl Pts',(-3.89820260708225,-1.,-1.52510482991635));
#37247=CARTESIAN_POINT('Ctrl Pts',(-3.90243719631596,-1.,-1.52974216056287));
#37248=CARTESIAN_POINT('Ctrl Pts',(-3.90560462813969,-1.,-1.53323321827755));
#37249=CARTESIAN_POINT('Ctrl Pts',(-3.90771246855019,-1.,-1.53556639217905));
#37250=CARTESIAN_POINT('Ctrl Pts',(-3.90876544355381,-1.,-1.53673442965256));
#37251=CARTESIAN_POINT('',(-3.85054988729471,-1.,-1.67727921511438));
#37252=CARTESIAN_POINT('',(-3.90876544355381,-1.,-1.53673442965256));
#37253=CARTESIAN_POINT('',(-3.38171594275765,-1.,-1.62064718014094));
#37254=CARTESIAN_POINT('Ctrl Pts',(-3.85054988729471,-1.,-1.67727921511438));
#37255=CARTESIAN_POINT('Ctrl Pts',(-3.84897939430696,-1.,-1.67736057656533));
#37256=CARTESIAN_POINT('Ctrl Pts',(-3.84583912296459,-1.,-1.6775199114018));
#37257=CARTESIAN_POINT('Ctrl Pts',(-3.84113085985244,-1.,-1.67774874946079));
#37258=CARTESIAN_POINT('Ctrl Pts',(-3.83485746513989,-1.,-1.67803353064351));
#37259=CARTESIAN_POINT('Ctrl Pts',(-3.82702289286713,-1.,-1.6783555575934));
#37260=CARTESIAN_POINT('Ctrl Pts',(-3.81919554099578,-1.,-1.67864354605954));
#37261=CARTESIAN_POINT('Ctrl Pts',(-3.81137549624178,-1.,-1.6788973773827));
#37262=CARTESIAN_POINT('Ctrl Pts',(-3.80356289079005,-1.,-1.67911690648355));
#37263=CARTESIAN_POINT('Ctrl Pts',(-3.79575791578424,-1.,-1.67930196625548));
#37264=CARTESIAN_POINT('Ctrl Pts',(-3.7879608002176,-1.,-1.67945236653493));
#37265=CARTESIAN_POINT('Ctrl Pts',(-3.78017178197317,-1.,-1.67956789212141));
#37266=CARTESIAN_POINT('Ctrl Pts',(-3.77239107928502,-1.,-1.67964830084993));
#37267=CARTESIAN_POINT('Ctrl Pts',(-3.76461886684344,-1.,-1.67969332319245));
#37268=CARTESIAN_POINT('Ctrl Pts',(-3.75685523754493,-1.,-1.67970265841239));
#37269=CARTESIAN_POINT('Ctrl Pts',(-3.7491002239452,-1.,-1.67967598599525));
#37270=CARTESIAN_POINT('Ctrl Pts',(-3.74135385965401,-1.,-1.6796129868522));
#37271=CARTESIAN_POINT('Ctrl Pts',(-3.73361623282543,-1.,-1.67951336376402));
#37272=CARTESIAN_POINT('Ctrl Pts',(-3.72588753416396,-1.,-1.67937685856652));
#37273=CARTESIAN_POINT('Ctrl Pts',(-3.71816812842322,-1.,-1.67920328071708));
#37274=CARTESIAN_POINT('Ctrl Pts',(-3.71045854208343,-1.,-1.67899249793462));
#37275=CARTESIAN_POINT('Ctrl Pts',(-3.70275932351108,-1.,-1.67874436948667));
#37276=CARTESIAN_POINT('Ctrl Pts',(-3.6950709275959,-1.,-1.67845869064323));
#37277=CARTESIAN_POINT('Ctrl Pts',(-3.68739360236487,-1.,-1.67813513867965));
#37278=CARTESIAN_POINT('Ctrl Pts',(-3.67972724579124,-1.,-1.67777320475848));
#37279=CARTESIAN_POINT('Ctrl Pts',(-3.67207136294575,-1.,-1.67737217414874));
#37280=CARTESIAN_POINT('Ctrl Pts',(-3.66442538670968,-1.,-1.67693128053132));
#37281=CARTESIAN_POINT('Ctrl Pts',(-3.6567889441642,-1.,-1.67644983469449));
#37282=CARTESIAN_POINT('Ctrl Pts',(-3.64916213574667,-1.,-1.67592735946692));
#37283=CARTESIAN_POINT('Ctrl Pts',(-3.6415458297234,-1.,-1.67536373264848));
#37284=CARTESIAN_POINT('Ctrl Pts',(-3.63394189312924,-1.,-1.67475929882971));
#37285=CARTESIAN_POINT('Ctrl Pts',(-3.62635249450923,-1.,-1.67411452372271));
#37286=CARTESIAN_POINT('Ctrl Pts',(-3.61877947398184,-1.,-1.67342968196224));
#37287=CARTESIAN_POINT('Ctrl Pts',(-3.61122367156181,-1.,-1.67270452466968));
#37288=CARTESIAN_POINT('Ctrl Pts',(-3.603684308152,-1.,-1.67193797318597));
#37289=CARTESIAN_POINT('Ctrl Pts',(-3.59615824388807,-1.,-1.67112775290707));
#37290=CARTESIAN_POINT('Ctrl Pts',(-3.58864143097834,-1.,-1.67027110397604));
#37291=CARTESIAN_POINT('Ctrl Pts',(-3.58113044183829,-1.,-1.66936552908232));
#37292=CARTESIAN_POINT('Ctrl Pts',(-3.57362406285887,-1.,-1.668409574073));
#37293=CARTESIAN_POINT('Ctrl Pts',(-3.56612465179422,-1.,-1.66740349220305));
#37294=CARTESIAN_POINT('Ctrl Pts',(-3.55864015233602,-1.,-1.66635023293114));
#37295=CARTESIAN_POINT('Ctrl Pts',(-3.55118121342861,-1.,-1.66525401568994));
#37296=CARTESIAN_POINT('Ctrl Pts',(-3.54375747475014,-1.,-1.66411849222326));
#37297=CARTESIAN_POINT('Ctrl Pts',(-3.5363738506022,-1.,-1.66294490916111));
#37298=CARTESIAN_POINT('Ctrl Pts',(-3.52902746211093,-1.,-1.66173058912371));
#37299=CARTESIAN_POINT('Ctrl Pts',(-3.52170261543815,-1.,-1.66046645222279));
#37300=CARTESIAN_POINT('Ctrl Pts',(-3.5143763218894,-1.,-1.65913971687342));
#37301=CARTESIAN_POINT('Ctrl Pts',(-3.50702733146542,-1.,-1.65773832633632));
#37302=CARTESIAN_POINT('Ctrl Pts',(-3.4996447647794,-1.,-1.65625517961588));
#37303=CARTESIAN_POINT('Ctrl Pts',(-3.49223525300176,-1.,-1.65469162644468));
#37304=CARTESIAN_POINT('Ctrl Pts',(-3.48483492840894,-1.,-1.65306335367739));
#37305=CARTESIAN_POINT('Ctrl Pts',(-3.47749926256476,-1.,-1.65139534930322));
#37306=CARTESIAN_POINT('Ctrl Pts',(-3.47028140995992,-1.,-1.64971118698256));
#37307=CARTESIAN_POINT('Ctrl Pts',(-3.46321237515,-1.,-1.64802323352738));
#37308=CARTESIAN_POINT('Ctrl Pts',(-3.45628421062422,-1.,-1.64632429697521));
#37309=CARTESIAN_POINT('Ctrl Pts',(-3.44942242546795,-1.,-1.64457408708107));
#37310=CARTESIAN_POINT('Ctrl Pts',(-3.44250337701888,-1.,-1.64270733821113));
#37311=CARTESIAN_POINT('Ctrl Pts',(-3.43540451921548,-1.,-1.64065778702023));
#37312=CARTESIAN_POINT('Ctrl Pts',(-3.42804772926291,-1.,-1.63837876246926));
#37313=CARTESIAN_POINT('Ctrl Pts',(-3.42043974590882,-1.,-1.63586250099773));
#37314=CARTESIAN_POINT('Ctrl Pts',(-3.41272817148478,-1.,-1.63316667054044));
#37315=CARTESIAN_POINT('Ctrl Pts',(-3.40519422740235,-1.,-1.63041148964828));
#37316=CARTESIAN_POINT('Ctrl Pts',(-3.39818605297991,-1.,-1.62774916464408));
#37317=CARTESIAN_POINT('Ctrl Pts',(-3.39206617496906,-1.,-1.62533996116713));
#37318=CARTESIAN_POINT('Ctrl Pts',(-3.38715832179072,-1.,-1.6233278855625));
#37319=CARTESIAN_POINT('Ctrl Pts',(-3.38394285763222,-1.,-1.62192472202769));
#37320=CARTESIAN_POINT('Ctrl Pts',(-3.38243080602409,-1.,-1.62118047294498));
#37321=CARTESIAN_POINT('Ctrl Pts',(-3.38187506456922,-1.,-1.62083271135947));
#37322=CARTESIAN_POINT('Ctrl Pts',(-3.38173802621259,-1.,-1.62069086551492));
#37323=CARTESIAN_POINT('Ctrl Pts',(-3.38171594275765,-1.,-1.62064718014094));
#37324=CARTESIAN_POINT('',(-3.29885386921599,-1.,-1.78327315618183));
#37325=CARTESIAN_POINT('Origin',(0.,-1.,0.));
#37326=CARTESIAN_POINT('',(-3.62024382630768,-1.,-2.12928030988903));
#37327=CARTESIAN_POINT('Ctrl Pts',(-3.29885386921599,-1.,-1.78327315618183));
#37328=CARTESIAN_POINT('Ctrl Pts',(-3.29890219175522,-1.,-1.78326534445426));
#37329=CARTESIAN_POINT('Ctrl Pts',(-3.29909749657945,-1.,-1.78329283591903));
#37330=CARTESIAN_POINT('Ctrl Pts',(-3.29970549824337,-1.,-1.78353803106983));
#37331=CARTESIAN_POINT('Ctrl Pts',(-3.30119637003466,-1.,-1.7843238478823));
#37332=CARTESIAN_POINT('Ctrl Pts',(-3.30422155558973,-1.,-1.78610045419769));
#37333=CARTESIAN_POINT('Ctrl Pts',(-3.30873412266954,-1.,-1.78888832245965));
#37334=CARTESIAN_POINT('Ctrl Pts',(-3.31428038326763,-1.,-1.79242331350137));
#37335=CARTESIAN_POINT('Ctrl Pts',(-3.32055355101168,-1.,-1.79652817033444));
#37336=CARTESIAN_POINT('Ctrl Pts',(-3.3272108803981,-1.,-1.80100380443535));
#37337=CARTESIAN_POINT('Ctrl Pts',(-3.33392460276874,-1.,-1.80565802981138));
#37338=CARTESIAN_POINT('Ctrl Pts',(-3.34043216147532,-1.,-1.81033399625311));
#37339=CARTESIAN_POINT('Ctrl Pts',(-3.34660014370527,-1.,-1.81494618732772));
#37340=CARTESIAN_POINT('Ctrl Pts',(-3.35243086937451,-1.,-1.81948458796748));
#37341=CARTESIAN_POINT('Ctrl Pts',(-3.35800801557326,-1.,-1.82398496829247));
#37342=CARTESIAN_POINT('Ctrl Pts',(-3.36345722124127,-1.,-1.82850752153182));
#37343=CARTESIAN_POINT('Ctrl Pts',(-3.36890396271864,-1.,-1.83311391452338));
#37344=CARTESIAN_POINT('Ctrl Pts',(-3.37442462015914,-1.,-1.83784072967111));
#37345=CARTESIAN_POINT('Ctrl Pts',(-3.38002968341222,-1.,-1.84269016931679));
#37346=CARTESIAN_POINT('Ctrl Pts',(-3.38569092349639,-1.,-1.84764441927778));
#37347=CARTESIAN_POINT('Ctrl Pts',(-3.39135802549415,-1.,-1.85267433291778));
#37348=CARTESIAN_POINT('Ctrl Pts',(-3.39697816833056,-1.,-1.85774972037055));
#37349=CARTESIAN_POINT('Ctrl Pts',(-3.40251742305445,-1.,-1.86285057051228));
#37350=CARTESIAN_POINT('Ctrl Pts',(-3.40797080000513,-1.,-1.86797231196635));
#37351=CARTESIAN_POINT('Ctrl Pts',(-3.41335043875182,-1.,-1.87311957248106));
#37352=CARTESIAN_POINT('Ctrl Pts',(-3.4186785838376,-1.,-1.87830245689338));
#37353=CARTESIAN_POINT('Ctrl Pts',(-3.42397908819741,-1.,-1.88353205062063));
#37354=CARTESIAN_POINT('Ctrl Pts',(-3.42926852222174,-1.,-1.88881571322018));
#37355=CARTESIAN_POINT('Ctrl Pts',(-3.43455074411591,-1.,-1.89415420002553));
#37356=CARTESIAN_POINT('Ctrl Pts',(-3.43982185678105,-1.,-1.89954426803392));
#37357=CARTESIAN_POINT('Ctrl Pts',(-3.44507323983374,-1.,-1.90498026502308));
#37358=CARTESIAN_POINT('Ctrl Pts',(-3.45029522038885,-1.,-1.91045605593638));
#37359=CARTESIAN_POINT('Ctrl Pts',(-3.45548074309943,-1.,-1.9159669478406));
#37360=CARTESIAN_POINT('Ctrl Pts',(-3.4606282172248,-1.,-1.9215111821321));
#37361=CARTESIAN_POINT('Ctrl Pts',(-3.46573953254084,-1.,-1.92708888591159));
#37362=CARTESIAN_POINT('Ctrl Pts',(-3.47081872409783,-1.,-1.93270136427083));
#37363=CARTESIAN_POINT('Ctrl Pts',(-3.47587040389916,-1.,-1.93835026973888));
#37364=CARTESIAN_POINT('Ctrl Pts',(-3.48089825770411,-1.,-1.94403680554062));
#37365=CARTESIAN_POINT('Ctrl Pts',(-3.485903616108,-1.,-1.94976096795902));
#37366=CARTESIAN_POINT('Ctrl Pts',(-3.49088618670967,-1.,-1.95552193112071));
#37367=CARTESIAN_POINT('Ctrl Pts',(-3.49584466573045,-1.,-1.96131836776489));
#37368=CARTESIAN_POINT('Ctrl Pts',(-3.50077740176262,-1.,-1.9671487972405));
#37369=CARTESIAN_POINT('Ctrl Pts',(-3.505683018611,-1.,-1.9730119116298));
#37370=CARTESIAN_POINT('Ctrl Pts',(-3.51056110478334,-1.,-1.97890693666316));
#37371=CARTESIAN_POINT('Ctrl Pts',(-3.51541198728362,-1.,-1.98483351061066));
#37372=CARTESIAN_POINT('Ctrl Pts',(-3.52023644289195,-1.,-1.99079153006143));
#37373=CARTESIAN_POINT('Ctrl Pts',(-3.52503542491745,-1.,-1.99678100339305));
#37374=CARTESIAN_POINT('Ctrl Pts',(-3.52980980250181,-1.,-2.00280191090341));
#37375=CARTESIAN_POINT('Ctrl Pts',(-3.53456004727321,-1.,-2.00885403604685));
#37376=CARTESIAN_POINT('Ctrl Pts',(-3.53928627453503,-1.,-2.0149369884727));
#37377=CARTESIAN_POINT('Ctrl Pts',(-3.54398838254011,-1.,-2.0210502798303));
#37378=CARTESIAN_POINT('Ctrl Pts',(-3.54866616282173,-1.,-2.02719338376144));
#37379=CARTESIAN_POINT('Ctrl Pts',(-3.55331941294018,-1.,-2.03336579658174));
#37380=CARTESIAN_POINT('Ctrl Pts',(-3.55794807265052,-1.,-2.03956711120099));
#37381=CARTESIAN_POINT('Ctrl Pts',(-3.5625522387181,-1.,-2.04579702159056));
#37382=CARTESIAN_POINT('Ctrl Pts',(-3.56713209978207,-1.,-2.0520552817309));
#37383=CARTESIAN_POINT('Ctrl Pts',(-3.57168789423507,-1.,-2.05834167687523));
#37384=CARTESIAN_POINT('Ctrl Pts',(-3.576219862243,-1.,-2.06465599229174));
#37385=CARTESIAN_POINT('Ctrl Pts',(-3.58072819250442,-1.,-2.07099797605747));
#37386=CARTESIAN_POINT('Ctrl Pts',(-3.58521300039299,-1.,-2.07736732842117));
#37387=CARTESIAN_POINT('Ctrl Pts',(-3.58967435355088,-1.,-2.08376373048756));
#37388=CARTESIAN_POINT('Ctrl Pts',(-3.59411228625588,-1.,-2.09018686331416));
#37389=CARTESIAN_POINT('Ctrl Pts',(-3.59852681775485,-1.,-2.09663642986631));
#37390=CARTESIAN_POINT('Ctrl Pts',(-3.60291797088734,-1.,-2.1031121772821));
#37391=CARTESIAN_POINT('Ctrl Pts',(-3.60728578532601,-1.,-2.10961391334462));
#37392=CARTESIAN_POINT('Ctrl Pts',(-3.61163030609447,-1.,-2.11614149815106));
#37393=CARTESIAN_POINT('Ctrl Pts',(-3.61508732216891,-1.,-2.12138417126355));
#37394=CARTESIAN_POINT('Ctrl Pts',(-3.61766963590482,-1.,-2.12532774376758));
#37395=CARTESIAN_POINT('Ctrl Pts',(-3.61938653649098,-1.,-2.12796193131368));
#37396=CARTESIAN_POINT('Ctrl Pts',(-3.62024382630768,-1.,-2.12928030988903));
#37397=CARTESIAN_POINT('',(-3.54075895182139,-1.,-2.25898783642071));
#37398=CARTESIAN_POINT('',(-3.62024382630768,-1.,-2.12928030988903));
#37399=CARTESIAN_POINT('',(-3.08655633322212,-1.,-2.1297112484669));
#37400=CARTESIAN_POINT('Ctrl Pts',(-3.54075895182139,-1.,-2.25898783642071));
#37401=CARTESIAN_POINT('Ctrl Pts',(-3.53919506647335,-1.,-2.2588225169468));
#37402=CARTESIAN_POINT('Ctrl Pts',(-3.53606853162228,-1.,-2.25848864343951));
#37403=CARTESIAN_POINT('Ctrl Pts',(-3.53138243688262,-1.,-2.25797812950104));
#37404=CARTESIAN_POINT('Ctrl Pts',(-3.52514172847711,-1.,-2.25727802940898));
#37405=CARTESIAN_POINT('Ctrl Pts',(-3.51735323667612,-1.,-2.25637049455044));
#37406=CARTESIAN_POINT('Ctrl Pts',(-3.50957720117341,-1.,-2.25543046979799));
#37407=CARTESIAN_POINT('Ctrl Pts',(-3.50181372617971,-1.,-2.25445785151868));
#37408=CARTESIAN_POINT('Ctrl Pts',(-3.49406296494791,-1.,-2.2534525170976));
#37409=CARTESIAN_POINT('Ctrl Pts',(-3.48632513240961,-1.,-2.25241433138695));
#37410=CARTESIAN_POINT('Ctrl Pts',(-3.47860048448691,-1.,-2.25134314238687));
#37411=CARTESIAN_POINT('Ctrl Pts',(-3.47088928979888,-1.,-2.25023877475942));
#37412=CARTESIAN_POINT('Ctrl Pts',(-3.46319180177573,-1.,-2.2491010234604));
#37413=CARTESIAN_POINT('Ctrl Pts',(-3.45550823512049,-1.,-2.2479296496077));
#37414=CARTESIAN_POINT('Ctrl Pts',(-3.44783872863151,-1.,-2.2467243706995));
#37415=CARTESIAN_POINT('Ctrl Pts',(-3.4401833646032,-1.,-2.24548487526022));
#37416=CARTESIAN_POINT('Ctrl Pts',(-3.43254222614803,-1.,-2.24421085338727));
#37417=CARTESIAN_POINT('Ctrl Pts',(-3.42491544683008,-1.,-2.24290202531101));
#37418=CARTESIAN_POINT('Ctrl Pts',(-3.41730325539172,-1.,-2.24155816587844));
#37419=CARTESIAN_POINT('Ctrl Pts',(-3.40970604190328,-1.,-2.24017914395289));
#37420=CARTESIAN_POINT('Ctrl Pts',(-3.40212434705647,-1.,-2.2387649112415));
#37421=CARTESIAN_POINT('Ctrl Pts',(-3.39455873448189,-1.,-2.23731541452791));
#37422=CARTESIAN_POINT('Ctrl Pts',(-3.38700968549563,-1.,-2.23583052276308));
#37423=CARTESIAN_POINT('Ctrl Pts',(-3.37947749555632,-1.,-2.23430995599561));
#37424=CARTESIAN_POINT('Ctrl Pts',(-3.37196214349304,-1.,-2.23275319569221));
#37425=CARTESIAN_POINT('Ctrl Pts',(-3.36446325227848,-1.,-2.23115945849739));
#37426=CARTESIAN_POINT('Ctrl Pts',(-3.35698038165483,-1.,-2.22952789880982));
#37427=CARTESIAN_POINT('Ctrl Pts',(-3.34951327111096,-1.,-2.22785777756576));
#37428=CARTESIAN_POINT('Ctrl Pts',(-3.34206209449375,-1.,-2.22614863918047));
#37429=CARTESIAN_POINT('Ctrl Pts',(-3.33462772849598,-1.,-2.22440049878511));
#37430=CARTESIAN_POINT('Ctrl Pts',(-3.3272119632604,-1.,-2.22261398879635));
#37431=CARTESIAN_POINT('Ctrl Pts',(-3.31981686778022,-1.,-2.22078990842776));
#37432=CARTESIAN_POINT('Ctrl Pts',(-3.31244421655666,-1.,-2.21892881679086));
#37433=CARTESIAN_POINT('Ctrl Pts',(-3.30509487819569,-1.,-2.21703059947836));
#37434=CARTESIAN_POINT('Ctrl Pts',(-3.29776825193159,-1.,-2.21509406923368));
#37435=CARTESIAN_POINT('Ctrl Pts',(-3.29046159238343,-1.,-2.21311648827391));
#37436=CARTESIAN_POINT('Ctrl Pts',(-3.28317133333131,-1.,-2.21109449750641));
#37437=CARTESIAN_POINT('Ctrl Pts',(-3.2758944800554,-1.,-2.2090250941743));
#37438=CARTESIAN_POINT('Ctrl Pts',(-3.26863006136782,-1.,-2.20690665217743));
#37439=CARTESIAN_POINT('Ctrl Pts',(-3.26138036637705,-1.,-2.20473979048678));
#37440=CARTESIAN_POINT('Ctrl Pts',(-3.25415277957775,-1.,-2.20252866491545));
#37441=CARTESIAN_POINT('Ctrl Pts',(-3.24695715874338,-1.,-2.20027910880981));
#37442=CARTESIAN_POINT('Ctrl Pts',(-3.23980245361308,-1.,-2.19799623693253));
#37443=CARTESIAN_POINT('Ctrl Pts',(-3.23269332296933,-1.,-2.19568204933168));
#37444=CARTESIAN_POINT('Ctrl Pts',(-3.22562734221646,-1.,-2.19333345123538));
#37445=CARTESIAN_POINT('Ctrl Pts',(-3.21859043114095,-1.,-2.19093901948667));
#37446=CARTESIAN_POINT('Ctrl Pts',(-3.21156188355769,-1.,-2.18848253363901));
#37447=CARTESIAN_POINT('Ctrl Pts',(-3.20452259717976,-1.,-2.18594876115934));
#37448=CARTESIAN_POINT('Ctrl Pts',(-3.19746293740411,-1.,-2.18332898656602));
#37449=CARTESIAN_POINT('Ctrl Pts',(-3.19038924261573,-1.,-2.18062558031778));
#37450=CARTESIAN_POINT('Ctrl Pts',(-3.18333474627807,-1.,-2.17785968847142));
#37451=CARTESIAN_POINT('Ctrl Pts',(-3.17635032802523,-1.,-2.17506466903694));
#37452=CARTESIAN_POINT('Ctrl Pts',(-3.16948480019497,-1.,-2.17227212063817));
#37453=CARTESIAN_POINT('Ctrl Pts',(-3.16276685102972,-1.,-2.16949910801219));
#37454=CARTESIAN_POINT('Ctrl Pts',(-3.15618975593656,-1.,-2.1667372844769));
#37455=CARTESIAN_POINT('Ctrl Pts',(-3.14968624389054,-1.,-2.16393520288072));
#37456=CARTESIAN_POINT('Ctrl Pts',(-3.14314440427022,-1.,-2.16100905914435));
#37457=CARTESIAN_POINT('Ctrl Pts',(-3.13645356563038,-1.,-2.15787423530676));
#37458=CARTESIAN_POINT('Ctrl Pts',(-3.12954386795646,-1.,-2.1544724138292));
#37459=CARTESIAN_POINT('Ctrl Pts',(-3.12242318151938,-1.,-2.15079698090585));
#37460=CARTESIAN_POINT('Ctrl Pts',(-3.11522827016855,-1.,-2.14692798457532));
#37461=CARTESIAN_POINT('Ctrl Pts',(-3.10821808668859,-1.,-2.14302815601973));
#37462=CARTESIAN_POINT('Ctrl Pts',(-3.10171267391049,-1.,-2.13930228863751));
#37463=CARTESIAN_POINT('Ctrl Pts',(-3.0960450242104,-1.,-2.13596538661048));
#37464=CARTESIAN_POINT('Ctrl Pts',(-3.09151235281963,-1.,-2.13321032560893));
#37465=CARTESIAN_POINT('Ctrl Pts',(-3.08855597949761,-1.,-2.13132142793017));
#37466=CARTESIAN_POINT('Ctrl Pts',(-3.08717896996099,-1.,-2.13034980480424));
#37467=CARTESIAN_POINT('Ctrl Pts',(-3.08668447250322,-1.,-2.12991938762374));
#37468=CARTESIAN_POINT('Ctrl Pts',(-3.08657131089497,-1.,-2.1297578506149));
#37469=CARTESIAN_POINT('Ctrl Pts',(-3.08655633322212,-1.,-2.1297112484669));
#37470=CARTESIAN_POINT('',(-2.97927412174388,-1.,-2.27737254473378));
#37471=CARTESIAN_POINT('Origin',(0.,-1.,0.));
#37472=CARTESIAN_POINT('',(-3.24257979115744,-1.,-2.66939624221984));
#37473=CARTESIAN_POINT('Ctrl Pts',(-2.97927412174388,-1.,-2.27737254473378));
#37474=CARTESIAN_POINT('Ctrl Pts',(-2.97932307137589,-1.,-2.27737238849212));
#37475=CARTESIAN_POINT('Ctrl Pts',(-2.97951167106106,-1.,-2.27743009389704));
#37476=CARTESIAN_POINT('Ctrl Pts',(-2.98007383024333,-1.,-2.27776738270369));
#37477=CARTESIAN_POINT('Ctrl Pts',(-2.98142341809623,-1.,-2.27877674853833));
#37478=CARTESIAN_POINT('Ctrl Pts',(-2.98413343613858,-1.,-2.28100472516582));
#37479=CARTESIAN_POINT('Ctrl Pts',(-2.98815432734929,-1.,-2.28446419116036));
#37480=CARTESIAN_POINT('Ctrl Pts',(-2.9930793098434,-1.,-2.28882328690601));
#37481=CARTESIAN_POINT('Ctrl Pts',(-2.99863310340004,-1.,-2.29385894577999));
#37482=CARTESIAN_POINT('Ctrl Pts',(-3.00450832658822,-1.,-2.29932091315939));
#37483=CARTESIAN_POINT('Ctrl Pts',(-3.01041131063882,-1.,-2.30496809486528));
#37484=CARTESIAN_POINT('Ctrl Pts',(-3.01610726819019,-1.,-2.31060449886577));
#37485=CARTESIAN_POINT('Ctrl Pts',(-3.02147780668029,-1.,-2.31612479121528));
#37486=CARTESIAN_POINT('Ctrl Pts',(-3.02652678416478,-1.,-2.32151944306299));
#37487=CARTESIAN_POINT('Ctrl Pts',(-3.03133125185047,-1.,-2.32683687412027));
#37488=CARTESIAN_POINT('Ctrl Pts',(-3.03600588555765,-1.,-2.33215619079807));
#37489=CARTESIAN_POINT('Ctrl Pts',(-3.04066496998569,-1.,-2.33755792953726));
#37490=CARTESIAN_POINT('Ctrl Pts',(-3.04537822217311,-1.,-2.3430901708402));
#37491=CARTESIAN_POINT('Ctrl Pts',(-3.05015565829976,-1.,-2.34875673090816));
#37492=CARTESIAN_POINT('Ctrl Pts',(-3.05497218368188,-1.,-2.35453559889506));
#37493=CARTESIAN_POINT('Ctrl Pts',(-3.05978266240056,-1.,-2.36039011602084));
#37494=CARTESIAN_POINT('Ctrl Pts',(-3.06453964643152,-1.,-2.36628220107001));
#37495=CARTESIAN_POINT('Ctrl Pts',(-3.06921275497472,-1.,-2.37218678163157));
#37496=CARTESIAN_POINT('Ctrl Pts',(-3.07379777492133,-1.,-2.37809856205524));
#37497=CARTESIAN_POINT('Ctrl Pts',(-3.07830597244301,-1.,-2.38402401216107));
#37498=CARTESIAN_POINT('Ctrl Pts',(-3.08275773747083,-1.,-2.38997659219192));
#37499=CARTESIAN_POINT('Ctrl Pts',(-3.08717489512919,-1.,-2.39597098250635));
#37500=CARTESIAN_POINT('Ctrl Pts',(-3.09157266051115,-1.,-2.40201704423352));
#37501=CARTESIAN_POINT('Ctrl Pts',(-3.09595472616093,-1.,-2.40811612696382));
#37502=CARTESIAN_POINT('Ctrl Pts',(-3.10031775027683,-1.,-2.41426441798067));
#37503=CARTESIAN_POINT('Ctrl Pts',(-3.10465410280902,-1.,-2.42045498612494));
#37504=CARTESIAN_POINT('Ctrl Pts',(-3.10895518969592,-1.,-2.42668025870013));
#37505=CARTESIAN_POINT('Ctrl Pts',(-3.11321477659012,-1.,-2.4329344968514));
#37506=CARTESIAN_POINT('Ctrl Pts',(-3.11743156744182,-1.,-2.43921571477975));
#37507=CARTESIAN_POINT('Ctrl Pts',(-3.12160740887768,-1.,-2.44552433364716));
#37508=CARTESIAN_POINT('Ctrl Pts',(-3.12574608210849,-1.,-2.45186227369848));
#37509=CARTESIAN_POINT('Ctrl Pts',(-3.12985188384372,-1.,-2.45823188859366));
#37510=CARTESIAN_POINT('Ctrl Pts',(-3.13392826623902,-1.,-2.4646349433237));
#37511=CARTESIAN_POINT('Ctrl Pts',(-3.13797654408931,-1.,-2.47107164236827));
#37512=CARTESIAN_POINT('Ctrl Pts',(-3.14199655778845,-1.,-2.47754112428027));
#37513=CARTESIAN_POINT('Ctrl Pts',(-3.1459872272388,-1.,-2.48404187418376));
#37514=CARTESIAN_POINT('Ctrl Pts',(-3.14994715298903,-1.,-2.49057217131985));
#37515=CARTESIAN_POINT('Ctrl Pts',(-3.15387518039064,-1.,-2.49713050858911));
#37516=CARTESIAN_POINT('Ctrl Pts',(-3.15777102413998,-1.,-2.50371605688287));
#37517=CARTESIAN_POINT('Ctrl Pts',(-3.16163506380211,-1.,-2.51032851007939));
#37518=CARTESIAN_POINT('Ctrl Pts',(-3.16546808277069,-1.,-2.51696788755615));
#37519=CARTESIAN_POINT('Ctrl Pts',(-3.16927102130751,-1.,-2.523634346718));
#37520=CARTESIAN_POINT('Ctrl Pts',(-3.17304474093574,-1.,-2.5303280040691));
#37521=CARTESIAN_POINT('Ctrl Pts',(-3.17678974135225,-1.,-2.53704871950871));
#37522=CARTESIAN_POINT('Ctrl Pts',(-3.18050619750515,-1.,-2.54379612552948));
#37523=CARTESIAN_POINT('Ctrl Pts',(-3.18419408529482,-1.,-2.55056972387638));
#37524=CARTESIAN_POINT('Ctrl Pts',(-3.1878532811617,-1.,-2.55736896206016));
#37525=CARTESIAN_POINT('Ctrl Pts',(-3.19148366395201,-1.,-2.56419331092909));
#37526=CARTESIAN_POINT('Ctrl Pts',(-3.19508523784548,-1.,-2.57104235898053));
#37527=CARTESIAN_POINT('Ctrl Pts',(-3.19865814628955,-1.,-2.577915819091));
#37528=CARTESIAN_POINT('Ctrl Pts',(-3.20220261408685,-1.,-2.58481347777953));
#37529=CARTESIAN_POINT('Ctrl Pts',(-3.20571891028879,-1.,-2.59173516023605));
#37530=CARTESIAN_POINT('Ctrl Pts',(-3.2092073056959,-1.,-2.59868069194267));
#37531=CARTESIAN_POINT('Ctrl Pts',(-3.21266802609297,-1.,-2.60564985359699));
#37532=CARTESIAN_POINT('Ctrl Pts',(-3.21610123232465,-1.,-2.61264236718662));
#37533=CARTESIAN_POINT('Ctrl Pts',(-3.21950704108654,-1.,-2.61965792832396));
#37534=CARTESIAN_POINT('Ctrl Pts',(-3.222885536128,-1.,-2.62669622735548));
#37535=CARTESIAN_POINT('Ctrl Pts',(-3.22623678292539,-1.,-2.63375697391438));
#37536=CARTESIAN_POINT('Ctrl Pts',(-3.2295608435934,-1.,-2.64083992182478));
#37537=CARTESIAN_POINT('Ctrl Pts',(-3.23285778738558,-1.,-2.64794488744246));
#37538=CARTESIAN_POINT('Ctrl Pts',(-3.23612768065687,-1.,-2.6550717396303));
#37539=CARTESIAN_POINT('Ctrl Pts',(-3.23872200036311,-1.,-2.6607906631973));
#37540=CARTESIAN_POINT('Ctrl Pts',(-3.24065561087681,-1.,-2.66508964664767));
#37541=CARTESIAN_POINT('Ctrl Pts',(-3.24193929584813,-1.,-2.66795998539861));
#37542=CARTESIAN_POINT('Ctrl Pts',(-3.24257979115744,-1.,-2.66939624221984));
#37543=CARTESIAN_POINT('',(-3.14378277984898,-1.,-2.78507268004356));
#37544=CARTESIAN_POINT('',(-3.24257979115744,-1.,-2.66939624221984));
#37545=CARTESIAN_POINT('',(-2.71539546306948,-1.,-2.58633475774921));
#37546=CARTESIAN_POINT('Ctrl Pts',(-3.14378277984898,-1.,-2.78507268004356));
#37547=CARTESIAN_POINT('Ctrl Pts',(-3.14226401018816,-1.,-2.7846647503589));
#37548=CARTESIAN_POINT('Ctrl Pts',(-3.13922819749279,-1.,-2.78384588958165));
#37549=CARTESIAN_POINT('Ctrl Pts',(-3.13467965833037,-1.,-2.78260859419319));
#37550=CARTESIAN_POINT('Ctrl Pts',(-3.12862530318457,-1.,-2.78094085161413));
#37551=CARTESIAN_POINT('Ctrl Pts',(-3.12107467037201,-1.,-2.77882610146731));
#37552=CARTESIAN_POINT('Ctrl Pts',(-3.11354142303921,-1.,-2.77668121002545));
#37553=CARTESIAN_POINT('Ctrl Pts',(-3.10602568032564,-1.,-2.77450609123362));
#37554=CARTESIAN_POINT('Ctrl Pts',(-3.0985276127786,-1.,-2.77230064796057));
#37555=CARTESIAN_POINT('Ctrl Pts',(-3.09104745382531,-1.,-2.7700647803451));
#37556=CARTESIAN_POINT('Ctrl Pts',(-3.08358548001504,-1.,-2.76779837829373));
#37557=CARTESIAN_POINT('Ctrl Pts',(-3.07614198408862,-1.,-2.76550131064852));
#37558=CARTESIAN_POINT('Ctrl Pts',(-3.0687172484321,-1.,-2.76317341453493));
#37559=CARTESIAN_POINT('Ctrl Pts',(-3.06131152247454,-1.,-2.76081448759882));
#37560=CARTESIAN_POINT('Ctrl Pts',(-3.05392498749847,-1.,-2.75842427252931));
#37561=CARTESIAN_POINT('Ctrl Pts',(-3.04655777351067,-1.,-2.75600247455925));
#37562=CARTESIAN_POINT('Ctrl Pts',(-3.03921001107977,-1.,-2.75354880060314));
#37563=CARTESIAN_POINT('Ctrl Pts',(-3.03188187589107,-1.,-2.75106299522979));
#37564=CARTESIAN_POINT('Ctrl Pts',(-3.02457362909245,-1.,-2.7485448718414));
#37565=CARTESIAN_POINT('Ctrl Pts',(-3.01728567646611,-1.,-2.74599436193625));
#37566=CARTESIAN_POINT('Ctrl Pts',(-3.01001855960162,-1.,-2.74341150239887));
#37567=CARTESIAN_POINT('Ctrl Pts',(-3.00277284351521,-1.,-2.74079632883931));
#37568=CARTESIAN_POINT('Ctrl Pts',(-2.99554902409778,-1.,-2.73814878711641));
#37569=CARTESIAN_POINT('Ctrl Pts',(-2.9883474369644,-1.,-2.73546864694536));
#37570=CARTESIAN_POINT('Ctrl Pts',(-2.98116814232129,-1.,-2.73275539286497));
#37571=CARTESIAN_POINT('Ctrl Pts',(-2.97401089032677,-1.,-2.73000819218414));
#37572=CARTESIAN_POINT('Ctrl Pts',(-2.96687537842451,-1.,-2.72722614084076));
#37573=CARTESIAN_POINT('Ctrl Pts',(-2.95976146492576,-1.,-2.72440846811729));
#37574=CARTESIAN_POINT('Ctrl Pts',(-2.95266939280621,-1.,-2.72155475123364));
#37575=CARTESIAN_POINT('Ctrl Pts',(-2.94560002559806,-1.,-2.71866514227965));
#37576=CARTESIAN_POINT('Ctrl Pts',(-2.93855503247266,-1.,-2.7157405459259));
#37577=CARTESIAN_POINT('Ctrl Pts',(-2.93153633192595,-1.,-2.71278207520817));
#37578=CARTESIAN_POINT('Ctrl Pts',(-2.92454558914778,-1.,-2.70979055994754));
#37579=CARTESIAN_POINT('Ctrl Pts',(-2.91758367994737,-1.,-2.70676602302518));
#37580=CARTESIAN_POINT('Ctrl Pts',(-2.91065019668329,-1.,-2.70370719782113));
#37581=CARTESIAN_POINT('Ctrl Pts',(-2.90374285605838,-1.,-2.70061095078692));
#37582=CARTESIAN_POINT('Ctrl Pts',(-2.89685866123671,-1.,-2.69747340630625));
#37583=CARTESIAN_POINT('Ctrl Pts',(-2.88999512410309,-1.,-2.69429113011374));
#37584=CARTESIAN_POINT('Ctrl Pts',(-2.88315153980466,-1.,-2.69106236420198));
#37585=CARTESIAN_POINT('Ctrl Pts',(-2.8763300724388,-1.,-2.68778807801686));
#37586=CARTESIAN_POINT('Ctrl Pts',(-2.86953736547238,-1.,-2.68447353139599));
#37587=CARTESIAN_POINT('Ctrl Pts',(-2.86278224277689,-1.,-2.68112602796308));
#37588=CARTESIAN_POINT('Ctrl Pts',(-2.85607274378018,-1.,-2.67775201955724));
#37589=CARTESIAN_POINT('Ctrl Pts',(-2.84941315703092,-1.,-2.67435421039677));
#37590=CARTESIAN_POINT('Ctrl Pts',(-2.84280157191323,-1.,-2.67092916452125));
#37591=CARTESIAN_POINT('Ctrl Pts',(-2.83622586853982,-1.,-2.66746339678107));
#37592=CARTESIAN_POINT('Ctrl Pts',(-2.82966813308998,-1.,-2.6639376472693));
#37593=CARTESIAN_POINT('Ctrl Pts',(-2.82311188135078,-1.,-2.66033388273461));
#37594=CARTESIAN_POINT('Ctrl Pts',(-2.81654896073883,-1.,-2.65664198781344));
#37595=CARTESIAN_POINT('Ctrl Pts',(-2.80998526078165,-1.,-2.65286529532208));
#37596=CARTESIAN_POINT('Ctrl Pts',(-2.80345029781152,-1.,-2.64902988983337));
#37597=CARTESIAN_POINT('Ctrl Pts',(-2.79698910670736,-1.,-2.64517667799319));
#37598=CARTESIAN_POINT('Ctrl Pts',(-2.79064495573224,-1.,-2.64134450532584));
#37599=CARTESIAN_POINT('Ctrl Pts',(-2.78444351041571,-1.,-2.637554714303));
#37600=CARTESIAN_POINT('Ctrl Pts',(-2.77837943466449,-1.,-2.63379800904599));
#37601=CARTESIAN_POINT('Ctrl Pts',(-2.77239433377921,-1.,-2.63001305229625));
#37602=CARTESIAN_POINT('Ctrl Pts',(-2.76639078479021,-1.,-2.62609956506355));
#37603=CARTESIAN_POINT('Ctrl Pts',(-2.76027271596686,-1.,-2.62195665834605));
#37604=CARTESIAN_POINT('Ctrl Pts',(-2.7539802502603,-1.,-2.61751580407667));
#37605=CARTESIAN_POINT('Ctrl Pts',(-2.74752219567252,-1.,-2.61277170105813));
#37606=CARTESIAN_POINT('Ctrl Pts',(-2.7410211099909,-1.,-2.60782480638448));
#37607=CARTESIAN_POINT('Ctrl Pts',(-2.73470730109615,-1.,-2.60287635688728));
#37608=CARTESIAN_POINT('Ctrl Pts',(-2.7288648348152,-1.,-2.59817869034746));
#37609=CARTESIAN_POINT('Ctrl Pts',(-2.72378896977134,-1.,-2.59399625537278));
#37610=CARTESIAN_POINT('Ctrl Pts',(-2.71974308958086,-1.,-2.59056604771971));
#37611=CARTESIAN_POINT('Ctrl Pts',(-2.71711860281815,-1.,-2.58823792682672));
#37612=CARTESIAN_POINT('Ctrl Pts',(-2.71591054189786,-1.,-2.58706285424358));
#37613=CARTESIAN_POINT('Ctrl Pts',(-2.71548946460575,-1.,-2.58656037976753));
#37614=CARTESIAN_POINT('Ctrl Pts',(-2.71540296616024,-1.,-2.58638312917167));
#37615=CARTESIAN_POINT('Ctrl Pts',(-2.71539546306948,-1.,-2.58633475774921));
#37616=CARTESIAN_POINT('',(-2.58633475775051,-1.,-2.71539546306824));
#37617=CARTESIAN_POINT('Origin',(0.,-1.,0.));
#37618=CARTESIAN_POINT('',(-2.78507268004356,-1.,-3.14378277984898));
#37619=CARTESIAN_POINT('Ctrl Pts',(-2.58633475775051,-1.,-2.71539546306824));
#37620=CARTESIAN_POINT('Ctrl Pts',(-2.58638312917291,-1.,-2.71540296615967));
#37621=CARTESIAN_POINT('Ctrl Pts',(-2.58656037976884,-1.,-2.71548946460616));
#37622=CARTESIAN_POINT('Ctrl Pts',(-2.58706285424469,-1.,-2.71591054189884));
#37623=CARTESIAN_POINT('Ctrl Pts',(-2.58823792682724,-1.,-2.7171186028189));
#37624=CARTESIAN_POINT('Ctrl Pts',(-2.59056604771863,-1.,-2.7197430895797));
#37625=CARTESIAN_POINT('Ctrl Pts',(-2.59399625537407,-1.,-2.72378896977273));
#37626=CARTESIAN_POINT('Ctrl Pts',(-2.5981786903501,-1.,-2.72886483481804));
#37627=CARTESIAN_POINT('Ctrl Pts',(-2.60287635689,-1.,-2.73470730109906));
#37628=CARTESIAN_POINT('Ctrl Pts',(-2.60782480638629,-1.,-2.74102110999284));
#37629=CARTESIAN_POINT('Ctrl Pts',(-2.61277170105864,-1.,-2.74752219567307));
#37630=CARTESIAN_POINT('Ctrl Pts',(-2.61751580407608,-1.,-2.75398025025967));
#37631=CARTESIAN_POINT('Ctrl Pts',(-2.62195665834491,-1.,-2.76027271596564));
#37632=CARTESIAN_POINT('Ctrl Pts',(-2.6260995650624,-1.,-2.76639078478898));
#37633=CARTESIAN_POINT('Ctrl Pts',(-2.63001305229548,-1.,-2.77239433377839));
#37634=CARTESIAN_POINT('Ctrl Pts',(-2.63379800904575,-1.,-2.77837943466423));
#37635=CARTESIAN_POINT('Ctrl Pts',(-2.63755471430322,-1.,-2.78444351041594));
#37636=CARTESIAN_POINT('Ctrl Pts',(-2.64134450532632,-1.,-2.79064495573275));
#37637=CARTESIAN_POINT('Ctrl Pts',(-2.6451766779937,-1.,-2.7969891067079));
#37638=CARTESIAN_POINT('Ctrl Pts',(-2.64902988983373,-1.,-2.80345029781191));
#37639=CARTESIAN_POINT('Ctrl Pts',(-2.65286529532221,-1.,-2.80998526078179));
#37640=CARTESIAN_POINT('Ctrl Pts',(-2.65664198781335,-1.,-2.81654896073874));
#37641=CARTESIAN_POINT('Ctrl Pts',(-2.66033388273437,-1.,-2.82311188135053));
#37642=CARTESIAN_POINT('Ctrl Pts',(-2.66393764726902,-1.,-2.82966813308969));
#37643=CARTESIAN_POINT('Ctrl Pts',(-2.66746339678085,-1.,-2.8362258685396));
#37644=CARTESIAN_POINT('Ctrl Pts',(-2.67092916452117,-1.,-2.84280157191314));
#37645=CARTESIAN_POINT('Ctrl Pts',(-2.67435421039682,-1.,-2.84941315703096));
#37646=CARTESIAN_POINT('Ctrl Pts',(-2.67775201955736,-1.,-2.85607274378031));
#37647=CARTESIAN_POINT('Ctrl Pts',(-2.68112602796323,-1.,-2.86278224277705));
#37648=CARTESIAN_POINT('Ctrl Pts',(-2.68447353139611,-1.,-2.8695373654725));
#37649=CARTESIAN_POINT('Ctrl Pts',(-2.68778807801691,-1.,-2.87633007243885));
#37650=CARTESIAN_POINT('Ctrl Pts',(-2.69106236420197,-1.,-2.88315153980464));
#37651=CARTESIAN_POINT('Ctrl Pts',(-2.69429113011369,-1.,-2.88999512410304));
#37652=CARTESIAN_POINT('Ctrl Pts',(-2.69747340630621,-1.,-2.89685866123668));
#37653=CARTESIAN_POINT('Ctrl Pts',(-2.70061095078692,-1.,-2.90374285605839));
#37654=CARTESIAN_POINT('Ctrl Pts',(-2.70370719782114,-1.,-2.91065019668331));
#37655=CARTESIAN_POINT('Ctrl Pts',(-2.70676602302518,-1.,-2.91758367994738));
#37656=CARTESIAN_POINT('Ctrl Pts',(-2.70979055994751,-1.,-2.92454558914774));
#37657=CARTESIAN_POINT('Ctrl Pts',(-2.71278207520807,-1.,-2.93153633192583));
#37658=CARTESIAN_POINT('Ctrl Pts',(-2.71574054592575,-1.,-2.93855503247248));
#37659=CARTESIAN_POINT('Ctrl Pts',(-2.71866514227952,-1.,-2.94560002559789));
#37660=CARTESIAN_POINT('Ctrl Pts',(-2.72155475123361,-1.,-2.95266939280617));
#37661=CARTESIAN_POINT('Ctrl Pts',(-2.72440846811745,-1.,-2.95976146492595));
#37662=CARTESIAN_POINT('Ctrl Pts',(-2.72722614084112,-1.,-2.96687537842492));
#37663=CARTESIAN_POINT('Ctrl Pts',(-2.7300081921846,-1.,-2.97401089032729));
#37664=CARTESIAN_POINT('Ctrl Pts',(-2.73275539286537,-1.,-2.98116814232175));
#37665=CARTESIAN_POINT('Ctrl Pts',(-2.73546864694548,-1.,-2.98834743696455));
#37666=CARTESIAN_POINT('Ctrl Pts',(-2.73814878711609,-1.,-2.99554902409741));
#37667=CARTESIAN_POINT('Ctrl Pts',(-2.74079632883852,-1.,-3.00277284351431));
#37668=CARTESIAN_POINT('Ctrl Pts',(-2.7434115023978,-1.,-3.01001855960041));
#37669=CARTESIAN_POINT('Ctrl Pts',(-2.74599436193528,-1.,-3.01728567646502));
#37670=CARTESIAN_POINT('Ctrl Pts',(-2.74854487184099,-1.,-3.02457362909199));
#37671=CARTESIAN_POINT('Ctrl Pts',(-2.75106299523032,-1.,-3.03188187589168));
#37672=CARTESIAN_POINT('Ctrl Pts',(-2.75354880060473,-1.,-3.03921001108158));
#37673=CARTESIAN_POINT('Ctrl Pts',(-2.7560024745616,-1.,-3.04655777351333));
#37674=CARTESIAN_POINT('Ctrl Pts',(-2.75842427253164,-1.,-3.05392498750112));
#37675=CARTESIAN_POINT('Ctrl Pts',(-2.76081448760011,-1.,-3.06131152247599));
#37676=CARTESIAN_POINT('Ctrl Pts',(-2.76317341453415,-1.,-3.06871724843121));
#37677=CARTESIAN_POINT('Ctrl Pts',(-2.76550131064522,-1.,-3.07614198408488));
#37678=CARTESIAN_POINT('Ctrl Pts',(-2.76779837828843,-1.,-3.08358548000904));
#37679=CARTESIAN_POINT('Ctrl Pts',(-2.77006478033937,-1.,-3.09104745381882));
#37680=CARTESIAN_POINT('Ctrl Pts',(-2.77230064795679,-1.,-3.09852761277432));
#37681=CARTESIAN_POINT('Ctrl Pts',(-2.7745060912343,-1.,-3.10602568032641));
#37682=CARTESIAN_POINT('Ctrl Pts',(-2.77668121003225,-1.,-3.11354142304692));
#37683=CARTESIAN_POINT('Ctrl Pts',(-2.77882610147986,-1.,-3.12107467038623));
#37684=CARTESIAN_POINT('Ctrl Pts',(-2.78094085162947,-1.,-3.12862530320194));
#37685=CARTESIAN_POINT('Ctrl Pts',(-2.78260859420629,-1.,-3.1346796583452));
#37686=CARTESIAN_POINT('Ctrl Pts',(-2.78384588958965,-1.,-3.13922819750185));
#37687=CARTESIAN_POINT('Ctrl Pts',(-2.78466475036183,-1.,-3.14226401019149));
#37688=CARTESIAN_POINT('Ctrl Pts',(-2.78507268004356,-1.,-3.14378277984898));
#37689=CARTESIAN_POINT('',(-2.66939624221984,-1.,-3.24257979115744));
#37690=CARTESIAN_POINT('',(-2.78507268004356,-1.,-3.14378277984898));
#37691=CARTESIAN_POINT('',(-2.27737254473521,-1.,-2.97927412174279));
#37692=CARTESIAN_POINT('Ctrl Pts',(-2.66939624221984,-1.,-3.24257979115744));
#37693=CARTESIAN_POINT('Ctrl Pts',(-2.66795998539579,-1.,-3.24193929584471));
#37694=CARTESIAN_POINT('Ctrl Pts',(-2.66508964663997,-1.,-3.24065561086749));
#37695=CARTESIAN_POINT('Ctrl Pts',(-2.6607906631847,-1.,-3.23872200034785));
#37696=CARTESIAN_POINT('Ctrl Pts',(-2.65507173961555,-1.,-3.236127680639));
#37697=CARTESIAN_POINT('Ctrl Pts',(-2.64794488743038,-1.,-3.23285778737096));
#37698=CARTESIAN_POINT('Ctrl Pts',(-2.64083992181823,-1.,-3.22956084358547));
#37699=CARTESIAN_POINT('Ctrl Pts',(-2.63375697391372,-1.,-3.2262367829246));
#37700=CARTESIAN_POINT('Ctrl Pts',(-2.62669622735912,-1.,-3.2228855361324));
#37701=CARTESIAN_POINT('Ctrl Pts',(-2.61965792832947,-1.,-3.21950704109321));
#37702=CARTESIAN_POINT('Ctrl Pts',(-2.61264236719171,-1.,-3.21610123233082));
#37703=CARTESIAN_POINT('Ctrl Pts',(-2.60564985360017,-1.,-3.21266802609682));
#37704=CARTESIAN_POINT('Ctrl Pts',(-2.59868069194342,-1.,-3.20920730569681));
#37705=CARTESIAN_POINT('Ctrl Pts',(-2.59173516023481,-1.,-3.2057189102873));
#37706=CARTESIAN_POINT('Ctrl Pts',(-2.58481347777729,-1.,-3.20220261408414));
#37707=CARTESIAN_POINT('Ctrl Pts',(-2.57791581908875,-1.,-3.19865814628682));
#37708=CARTESIAN_POINT('Ctrl Pts',(-2.57104235897899,-1.,-3.19508523784363));
#37709=CARTESIAN_POINT('Ctrl Pts',(-2.56419331092858,-1.,-3.19148366395139));
#37710=CARTESIAN_POINT('Ctrl Pts',(-2.55736896206056,-1.,-3.18785328116218));
#37711=CARTESIAN_POINT('Ctrl Pts',(-2.55056972387731,-1.,-3.18419408529594));
#37712=CARTESIAN_POINT('Ctrl Pts',(-2.54379612553051,-1.,-3.1805061975064));
#37713=CARTESIAN_POINT('Ctrl Pts',(-2.53704871950948,-1.,-3.17678974135318));
#37714=CARTESIAN_POINT('Ctrl Pts',(-2.53032800406941,-1.,-3.17304474093612));
#37715=CARTESIAN_POINT('Ctrl Pts',(-2.52363434671788,-1.,-3.16927102130736));
#37716=CARTESIAN_POINT('Ctrl Pts',(-2.51696788755577,-1.,-3.16546808277023));
#37717=CARTESIAN_POINT('Ctrl Pts',(-2.51032851007894,-1.,-3.16163506380157));
#37718=CARTESIAN_POINT('Ctrl Pts',(-2.50371605688252,-1.,-3.15777102413957));
#37719=CARTESIAN_POINT('Ctrl Pts',(-2.49713050858896,-1.,-3.15387518039046));
#37720=CARTESIAN_POINT('Ctrl Pts',(-2.49057217131988,-1.,-3.14994715298907));
#37721=CARTESIAN_POINT('Ctrl Pts',(-2.4840418741839,-1.,-3.14598722723896));
#37722=CARTESIAN_POINT('Ctrl Pts',(-2.47754112428043,-1.,-3.14199655778863));
#37723=CARTESIAN_POINT('Ctrl Pts',(-2.47107164236838,-1.,-3.13797654408943));
#37724=CARTESIAN_POINT('Ctrl Pts',(-2.46463494332374,-1.,-3.13392826623906));
#37725=CARTESIAN_POINT('Ctrl Pts',(-2.45823188859366,-1.,-3.12985188384371));
#37726=CARTESIAN_POINT('Ctrl Pts',(-2.45186227369846,-1.,-3.12574608210847));
#37727=CARTESIAN_POINT('Ctrl Pts',(-2.44552433364715,-1.,-3.12160740887768));
#37728=CARTESIAN_POINT('Ctrl Pts',(-2.43921571477977,-1.,-3.11743156744186));
#37729=CARTESIAN_POINT('Ctrl Pts',(-2.43293449685144,-1.,-3.11321477659018));
#37730=CARTESIAN_POINT('Ctrl Pts',(-2.42668025870015,-1.,-3.10895518969595));
#37731=CARTESIAN_POINT('Ctrl Pts',(-2.42045498612489,-1.,-3.10465410280896));
#37732=CARTESIAN_POINT('Ctrl Pts',(-2.41426441798057,-1.,-3.1003177502767));
#37733=CARTESIAN_POINT('Ctrl Pts',(-2.40811612696369,-1.,-3.09595472616076));
#37734=CARTESIAN_POINT('Ctrl Pts',(-2.40201704423341,-1.,-3.091572660511));
#37735=CARTESIAN_POINT('Ctrl Pts',(-2.39597098250631,-1.,-3.08717489512914));
#37736=CARTESIAN_POINT('Ctrl Pts',(-2.38997659219199,-1.,-3.08275773747093));
#37737=CARTESIAN_POINT('Ctrl Pts',(-2.38402401216126,-1.,-3.07830597244326));
#37738=CARTESIAN_POINT('Ctrl Pts',(-2.37809856205548,-1.,-3.07379777492165));
#37739=CARTESIAN_POINT('Ctrl Pts',(-2.37218678163178,-1.,-3.069212754975));
#37740=CARTESIAN_POINT('Ctrl Pts',(-2.36628220107009,-1.,-3.06453964643162));
#37741=CARTESIAN_POINT('Ctrl Pts',(-2.36039011602072,-1.,-3.0597826624004));
#37742=CARTESIAN_POINT('Ctrl Pts',(-2.35453559889474,-1.,-3.05497218368146));
#37743=CARTESIAN_POINT('Ctrl Pts',(-2.34875673090771,-1.,-3.05015565829918));
#37744=CARTESIAN_POINT('Ctrl Pts',(-2.34309017083977,-1.,-3.04537822217256));
#37745=CARTESIAN_POINT('Ctrl Pts',(-2.33755792953706,-1.,-3.04066496998544));
#37746=CARTESIAN_POINT('Ctrl Pts',(-2.33215619079829,-1.,-3.03600588555793));
#37747=CARTESIAN_POINT('Ctrl Pts',(-2.32683687412097,-1.,-3.03133125185136));
#37748=CARTESIAN_POINT('Ctrl Pts',(-2.32151944306402,-1.,-3.02652678416611));
#37749=CARTESIAN_POINT('Ctrl Pts',(-2.31612479121631,-1.,-3.02147780668161));
#37750=CARTESIAN_POINT('Ctrl Pts',(-2.31060449886629,-1.,-3.01610726819086));
#37751=CARTESIAN_POINT('Ctrl Pts',(-2.30496809486482,-1.,-3.01041131063823));
#37752=CARTESIAN_POINT('Ctrl Pts',(-2.29932091315775,-1.,-3.00450832658613));
#37753=CARTESIAN_POINT('Ctrl Pts',(-2.29385894577754,-1.,-2.99863310339691));
#37754=CARTESIAN_POINT('Ctrl Pts',(-2.28882328690362,-1.,-2.99307930984034));
#37755=CARTESIAN_POINT('Ctrl Pts',(-2.28446419115919,-1.,-2.9881543273478));
#37756=CARTESIAN_POINT('Ctrl Pts',(-2.28100472516679,-1.,-2.98413343613983));
#37757=CARTESIAN_POINT('Ctrl Pts',(-2.27877674853766,-1.,-2.9814234180956));
#37758=CARTESIAN_POINT('Ctrl Pts',(-2.27776738270289,-1.,-2.98007383024207));
#37759=CARTESIAN_POINT('Ctrl Pts',(-2.27743009389684,-1.,-2.9795116710597));
#37760=CARTESIAN_POINT('Ctrl Pts',(-2.27737238849287,-1.,-2.97932307137477));
#37761=CARTESIAN_POINT('Ctrl Pts',(-2.27737254473521,-1.,-2.97927412174279));
#37762=CARTESIAN_POINT('',(-2.12971124846838,-1.,-3.08655633322109));
#37763=CARTESIAN_POINT('Origin',(0.,-1.,0.));
#37764=CARTESIAN_POINT('',(-2.25898783642071,-1.,-3.54075895182139));
#37765=CARTESIAN_POINT('Ctrl Pts',(-2.12971124846838,-1.,-3.08655633322109));
#37766=CARTESIAN_POINT('Ctrl Pts',(-2.1297578506162,-1.,-3.0865713108946));
#37767=CARTESIAN_POINT('Ctrl Pts',(-2.12991938762497,-1.,-3.08668447250383));
#37768=CARTESIAN_POINT('Ctrl Pts',(-2.13034980480519,-1.,-3.08717896996213));
#37769=CARTESIAN_POINT('Ctrl Pts',(-2.13132142793056,-1.,-3.08855597949844));
#37770=CARTESIAN_POINT('Ctrl Pts',(-2.13321032560805,-1.,-3.09151235281832));
#37771=CARTESIAN_POINT('Ctrl Pts',(-2.13596538661154,-1.,-3.09604502421197));
#37772=CARTESIAN_POINT('Ctrl Pts',(-2.13930228863968,-1.,-3.1017126739137));
#37773=CARTESIAN_POINT('Ctrl Pts',(-2.14302815602195,-1.,-3.10821808669189));
#37774=CARTESIAN_POINT('Ctrl Pts',(-2.1469279845768,-1.,-3.11522827017075));
#37775=CARTESIAN_POINT('Ctrl Pts',(-2.15079698090627,-1.,-3.12242318152001));
#37776=CARTESIAN_POINT('Ctrl Pts',(-2.15447241382872,-1.,-3.12954386795575));
#37777=CARTESIAN_POINT('Ctrl Pts',(-2.15787423530583,-1.,-3.136453565629));
#37778=CARTESIAN_POINT('Ctrl Pts',(-2.16100905914341,-1.,-3.14314440426882));
#37779=CARTESIAN_POINT('Ctrl Pts',(-2.16393520288009,-1.,-3.14968624388961));
#37780=CARTESIAN_POINT('Ctrl Pts',(-2.1667372844767,-1.,-3.15618975593627));
#37781=CARTESIAN_POINT('Ctrl Pts',(-2.16949910801237,-1.,-3.16276685102999));
#37782=CARTESIAN_POINT('Ctrl Pts',(-2.17227212063857,-1.,-3.16948480019555));
#37783=CARTESIAN_POINT('Ctrl Pts',(-2.17506466903736,-1.,-3.17635032802584));
#37784=CARTESIAN_POINT('Ctrl Pts',(-2.17785968847172,-1.,-3.18333474627851));
#37785=CARTESIAN_POINT('Ctrl Pts',(-2.18062558031789,-1.,-3.19038924261589));
#37786=CARTESIAN_POINT('Ctrl Pts',(-2.18332898656595,-1.,-3.197462937404));
#37787=CARTESIAN_POINT('Ctrl Pts',(-2.18594876115914,-1.,-3.20452259717947));
#37788=CARTESIAN_POINT('Ctrl Pts',(-2.18848253363878,-1.,-3.21156188355736));
#37789=CARTESIAN_POINT('Ctrl Pts',(-2.1909390194865,-1.,-3.21859043114069));
#37790=CARTESIAN_POINT('Ctrl Pts',(-2.19333345123531,-1.,-3.22562734221636));
#37791=CARTESIAN_POINT('Ctrl Pts',(-2.19568204933172,-1.,-3.23269332296938));
#37792=CARTESIAN_POINT('Ctrl Pts',(-2.19799623693263,-1.,-3.23980245361323));
#37793=CARTESIAN_POINT('Ctrl Pts',(-2.20027910880993,-1.,-3.24695715874356));
#37794=CARTESIAN_POINT('Ctrl Pts',(-2.20252866491554,-1.,-3.25415277957789));
#37795=CARTESIAN_POINT('Ctrl Pts',(-2.20473979048682,-1.,-3.26138036637711));
#37796=CARTESIAN_POINT('Ctrl Pts',(-2.20690665217741,-1.,-3.2686300613678));
#37797=CARTESIAN_POINT('Ctrl Pts',(-2.20902509417425,-1.,-3.27589448005534));
#37798=CARTESIAN_POINT('Ctrl Pts',(-2.21109449750638,-1.,-3.28317133333127));
#37799=CARTESIAN_POINT('Ctrl Pts',(-2.21311648827391,-1.,-3.29046159238344));
#37800=CARTESIAN_POINT('Ctrl Pts',(-2.2150940692337,-1.,-3.29776825193162));
#37801=CARTESIAN_POINT('Ctrl Pts',(-2.21703059947837,-1.,-3.3050948781957));
#37802=CARTESIAN_POINT('Ctrl Pts',(-2.21892881679083,-1.,-3.31244421655662));
#37803=CARTESIAN_POINT('Ctrl Pts',(-2.22078990842768,-1.,-3.31981686778008));
#37804=CARTESIAN_POINT('Ctrl Pts',(-2.22261398879623,-1.,-3.32721196326019));
#37805=CARTESIAN_POINT('Ctrl Pts',(-2.224400498785,-1.,-3.3346277284958));
#37806=CARTESIAN_POINT('Ctrl Pts',(-2.22614863918044,-1.,-3.34206209449371));
#37807=CARTESIAN_POINT('Ctrl Pts',(-2.22785777756588,-1.,-3.34951327111117));
#37808=CARTESIAN_POINT('Ctrl Pts',(-2.22952789881011,-1.,-3.35698038165529));
#37809=CARTESIAN_POINT('Ctrl Pts',(-2.23115945849777,-1.,-3.36446325227908));
#37810=CARTESIAN_POINT('Ctrl Pts',(-2.23275319569253,-1.,-3.37196214349356));
#37811=CARTESIAN_POINT('Ctrl Pts',(-2.23430995599572,-1.,-3.37947749555649));
#37812=CARTESIAN_POINT('Ctrl Pts',(-2.23583052276281,-1.,-3.38700968549522));
#37813=CARTESIAN_POINT('Ctrl Pts',(-2.23731541452727,-1.,-3.39455873448088));
#37814=CARTESIAN_POINT('Ctrl Pts',(-2.23876491124064,-1.,-3.40212434705511));
#37815=CARTESIAN_POINT('Ctrl Pts',(-2.24017914395211,-1.,-3.40970604190205));
#37816=CARTESIAN_POINT('Ctrl Pts',(-2.24155816587811,-1.,-3.41730325539119));
#37817=CARTESIAN_POINT('Ctrl Pts',(-2.24290202531144,-1.,-3.42491544683075));
#37818=CARTESIAN_POINT('Ctrl Pts',(-2.24421085338856,-1.,-3.43254222615007));
#37819=CARTESIAN_POINT('Ctrl Pts',(-2.24548487526212,-1.,-3.44018336460619));
#37820=CARTESIAN_POINT('Ctrl Pts',(-2.24672437070139,-1.,-3.44783872863448));
#37821=CARTESIAN_POINT('Ctrl Pts',(-2.24792964960874,-1.,-3.45550823512213));
#37822=CARTESIAN_POINT('Ctrl Pts',(-2.24910102345977,-1.,-3.46319180177474));
#37823=CARTESIAN_POINT('Ctrl Pts',(-2.25023877475674,-1.,-3.47088928979467));
#37824=CARTESIAN_POINT('Ctrl Pts',(-2.25134314238258,-1.,-3.47860048448015));
#37825=CARTESIAN_POINT('Ctrl Pts',(-2.25241433138231,-1.,-3.48632513240231));
#37826=CARTESIAN_POINT('Ctrl Pts',(-2.25345251709453,-1.,-3.49406296494309));
#37827=CARTESIAN_POINT('Ctrl Pts',(-2.25445785151923,-1.,-3.50181372618058));
#37828=CARTESIAN_POINT('Ctrl Pts',(-2.25543046980351,-1.,-3.50957720118209));
#37829=CARTESIAN_POINT('Ctrl Pts',(-2.25637049456061,-1.,-3.51735323669213));
#37830=CARTESIAN_POINT('Ctrl Pts',(-2.25727802942141,-1.,-3.52514172849666));
#37831=CARTESIAN_POINT('Ctrl Pts',(-2.25797812951166,-1.,-3.53138243689932));
#37832=CARTESIAN_POINT('Ctrl Pts',(-2.25848864344599,-1.,-3.53606853163247));
#37833=CARTESIAN_POINT('Ctrl Pts',(-2.25882251694918,-1.,-3.5391950664771));
#37834=CARTESIAN_POINT('Ctrl Pts',(-2.25898783642071,-1.,-3.54075895182139));
#37835=CARTESIAN_POINT('',(-2.12928030988903,-1.,-3.62024382630768));
#37836=CARTESIAN_POINT('',(-2.25898783642071,-1.,-3.54075895182139));
#37837=CARTESIAN_POINT('',(-1.78327315618341,-1.,-3.29885386921513));
#37838=CARTESIAN_POINT('Ctrl Pts',(-2.12928030988903,-1.,-3.62024382630768));
#37839=CARTESIAN_POINT('Ctrl Pts',(-2.12796193131142,-1.,-3.61938653648716));
#37840=CARTESIAN_POINT('Ctrl Pts',(-2.12532774376144,-1.,-3.61766963589442));
#37841=CARTESIAN_POINT('Ctrl Pts',(-2.12138417125349,-1.,-3.61508732215187));
#37842=CARTESIAN_POINT('Ctrl Pts',(-2.11614149813928,-1.,-3.61163030607452));
#37843=CARTESIAN_POINT('Ctrl Pts',(-2.10961391333497,-1.,-3.60728578530968));
#37844=CARTESIAN_POINT('Ctrl Pts',(-2.10311217727687,-1.,-3.60291797087849));
#37845=CARTESIAN_POINT('Ctrl Pts',(-2.09663642986579,-1.,-3.59852681775396));
#37846=CARTESIAN_POINT('Ctrl Pts',(-2.09018686331706,-1.,-3.5941122862608));
#37847=CARTESIAN_POINT('Ctrl Pts',(-2.08376373049196,-1.,-3.58967435355834));
#37848=CARTESIAN_POINT('Ctrl Pts',(-2.07736732842524,-1.,-3.58521300039988));
#37849=CARTESIAN_POINT('Ctrl Pts',(-2.07099797606,-1.,-3.58072819250872));
#37850=CARTESIAN_POINT('Ctrl Pts',(-2.06465599229234,-1.,-3.57621986224402));
#37851=CARTESIAN_POINT('Ctrl Pts',(-2.05834167687425,-1.,-3.5716878942334));
#37852=CARTESIAN_POINT('Ctrl Pts',(-2.05205528172911,-1.,-3.56713209977904));
#37853=CARTESIAN_POINT('Ctrl Pts',(-2.04579702158876,-1.,-3.56255223871505));
#37854=CARTESIAN_POINT('Ctrl Pts',(-2.03956711119976,-1.,-3.55794807264844));
#37855=CARTESIAN_POINT('Ctrl Pts',(-2.03336579658133,-1.,-3.55331941293949));
#37856=CARTESIAN_POINT('Ctrl Pts',(-2.02719338376175,-1.,-3.54866616282227));
#37857=CARTESIAN_POINT('Ctrl Pts',(-2.02105027983104,-1.,-3.54398838254136));
#37858=CARTESIAN_POINT('Ctrl Pts',(-2.01493698847351,-1.,-3.53928627453642));
#37859=CARTESIAN_POINT('Ctrl Pts',(-2.00885403604746,-1.,-3.53456004727424));
#37860=CARTESIAN_POINT('Ctrl Pts',(-2.00280191090366,-1.,-3.52980980250224));
#37861=CARTESIAN_POINT('Ctrl Pts',(-1.99678100339296,-1.,-3.52503542491728));
#37862=CARTESIAN_POINT('Ctrl Pts',(-1.99079153006112,-1.,-3.52023644289142));
#37863=CARTESIAN_POINT('Ctrl Pts',(-1.9848335106103,-1.,-3.51541198728301));
#37864=CARTESIAN_POINT('Ctrl Pts',(-1.97890693666288,-1.,-3.51056110478287));
#37865=CARTESIAN_POINT('Ctrl Pts',(-1.97301191162968,-1.,-3.5056830186108));
#37866=CARTESIAN_POINT('Ctrl Pts',(-1.96714879724052,-1.,-3.50077740176267));
#37867=CARTESIAN_POINT('Ctrl Pts',(-1.961318367765,-1.,-3.49584466573064));
#37868=CARTESIAN_POINT('Ctrl Pts',(-1.95552193112084,-1.,-3.49088618670987));
#37869=CARTESIAN_POINT('Ctrl Pts',(-1.94976096795911,-1.,-3.48590361610814));
#37870=CARTESIAN_POINT('Ctrl Pts',(-1.94403680554065,-1.,-3.48089825770416));
#37871=CARTESIAN_POINT('Ctrl Pts',(-1.93835026973887,-1.,-3.47587040389915));
#37872=CARTESIAN_POINT('Ctrl Pts',(-1.93270136427081,-1.,-3.47081872409781));
#37873=CARTESIAN_POINT('Ctrl Pts',(-1.92708888591158,-1.,-3.46573953254084));
#37874=CARTESIAN_POINT('Ctrl Pts',(-1.92151118213212,-1.,-3.46062821722485));
#37875=CARTESIAN_POINT('Ctrl Pts',(-1.91596694784064,-1.,-3.4554807430995));
#37876=CARTESIAN_POINT('Ctrl Pts',(-1.91045605593639,-1.,-3.45029522038888));
#37877=CARTESIAN_POINT('Ctrl Pts',(-1.90498026502305,-1.,-3.44507323983367));
#37878=CARTESIAN_POINT('Ctrl Pts',(-1.89954426803384,-1.,-3.4398218567809));
#37879=CARTESIAN_POINT('Ctrl Pts',(-1.89415420002542,-1.,-3.43455074411571));
#37880=CARTESIAN_POINT('Ctrl Pts',(-1.88881571322009,-1.,-3.42926852222158));
#37881=CARTESIAN_POINT('Ctrl Pts',(-1.8835320506206,-1.,-3.42397908819736));
#37882=CARTESIAN_POINT('Ctrl Pts',(-1.87830245689344,-1.,-3.41867858383771));
#37883=CARTESIAN_POINT('Ctrl Pts',(-1.87311957248121,-1.,-3.41335043875209));
#37884=CARTESIAN_POINT('Ctrl Pts',(-1.86797231196654,-1.,-3.40797080000549));
#37885=CARTESIAN_POINT('Ctrl Pts',(-1.86285057051245,-1.,-3.40251742305476));
#37886=CARTESIAN_POINT('Ctrl Pts',(-1.85774972037062,-1.,-3.39697816833067));
#37887=CARTESIAN_POINT('Ctrl Pts',(-1.85267433291769,-1.,-3.39135802549398));
#37888=CARTESIAN_POINT('Ctrl Pts',(-1.84764441927753,-1.,-3.38569092349592));
#37889=CARTESIAN_POINT('Ctrl Pts',(-1.84269016931643,-1.,-3.38002968341157));
#37890=CARTESIAN_POINT('Ctrl Pts',(-1.83784072967077,-1.,-3.37442462015853));
#37891=CARTESIAN_POINT('Ctrl Pts',(-1.83311391452322,-1.,-3.36890396271836));
#37892=CARTESIAN_POINT('Ctrl Pts',(-1.82850752153199,-1.,-3.36345722124158));
#37893=CARTESIAN_POINT('Ctrl Pts',(-1.82398496829301,-1.,-3.35800801557424));
#37894=CARTESIAN_POINT('Ctrl Pts',(-1.81948458796829,-1.,-3.35243086937598));
#37895=CARTESIAN_POINT('Ctrl Pts',(-1.81494618732853,-1.,-3.34660014370673));
#37896=CARTESIAN_POINT('Ctrl Pts',(-1.81033399625352,-1.,-3.34043216147606));
#37897=CARTESIAN_POINT('Ctrl Pts',(-1.80565802981102,-1.,-3.33392460276808));
#37898=CARTESIAN_POINT('Ctrl Pts',(-1.80100380443406,-1.,-3.32721088039578));
#37899=CARTESIAN_POINT('Ctrl Pts',(-1.79652817033251,-1.,-3.3205535510082));
#37900=CARTESIAN_POINT('Ctrl Pts',(-1.79242331349949,-1.,-3.31428038326424));
#37901=CARTESIAN_POINT('Ctrl Pts',(-1.78888832245873,-1.,-3.30873412266788));
#37902=CARTESIAN_POINT('Ctrl Pts',(-1.78610045419846,-1.,-3.30422155559112));
#37903=CARTESIAN_POINT('Ctrl Pts',(-1.78432384788174,-1.,-3.30119637003393));
#37904=CARTESIAN_POINT('Ctrl Pts',(-1.78353803106924,-1.,-3.299705498242));
#37905=CARTESIAN_POINT('Ctrl Pts',(-1.78329283591905,-1.,-3.29909749657808));
#37906=CARTESIAN_POINT('Ctrl Pts',(-1.78326534445518,-1.,-3.29890219175423));
#37907=CARTESIAN_POINT('Ctrl Pts',(-1.78327315618341,-1.,-3.29885386921513));
#37908=CARTESIAN_POINT('',(-1.62064718014256,-1.,-3.38171594275687));
#37909=CARTESIAN_POINT('Origin',(0.,-1.,0.));
#37910=CARTESIAN_POINT('',(-1.67727921511438,-1.,-3.85054988729471));
#37911=CARTESIAN_POINT('Ctrl Pts',(-1.62064718014256,-1.,-3.38171594275687));
#37912=CARTESIAN_POINT('Ctrl Pts',(-1.62069086551626,-1.,-3.38173802621242));
#37913=CARTESIAN_POINT('Ctrl Pts',(-1.62083271136059,-1.,-3.38187506457001));
#37914=CARTESIAN_POINT('Ctrl Pts',(-1.62118047294574,-1.,-3.38243080602536));
#37915=CARTESIAN_POINT('Ctrl Pts',(-1.62192472202795,-1.,-3.3839428576331));
#37916=CARTESIAN_POINT('Ctrl Pts',(-1.62332788556183,-1.,-3.38715832178929));
#37917=CARTESIAN_POINT('Ctrl Pts',(-1.62533996116793,-1.,-3.39206617497078));
#37918=CARTESIAN_POINT('Ctrl Pts',(-1.62774916464571,-1.,-3.39818605298342));
#37919=CARTESIAN_POINT('Ctrl Pts',(-1.63041148964996,-1.,-3.40519422740596));
#37920=CARTESIAN_POINT('Ctrl Pts',(-1.63316667054156,-1.,-3.41272817148719));
#37921=CARTESIAN_POINT('Ctrl Pts',(-1.63586250099804,-1.,-3.4204397459095));
#37922=CARTESIAN_POINT('Ctrl Pts',(-1.6383787624689,-1.,-3.42804772926213));
#37923=CARTESIAN_POINT('Ctrl Pts',(-1.64065778701952,-1.,-3.43540451921397));
#37924=CARTESIAN_POINT('Ctrl Pts',(-1.64270733821042,-1.,-3.44250337701736));
#37925=CARTESIAN_POINT('Ctrl Pts',(-1.64457408708059,-1.,-3.44942242546693));
#37926=CARTESIAN_POINT('Ctrl Pts',(-1.64632429697506,-1.,-3.4562842106239));
#37927=CARTESIAN_POINT('Ctrl Pts',(-1.64802323352752,-1.,-3.46321237515029));
#37928=CARTESIAN_POINT('Ctrl Pts',(-1.64971118698285,-1.,-3.47028140996055));
#37929=CARTESIAN_POINT('Ctrl Pts',(-1.65139534930353,-1.,-3.47749926256543));
#37930=CARTESIAN_POINT('Ctrl Pts',(-1.65306335367762,-1.,-3.48483492840942));
#37931=CARTESIAN_POINT('Ctrl Pts',(-1.65469162644476,-1.,-3.49223525300194));
#37932=CARTESIAN_POINT('Ctrl Pts',(-1.65625517961583,-1.,-3.49964476477929));
#37933=CARTESIAN_POINT('Ctrl Pts',(-1.65773832633617,-1.,-3.5070273314651));
#37934=CARTESIAN_POINT('Ctrl Pts',(-1.65913971687324,-1.,-3.51437632188903));
#37935=CARTESIAN_POINT('Ctrl Pts',(-1.66046645222266,-1.,-3.52170261543787));
#37936=CARTESIAN_POINT('Ctrl Pts',(-1.66173058912365,-1.,-3.52902746211081));
#37937=CARTESIAN_POINT('Ctrl Pts',(-1.66294490916113,-1.,-3.53637385060225));
#37938=CARTESIAN_POINT('Ctrl Pts',(-1.66411849222334,-1.,-3.5437574747503));
#37939=CARTESIAN_POINT('Ctrl Pts',(-1.66525401569004,-1.,-3.5511812134288));
#37940=CARTESIAN_POINT('Ctrl Pts',(-1.66635023293121,-1.,-3.55864015233617));
#37941=CARTESIAN_POINT('Ctrl Pts',(-1.66740349220308,-1.,-3.56612465179429));
#37942=CARTESIAN_POINT('Ctrl Pts',(-1.66840957407299,-1.,-3.57362406285884));
#37943=CARTESIAN_POINT('Ctrl Pts',(-1.66936552908228,-1.,-3.58113044183823));
#37944=CARTESIAN_POINT('Ctrl Pts',(-1.67027110397601,-1.,-3.5886414309783));
#37945=CARTESIAN_POINT('Ctrl Pts',(-1.67112775290706,-1.,-3.59615824388808));
#37946=CARTESIAN_POINT('Ctrl Pts',(-1.67193797318598,-1.,-3.60368430815203));
#37947=CARTESIAN_POINT('Ctrl Pts',(-1.67270452466968,-1.,-3.61122367156182));
#37948=CARTESIAN_POINT('Ctrl Pts',(-1.67342968196223,-1.,-3.61877947398179));
#37949=CARTESIAN_POINT('Ctrl Pts',(-1.67411452372265,-1.,-3.62635249450908));
#37950=CARTESIAN_POINT('Ctrl Pts',(-1.67475929882962,-1.,-3.63394189312902));
#37951=CARTESIAN_POINT('Ctrl Pts',(-1.67536373264839,-1.,-3.6415458297232));
#37952=CARTESIAN_POINT('Ctrl Pts',(-1.6759273594669,-1.,-3.64916213574663));
#37953=CARTESIAN_POINT('Ctrl Pts',(-1.67644983469459,-1.,-3.65678894416442));
#37954=CARTESIAN_POINT('Ctrl Pts',(-1.67693128053153,-1.,-3.66442538671018));
#37955=CARTESIAN_POINT('Ctrl Pts',(-1.67737217414901,-1.,-3.67207136294639));
#37956=CARTESIAN_POINT('Ctrl Pts',(-1.67777320475872,-1.,-3.6797272457918));
#37957=CARTESIAN_POINT('Ctrl Pts',(-1.67813513867973,-1.,-3.68739360236505));
#37958=CARTESIAN_POINT('Ctrl Pts',(-1.67845869064304,-1.,-3.69507092759545));
#37959=CARTESIAN_POINT('Ctrl Pts',(-1.6787443694862,-1.,-3.70275932350998));
#37960=CARTESIAN_POINT('Ctrl Pts',(-1.67899249793398,-1.,-3.71045854208195));
#37961=CARTESIAN_POINT('Ctrl Pts',(-1.6792032807165,-1.,-3.71816812842188));
#37962=CARTESIAN_POINT('Ctrl Pts',(-1.67937685856627,-1.,-3.72588753416339));
#37963=CARTESIAN_POINT('Ctrl Pts',(-1.67951336376434,-1.,-3.73361623282617));
#37964=CARTESIAN_POINT('Ctrl Pts',(-1.67961298685316,-1.,-3.74135385965622));
#37965=CARTESIAN_POINT('Ctrl Pts',(-1.67967598599665,-1.,-3.74910022394845));
#37966=CARTESIAN_POINT('Ctrl Pts',(-1.67970265841379,-1.,-3.75685523754816));
#37967=CARTESIAN_POINT('Ctrl Pts',(-1.67969332319322,-1.,-3.76461886684523));
#37968=CARTESIAN_POINT('Ctrl Pts',(-1.67964830084946,-1.,-3.77239107928394));
#37969=CARTESIAN_POINT('Ctrl Pts',(-1.67956789211943,-1.,-3.78017178196859));
#37970=CARTESIAN_POINT('Ctrl Pts',(-1.67945236653175,-1.,-3.78796080021026));
#37971=CARTESIAN_POINT('Ctrl Pts',(-1.67930196625203,-1.,-3.7957579157763));
#37972=CARTESIAN_POINT('Ctrl Pts',(-1.67911690648128,-1.,-3.80356289078481));
#37973=CARTESIAN_POINT('Ctrl Pts',(-1.67889737738311,-1.,-3.81137549624273));
#37974=CARTESIAN_POINT('Ctrl Pts',(-1.67864354606363,-1.,-3.81919554100522));
#37975=CARTESIAN_POINT('Ctrl Pts',(-1.67835555760094,-1.,-3.82702289288453));
#37976=CARTESIAN_POINT('Ctrl Pts',(-1.67803353065273,-1.,-3.83485746516115));
#37977=CARTESIAN_POINT('Ctrl Pts',(-1.67774874946867,-1.,-3.8411308598706));
#37978=CARTESIAN_POINT('Ctrl Pts',(-1.67751991140661,-1.,-3.84583912297567));
#37979=CARTESIAN_POINT('Ctrl Pts',(-1.6773605765671,-1.,-3.84897939431104));
#37980=CARTESIAN_POINT('Ctrl Pts',(-1.67727921511438,-1.,-3.85054988729471));
#37981=CARTESIAN_POINT('',(-1.53673442965255,-1.,-3.90876544355381));
#37982=CARTESIAN_POINT('',(-1.67727921511438,-1.,-3.85054988729471));
#37983=CARTESIAN_POINT('',(-1.24526366418208,-1.,-3.5372048861591));
#37984=CARTESIAN_POINT('Ctrl Pts',(-1.53673442965255,-1.,-3.90876544355381));
#37985=CARTESIAN_POINT('Ctrl Pts',(-1.53556639217742,-1.,-3.90771246854607));
#37986=CARTESIAN_POINT('Ctrl Pts',(-1.53323321827311,-1.,-3.90560462812846));
#37987=CARTESIAN_POINT('Ctrl Pts',(-1.5297421605556,-1.,-3.90243719629755));
#37988=CARTESIAN_POINT('Ctrl Pts',(-1.52510482990784,-1.,-3.8982026070607));
#37989=CARTESIAN_POINT('Ctrl Pts',(-1.51933724328609,-1.,-3.89289043531893));
#37990=CARTESIAN_POINT('Ctrl Pts',(-1.51359883110181,-1.,-3.88755930032927));
#37991=CARTESIAN_POINT('Ctrl Pts',(-1.50788973857719,-1.,-3.88220917950443));
#37992=CARTESIAN_POINT('Ctrl Pts',(-1.50221016176766,-1.,-3.87684006372665));
#37993=CARTESIAN_POINT('Ctrl Pts',(-1.4965603539944,-1.,-3.8714519699927));
#37994=CARTESIAN_POINT('Ctrl Pts',(-1.49094061164604,-1.,-3.86604492575933));
#37995=CARTESIAN_POINT('Ctrl Pts',(-1.48535125510102,-1.,-3.86061894706551));
#37996=CARTESIAN_POINT('Ctrl Pts',(-1.47979260991063,-1.,-3.85517401698952));
#37997=CARTESIAN_POINT('Ctrl Pts',(-1.47426499018467,-1.,-3.84971006847096));
#37998=CARTESIAN_POINT('Ctrl Pts',(-1.46876867426375,-1.,-3.84422695454469));
#37999=CARTESIAN_POINT('Ctrl Pts',(-1.46330391180621,-1.,-3.83872447159309));
#38000=CARTESIAN_POINT('Ctrl Pts',(-1.45787095220763,-1.,-3.83320241775199));
#38001=CARTESIAN_POINT('Ctrl Pts',(-1.45247006796807,-1.,-3.82766064519));
#38002=CARTESIAN_POINT('Ctrl Pts',(-1.44710157648562,-1.,-3.82209910620591));
#38003=CARTESIAN_POINT('Ctrl Pts',(-1.44176587041401,-1.,-3.8165179239855));
#38004=CARTESIAN_POINT('Ctrl Pts',(-1.43646341556783,-1.,-3.81091737726965));
#38005=CARTESIAN_POINT('Ctrl Pts',(-1.43119469921364,-1.,-3.80529775429916));
#38006=CARTESIAN_POINT('Ctrl Pts',(-1.42596018777301,-1.,-3.79965923196365));
#38007=CARTESIAN_POINT('Ctrl Pts',(-1.42076028482828,-1.,-3.7940017574439));
#38008=CARTESIAN_POINT('Ctrl Pts',(-1.41559527803808,-1.,-3.78832489879369));
#38009=CARTESIAN_POINT('Ctrl Pts',(-1.41046532282567,-1.,-3.78262780065406));
#38010=CARTESIAN_POINT('Ctrl Pts',(-1.40537056004702,-1.,-3.77690952014209));
#38011=CARTESIAN_POINT('Ctrl Pts',(-1.40031121335495,-1.,-3.77116930621804));
#38012=CARTESIAN_POINT('Ctrl Pts',(-1.39528769118054,-1.,-3.76540689249078));
#38013=CARTESIAN_POINT('Ctrl Pts',(-1.39030069388926,-1.,-3.75962280650875));
#38014=CARTESIAN_POINT('Ctrl Pts',(-1.38535129801185,-1.,-3.75381861212728));
#38015=CARTESIAN_POINT('Ctrl Pts',(-1.38044070763302,-1.,-3.74799617204744));
#38016=CARTESIAN_POINT('Ctrl Pts',(-1.3755700297169,-1.,-3.7421569816256));
#38017=CARTESIAN_POINT('Ctrl Pts',(-1.37074003422739,-1.,-3.73630145885809));
#38018=CARTESIAN_POINT('Ctrl Pts',(-1.36595093298674,-1.,-3.73042829011293));
#38019=CARTESIAN_POINT('Ctrl Pts',(-1.36120211416353,-1.,-3.72453364678279));
#38020=CARTESIAN_POINT('Ctrl Pts',(-1.35649266705038,-1.,-3.71861271513318));
#38021=CARTESIAN_POINT('Ctrl Pts',(-1.35182193384426,-1.,-3.71266130563061));
#38022=CARTESIAN_POINT('Ctrl Pts',(-1.34719008463535,-1.,-3.7066775318825));
#38023=CARTESIAN_POINT('Ctrl Pts',(-1.3425986075293,-1.,-3.70066324015112));
#38024=CARTESIAN_POINT('Ctrl Pts',(-1.33805103398214,-1.,-3.69462613305692));
#38025=CARTESIAN_POINT('Ctrl Pts',(-1.33355191034515,-1.,-3.68857672413013));
#38026=CARTESIAN_POINT('Ctrl Pts',(-1.32910547072734,-1.,-3.68252441182534));
#38027=CARTESIAN_POINT('Ctrl Pts',(-1.32471430856413,-1.,-3.67647355257906));
#38028=CARTESIAN_POINT('Ctrl Pts',(-1.3203782813777,-1.,-3.67042021752668));
#38029=CARTESIAN_POINT('Ctrl Pts',(-1.31609271239922,-1.,-3.66434688899822));
#38030=CARTESIAN_POINT('Ctrl Pts',(-1.31185038411231,-1.,-3.65822827358655));
#38031=CARTESIAN_POINT('Ctrl Pts',(-1.30764479590051,-1.,-3.65204081987101));
#38032=CARTESIAN_POINT('Ctrl Pts',(-1.30347327603778,-1.,-3.64577181380125));
#38033=CARTESIAN_POINT('Ctrl Pts',(-1.29933955906463,-1.,-3.6394268987279));
#38034=CARTESIAN_POINT('Ctrl Pts',(-1.29525810207744,-1.,-3.63304271630995));
#38035=CARTESIAN_POINT('Ctrl Pts',(-1.29125046021853,-1.,-3.62667616004299));
#38036=CARTESIAN_POINT('Ctrl Pts',(-1.2873375502936,-1.,-3.62038148492295));
#38037=CARTESIAN_POINT('Ctrl Pts',(-1.28353255117754,-1.,-3.61418935913793));
#38038=CARTESIAN_POINT('Ctrl Pts',(-1.27983492861703,-1.,-3.60808907746372));
#38039=CARTESIAN_POINT('Ctrl Pts',(-1.27622049908664,-1.,-3.60199947736404));
#38040=CARTESIAN_POINT('Ctrl Pts',(-1.27264798379365,-1.,-3.59578698050164));
#38041=CARTESIAN_POINT('Ctrl Pts',(-1.26907758484766,-1.,-3.5893180784647));
#38042=CARTESIAN_POINT('Ctrl Pts',(-1.26548706249891,-1.,-3.58250452868699));
#38043=CARTESIAN_POINT('Ctrl Pts',(-1.26188667142784,-1.,-3.5753456065164));
#38044=CARTESIAN_POINT('Ctrl Pts',(-1.25834000485626,-1.,-3.56798645995025));
#38045=CARTESIAN_POINT('Ctrl Pts',(-1.25496090899873,-1.,-3.56071094990825));
#38046=CARTESIAN_POINT('Ctrl Pts',(-1.25188792940508,-1.,-3.5538728741862));
#38047=CARTESIAN_POINT('Ctrl Pts',(-1.24926408627938,-1.,-3.54784190282889));
#38048=CARTESIAN_POINT('Ctrl Pts',(-1.2472164623202,-1.,-3.54294877426113));
#38049=CARTESIAN_POINT('Ctrl Pts',(-1.24593497225964,-1.,-3.53968291129942));
#38050=CARTESIAN_POINT('Ctrl Pts',(-1.2453920538873,-1.,-3.53808746578052));
#38051=CARTESIAN_POINT('Ctrl Pts',(-1.24524498991133,-1.,-3.53744859265385));
#38052=CARTESIAN_POINT('Ctrl Pts',(-1.24524838931864,-1.,-3.53725139174402));
#38053=CARTESIAN_POINT('Ctrl Pts',(-1.24526366418208,-1.,-3.5372048861591));
#38054=CARTESIAN_POINT('',(-1.071677399622,-1.,-3.59360648251021));
#38055=CARTESIAN_POINT('Origin',(0.,-1.,0.));
#38056=CARTESIAN_POINT('',(-1.05427041296137,-1.,-4.06552750530042));
#38057=CARTESIAN_POINT('Ctrl Pts',(-1.071677399622,-1.,-3.59360648251021));
#38058=CARTESIAN_POINT('Ctrl Pts',(-1.07171709254271,-1.,-3.59363512797985));
#38059=CARTESIAN_POINT('Ctrl Pts',(-1.07183575450716,-1.,-3.59379266874663));
#38060=CARTESIAN_POINT('Ctrl Pts',(-1.07209229745284,-1.,-3.59439597));
#38061=CARTESIAN_POINT('Ctrl Pts',(-1.07259084660947,-1.,-3.59600583195037));
#38062=CARTESIAN_POINT('Ctrl Pts',(-1.0734737254567,-1.,-3.59940121154383));
#38063=CARTESIAN_POINT('Ctrl Pts',(-1.0746932716863,-1.,-3.6045633988796));
#38064=CARTESIAN_POINT('Ctrl Pts',(-1.07611545402841,-1.,-3.61098481349577));
#38065=CARTESIAN_POINT('Ctrl Pts',(-1.07764868137729,-1.,-3.61832318504957));
#38066=CARTESIAN_POINT('Ctrl Pts',(-1.07919137290815,-1.,-3.62619537902616));
#38067=CARTESIAN_POINT('Ctrl Pts',(-1.08064765719887,-1.,-3.63423373196602));
#38068=CARTESIAN_POINT('Ctrl Pts',(-1.08194278850972,-1.,-3.64214167843595));
#38069=CARTESIAN_POINT('Ctrl Pts',(-1.08304289898577,-1.,-3.64976441208197));
#38070=CARTESIAN_POINT('Ctrl Pts',(-1.08395671077761,-1.,-3.65709649161004));
#38071=CARTESIAN_POINT('Ctrl Pts',(-1.0847180992287,-1.,-3.66422237895256));
#38072=CARTESIAN_POINT('Ctrl Pts',(-1.0853733414448,-1.,-3.67127347729632));
#38073=CARTESIAN_POINT('Ctrl Pts',(-1.08596755755768,-1.,-3.67838211685148));
#38074=CARTESIAN_POINT('Ctrl Pts',(-1.08652888882609,-1.,-3.68562817420864));
#38075=CARTESIAN_POINT('Ctrl Pts',(-1.08706319540292,-1.,-3.69302062410229));
#38076=CARTESIAN_POINT('Ctrl Pts',(-1.08756311291324,-1.,-3.70052690909884));
#38077=CARTESIAN_POINT('Ctrl Pts',(-1.0880136731219,-1.,-3.70809084139476));
#38078=CARTESIAN_POINT('Ctrl Pts',(-1.08839887334777,-1.,-3.71565372339063));
#38079=CARTESIAN_POINT('Ctrl Pts',(-1.08870887220072,-1.,-3.72317741369364));
#38080=CARTESIAN_POINT('Ctrl Pts',(-1.08894337390925,-1.,-3.73065515162949));
#38081=CARTESIAN_POINT('Ctrl Pts',(-1.08910769013288,-1.,-3.73809879348209));
#38082=CARTESIAN_POINT('Ctrl Pts',(-1.08921040494013,-1.,-3.74553121371745));
#38083=CARTESIAN_POINT('Ctrl Pts',(-1.08926054632927,-1.,-3.75297711748138));
#38084=CARTESIAN_POINT('Ctrl Pts',(-1.08926462734287,-1.,-3.76045342580226));
#38085=CARTESIAN_POINT('Ctrl Pts',(-1.08922484204263,-1.,-3.76796340094469));
#38086=CARTESIAN_POINT('Ctrl Pts',(-1.08914072791275,-1.,-3.7755019940944));
#38087=CARTESIAN_POINT('Ctrl Pts',(-1.08901018614638,-1.,-3.78305911299511));
#38088=CARTESIAN_POINT('Ctrl Pts',(-1.08883071512097,-1.,-3.79062357974401));
#38089=CARTESIAN_POINT('Ctrl Pts',(-1.08860064435776,-1.,-3.79818708705252));
#38090=CARTESIAN_POINT('Ctrl Pts',(-1.08832009255378,-1.,-3.80574726657656));
#38091=CARTESIAN_POINT('Ctrl Pts',(-1.08799030610861,-1.,-3.81330554446324));
#38092=CARTESIAN_POINT('Ctrl Pts',(-1.08761321539442,-1.,-3.82086569676321));
#38093=CARTESIAN_POINT('Ctrl Pts',(-1.08719091307558,-1.,-3.82843215316985));
#38094=CARTESIAN_POINT('Ctrl Pts',(-1.08672515456901,-1.,-3.83600837071702));
#38095=CARTESIAN_POINT('Ctrl Pts',(-1.08621688337601,-1.,-3.84359528764934));
#38096=CARTESIAN_POINT('Ctrl Pts',(-1.08566647671838,-1.,-3.85119211322732));
#38097=CARTESIAN_POINT('Ctrl Pts',(-1.08507395120054,-1.,-3.85879698702511));
#38098=CARTESIAN_POINT('Ctrl Pts',(-1.08443918607926,-1.,-3.86640769434269));
#38099=CARTESIAN_POINT('Ctrl Pts',(-1.0837621330751,-1.,-3.87402233722563));
#38100=CARTESIAN_POINT('Ctrl Pts',(-1.08304304871042,-1.,-3.88164007721365));
#38101=CARTESIAN_POINT('Ctrl Pts',(-1.08228241999363,-1.,-3.88926088975182));
#38102=CARTESIAN_POINT('Ctrl Pts',(-1.08148086931373,-1.,-3.89688525098408));
#38103=CARTESIAN_POINT('Ctrl Pts',(-1.08063906483822,-1.,-3.90451384092564));
#38104=CARTESIAN_POINT('Ctrl Pts',(-1.0797576350746,-1.,-3.91214726022096));
#38105=CARTESIAN_POINT('Ctrl Pts',(-1.07883706663524,-1.,-3.91978568924062));
#38106=CARTESIAN_POINT('Ctrl Pts',(-1.07787771707155,-1.,-3.92742893349684));
#38107=CARTESIAN_POINT('Ctrl Pts',(-1.07687985975348,-1.,-3.93507657572743));
#38108=CARTESIAN_POINT('Ctrl Pts',(-1.07584371946428,-1.,-3.94272809633271));
#38109=CARTESIAN_POINT('Ctrl Pts',(-1.07476950921607,-1.,-3.95038299600754));
#38110=CARTESIAN_POINT('Ctrl Pts',(-1.07365747426551,-1.,-3.95804094429606));
#38111=CARTESIAN_POINT('Ctrl Pts',(-1.07250789943095,-1.,-3.96570179322681));
#38112=CARTESIAN_POINT('Ctrl Pts',(-1.07132109206252,-1.,-3.97336550222571));
#38113=CARTESIAN_POINT('Ctrl Pts',(-1.07009737257815,-1.,-3.98103208801289));
#38114=CARTESIAN_POINT('Ctrl Pts',(-1.06883706263912,-1.,-3.98870156857298));
#38115=CARTESIAN_POINT('Ctrl Pts',(-1.06754047381188,-1.,-3.99637389919958));
#38116=CARTESIAN_POINT('Ctrl Pts',(-1.06620789963406,-1.,-4.00404894951804));
#38117=CARTESIAN_POINT('Ctrl Pts',(-1.06483961342894,-1.,-4.0117265418656));
#38118=CARTESIAN_POINT('Ctrl Pts',(-1.06343586496094,-1.,-4.0194064749539));
#38119=CARTESIAN_POINT('Ctrl Pts',(-1.06199687787488,-1.,-4.02708855235732));
#38120=CARTESIAN_POINT('Ctrl Pts',(-1.06052284712114,-1.,-4.03477261142549));
#38121=CARTESIAN_POINT('Ctrl Pts',(-1.05901393667039,-1.,-4.04245854429333));
#38122=CARTESIAN_POINT('Ctrl Pts',(-1.05747027728537,-1.,-4.05014628387112));
#38123=CARTESIAN_POINT('Ctrl Pts',(-1.0562076270849,-1.,-4.05629789308941));
#38124=CARTESIAN_POINT('Ctrl Pts',(-1.05524507177901,-1.,-4.06091239150293));
#38125=CARTESIAN_POINT('Ctrl Pts',(-1.05459645194934,-1.,-4.06398907542679));
#38126=CARTESIAN_POINT('Ctrl Pts',(-1.05427041296137,-1.,-4.06552750530042));
#38127=CARTESIAN_POINT('',(-0.906349047628866,-1.,-4.10104028313088));
#38128=CARTESIAN_POINT('',(-1.05427041296137,-1.,-4.06552750530042));
#38129=CARTESIAN_POINT('',(-0.676591647975429,-1.,-3.68845817949586));
#38130=CARTESIAN_POINT('Ctrl Pts',(-0.906349047628866,-1.,-4.10104028313088));
#38131=CARTESIAN_POINT('Ctrl Pts',(-0.905360112215337,-1.,-4.09981755067523));
#38132=CARTESIAN_POINT('Ctrl Pts',(-0.903385402441587,-1.,-4.09737067245935));
#38133=CARTESIAN_POINT('Ctrl Pts',(-0.900432820941675,-1.,-4.09369611522387));
#38134=CARTESIAN_POINT('Ctrl Pts',(-0.896515019231333,-1.,-4.08878822246833));
#38135=CARTESIAN_POINT('Ctrl Pts',(-0.891649447916278,-1.,-4.08263920304799));
#38136=CARTESIAN_POINT('Ctrl Pts',(-0.886815658358501,-1.,-4.07647601773635));
#38137=CARTESIAN_POINT('Ctrl Pts',(-0.882013797525692,-1.,-4.07029866694192));
#38138=CARTESIAN_POINT('Ctrl Pts',(-0.877244060485837,-1.,-4.06410717232905));
#38139=CARTESIAN_POINT('Ctrl Pts',(-0.872506694782446,-1.,-4.0579015903134));
#38140=CARTESIAN_POINT('Ctrl Pts',(-0.867801988859917,-1.,-4.05168199437909));
#38141=CARTESIAN_POINT('Ctrl Pts',(-0.863130256643259,-1.,-4.04544845048584));
#38142=CARTESIAN_POINT('Ctrl Pts',(-0.858491822322827,-1.,-4.03920099284773));
#38143=CARTESIAN_POINT('Ctrl Pts',(-0.853887006631755,-1.,-4.03293960436756));
#38144=CARTESIAN_POINT('Ctrl Pts',(-0.849316107474245,-1.,-4.02666418343164));
#38145=CARTESIAN_POINT('Ctrl Pts',(-0.844779403287745,-1.,-4.02037456798441));
#38146=CARTESIAN_POINT('Ctrl Pts',(-0.840277171975855,-1.,-4.01407059766103));
#38147=CARTESIAN_POINT('Ctrl Pts',(-0.835809705809646,-1.,-4.00775216907856));
#38148=CARTESIAN_POINT('Ctrl Pts',(-0.831377325741622,-1.,-4.00141928477507));
#38149=CARTESIAN_POINT('Ctrl Pts',(-0.826980400320789,-1.,-3.99507212784431));
#38150=CARTESIAN_POINT('Ctrl Pts',(-0.822619346022119,-1.,-3.98871104646485));
#38151=CARTESIAN_POINT('Ctrl Pts',(-0.818294599022293,-1.,-3.98233640155404));
#38152=CARTESIAN_POINT('Ctrl Pts',(-0.814006592328844,-1.,-3.97594844078811));
#38153=CARTESIAN_POINT('Ctrl Pts',(-0.809755732818091,-1.,-3.96954717513232));
#38154=CARTESIAN_POINT('Ctrl Pts',(-0.805542372178361,-1.,-3.96313222295815));
#38155=CARTESIAN_POINT('Ctrl Pts',(-0.801366797727049,-1.,-3.95670276375108));
#38156=CARTESIAN_POINT('Ctrl Pts',(-0.797229296085316,-1.,-3.95025788827136));
#38157=CARTESIAN_POINT('Ctrl Pts',(-0.793130205640961,-1.,-3.94379688971283));
#38158=CARTESIAN_POINT('Ctrl Pts',(-0.789069971469333,-1.,-3.93731956885676));
#38159=CARTESIAN_POINT('Ctrl Pts',(-0.785049202786507,-1.,-3.93082655631789));
#38160=CARTESIAN_POINT('Ctrl Pts',(-0.781068718228451,-1.,-3.92431956510441));
#38161=CARTESIAN_POINT('Ctrl Pts',(-0.777129415664956,-1.,-3.9178006233448));
#38162=CARTESIAN_POINT('Ctrl Pts',(-0.773232154506321,-1.,-3.91127138115243));
#38163=CARTESIAN_POINT('Ctrl Pts',(-0.769377629847874,-1.,-3.90473237182633));
#38164=CARTESIAN_POINT('Ctrl Pts',(-0.765566256401295,-1.,-3.89818233104378));
#38165=CARTESIAN_POINT('Ctrl Pts',(-0.76179802879397,-1.,-3.89161738162245));
#38166=CARTESIAN_POINT('Ctrl Pts',(-0.758072800564801,-1.,-3.88503262662689));
#38167=CARTESIAN_POINT('Ctrl Pts',(-0.754390577396856,-1.,-3.87842382520065));
#38168=CARTESIAN_POINT('Ctrl Pts',(-0.750751822383028,-1.,-3.87178914078374));
#38169=CARTESIAN_POINT('Ctrl Pts',(-0.747157716488871,-1.,-3.86513062969889));
#38170=CARTESIAN_POINT('Ctrl Pts',(-0.743610542737012,-1.,-3.85845645217594));
#38171=CARTESIAN_POINT('Ctrl Pts',(-0.740113146827137,-1.,-3.85177770351215));
#38172=CARTESIAN_POINT('Ctrl Pts',(-0.736668240497117,-1.,-3.84510432881213));
#38173=CARTESIAN_POINT('Ctrl Pts',(-0.733277703756078,-1.,-3.83844103658009));
#38174=CARTESIAN_POINT('Ctrl Pts',(-0.729942010490168,-1.,-3.83178392403383));
#38175=CARTESIAN_POINT('Ctrl Pts',(-0.726659281876664,-1.,-3.82511495756713));
#38176=CARTESIAN_POINT('Ctrl Pts',(-0.723426346019423,-1.,-3.81840802610835));
#38177=CARTESIAN_POINT('Ctrl Pts',(-0.720240466589236,-1.,-3.81163885127344));
#38178=CARTESIAN_POINT('Ctrl Pts',(-0.717100993669114,-1.,-3.80479445759309));
#38179=CARTESIAN_POINT('Ctrl Pts',(-0.714010733006641,-1.,-3.79788100314975));
#38180=CARTESIAN_POINT('Ctrl Pts',(-0.710978231689017,-1.,-3.79093694007094));
#38181=CARTESIAN_POINT('Ctrl Pts',(-0.708015879375459,-1.,-3.78402183336605));
#38182=CARTESIAN_POINT('Ctrl Pts',(-0.705135847999817,-1.,-3.77719254217129));
#38183=CARTESIAN_POINT('Ctrl Pts',(-0.702346356621552,-1.,-3.77048141872872));
#38184=CARTESIAN_POINT('Ctrl Pts',(-0.699648552230917,-1.,-3.76387780603759));
#38185=CARTESIAN_POINT('Ctrl Pts',(-0.697031245659744,-1.,-3.75729775767023));
#38186=CARTESIAN_POINT('Ctrl Pts',(-0.694474562581493,-1.,-3.75060288243455));
#38187=CARTESIAN_POINT('Ctrl Pts',(-0.69196008040082,-1.,-3.74365508986712));
#38188=CARTESIAN_POINT('Ctrl Pts',(-0.689479637354814,-1.,-3.73636374475077));
#38189=CARTESIAN_POINT('Ctrl Pts',(-0.687043475232355,-1.,-3.72872973554051));
#38190=CARTESIAN_POINT('Ctrl Pts',(-0.684691698167848,-1.,-3.7209063713926));
#38191=CARTESIAN_POINT('Ctrl Pts',(-0.68249234510893,-1.,-3.71319182789943));
#38192=CARTESIAN_POINT('Ctrl Pts',(-0.680526909710877,-1.,-3.70595722031785));
#38193=CARTESIAN_POINT('Ctrl Pts',(-0.678878822226026,-1.,-3.69959004073005));
#38194=CARTESIAN_POINT('Ctrl Pts',(-0.677621861865498,-1.,-3.69443683573598));
#38195=CARTESIAN_POINT('Ctrl Pts',(-0.676867042599401,-1.,-3.69101071175464));
#38196=CARTESIAN_POINT('Ctrl Pts',(-0.676580391119396,-1.,-3.68934997767243));
#38197=CARTESIAN_POINT('Ctrl Pts',(-0.676535079520807,-1.,-3.68869596425969));
#38198=CARTESIAN_POINT('Ctrl Pts',(-0.676569286094606,-1.,-3.68850172300477));
#38199=CARTESIAN_POINT('Ctrl Pts',(-0.676591647975429,-1.,-3.68845817949586));
#38200=CARTESIAN_POINT('',(-0.496319364829374,-1.,-3.71701050416802));
#38201=CARTESIAN_POINT('Origin',(0.,-1.,0.));
#38202=CARTESIAN_POINT('',(-0.405301974318349,-1.,-4.18039834341342));
#38203=CARTESIAN_POINT('Ctrl Pts',(-0.496319364829374,-1.,-3.71701050416802));
#38204=CARTESIAN_POINT('Ctrl Pts',(-0.496354087925646,-1.,-3.71704500630521));
#38205=CARTESIAN_POINT('Ctrl Pts',(-0.496446644158827,-1.,-3.71721917030465));
#38206=CARTESIAN_POINT('Ctrl Pts',(-0.496605651526314,-1.,-3.71785517607694));
#38207=CARTESIAN_POINT('Ctrl Pts',(-0.496846224822535,-1.,-3.7195232082259));
#38208=CARTESIAN_POINT('Ctrl Pts',(-0.497187079575794,-1.,-3.72301489774241));
#38209=CARTESIAN_POINT('Ctrl Pts',(-0.497584067153279,-1.,-3.72830430904794));
#38210=CARTESIAN_POINT('Ctrl Pts',(-0.497984209510495,-1.,-3.73486914372834));
#38211=CARTESIAN_POINT('Ctrl Pts',(-0.498350586058176,-1.,-3.74235701735109));
#38212=CARTESIAN_POINT('Ctrl Pts',(-0.498642802042929,-1.,-3.75037362168103));
#38213=CARTESIAN_POINT('Ctrl Pts',(-0.498823681615513,-1.,-3.75854082221127));
#38214=CARTESIAN_POINT('Ctrl Pts',(-0.498865792335185,-1.,-3.76655401191144));
#38215=CARTESIAN_POINT('Ctrl Pts',(-0.498759900365687,-1.,-3.77425499225089));
#38216=CARTESIAN_POINT('Ctrl Pts',(-0.498515471679378,-1.,-3.78163975337189));
#38217=CARTESIAN_POINT('Ctrl Pts',(-0.498152751800819,-1.,-3.78879701661152));
#38218=CARTESIAN_POINT('Ctrl Pts',(-0.49769689210058,-1.,-3.79586380669959));
#38219=CARTESIAN_POINT('Ctrl Pts',(-0.497171756201091,-1.,-3.80297788298545));
#38220=CARTESIAN_POINT('Ctrl Pts',(-0.496592643443789,-1.,-3.81022254090909));
#38221=CARTESIAN_POINT('Ctrl Pts',(-0.495963937875572,-1.,-3.81760756144099));
#38222=CARTESIAN_POINT('Ctrl Pts',(-0.495283458893903,-1.,-3.82509963594156));
#38223=CARTESIAN_POINT('Ctrl Pts',(-0.494545212256425,-1.,-3.8326409268245));
#38224=CARTESIAN_POINT('Ctrl Pts',(-0.493742574629117,-1.,-3.84017095578438));
#38225=CARTESIAN_POINT('Ctrl Pts',(-0.492871792414095,-1.,-3.84765051147965));
#38226=CARTESIAN_POINT('Ctrl Pts',(-0.49193363108376,-1.,-3.85507287020223));
#38227=CARTESIAN_POINT('Ctrl Pts',(-0.490931482170849,-1.,-3.86245057319215));
#38228=CARTESIAN_POINT('Ctrl Pts',(-0.489870245704899,-1.,-3.86980755613694));
#38229=CARTESIAN_POINT('Ctrl Pts',(-0.488754973798281,-1.,-3.87716963231115));
#38230=CARTESIAN_POINT('Ctrl Pts',(-0.487589452275179,-1.,-3.88455453328156));
#38231=CARTESIAN_POINT('Ctrl Pts',(-0.486375337854133,-1.,-3.89196582437574));
#38232=CARTESIAN_POINT('Ctrl Pts',(-0.485112963522246,-1.,-3.89939844658529));
#38233=CARTESIAN_POINT('Ctrl Pts',(-0.483801835089161,-1.,-3.90684210358063));
#38234=CARTESIAN_POINT('Ctrl Pts',(-0.482441230340709,-1.,-3.91428536373749));
#38235=CARTESIAN_POINT('Ctrl Pts',(-0.481030798910735,-1.,-3.92171976072334));
#38236=CARTESIAN_POINT('Ctrl Pts',(-0.479571028525566,-1.,-3.92914297392067));
#38237=CARTESIAN_POINT('Ctrl Pts',(-0.478062927140957,-1.,-3.93655660689819));
#38238=CARTESIAN_POINT('Ctrl Pts',(-0.476507810658535,-1.,-3.94396469119385));
#38239=CARTESIAN_POINT('Ctrl Pts',(-0.47490705302179,-1.,-3.95137192932898));
#38240=CARTESIAN_POINT('Ctrl Pts',(-0.473261847236296,-1.,-3.95878201038332));
#38241=CARTESIAN_POINT('Ctrl Pts',(-0.471572978413493,-1.,-3.96619600864626));
#38242=CARTESIAN_POINT('Ctrl Pts',(-0.469840942829878,-1.,-3.97361320212413));
#38243=CARTESIAN_POINT('Ctrl Pts',(-0.46806604792014,-1.,-3.98103175589349));
#38244=CARTESIAN_POINT('Ctrl Pts',(-0.466248520883034,-1.,-3.98844946363258));
#38245=CARTESIAN_POINT('Ctrl Pts',(-0.464388610938995,-1.,-3.99586444320134));
#38246=CARTESIAN_POINT('Ctrl Pts',(-0.462486702616252,-1.,-4.00327590659129));
#38247=CARTESIAN_POINT('Ctrl Pts',(-0.460543280768577,-1.,-4.01068390573469));
#38248=CARTESIAN_POINT('Ctrl Pts',(-0.458558885637001,-1.,-4.01808900827647));
#38249=CARTESIAN_POINT('Ctrl Pts',(-0.456534070784968,-1.,-4.02549199038414));
#38250=CARTESIAN_POINT('Ctrl Pts',(-0.454469363020495,-1.,-4.03289354362745));
#38251=CARTESIAN_POINT('Ctrl Pts',(-0.452365214748779,-1.,-4.0402939222793));
#38252=CARTESIAN_POINT('Ctrl Pts',(-0.450222009543774,-1.,-4.0476929901797));
#38253=CARTESIAN_POINT('Ctrl Pts',(-0.448040082683976,-1.,-4.05509037796815));
#38254=CARTESIAN_POINT('Ctrl Pts',(-0.445819737468478,-1.,-4.06248560760596));
#38255=CARTESIAN_POINT('Ctrl Pts',(-0.443561262395408,-1.,-4.0698782192577));
#38256=CARTESIAN_POINT('Ctrl Pts',(-0.441264951396587,-1.,-4.07726792490256));
#38257=CARTESIAN_POINT('Ctrl Pts',(-0.438931108931613,-1.,-4.08465462294625));
#38258=CARTESIAN_POINT('Ctrl Pts',(-0.436560044913814,-1.,-4.09203832139439));
#38259=CARTESIAN_POINT('Ctrl Pts',(-0.434152073200643,-1.,-4.09941908688567));
#38260=CARTESIAN_POINT('Ctrl Pts',(-0.431707508679772,-1.,-4.10679698750219));
#38261=CARTESIAN_POINT('Ctrl Pts',(-0.429226666075372,-1.,-4.1141720278277));
#38262=CARTESIAN_POINT('Ctrl Pts',(-0.426709855706243,-1.,-4.1215441250121));
#38263=CARTESIAN_POINT('Ctrl Pts',(-0.424157375323155,-1.,-4.1289131463371));
#38264=CARTESIAN_POINT('Ctrl Pts',(-0.421569503103971,-1.,-4.13627893206433));
#38265=CARTESIAN_POINT('Ctrl Pts',(-0.4189464906678,-1.,-4.14364132317223));
#38266=CARTESIAN_POINT('Ctrl Pts',(-0.416288556008986,-1.,-4.15100018950989));
#38267=CARTESIAN_POINT('Ctrl Pts',(-0.413595877953269,-1.,-4.1583554501909));
#38268=CARTESIAN_POINT('Ctrl Pts',(-0.410868596148614,-1.,-4.16570705940731));
#38269=CARTESIAN_POINT('Ctrl Pts',(-0.408659167570153,-1.,-4.17158541009947));
#38270=CARTESIAN_POINT('Ctrl Pts',(-0.406986596326602,-1.,-4.17599251955585));
#38271=CARTESIAN_POINT('Ctrl Pts',(-0.405864662679631,-1.,-4.17892985789908));
#38272=CARTESIAN_POINT('Ctrl Pts',(-0.405301974318349,-1.,-4.18039834341342));
#38273=CARTESIAN_POINT('',(-0.253646344052521,-1.,-4.1923339003649));
#38274=CARTESIAN_POINT('',(-0.405301974318349,-1.,-4.18039834341342));
#38275=CARTESIAN_POINT('',(-0.0912596999166825,-1.,-3.74888939116255));
#38276=CARTESIAN_POINT('Ctrl Pts',(-0.253646344052521,-1.,-4.1923339003649));
#38277=CARTESIAN_POINT('Ctrl Pts',(-0.252860861572565,-1.,-4.19097151819241));
#38278=CARTESIAN_POINT('Ctrl Pts',(-0.251293239837693,-1.,-4.18824585244066));
#38279=CARTESIAN_POINT('Ctrl Pts',(-0.248951836910964,-1.,-4.18415464959491));
#38280=CARTESIAN_POINT('Ctrl Pts',(-0.245850033418583,-1.,-4.17869430192868));
#38281=CARTESIAN_POINT('Ctrl Pts',(-0.242006283923912,-1.,-4.17185984409533));
#38282=CARTESIAN_POINT('Ctrl Pts',(-0.238196140933977,-1.,-4.1650163665385));
#38283=CARTESIAN_POINT('Ctrl Pts',(-0.234419749543143,-1.,-4.1581638926525));
#38284=CARTESIAN_POINT('Ctrl Pts',(-0.230677299028738,-1.,-4.15130247435029));
#38285=CARTESIAN_POINT('Ctrl Pts',(-0.226969025061243,-1.,-4.14443220607733));
#38286=CARTESIAN_POINT('Ctrl Pts',(-0.223295201038383,-1.,-4.13755320553563));
#38287=CARTESIAN_POINT('Ctrl Pts',(-0.219656126701852,-1.,-4.13066558698156));
#38288=CARTESIAN_POINT('Ctrl Pts',(-0.216052116898425,-1.,-4.12376943492249));
#38289=CARTESIAN_POINT('Ctrl Pts',(-0.212483491087068,-1.,-4.11686478264545));
#38290=CARTESIAN_POINT('Ctrl Pts',(-0.208950559400172,-1.,-4.10995157639026));
#38291=CARTESIAN_POINT('Ctrl Pts',(-0.205453622198233,-1.,-4.10302969965374));
#38292=CARTESIAN_POINT('Ctrl Pts',(-0.201992979049984,-1.,-4.09609903751912));
#38293=CARTESIAN_POINT('Ctrl Pts',(-0.198568934800811,-1.,-4.08915953359753));
#38294=CARTESIAN_POINT('Ctrl Pts',(-0.195181806054714,-1.,-4.08221124060385));
#38295=CARTESIAN_POINT('Ctrl Pts',(-0.191831928181081,-1.,-4.07525439703137));
#38296=CARTESIAN_POINT('Ctrl Pts',(-0.188519658060255,-1.,-4.06828941192308));
#38297=CARTESIAN_POINT('Ctrl Pts',(-0.185245370038948,-1.,-4.06131670998589));
#38298=CARTESIAN_POINT('Ctrl Pts',(-0.18200945304855,-1.,-4.05433660358402));
#38299=CARTESIAN_POINT('Ctrl Pts',(-0.178812307240716,-1.,-4.04734916719722));
#38300=CARTESIAN_POINT('Ctrl Pts',(-0.175654339673757,-1.,-4.04035407891161));
#38301=CARTESIAN_POINT('Ctrl Pts',(-0.172535962484466,-1.,-4.03335057326093));
#38302=CARTESIAN_POINT('Ctrl Pts',(-0.169457601001653,-1.,-4.0263377970371));
#38303=CARTESIAN_POINT('Ctrl Pts',(-0.166419700015847,-1.,-4.01931510507143));
#38304=CARTESIAN_POINT('Ctrl Pts',(-0.163422730287459,-1.,-4.01228237022301));
#38305=CARTESIAN_POINT('Ctrl Pts',(-0.160467194882219,-1.,-4.00524031064509));
#38306=CARTESIAN_POINT('Ctrl Pts',(-0.15755363438381,-1.,-3.99819074631874));
#38307=CARTESIAN_POINT('Ctrl Pts',(-0.154682618338563,-1.,-3.99113582086059));
#38308=CARTESIAN_POINT('Ctrl Pts',(-0.151854737441405,-1.,-3.9840772985098));
#38309=CARTESIAN_POINT('Ctrl Pts',(-0.149070594803544,-1.,-3.97701581473643));
#38310=CARTESIAN_POINT('Ctrl Pts',(-0.146330797814513,-1.,-3.96995018565891));
#38311=CARTESIAN_POINT('Ctrl Pts',(-0.143635947692791,-1.,-3.96287658098896));
#38312=CARTESIAN_POINT('Ctrl Pts',(-0.140986665829937,-1.,-3.95579014116899));
#38313=CARTESIAN_POINT('Ctrl Pts',(-0.138383621255159,-1.,-3.94868667844355));
#38314=CARTESIAN_POINT('Ctrl Pts',(-0.135827558661188,-1.,-3.94156445130744));
#38315=CARTESIAN_POINT('Ctrl Pts',(-0.13331932279419,-1.,-3.93442567551035));
#38316=CARTESIAN_POINT('Ctrl Pts',(-0.130859892027799,-1.,-3.9272787679596));
#38317=CARTESIAN_POINT('Ctrl Pts',(-0.128450341339528,-1.,-3.92013513251642));
#38318=CARTESIAN_POINT('Ctrl Pts',(-0.126091793324137,-1.,-3.91300501605392));
#38319=CARTESIAN_POINT('Ctrl Pts',(-0.123785368272377,-1.,-3.90589336320508));
#38320=CARTESIAN_POINT('Ctrl Pts',(-0.121532144765723,-1.,-3.89879639336952));
#38321=CARTESIAN_POINT('Ctrl Pts',(-0.119333088190417,-1.,-3.89169600105201));
#38322=CARTESIAN_POINT('Ctrl Pts',(-0.117189150373144,-1.,-3.88456590045767));
#38323=CARTESIAN_POINT('Ctrl Pts',(-0.11510142664947,-1.,-3.87738168405343));
#38324=CARTESIAN_POINT('Ctrl Pts',(-0.113071304914562,-1.,-3.87013043445014));
#38325=CARTESIAN_POINT('Ctrl Pts',(-0.11110059303626,-1.,-3.86281867282965));
#38326=CARTESIAN_POINT('Ctrl Pts',(-0.109191717634944,-1.,-3.855485714969));
#38327=CARTESIAN_POINT('Ctrl Pts',(-0.107347597812184,-1.,-3.84819233070317));
#38328=CARTESIAN_POINT('Ctrl Pts',(-0.105571360916569,-1.,-3.84099658324803));
#38329=CARTESIAN_POINT('Ctrl Pts',(-0.103866063811623,-1.,-3.83393171228002));
#38330=CARTESIAN_POINT('Ctrl Pts',(-0.102234506488456,-1.,-3.82698737143255));
#38331=CARTESIAN_POINT('Ctrl Pts',(-0.100678769650632,-1.,-3.82007889742625));
#38332=CARTESIAN_POINT('Ctrl Pts',(-0.0992008728096516,-1.,-3.81306649386461));
#38333=CARTESIAN_POINT('Ctrl Pts',(-0.0978042222906645,-1.,-3.80581088847809));
#38334=CARTESIAN_POINT('Ctrl Pts',(-0.0964949352873133,-1.,-3.79822128513845));
#38335=CARTESIAN_POINT('Ctrl Pts',(-0.0952829885100802,-1.,-3.79030016353111));
#38336=CARTESIAN_POINT('Ctrl Pts',(-0.0941840095090815,-1.,-3.782205218991));
#38337=CARTESIAN_POINT('Ctrl Pts',(-0.093218554620318,-1.,-3.77424159971059));
#38338=CARTESIAN_POINT('Ctrl Pts',(-0.0924090589602692,-1.,-3.76678860031841));
#38339=CARTESIAN_POINT('Ctrl Pts',(-0.0917773084998337,-1.,-3.76024199359303));
#38340=CARTESIAN_POINT('Ctrl Pts',(-0.09134196227364,-1.,-3.75495560118212));
#38341=CARTESIAN_POINT('Ctrl Pts',(-0.0911323999574428,-1.,-3.75145357872422));
#38342=CARTESIAN_POINT('Ctrl Pts',(-0.0911090736805512,-1.,-3.74976844886346));
#38343=CARTESIAN_POINT('Ctrl Pts',(-0.0911666301812819,-1.,-3.74911539914542));
#38344=CARTESIAN_POINT('Ctrl Pts',(-0.0912308016421982,-1.,-3.74892890040974));
#38345=CARTESIAN_POINT('Ctrl Pts',(-0.0912596999166825,-1.,-3.74888939116255));
#38346=CARTESIAN_POINT('',(0.0912596999148854,-1.,-3.74888939116259));
#38347=CARTESIAN_POINT('Origin',(0.,-1.,0.));
#38348=CARTESIAN_POINT('',(0.253646344052522,-1.,-4.1923339003649));
#38349=CARTESIAN_POINT('Ctrl Pts',(0.0912596999148854,-1.,-3.74888939116259));
#38350=CARTESIAN_POINT('Ctrl Pts',(0.0912308016409229,-1.,-3.74892890041021));
#38351=CARTESIAN_POINT('Ctrl Pts',(0.0911666301806421,-1.,-3.74911539914664));
#38352=CARTESIAN_POINT('Ctrl Pts',(0.0911090736804568,-1.,-3.74976844886495));
#38353=CARTESIAN_POINT('Ctrl Pts',(0.0911323999576141,-1.,-3.75145357872511));
#38354=CARTESIAN_POINT('Ctrl Pts',(0.0913419622735849,-1.,-3.75495560118053));
#38355=CARTESIAN_POINT('Ctrl Pts',(0.0917773084999005,-1.,-3.76024199359493));
#38356=CARTESIAN_POINT('Ctrl Pts',(0.0924090589604052,-1.,-3.76678860032228));
#38357=CARTESIAN_POINT('Ctrl Pts',(0.0932185546204571,-1.,-3.77424159971456));
#38358=CARTESIAN_POINT('Ctrl Pts',(0.094184009509174,-1.,-3.78220521899366));
#38359=CARTESIAN_POINT('Ctrl Pts',(0.0952829885101065,-1.,-3.79030016353186));
#38360=CARTESIAN_POINT('Ctrl Pts',(0.0964949352872842,-1.,-3.7982212851376));
#38361=CARTESIAN_POINT('Ctrl Pts',(0.0978042222906071,-1.,-3.80581088847642));
#38362=CARTESIAN_POINT('Ctrl Pts',(0.099200872809594,-1.,-3.81306649386293));
#38363=CARTESIAN_POINT('Ctrl Pts',(0.100678769650594,-1.,-3.82007889742512));
#38364=CARTESIAN_POINT('Ctrl Pts',(0.102234506488445,-1.,-3.8269873714322));
#38365=CARTESIAN_POINT('Ctrl Pts',(0.103866063811634,-1.,-3.83393171228034));
#38366=CARTESIAN_POINT('Ctrl Pts',(0.105571360916593,-1.,-3.84099658324873));
#38367=CARTESIAN_POINT('Ctrl Pts',(0.107347597812208,-1.,-3.84819233070391));
#38368=CARTESIAN_POINT('Ctrl Pts',(0.10919171763496,-1.,-3.85548571496953));
#38369=CARTESIAN_POINT('Ctrl Pts',(0.111100593036266,-1.,-3.86281867282984));
#38370=CARTESIAN_POINT('Ctrl Pts',(0.113071304914558,-1.,-3.87013043445001));
#38371=CARTESIAN_POINT('Ctrl Pts',(0.11510142664946,-1.,-3.87738168405308));
#38372=CARTESIAN_POINT('Ctrl Pts',(0.117189150373134,-1.,-3.88456590045726));
#38373=CARTESIAN_POINT('Ctrl Pts',(0.11933308819041,-1.,-3.8916960010517));
#38374=CARTESIAN_POINT('Ctrl Pts',(0.121532144765721,-1.,-3.89879639336939));
#38375=CARTESIAN_POINT('Ctrl Pts',(0.123785368272379,-1.,-3.90589336320515));
#38376=CARTESIAN_POINT('Ctrl Pts',(0.126091793324141,-1.,-3.91300501605411));
#38377=CARTESIAN_POINT('Ctrl Pts',(0.128450341339532,-1.,-3.92013513251664));
#38378=CARTESIAN_POINT('Ctrl Pts',(0.130859892027801,-1.,-3.92727876795977));
#38379=CARTESIAN_POINT('Ctrl Pts',(0.13331932279419,-1.,-3.93442567551042));
#38380=CARTESIAN_POINT('Ctrl Pts',(0.135827558661188,-1.,-3.94156445130741));
#38381=CARTESIAN_POINT('Ctrl Pts',(0.138383621255161,-1.,-3.94868667844347));
#38382=CARTESIAN_POINT('Ctrl Pts',(0.140986665829942,-1.,-3.95579014116894));
#38383=CARTESIAN_POINT('Ctrl Pts',(0.143635947692798,-1.,-3.96287658098896));
#38384=CARTESIAN_POINT('Ctrl Pts',(0.14633079781452,-1.,-3.96995018565893));
#38385=CARTESIAN_POINT('Ctrl Pts',(0.149070594803544,-1.,-3.97701581473644));
#38386=CARTESIAN_POINT('Ctrl Pts',(0.151854737441398,-1.,-3.98407729850975));
#38387=CARTESIAN_POINT('Ctrl Pts',(0.154682618338547,-1.,-3.99113582086043));
#38388=CARTESIAN_POINT('Ctrl Pts',(0.15755363438379,-1.,-3.9981907463185));
#38389=CARTESIAN_POINT('Ctrl Pts',(0.160467194882202,-1.,-4.00524031064487));
#38390=CARTESIAN_POINT('Ctrl Pts',(0.163422730287456,-1.,-4.01228237022296));
#38391=CARTESIAN_POINT('Ctrl Pts',(0.166419700015865,-1.,-4.01931510507167));
#38392=CARTESIAN_POINT('Ctrl Pts',(0.169457601001691,-1.,-4.02633779703764));
#38393=CARTESIAN_POINT('Ctrl Pts',(0.172535962484514,-1.,-4.03335057326163));
#38394=CARTESIAN_POINT('Ctrl Pts',(0.175654339673797,-1.,-4.04035407891222));
#38395=CARTESIAN_POINT('Ctrl Pts',(0.178812307240728,-1.,-4.04734916719741));
#38396=CARTESIAN_POINT('Ctrl Pts',(0.182009453048519,-1.,-4.05433660358353));
#38397=CARTESIAN_POINT('Ctrl Pts',(0.185245370038873,-1.,-4.06131670998469));
#38398=CARTESIAN_POINT('Ctrl Pts',(0.188519658060155,-1.,-4.06828941192147));
#38399=CARTESIAN_POINT('Ctrl Pts',(0.19183192818099,-1.,-4.07525439702992));
#38400=CARTESIAN_POINT('Ctrl Pts',(0.195181806054675,-1.,-4.08221124060322));
#38401=CARTESIAN_POINT('Ctrl Pts',(0.198568934800861,-1.,-4.08915953359833));
#38402=CARTESIAN_POINT('Ctrl Pts',(0.201992979050135,-1.,-4.09609903752152));
#38403=CARTESIAN_POINT('Ctrl Pts',(0.205453622198454,-1.,-4.10302969965728));
#38404=CARTESIAN_POINT('Ctrl Pts',(0.208950559400392,-1.,-4.10995157639377));
#38405=CARTESIAN_POINT('Ctrl Pts',(0.212483491087189,-1.,-4.11686478264739));
#38406=CARTESIAN_POINT('Ctrl Pts',(0.216052116898351,-1.,-4.12376943492132));
#38407=CARTESIAN_POINT('Ctrl Pts',(0.219656126701541,-1.,-4.13066558697658));
#38408=CARTESIAN_POINT('Ctrl Pts',(0.223295201037885,-1.,-4.13755320552764));
#38409=CARTESIAN_POINT('Ctrl Pts',(0.226969025060705,-1.,-4.14443220606869));
#38410=CARTESIAN_POINT('Ctrl Pts',(0.230677299028383,-1.,-4.15130247434459));
#38411=CARTESIAN_POINT('Ctrl Pts',(0.234419749543207,-1.,-4.15816389265352));
#38412=CARTESIAN_POINT('Ctrl Pts',(0.238196140934616,-1.,-4.16501636654877));
#38413=CARTESIAN_POINT('Ctrl Pts',(0.242006283925088,-1.,-4.17185984411426));
#38414=CARTESIAN_POINT('Ctrl Pts',(0.245850033420019,-1.,-4.1786943019518));
#38415=CARTESIAN_POINT('Ctrl Pts',(0.248951836912189,-1.,-4.18415464961466));
#38416=CARTESIAN_POINT('Ctrl Pts',(0.25129323983844,-1.,-4.18824585245272));
#38417=CARTESIAN_POINT('Ctrl Pts',(0.25286086157284,-1.,-4.19097151819684));
#38418=CARTESIAN_POINT('Ctrl Pts',(0.253646344052522,-1.,-4.1923339003649));
#38419=CARTESIAN_POINT('',(0.40530197431835,-1.,-4.18039834341342));
#38420=CARTESIAN_POINT('',(0.253646344052522,-1.,-4.1923339003649));
#38421=CARTESIAN_POINT('',(0.496319364827592,-1.,-3.71701050416825));
#38422=CARTESIAN_POINT('Ctrl Pts',(0.40530197431835,-1.,-4.18039834341342));
#38423=CARTESIAN_POINT('Ctrl Pts',(0.405864662679209,-1.,-4.17892985789466));
#38424=CARTESIAN_POINT('Ctrl Pts',(0.406986596325454,-1.,-4.17599251954382));
#38425=CARTESIAN_POINT('Ctrl Pts',(0.408659167568273,-1.,-4.17158541007977));
#38426=CARTESIAN_POINT('Ctrl Pts',(0.410868596146414,-1.,-4.16570705938425));
#38427=CARTESIAN_POINT('Ctrl Pts',(0.41359587795147,-1.,-4.15835545017202));
#38428=CARTESIAN_POINT('Ctrl Pts',(0.416288556008011,-1.,-4.15100018949965));
#38429=CARTESIAN_POINT('Ctrl Pts',(0.418946490667702,-1.,-4.14364132317121));
#38430=CARTESIAN_POINT('Ctrl Pts',(0.421569503104512,-1.,-4.13627893207002));
#38431=CARTESIAN_POINT('Ctrl Pts',(0.424157375323975,-1.,-4.12891314634572));
#38432=CARTESIAN_POINT('Ctrl Pts',(0.426709855707,-1.,-4.12154412502007));
#38433=CARTESIAN_POINT('Ctrl Pts',(0.429226666075844,-1.,-4.11417202783267));
#38434=CARTESIAN_POINT('Ctrl Pts',(0.431707508679883,-1.,-4.10679698750336));
#38435=CARTESIAN_POINT('Ctrl Pts',(0.43415207320046,-1.,-4.09941908688373));
#38436=CARTESIAN_POINT('Ctrl Pts',(0.436560044913482,-1.,-4.09203832139089));
#38437=CARTESIAN_POINT('Ctrl Pts',(0.438931108931279,-1.,-4.08465462294273));
#38438=CARTESIAN_POINT('Ctrl Pts',(0.44126495139636,-1.,-4.07726792490016));
#38439=CARTESIAN_POINT('Ctrl Pts',(0.443561262395332,-1.,-4.0698782192569));
#38440=CARTESIAN_POINT('Ctrl Pts',(0.445819737468537,-1.,-4.06248560760659));
#38441=CARTESIAN_POINT('Ctrl Pts',(0.448040082684114,-1.,-4.0550903779696));
#38442=CARTESIAN_POINT('Ctrl Pts',(0.450222009543926,-1.,-4.0476929901813));
#38443=CARTESIAN_POINT('Ctrl Pts',(0.452365214748892,-1.,-4.04029392228049));
#38444=CARTESIAN_POINT('Ctrl Pts',(0.454469363020541,-1.,-4.03289354362794));
#38445=CARTESIAN_POINT('Ctrl Pts',(0.45653407078495,-1.,-4.02549199038394));
#38446=CARTESIAN_POINT('Ctrl Pts',(0.458558885636945,-1.,-4.01808900827587));
#38447=CARTESIAN_POINT('Ctrl Pts',(0.460543280768514,-1.,-4.01068390573399));
#38448=CARTESIAN_POINT('Ctrl Pts',(0.462486702616204,-1.,-4.00327590659075));
#38449=CARTESIAN_POINT('Ctrl Pts',(0.464388610938975,-1.,-3.9958644432011));
#38450=CARTESIAN_POINT('Ctrl Pts',(0.466248520883039,-1.,-3.98844946363262));
#38451=CARTESIAN_POINT('Ctrl Pts',(0.468066047920157,-1.,-3.98103175589371));
#38452=CARTESIAN_POINT('Ctrl Pts',(0.469840942829895,-1.,-3.97361320212436));
#38453=CARTESIAN_POINT('Ctrl Pts',(0.471572978413503,-1.,-3.96619600864643));
#38454=CARTESIAN_POINT('Ctrl Pts',(0.473261847236297,-1.,-3.95878201038338));
#38455=CARTESIAN_POINT('Ctrl Pts',(0.47490705302179,-1.,-3.95137192932897));
#38456=CARTESIAN_POINT('Ctrl Pts',(0.476507810658537,-1.,-3.94396469119383));
#38457=CARTESIAN_POINT('Ctrl Pts',(0.478062927140964,-1.,-3.93655660689819));
#38458=CARTESIAN_POINT('Ctrl Pts',(0.479571028525578,-1.,-3.92914297392071));
#38459=CARTESIAN_POINT('Ctrl Pts',(0.481030798910748,-1.,-3.92171976072341));
#38460=CARTESIAN_POINT('Ctrl Pts',(0.482441230340713,-1.,-3.91428536373751));
#38461=CARTESIAN_POINT('Ctrl Pts',(0.48380183508915,-1.,-3.90684210358056));
#38462=CARTESIAN_POINT('Ctrl Pts',(0.485112963522222,-1.,-3.89939844658513));
#38463=CARTESIAN_POINT('Ctrl Pts',(0.486375337854103,-1.,-3.89196582437552));
#38464=CARTESIAN_POINT('Ctrl Pts',(0.487589452275154,-1.,-3.88455453328138));
#38465=CARTESIAN_POINT('Ctrl Pts',(0.488754973798273,-1.,-3.87716963231109));
#38466=CARTESIAN_POINT('Ctrl Pts',(0.489870245704917,-1.,-3.86980755613707));
#38467=CARTESIAN_POINT('Ctrl Pts',(0.490931482170891,-1.,-3.86245057319246));
#38468=CARTESIAN_POINT('Ctrl Pts',(0.491933631083813,-1.,-3.85507287020263));
#38469=CARTESIAN_POINT('Ctrl Pts',(0.49287179241414,-1.,-3.84765051147999));
#38470=CARTESIAN_POINT('Ctrl Pts',(0.493742574629134,-1.,-3.84017095578451));
#38471=CARTESIAN_POINT('Ctrl Pts',(0.494545212256401,-1.,-3.83264092682431));
#38472=CARTESIAN_POINT('Ctrl Pts',(0.495283458893837,-1.,-3.82509963594103));
#38473=CARTESIAN_POINT('Ctrl Pts',(0.495963937875479,-1.,-3.81760756144025));
#38474=CARTESIAN_POINT('Ctrl Pts',(0.496592643443704,-1.,-3.81022254090839));
#38475=CARTESIAN_POINT('Ctrl Pts',(0.497171756201051,-1.,-3.80297788298514));
#38476=CARTESIAN_POINT('Ctrl Pts',(0.497696892100624,-1.,-3.79586380669994));
#38477=CARTESIAN_POINT('Ctrl Pts',(0.498152751800958,-1.,-3.78879701661264));
#38478=CARTESIAN_POINT('Ctrl Pts',(0.498515471679584,-1.,-3.78163975337356));
#38479=CARTESIAN_POINT('Ctrl Pts',(0.498759900365891,-1.,-3.77425499225255));
#38480=CARTESIAN_POINT('Ctrl Pts',(0.49886579233529,-1.,-3.76655401191229));
#38481=CARTESIAN_POINT('Ctrl Pts',(0.498823681615421,-1.,-3.75854082221052));
#38482=CARTESIAN_POINT('Ctrl Pts',(0.498642802042605,-1.,-3.75037362167839));
#38483=CARTESIAN_POINT('Ctrl Pts',(0.498350586057692,-1.,-3.74235701734714));
#38484=CARTESIAN_POINT('Ctrl Pts',(0.497984209510024,-1.,-3.73486914372449));
#38485=CARTESIAN_POINT('Ctrl Pts',(0.497584067153049,-1.,-3.72830430904606));
#38486=CARTESIAN_POINT('Ctrl Pts',(0.497187079575988,-1.,-3.72301489774398));
#38487=CARTESIAN_POINT('Ctrl Pts',(0.496846224822563,-1.,-3.71952320822499));
#38488=CARTESIAN_POINT('Ctrl Pts',(0.496605651525989,-1.,-3.71785517607549));
#38489=CARTESIAN_POINT('Ctrl Pts',(0.496446644158005,-1.,-3.71721917030355));
#38490=CARTESIAN_POINT('Ctrl Pts',(0.496354087924312,-1.,-3.71704500630495));
#38491=CARTESIAN_POINT('Ctrl Pts',(0.496319364827592,-1.,-3.71701050416825));
#38492=CARTESIAN_POINT('',(0.676591647973661,-1.,-3.68845817949618));
#38493=CARTESIAN_POINT('Origin',(0.,-1.,0.));
#38494=CARTESIAN_POINT('',(0.906349047628866,-1.,-4.10104028313088));
#38495=CARTESIAN_POINT('Ctrl Pts',(0.676591647973661,-1.,-3.68845817949618));
#38496=CARTESIAN_POINT('Ctrl Pts',(0.67656928609342,-1.,-3.68850172300543));
#38497=CARTESIAN_POINT('Ctrl Pts',(0.676535079520365,-1.,-3.68869596426099));
#38498=CARTESIAN_POINT('Ctrl Pts',(0.676580391119535,-1.,-3.68934997767391));
#38499=CARTESIAN_POINT('Ctrl Pts',(0.676867042599711,-1.,-3.6910107117555));
#38500=CARTESIAN_POINT('Ctrl Pts',(0.677621861865196,-1.,-3.69443683573443));
#38501=CARTESIAN_POINT('Ctrl Pts',(0.678878822226389,-1.,-3.69959004073192));
#38502=CARTESIAN_POINT('Ctrl Pts',(0.680526909711617,-1.,-3.70595722032165));
#38503=CARTESIAN_POINT('Ctrl Pts',(0.682492345109689,-1.,-3.71319182790334));
#38504=CARTESIAN_POINT('Ctrl Pts',(0.684691698168355,-1.,-3.7209063713952));
#38505=CARTESIAN_POINT('Ctrl Pts',(0.687043475232499,-1.,-3.72872973554125));
#38506=CARTESIAN_POINT('Ctrl Pts',(0.689479637354651,-1.,-3.73636374474993));
#38507=CARTESIAN_POINT('Ctrl Pts',(0.691960080400503,-1.,-3.74365508986548));
#38508=CARTESIAN_POINT('Ctrl Pts',(0.694474562581173,-1.,-3.7506028824329));
#38509=CARTESIAN_POINT('Ctrl Pts',(0.69703124565953,-1.,-3.75729775766913));
#38510=CARTESIAN_POINT('Ctrl Pts',(0.699648552230851,-1.,-3.76387780603725));
#38511=CARTESIAN_POINT('Ctrl Pts',(0.702346356621613,-1.,-3.77048141872904));
#38512=CARTESIAN_POINT('Ctrl Pts',(0.705135847999949,-1.,-3.77719254217197));
#38513=CARTESIAN_POINT('Ctrl Pts',(0.7080158793756,-1.,-3.78402183336678));
#38514=CARTESIAN_POINT('Ctrl Pts',(0.710978231689117,-1.,-3.79093694007146));
#38515=CARTESIAN_POINT('Ctrl Pts',(0.714010733006677,-1.,-3.79788100314994));
#38516=CARTESIAN_POINT('Ctrl Pts',(0.717100993669091,-1.,-3.80479445759296));
#38517=CARTESIAN_POINT('Ctrl Pts',(0.720240466589172,-1.,-3.81163885127309));
#38518=CARTESIAN_POINT('Ctrl Pts',(0.723426346019349,-1.,-3.81840802610795));
#38519=CARTESIAN_POINT('Ctrl Pts',(0.726659281876608,-1.,-3.82511495756682));
#38520=CARTESIAN_POINT('Ctrl Pts',(0.729942010490145,-1.,-3.83178392403371));
#38521=CARTESIAN_POINT('Ctrl Pts',(0.73327770375609,-1.,-3.83844103658016));
#38522=CARTESIAN_POINT('Ctrl Pts',(0.736668240497151,-1.,-3.84510432881231));
#38523=CARTESIAN_POINT('Ctrl Pts',(0.740113146827176,-1.,-3.85177770351237));
#38524=CARTESIAN_POINT('Ctrl Pts',(0.743610542737041,-1.,-3.85845645217611));
#38525=CARTESIAN_POINT('Ctrl Pts',(0.747157716488884,-1.,-3.86513062969896));
#38526=CARTESIAN_POINT('Ctrl Pts',(0.750751822383023,-1.,-3.87178914078372));
#38527=CARTESIAN_POINT('Ctrl Pts',(0.754390577396846,-1.,-3.87842382520058));
#38528=CARTESIAN_POINT('Ctrl Pts',(0.758072800564798,-1.,-3.88503262662684));
#38529=CARTESIAN_POINT('Ctrl Pts',(0.761798028793978,-1.,-3.89161738162245));
#38530=CARTESIAN_POINT('Ctrl Pts',(0.765566256401306,-1.,-3.89818233104381));
#38531=CARTESIAN_POINT('Ctrl Pts',(0.769377629847876,-1.,-3.90473237182634));
#38532=CARTESIAN_POINT('Ctrl Pts',(0.773232154506305,-1.,-3.91127138115238));
#38533=CARTESIAN_POINT('Ctrl Pts',(0.777129415664915,-1.,-3.91780062334464));
#38534=CARTESIAN_POINT('Ctrl Pts',(0.781068718228395,-1.,-3.92431956510418));
#38535=CARTESIAN_POINT('Ctrl Pts',(0.785049202786458,-1.,-3.93082655631769));
#38536=CARTESIAN_POINT('Ctrl Pts',(0.789069971469323,-1.,-3.93731956885671));
#38537=CARTESIAN_POINT('Ctrl Pts',(0.793130205641017,-1.,-3.94379688971307));
#38538=CARTESIAN_POINT('Ctrl Pts',(0.797229296085438,-1.,-3.95025788827189));
#38539=CARTESIAN_POINT('Ctrl Pts',(0.801366797727206,-1.,-3.95670276375176));
#38540=CARTESIAN_POINT('Ctrl Pts',(0.805542372178495,-1.,-3.96313222295874));
#38541=CARTESIAN_POINT('Ctrl Pts',(0.809755732818134,-1.,-3.96954717513251));
#38542=CARTESIAN_POINT('Ctrl Pts',(0.814006592328737,-1.,-3.97594844078763));
#38543=CARTESIAN_POINT('Ctrl Pts',(0.818294599022033,-1.,-3.98233640155287));
#38544=CARTESIAN_POINT('Ctrl Pts',(0.822619346021769,-1.,-3.98871104646328));
#38545=CARTESIAN_POINT('Ctrl Pts',(0.826980400320473,-1.,-3.99507212784289));
#38546=CARTESIAN_POINT('Ctrl Pts',(0.831377325741487,-1.,-4.00141928477447));
#38547=CARTESIAN_POINT('Ctrl Pts',(0.835809705809821,-1.,-4.00775216907934));
#38548=CARTESIAN_POINT('Ctrl Pts',(0.84027717197638,-1.,-4.01407059766338));
#38549=CARTESIAN_POINT('Ctrl Pts',(0.844779403288517,-1.,-4.02037456798787));
#38550=CARTESIAN_POINT('Ctrl Pts',(0.849316107475012,-1.,-4.02666418343508));
#38551=CARTESIAN_POINT('Ctrl Pts',(0.853887006632178,-1.,-4.03293960436946));
#38552=CARTESIAN_POINT('Ctrl Pts',(0.858491822322571,-1.,-4.03920099284658));
#38553=CARTESIAN_POINT('Ctrl Pts',(0.863130256642173,-1.,-4.04544845048097));
#38554=CARTESIAN_POINT('Ctrl Pts',(0.867801988858176,-1.,-4.05168199437128));
#38555=CARTESIAN_POINT('Ctrl Pts',(0.872506694780563,-1.,-4.05790159030495));
#38556=CARTESIAN_POINT('Ctrl Pts',(0.877244060484595,-1.,-4.06410717232347));
#38557=CARTESIAN_POINT('Ctrl Pts',(0.882013797525916,-1.,-4.07029866694292));
#38558=CARTESIAN_POINT('Ctrl Pts',(0.886815658360739,-1.,-4.07647601774639));
#38559=CARTESIAN_POINT('Ctrl Pts',(0.891649447920401,-1.,-4.08263920306651));
#38560=CARTESIAN_POINT('Ctrl Pts',(0.896515019236368,-1.,-4.08878822249095));
#38561=CARTESIAN_POINT('Ctrl Pts',(0.900432820945975,-1.,-4.09369611524319));
#38562=CARTESIAN_POINT('Ctrl Pts',(0.903385402444212,-1.,-4.09737067247114));
#38563=CARTESIAN_POINT('Ctrl Pts',(0.905360112216302,-1.,-4.09981755067956));
#38564=CARTESIAN_POINT('Ctrl Pts',(0.906349047628866,-1.,-4.10104028313088));
#38565=CARTESIAN_POINT('',(1.05427041296137,-1.,-4.06552750530042));
#38566=CARTESIAN_POINT('',(0.906349047628866,-1.,-4.10104028313088));
#38567=CARTESIAN_POINT('',(1.07167739962028,-1.,-3.59360648251073));
#38568=CARTESIAN_POINT('Ctrl Pts',(1.05427041296137,-1.,-4.06552750530042));
#38569=CARTESIAN_POINT('Ctrl Pts',(1.05459645194823,-1.,-4.06398907542249));
#38570=CARTESIAN_POINT('Ctrl Pts',(1.05524507177599,-1.,-4.06091239149123));
#38571=CARTESIAN_POINT('Ctrl Pts',(1.05620762707996,-1.,-4.05629789307025));
#38572=CARTESIAN_POINT('Ctrl Pts',(1.05747027727959,-1.,-4.05014628384869));
#38573=CARTESIAN_POINT('Ctrl Pts',(1.05901393666566,-1.,-4.04245854427496));
#38574=CARTESIAN_POINT('Ctrl Pts',(1.06052284711857,-1.,-4.03477261141553));
#38575=CARTESIAN_POINT('Ctrl Pts',(1.06199687787462,-1.,-4.02708855235633));
#38576=CARTESIAN_POINT('Ctrl Pts',(1.06343586496236,-1.,-4.01940647495943));
#38577=CARTESIAN_POINT('Ctrl Pts',(1.06483961343109,-1.,-4.01172654187398));
#38578=CARTESIAN_POINT('Ctrl Pts',(1.06620789963606,-1.,-4.00404894952579));
#38579=CARTESIAN_POINT('Ctrl Pts',(1.06754047381312,-1.,-3.99637389920441));
#38580=CARTESIAN_POINT('Ctrl Pts',(1.06883706263941,-1.,-3.98870156857412));
#38581=CARTESIAN_POINT('Ctrl Pts',(1.07009737257767,-1.,-3.98103208801101));
#38582=CARTESIAN_POINT('Ctrl Pts',(1.07132109206164,-1.,-3.9733655022223));
#38583=CARTESIAN_POINT('Ctrl Pts',(1.07250789943007,-1.,-3.96570179322338));
#38584=CARTESIAN_POINT('Ctrl Pts',(1.07365747426491,-1.,-3.95804094429373));
#38585=CARTESIAN_POINT('Ctrl Pts',(1.07476950921587,-1.,-3.95038299600676));
#38586=CARTESIAN_POINT('Ctrl Pts',(1.07584371946443,-1.,-3.94272809633331));
#38587=CARTESIAN_POINT('Ctrl Pts',(1.07687985975384,-1.,-3.93507657572883));
#38588=CARTESIAN_POINT('Ctrl Pts',(1.07787771707195,-1.,-3.9274289334984));
#38589=CARTESIAN_POINT('Ctrl Pts',(1.07883706663554,-1.,-3.91978568924178));
#38590=CARTESIAN_POINT('Ctrl Pts',(1.07975763507473,-1.,-3.91214726022143));
#38591=CARTESIAN_POINT('Ctrl Pts',(1.08063906483818,-1.,-3.90451384092545));
#38592=CARTESIAN_POINT('Ctrl Pts',(1.08148086931358,-1.,-3.8968852509835));
#38593=CARTESIAN_POINT('Ctrl Pts',(1.08228241999346,-1.,-3.88926088975114));
#38594=CARTESIAN_POINT('Ctrl Pts',(1.08304304871028,-1.,-3.88164007721313));
#38595=CARTESIAN_POINT('Ctrl Pts',(1.08376213307504,-1.,-3.8740223372254));
#38596=CARTESIAN_POINT('Ctrl Pts',(1.08443918607927,-1.,-3.86640769434274));
#38597=CARTESIAN_POINT('Ctrl Pts',(1.08507395120059,-1.,-3.85879698702532));
#38598=CARTESIAN_POINT('Ctrl Pts',(1.08566647671844,-1.,-3.85119211322755));
#38599=CARTESIAN_POINT('Ctrl Pts',(1.08621688337604,-1.,-3.8435952876495));
#38600=CARTESIAN_POINT('Ctrl Pts',(1.08672515456902,-1.,-3.83600837071708));
#38601=CARTESIAN_POINT('Ctrl Pts',(1.08719091307558,-1.,-3.82843215316984));
#38602=CARTESIAN_POINT('Ctrl Pts',(1.08761321539442,-1.,-3.82086569676319));
#38603=CARTESIAN_POINT('Ctrl Pts',(1.08799030610862,-1.,-3.81330554446323));
#38604=CARTESIAN_POINT('Ctrl Pts',(1.0883200925538,-1.,-3.8057472665766));
#38605=CARTESIAN_POINT('Ctrl Pts',(1.08860064435778,-1.,-3.79818708705259));
#38606=CARTESIAN_POINT('Ctrl Pts',(1.08883071512098,-1.,-3.79062357974404));
#38607=CARTESIAN_POINT('Ctrl Pts',(1.08901018614636,-1.,-3.78305911299504));
#38608=CARTESIAN_POINT('Ctrl Pts',(1.0891407279127,-1.,-3.77550199409424));
#38609=CARTESIAN_POINT('Ctrl Pts',(1.08922484204256,-1.,-3.76796340094448));
#38610=CARTESIAN_POINT('Ctrl Pts',(1.08926462734281,-1.,-3.76045342580208));
#38611=CARTESIAN_POINT('Ctrl Pts',(1.08926054632925,-1.,-3.75297711748132));
#38612=CARTESIAN_POINT('Ctrl Pts',(1.08921040494017,-1.,-3.74553121371757));
#38613=CARTESIAN_POINT('Ctrl Pts',(1.08910769013297,-1.,-3.73809879348239));
#38614=CARTESIAN_POINT('Ctrl Pts',(1.08894337390937,-1.,-3.73065515162988));
#38615=CARTESIAN_POINT('Ctrl Pts',(1.08870887220082,-1.,-3.72317741369398));
#38616=CARTESIAN_POINT('Ctrl Pts',(1.0883988733478,-1.,-3.71565372339075));
#38617=CARTESIAN_POINT('Ctrl Pts',(1.08801367312185,-1.,-3.70809084139457));
#38618=CARTESIAN_POINT('Ctrl Pts',(1.08756311291309,-1.,-3.70052690909833));
#38619=CARTESIAN_POINT('Ctrl Pts',(1.08706319540271,-1.,-3.69302062410157));
#38620=CARTESIAN_POINT('Ctrl Pts',(1.0865288888259,-1.,-3.68562817420797));
#38621=CARTESIAN_POINT('Ctrl Pts',(1.0859675575576,-1.,-3.67838211685118));
#38622=CARTESIAN_POINT('Ctrl Pts',(1.0853733414449,-1.,-3.67127347729666));
#38623=CARTESIAN_POINT('Ctrl Pts',(1.08471809922901,-1.,-3.66422237895365));
#38624=CARTESIAN_POINT('Ctrl Pts',(1.08395671077807,-1.,-3.65709649161166));
#38625=CARTESIAN_POINT('Ctrl Pts',(1.08304289898623,-1.,-3.64976441208358));
#38626=CARTESIAN_POINT('Ctrl Pts',(1.08194278850996,-1.,-3.64214167843677));
#38627=CARTESIAN_POINT('Ctrl Pts',(1.08064765719867,-1.,-3.63423373196529));
#38628=CARTESIAN_POINT('Ctrl Pts',(1.07919137290742,-1.,-3.62619537902361));
#38629=CARTESIAN_POINT('Ctrl Pts',(1.07764868137619,-1.,-3.61832318504575));
#38630=CARTESIAN_POINT('Ctrl Pts',(1.07611545402734,-1.,-3.61098481349204));
#38631=CARTESIAN_POINT('Ctrl Pts',(1.07469327168578,-1.,-3.60456339887778));
#38632=CARTESIAN_POINT('Ctrl Pts',(1.07347372545714,-1.,-3.59940121154535));
#38633=CARTESIAN_POINT('Ctrl Pts',(1.07259084660935,-1.,-3.59600583194946));
#38634=CARTESIAN_POINT('Ctrl Pts',(1.07209229745229,-1.,-3.59439596999862));
#38635=CARTESIAN_POINT('Ctrl Pts',(1.07183575450617,-1.,-3.59379266874567));
#38636=CARTESIAN_POINT('Ctrl Pts',(1.07171709254135,-1.,-3.5936351279798));
#38637=CARTESIAN_POINT('Ctrl Pts',(1.07167739962028,-1.,-3.59360648251073));
#38638=CARTESIAN_POINT('',(1.24526366418038,-1.,-3.5372048861597));
#38639=CARTESIAN_POINT('Origin',(0.,-1.,0.));
#38640=CARTESIAN_POINT('',(1.53673442965256,-1.,-3.90876544355381));
#38641=CARTESIAN_POINT('Ctrl Pts',(1.24526366418038,-1.,-3.5372048861597));
#38642=CARTESIAN_POINT('Ctrl Pts',(1.24524838931757,-1.,-3.53725139174486));
#38643=CARTESIAN_POINT('Ctrl Pts',(1.2452449899111,-1.,-3.5374485926552));
#38644=CARTESIAN_POINT('Ctrl Pts',(1.24539205388767,-1.,-3.53808746578196));
#38645=CARTESIAN_POINT('Ctrl Pts',(1.24593497226008,-1.,-3.53968291130022));
#38646=CARTESIAN_POINT('Ctrl Pts',(1.24721646231966,-1.,-3.54294877425964));
#38647=CARTESIAN_POINT('Ctrl Pts',(1.24926408628003,-1.,-3.54784190283068));
#38648=CARTESIAN_POINT('Ctrl Pts',(1.2518879294064,-1.,-3.55387287418985));
#38649=CARTESIAN_POINT('Ctrl Pts',(1.25496090900009,-1.,-3.56071094991199));
#38650=CARTESIAN_POINT('Ctrl Pts',(1.25834000485716,-1.,-3.56798645995275));
#38651=CARTESIAN_POINT('Ctrl Pts',(1.2618866714281,-1.,-3.5753456065171));
#38652=CARTESIAN_POINT('Ctrl Pts',(1.26548706249862,-1.,-3.58250452868618));
#38653=CARTESIAN_POINT('Ctrl Pts',(1.26907758484709,-1.,-3.58931807846313));
#38654=CARTESIAN_POINT('Ctrl Pts',(1.27264798379307,-1.,-3.59578698050006));
#38655=CARTESIAN_POINT('Ctrl Pts',(1.27622049908625,-1.,-3.60199947736298));
#38656=CARTESIAN_POINT('Ctrl Pts',(1.27983492861691,-1.,-3.60808907746339));
#38657=CARTESIAN_POINT('Ctrl Pts',(1.28353255117765,-1.,-3.61418935913823));
#38658=CARTESIAN_POINT('Ctrl Pts',(1.28733755029384,-1.,-3.6203814849236));
#38659=CARTESIAN_POINT('Ctrl Pts',(1.29125046021878,-1.,-3.62667616004369));
#38660=CARTESIAN_POINT('Ctrl Pts',(1.29525810207762,-1.,-3.63304271631046));
#38661=CARTESIAN_POINT('Ctrl Pts',(1.2993395590647,-1.,-3.63942689872808));
#38662=CARTESIAN_POINT('Ctrl Pts',(1.30347327603774,-1.,-3.64577181380113));
#38663=CARTESIAN_POINT('Ctrl Pts',(1.30764479590039,-1.,-3.65204081987068));
#38664=CARTESIAN_POINT('Ctrl Pts',(1.31185038411218,-1.,-3.65822827358617));
#38665=CARTESIAN_POINT('Ctrl Pts',(1.31609271239911,-1.,-3.66434688899793));
#38666=CARTESIAN_POINT('Ctrl Pts',(1.32037828137766,-1.,-3.67042021752656));
#38667=CARTESIAN_POINT('Ctrl Pts',(1.32471430856415,-1.,-3.67647355257912));
#38668=CARTESIAN_POINT('Ctrl Pts',(1.3291054707274,-1.,-3.68252441182551));
#38669=CARTESIAN_POINT('Ctrl Pts',(1.33355191034523,-1.,-3.68857672413033));
#38670=CARTESIAN_POINT('Ctrl Pts',(1.33805103398219,-1.,-3.69462613305708));
#38671=CARTESIAN_POINT('Ctrl Pts',(1.34259860752933,-1.,-3.70066324015119));
#38672=CARTESIAN_POINT('Ctrl Pts',(1.34719008463534,-1.,-3.70667753188248));
#38673=CARTESIAN_POINT('Ctrl Pts',(1.35182193384424,-1.,-3.71266130563054));
#38674=CARTESIAN_POINT('Ctrl Pts',(1.35649266705037,-1.,-3.71861271513313));
#38675=CARTESIAN_POINT('Ctrl Pts',(1.36120211416354,-1.,-3.72453364678279));
#38676=CARTESIAN_POINT('Ctrl Pts',(1.36595093298676,-1.,-3.73042829011295));
#38677=CARTESIAN_POINT('Ctrl Pts',(1.37074003422739,-1.,-3.7363014588581));
#38678=CARTESIAN_POINT('Ctrl Pts',(1.37557002971687,-1.,-3.74215698162555));
#38679=CARTESIAN_POINT('Ctrl Pts',(1.38044070763295,-1.,-3.74799617204729));
#38680=CARTESIAN_POINT('Ctrl Pts',(1.38535129801176,-1.,-3.75381861212707));
#38681=CARTESIAN_POINT('Ctrl Pts',(1.39030069388918,-1.,-3.75962280650855));
#38682=CARTESIAN_POINT('Ctrl Pts',(1.39528769118052,-1.,-3.76540689249074));
#38683=CARTESIAN_POINT('Ctrl Pts',(1.40031121335505,-1.,-3.77116930621827));
#38684=CARTESIAN_POINT('Ctrl Pts',(1.40537056004722,-1.,-3.77690952014259));
#38685=CARTESIAN_POINT('Ctrl Pts',(1.41046532282593,-1.,-3.78262780065471));
#38686=CARTESIAN_POINT('Ctrl Pts',(1.4155952780383,-1.,-3.78832489879426));
#38687=CARTESIAN_POINT('Ctrl Pts',(1.42076028482836,-1.,-3.79400175744408));
#38688=CARTESIAN_POINT('Ctrl Pts',(1.42596018777283,-1.,-3.7996592319632));
#38689=CARTESIAN_POINT('Ctrl Pts',(1.4311946992132,-1.,-3.80529775429805));
#38690=CARTESIAN_POINT('Ctrl Pts',(1.43646341556724,-1.,-3.81091737726815));
#38691=CARTESIAN_POINT('Ctrl Pts',(1.44176587041347,-1.,-3.81651792398414));
#38692=CARTESIAN_POINT('Ctrl Pts',(1.44710157648539,-1.,-3.82209910620533));
#38693=CARTESIAN_POINT('Ctrl Pts',(1.45247006796836,-1.,-3.82766064519075));
#38694=CARTESIAN_POINT('Ctrl Pts',(1.45787095220852,-1.,-3.83320241775423));
#38695=CARTESIAN_POINT('Ctrl Pts',(1.46330391180752,-1.,-3.83872447159639));
#38696=CARTESIAN_POINT('Ctrl Pts',(1.46876867426504,-1.,-3.84422695454796));
#38697=CARTESIAN_POINT('Ctrl Pts',(1.47426499018538,-1.,-3.84971006847277));
#38698=CARTESIAN_POINT('Ctrl Pts',(1.4797926099102,-1.,-3.85517401698843));
#38699=CARTESIAN_POINT('Ctrl Pts',(1.48535125509919,-1.,-3.86061894706087));
#38700=CARTESIAN_POINT('Ctrl Pts',(1.4909406116431,-1.,-3.86604492575189));
#38701=CARTESIAN_POINT('Ctrl Pts',(1.49656035399122,-1.,-3.87145196998465));
#38702=CARTESIAN_POINT('Ctrl Pts',(1.50221016176556,-1.,-3.87684006372134));
#38703=CARTESIAN_POINT('Ctrl Pts',(1.50788973857757,-1.,-3.88220917950538));
#38704=CARTESIAN_POINT('Ctrl Pts',(1.51359883110559,-1.,-3.88755930033884));
#38705=CARTESIAN_POINT('Ctrl Pts',(1.51933724329305,-1.,-3.89289043533657));
#38706=CARTESIAN_POINT('Ctrl Pts',(1.52510482991635,-1.,-3.89820260708225));
#38707=CARTESIAN_POINT('Ctrl Pts',(1.52974216056287,-1.,-3.90243719631596));
#38708=CARTESIAN_POINT('Ctrl Pts',(1.53323321827755,-1.,-3.90560462813969));
#38709=CARTESIAN_POINT('Ctrl Pts',(1.53556639217905,-1.,-3.90771246855019));
#38710=CARTESIAN_POINT('Ctrl Pts',(1.53673442965256,-1.,-3.90876544355381));
#38711=CARTESIAN_POINT('',(1.67727921511438,-1.,-3.85054988729471));
#38712=CARTESIAN_POINT('',(1.53673442965256,-1.,-3.90876544355381));
#38713=CARTESIAN_POINT('',(1.62064718014093,-1.,-3.38171594275765));
#38714=CARTESIAN_POINT('Ctrl Pts',(1.67727921511438,-1.,-3.85054988729471));
#38715=CARTESIAN_POINT('Ctrl Pts',(1.67736057656533,-1.,-3.84897939430696));
#38716=CARTESIAN_POINT('Ctrl Pts',(1.6775199114018,-1.,-3.84583912296459));
#38717=CARTESIAN_POINT('Ctrl Pts',(1.67774874946079,-1.,-3.84113085985244));
#38718=CARTESIAN_POINT('Ctrl Pts',(1.67803353064351,-1.,-3.8348574651399));
#38719=CARTESIAN_POINT('Ctrl Pts',(1.6783555575934,-1.,-3.82702289286713));
#38720=CARTESIAN_POINT('Ctrl Pts',(1.67864354605954,-1.,-3.81919554099578));
#38721=CARTESIAN_POINT('Ctrl Pts',(1.6788973773827,-1.,-3.81137549624179));
#38722=CARTESIAN_POINT('Ctrl Pts',(1.67911690648355,-1.,-3.80356289079005));
#38723=CARTESIAN_POINT('Ctrl Pts',(1.67930196625548,-1.,-3.79575791578424));
#38724=CARTESIAN_POINT('Ctrl Pts',(1.67945236653493,-1.,-3.7879608002176));
#38725=CARTESIAN_POINT('Ctrl Pts',(1.67956789212141,-1.,-3.78017178197317));
#38726=CARTESIAN_POINT('Ctrl Pts',(1.67964830084993,-1.,-3.77239107928502));
#38727=CARTESIAN_POINT('Ctrl Pts',(1.67969332319245,-1.,-3.76461886684344));
#38728=CARTESIAN_POINT('Ctrl Pts',(1.67970265841239,-1.,-3.75685523754493));
#38729=CARTESIAN_POINT('Ctrl Pts',(1.67967598599525,-1.,-3.7491002239452));
#38730=CARTESIAN_POINT('Ctrl Pts',(1.6796129868522,-1.,-3.74135385965401));
#38731=CARTESIAN_POINT('Ctrl Pts',(1.67951336376402,-1.,-3.73361623282543));
#38732=CARTESIAN_POINT('Ctrl Pts',(1.67937685856652,-1.,-3.72588753416396));
#38733=CARTESIAN_POINT('Ctrl Pts',(1.67920328071708,-1.,-3.71816812842322));
#38734=CARTESIAN_POINT('Ctrl Pts',(1.67899249793462,-1.,-3.71045854208343));
#38735=CARTESIAN_POINT('Ctrl Pts',(1.67874436948667,-1.,-3.70275932351108));
#38736=CARTESIAN_POINT('Ctrl Pts',(1.67845869064323,-1.,-3.6950709275959));
#38737=CARTESIAN_POINT('Ctrl Pts',(1.67813513867965,-1.,-3.68739360236487));
#38738=CARTESIAN_POINT('Ctrl Pts',(1.67777320475848,-1.,-3.67972724579124));
#38739=CARTESIAN_POINT('Ctrl Pts',(1.67737217414874,-1.,-3.67207136294575));
#38740=CARTESIAN_POINT('Ctrl Pts',(1.67693128053132,-1.,-3.66442538670968));
#38741=CARTESIAN_POINT('Ctrl Pts',(1.67644983469449,-1.,-3.6567889441642));
#38742=CARTESIAN_POINT('Ctrl Pts',(1.67592735946692,-1.,-3.64916213574667));
#38743=CARTESIAN_POINT('Ctrl Pts',(1.67536373264848,-1.,-3.6415458297234));
#38744=CARTESIAN_POINT('Ctrl Pts',(1.67475929882971,-1.,-3.63394189312924));
#38745=CARTESIAN_POINT('Ctrl Pts',(1.67411452372271,-1.,-3.62635249450923));
#38746=CARTESIAN_POINT('Ctrl Pts',(1.67342968196224,-1.,-3.61877947398184));
#38747=CARTESIAN_POINT('Ctrl Pts',(1.67270452466968,-1.,-3.61122367156181));
#38748=CARTESIAN_POINT('Ctrl Pts',(1.67193797318597,-1.,-3.60368430815201));
#38749=CARTESIAN_POINT('Ctrl Pts',(1.67112775290707,-1.,-3.59615824388807));
#38750=CARTESIAN_POINT('Ctrl Pts',(1.67027110397604,-1.,-3.58864143097834));
#38751=CARTESIAN_POINT('Ctrl Pts',(1.66936552908232,-1.,-3.58113044183829));
#38752=CARTESIAN_POINT('Ctrl Pts',(1.668409574073,-1.,-3.57362406285887));
#38753=CARTESIAN_POINT('Ctrl Pts',(1.66740349220305,-1.,-3.56612465179422));
#38754=CARTESIAN_POINT('Ctrl Pts',(1.66635023293114,-1.,-3.55864015233602));
#38755=CARTESIAN_POINT('Ctrl Pts',(1.66525401568994,-1.,-3.55118121342861));
#38756=CARTESIAN_POINT('Ctrl Pts',(1.66411849222326,-1.,-3.54375747475014));
#38757=CARTESIAN_POINT('Ctrl Pts',(1.66294490916111,-1.,-3.5363738506022));
#38758=CARTESIAN_POINT('Ctrl Pts',(1.66173058912371,-1.,-3.52902746211093));
#38759=CARTESIAN_POINT('Ctrl Pts',(1.66046645222279,-1.,-3.52170261543816));
#38760=CARTESIAN_POINT('Ctrl Pts',(1.65913971687342,-1.,-3.5143763218894));
#38761=CARTESIAN_POINT('Ctrl Pts',(1.65773832633632,-1.,-3.50702733146542));
#38762=CARTESIAN_POINT('Ctrl Pts',(1.65625517961588,-1.,-3.4996447647794));
#38763=CARTESIAN_POINT('Ctrl Pts',(1.65469162644468,-1.,-3.49223525300176));
#38764=CARTESIAN_POINT('Ctrl Pts',(1.65306335367739,-1.,-3.48483492840894));
#38765=CARTESIAN_POINT('Ctrl Pts',(1.65139534930322,-1.,-3.47749926256476));
#38766=CARTESIAN_POINT('Ctrl Pts',(1.64971118698256,-1.,-3.47028140995992));
#38767=CARTESIAN_POINT('Ctrl Pts',(1.64802323352738,-1.,-3.46321237515));
#38768=CARTESIAN_POINT('Ctrl Pts',(1.64632429697521,-1.,-3.45628421062422));
#38769=CARTESIAN_POINT('Ctrl Pts',(1.64457408708107,-1.,-3.44942242546795));
#38770=CARTESIAN_POINT('Ctrl Pts',(1.64270733821113,-1.,-3.44250337701888));
#38771=CARTESIAN_POINT('Ctrl Pts',(1.64065778702023,-1.,-3.43540451921548));
#38772=CARTESIAN_POINT('Ctrl Pts',(1.63837876246926,-1.,-3.42804772926291));
#38773=CARTESIAN_POINT('Ctrl Pts',(1.63586250099773,-1.,-3.42043974590882));
#38774=CARTESIAN_POINT('Ctrl Pts',(1.63316667054044,-1.,-3.41272817148478));
#38775=CARTESIAN_POINT('Ctrl Pts',(1.63041148964828,-1.,-3.40519422740235));
#38776=CARTESIAN_POINT('Ctrl Pts',(1.62774916464408,-1.,-3.39818605297991));
#38777=CARTESIAN_POINT('Ctrl Pts',(1.62533996116713,-1.,-3.39206617496906));
#38778=CARTESIAN_POINT('Ctrl Pts',(1.6233278855625,-1.,-3.38715832179072));
#38779=CARTESIAN_POINT('Ctrl Pts',(1.62192472202769,-1.,-3.38394285763222));
#38780=CARTESIAN_POINT('Ctrl Pts',(1.62118047294498,-1.,-3.38243080602408));
#38781=CARTESIAN_POINT('Ctrl Pts',(1.62083271135947,-1.,-3.38187506456922));
#38782=CARTESIAN_POINT('Ctrl Pts',(1.62069086551492,-1.,-3.38173802621259));
#38783=CARTESIAN_POINT('Ctrl Pts',(1.62064718014093,-1.,-3.38171594275765));
#38784=CARTESIAN_POINT('',(1.78327315618183,-1.,-3.29885386921599));
#38785=CARTESIAN_POINT('Origin',(0.,-1.,0.));
#38786=CARTESIAN_POINT('',(2.12928030988903,-1.,-3.62024382630768));
#38787=CARTESIAN_POINT('Ctrl Pts',(1.78327315618183,-1.,-3.29885386921599));
#38788=CARTESIAN_POINT('Ctrl Pts',(1.78326534445426,-1.,-3.29890219175522));
#38789=CARTESIAN_POINT('Ctrl Pts',(1.78329283591903,-1.,-3.29909749657945));
#38790=CARTESIAN_POINT('Ctrl Pts',(1.78353803106983,-1.,-3.29970549824337));
#38791=CARTESIAN_POINT('Ctrl Pts',(1.7843238478823,-1.,-3.30119637003466));
#38792=CARTESIAN_POINT('Ctrl Pts',(1.78610045419769,-1.,-3.30422155558973));
#38793=CARTESIAN_POINT('Ctrl Pts',(1.78888832245965,-1.,-3.30873412266954));
#38794=CARTESIAN_POINT('Ctrl Pts',(1.79242331350137,-1.,-3.31428038326763));
#38795=CARTESIAN_POINT('Ctrl Pts',(1.79652817033444,-1.,-3.32055355101168));
#38796=CARTESIAN_POINT('Ctrl Pts',(1.80100380443535,-1.,-3.3272108803981));
#38797=CARTESIAN_POINT('Ctrl Pts',(1.80565802981138,-1.,-3.33392460276874));
#38798=CARTESIAN_POINT('Ctrl Pts',(1.81033399625311,-1.,-3.34043216147532));
#38799=CARTESIAN_POINT('Ctrl Pts',(1.81494618732772,-1.,-3.34660014370527));
#38800=CARTESIAN_POINT('Ctrl Pts',(1.81948458796748,-1.,-3.35243086937451));
#38801=CARTESIAN_POINT('Ctrl Pts',(1.82398496829247,-1.,-3.35800801557326));
#38802=CARTESIAN_POINT('Ctrl Pts',(1.82850752153182,-1.,-3.36345722124127));
#38803=CARTESIAN_POINT('Ctrl Pts',(1.83311391452338,-1.,-3.36890396271864));
#38804=CARTESIAN_POINT('Ctrl Pts',(1.83784072967111,-1.,-3.37442462015914));
#38805=CARTESIAN_POINT('Ctrl Pts',(1.84269016931679,-1.,-3.38002968341222));
#38806=CARTESIAN_POINT('Ctrl Pts',(1.84764441927778,-1.,-3.38569092349639));
#38807=CARTESIAN_POINT('Ctrl Pts',(1.85267433291778,-1.,-3.39135802549415));
#38808=CARTESIAN_POINT('Ctrl Pts',(1.85774972037055,-1.,-3.39697816833056));
#38809=CARTESIAN_POINT('Ctrl Pts',(1.86285057051228,-1.,-3.40251742305445));
#38810=CARTESIAN_POINT('Ctrl Pts',(1.86797231196635,-1.,-3.40797080000513));
#38811=CARTESIAN_POINT('Ctrl Pts',(1.87311957248106,-1.,-3.41335043875182));
#38812=CARTESIAN_POINT('Ctrl Pts',(1.87830245689338,-1.,-3.4186785838376));
#38813=CARTESIAN_POINT('Ctrl Pts',(1.88353205062063,-1.,-3.42397908819741));
#38814=CARTESIAN_POINT('Ctrl Pts',(1.88881571322018,-1.,-3.42926852222174));
#38815=CARTESIAN_POINT('Ctrl Pts',(1.89415420002553,-1.,-3.43455074411591));
#38816=CARTESIAN_POINT('Ctrl Pts',(1.89954426803392,-1.,-3.43982185678105));
#38817=CARTESIAN_POINT('Ctrl Pts',(1.90498026502308,-1.,-3.44507323983374));
#38818=CARTESIAN_POINT('Ctrl Pts',(1.91045605593638,-1.,-3.45029522038885));
#38819=CARTESIAN_POINT('Ctrl Pts',(1.9159669478406,-1.,-3.45548074309943));
#38820=CARTESIAN_POINT('Ctrl Pts',(1.9215111821321,-1.,-3.4606282172248));
#38821=CARTESIAN_POINT('Ctrl Pts',(1.92708888591159,-1.,-3.46573953254084));
#38822=CARTESIAN_POINT('Ctrl Pts',(1.93270136427083,-1.,-3.47081872409783));
#38823=CARTESIAN_POINT('Ctrl Pts',(1.93835026973888,-1.,-3.47587040389916));
#38824=CARTESIAN_POINT('Ctrl Pts',(1.94403680554062,-1.,-3.48089825770412));
#38825=CARTESIAN_POINT('Ctrl Pts',(1.94976096795902,-1.,-3.485903616108));
#38826=CARTESIAN_POINT('Ctrl Pts',(1.95552193112071,-1.,-3.49088618670967));
#38827=CARTESIAN_POINT('Ctrl Pts',(1.96131836776489,-1.,-3.49584466573045));
#38828=CARTESIAN_POINT('Ctrl Pts',(1.9671487972405,-1.,-3.50077740176262));
#38829=CARTESIAN_POINT('Ctrl Pts',(1.9730119116298,-1.,-3.505683018611));
#38830=CARTESIAN_POINT('Ctrl Pts',(1.97890693666316,-1.,-3.51056110478334));
#38831=CARTESIAN_POINT('Ctrl Pts',(1.98483351061066,-1.,-3.51541198728362));
#38832=CARTESIAN_POINT('Ctrl Pts',(1.99079153006143,-1.,-3.52023644289195));
#38833=CARTESIAN_POINT('Ctrl Pts',(1.99678100339305,-1.,-3.52503542491745));
#38834=CARTESIAN_POINT('Ctrl Pts',(2.00280191090341,-1.,-3.52980980250181));
#38835=CARTESIAN_POINT('Ctrl Pts',(2.00885403604685,-1.,-3.53456004727321));
#38836=CARTESIAN_POINT('Ctrl Pts',(2.0149369884727,-1.,-3.53928627453503));
#38837=CARTESIAN_POINT('Ctrl Pts',(2.0210502798303,-1.,-3.54398838254011));
#38838=CARTESIAN_POINT('Ctrl Pts',(2.02719338376144,-1.,-3.54866616282173));
#38839=CARTESIAN_POINT('Ctrl Pts',(2.03336579658174,-1.,-3.55331941294018));
#38840=CARTESIAN_POINT('Ctrl Pts',(2.03956711120099,-1.,-3.55794807265052));
#38841=CARTESIAN_POINT('Ctrl Pts',(2.04579702159056,-1.,-3.5625522387181));
#38842=CARTESIAN_POINT('Ctrl Pts',(2.0520552817309,-1.,-3.56713209978208));
#38843=CARTESIAN_POINT('Ctrl Pts',(2.05834167687523,-1.,-3.57168789423507));
#38844=CARTESIAN_POINT('Ctrl Pts',(2.06465599229174,-1.,-3.576219862243));
#38845=CARTESIAN_POINT('Ctrl Pts',(2.07099797605747,-1.,-3.58072819250442));
#38846=CARTESIAN_POINT('Ctrl Pts',(2.07736732842117,-1.,-3.58521300039299));
#38847=CARTESIAN_POINT('Ctrl Pts',(2.08376373048756,-1.,-3.58967435355088));
#38848=CARTESIAN_POINT('Ctrl Pts',(2.09018686331416,-1.,-3.59411228625588));
#38849=CARTESIAN_POINT('Ctrl Pts',(2.09663642986631,-1.,-3.59852681775485));
#38850=CARTESIAN_POINT('Ctrl Pts',(2.1031121772821,-1.,-3.60291797088734));
#38851=CARTESIAN_POINT('Ctrl Pts',(2.10961391334462,-1.,-3.60728578532601));
#38852=CARTESIAN_POINT('Ctrl Pts',(2.11614149815106,-1.,-3.61163030609447));
#38853=CARTESIAN_POINT('Ctrl Pts',(2.12138417126355,-1.,-3.61508732216891));
#38854=CARTESIAN_POINT('Ctrl Pts',(2.12532774376758,-1.,-3.61766963590482));
#38855=CARTESIAN_POINT('Ctrl Pts',(2.12796193131368,-1.,-3.61938653649098));
#38856=CARTESIAN_POINT('Ctrl Pts',(2.12928030988903,-1.,-3.62024382630768));
#38857=CARTESIAN_POINT('',(2.25898783642071,-1.,-3.54075895182139));
#38858=CARTESIAN_POINT('',(2.12928030988903,-1.,-3.62024382630768));
#38859=CARTESIAN_POINT('',(2.1297112484669,-1.,-3.08655633322212));
#38860=CARTESIAN_POINT('Ctrl Pts',(2.25898783642071,-1.,-3.54075895182139));
#38861=CARTESIAN_POINT('Ctrl Pts',(2.2588225169468,-1.,-3.53919506647335));
#38862=CARTESIAN_POINT('Ctrl Pts',(2.25848864343951,-1.,-3.53606853162228));
#38863=CARTESIAN_POINT('Ctrl Pts',(2.25797812950104,-1.,-3.53138243688262));
#38864=CARTESIAN_POINT('Ctrl Pts',(2.25727802940898,-1.,-3.52514172847711));
#38865=CARTESIAN_POINT('Ctrl Pts',(2.25637049455044,-1.,-3.51735323667612));
#38866=CARTESIAN_POINT('Ctrl Pts',(2.25543046979799,-1.,-3.50957720117341));
#38867=CARTESIAN_POINT('Ctrl Pts',(2.25445785151868,-1.,-3.50181372617971));
#38868=CARTESIAN_POINT('Ctrl Pts',(2.25345251709759,-1.,-3.49406296494791));
#38869=CARTESIAN_POINT('Ctrl Pts',(2.25241433138695,-1.,-3.48632513240961));
#38870=CARTESIAN_POINT('Ctrl Pts',(2.25134314238687,-1.,-3.47860048448691));
#38871=CARTESIAN_POINT('Ctrl Pts',(2.25023877475942,-1.,-3.47088928979889));
#38872=CARTESIAN_POINT('Ctrl Pts',(2.2491010234604,-1.,-3.46319180177573));
#38873=CARTESIAN_POINT('Ctrl Pts',(2.2479296496077,-1.,-3.45550823512049));
#38874=CARTESIAN_POINT('Ctrl Pts',(2.2467243706995,-1.,-3.44783872863151));
#38875=CARTESIAN_POINT('Ctrl Pts',(2.24548487526022,-1.,-3.4401833646032));
#38876=CARTESIAN_POINT('Ctrl Pts',(2.24421085338727,-1.,-3.43254222614803));
#38877=CARTESIAN_POINT('Ctrl Pts',(2.24290202531101,-1.,-3.42491544683008));
#38878=CARTESIAN_POINT('Ctrl Pts',(2.24155816587844,-1.,-3.41730325539172));
#38879=CARTESIAN_POINT('Ctrl Pts',(2.24017914395289,-1.,-3.40970604190328));
#38880=CARTESIAN_POINT('Ctrl Pts',(2.2387649112415,-1.,-3.40212434705647));
#38881=CARTESIAN_POINT('Ctrl Pts',(2.23731541452791,-1.,-3.39455873448189));
#38882=CARTESIAN_POINT('Ctrl Pts',(2.23583052276308,-1.,-3.38700968549563));
#38883=CARTESIAN_POINT('Ctrl Pts',(2.23430995599561,-1.,-3.37947749555632));
#38884=CARTESIAN_POINT('Ctrl Pts',(2.23275319569221,-1.,-3.37196214349304));
#38885=CARTESIAN_POINT('Ctrl Pts',(2.23115945849739,-1.,-3.36446325227848));
#38886=CARTESIAN_POINT('Ctrl Pts',(2.22952789880982,-1.,-3.35698038165483));
#38887=CARTESIAN_POINT('Ctrl Pts',(2.22785777756576,-1.,-3.34951327111096));
#38888=CARTESIAN_POINT('Ctrl Pts',(2.22614863918047,-1.,-3.34206209449375));
#38889=CARTESIAN_POINT('Ctrl Pts',(2.22440049878511,-1.,-3.33462772849598));
#38890=CARTESIAN_POINT('Ctrl Pts',(2.22261398879635,-1.,-3.3272119632604));
#38891=CARTESIAN_POINT('Ctrl Pts',(2.22078990842776,-1.,-3.31981686778022));
#38892=CARTESIAN_POINT('Ctrl Pts',(2.21892881679086,-1.,-3.31244421655666));
#38893=CARTESIAN_POINT('Ctrl Pts',(2.21703059947836,-1.,-3.30509487819569));
#38894=CARTESIAN_POINT('Ctrl Pts',(2.21509406923368,-1.,-3.29776825193159));
#38895=CARTESIAN_POINT('Ctrl Pts',(2.21311648827391,-1.,-3.29046159238343));
#38896=CARTESIAN_POINT('Ctrl Pts',(2.21109449750641,-1.,-3.28317133333131));
#38897=CARTESIAN_POINT('Ctrl Pts',(2.2090250941743,-1.,-3.2758944800554));
#38898=CARTESIAN_POINT('Ctrl Pts',(2.20690665217742,-1.,-3.26863006136782));
#38899=CARTESIAN_POINT('Ctrl Pts',(2.20473979048678,-1.,-3.26138036637705));
#38900=CARTESIAN_POINT('Ctrl Pts',(2.20252866491545,-1.,-3.25415277957775));
#38901=CARTESIAN_POINT('Ctrl Pts',(2.20027910880981,-1.,-3.24695715874338));
#38902=CARTESIAN_POINT('Ctrl Pts',(2.19799623693253,-1.,-3.23980245361308));
#38903=CARTESIAN_POINT('Ctrl Pts',(2.19568204933168,-1.,-3.23269332296933));
#38904=CARTESIAN_POINT('Ctrl Pts',(2.19333345123538,-1.,-3.22562734221646));
#38905=CARTESIAN_POINT('Ctrl Pts',(2.19093901948667,-1.,-3.21859043114095));
#38906=CARTESIAN_POINT('Ctrl Pts',(2.18848253363901,-1.,-3.21156188355769));
#38907=CARTESIAN_POINT('Ctrl Pts',(2.18594876115934,-1.,-3.20452259717976));
#38908=CARTESIAN_POINT('Ctrl Pts',(2.18332898656602,-1.,-3.19746293740411));
#38909=CARTESIAN_POINT('Ctrl Pts',(2.18062558031778,-1.,-3.19038924261573));
#38910=CARTESIAN_POINT('Ctrl Pts',(2.17785968847142,-1.,-3.18333474627807));
#38911=CARTESIAN_POINT('Ctrl Pts',(2.17506466903694,-1.,-3.17635032802523));
#38912=CARTESIAN_POINT('Ctrl Pts',(2.17227212063817,-1.,-3.16948480019497));
#38913=CARTESIAN_POINT('Ctrl Pts',(2.16949910801219,-1.,-3.16276685102972));
#38914=CARTESIAN_POINT('Ctrl Pts',(2.16673728447689,-1.,-3.15618975593656));
#38915=CARTESIAN_POINT('Ctrl Pts',(2.16393520288072,-1.,-3.14968624389054));
#38916=CARTESIAN_POINT('Ctrl Pts',(2.16100905914435,-1.,-3.14314440427022));
#38917=CARTESIAN_POINT('Ctrl Pts',(2.15787423530676,-1.,-3.13645356563038));
#38918=CARTESIAN_POINT('Ctrl Pts',(2.1544724138292,-1.,-3.12954386795646));
#38919=CARTESIAN_POINT('Ctrl Pts',(2.15079698090584,-1.,-3.12242318151938));
#38920=CARTESIAN_POINT('Ctrl Pts',(2.14692798457532,-1.,-3.11522827016855));
#38921=CARTESIAN_POINT('Ctrl Pts',(2.14302815601973,-1.,-3.1082180866886));
#38922=CARTESIAN_POINT('Ctrl Pts',(2.13930228863751,-1.,-3.10171267391049));
#38923=CARTESIAN_POINT('Ctrl Pts',(2.13596538661048,-1.,-3.0960450242104));
#38924=CARTESIAN_POINT('Ctrl Pts',(2.13321032560893,-1.,-3.09151235281963));
#38925=CARTESIAN_POINT('Ctrl Pts',(2.13132142793017,-1.,-3.08855597949761));
#38926=CARTESIAN_POINT('Ctrl Pts',(2.13034980480424,-1.,-3.08717896996098));
#38927=CARTESIAN_POINT('Ctrl Pts',(2.12991938762373,-1.,-3.08668447250322));
#38928=CARTESIAN_POINT('Ctrl Pts',(2.1297578506149,-1.,-3.08657131089497));
#38929=CARTESIAN_POINT('Ctrl Pts',(2.1297112484669,-1.,-3.08655633322212));
#38930=CARTESIAN_POINT('',(2.27737254473378,-1.,-2.97927412174388));
#38931=CARTESIAN_POINT('Origin',(0.,-1.,0.));
#38932=CARTESIAN_POINT('',(2.66939624221984,-1.,-3.24257979115744));
#38933=CARTESIAN_POINT('Ctrl Pts',(2.27737254473378,-1.,-2.97927412174388));
#38934=CARTESIAN_POINT('Ctrl Pts',(2.27737238849212,-1.,-2.97932307137589));
#38935=CARTESIAN_POINT('Ctrl Pts',(2.27743009389704,-1.,-2.97951167106106));
#38936=CARTESIAN_POINT('Ctrl Pts',(2.27776738270369,-1.,-2.98007383024333));
#38937=CARTESIAN_POINT('Ctrl Pts',(2.27877674853833,-1.,-2.98142341809623));
#38938=CARTESIAN_POINT('Ctrl Pts',(2.28100472516582,-1.,-2.98413343613858));
#38939=CARTESIAN_POINT('Ctrl Pts',(2.28446419116036,-1.,-2.98815432734929));
#38940=CARTESIAN_POINT('Ctrl Pts',(2.28882328690601,-1.,-2.9930793098434));
#38941=CARTESIAN_POINT('Ctrl Pts',(2.29385894577999,-1.,-2.99863310340004));
#38942=CARTESIAN_POINT('Ctrl Pts',(2.29932091315939,-1.,-3.00450832658822));
#38943=CARTESIAN_POINT('Ctrl Pts',(2.30496809486528,-1.,-3.01041131063882));
#38944=CARTESIAN_POINT('Ctrl Pts',(2.31060449886577,-1.,-3.01610726819019));
#38945=CARTESIAN_POINT('Ctrl Pts',(2.31612479121528,-1.,-3.02147780668029));
#38946=CARTESIAN_POINT('Ctrl Pts',(2.32151944306299,-1.,-3.02652678416478));
#38947=CARTESIAN_POINT('Ctrl Pts',(2.32683687412027,-1.,-3.03133125185047));
#38948=CARTESIAN_POINT('Ctrl Pts',(2.33215619079807,-1.,-3.03600588555765));
#38949=CARTESIAN_POINT('Ctrl Pts',(2.33755792953726,-1.,-3.04066496998569));
#38950=CARTESIAN_POINT('Ctrl Pts',(2.3430901708402,-1.,-3.04537822217311));
#38951=CARTESIAN_POINT('Ctrl Pts',(2.34875673090816,-1.,-3.05015565829976));
#38952=CARTESIAN_POINT('Ctrl Pts',(2.35453559889506,-1.,-3.05497218368188));
#38953=CARTESIAN_POINT('Ctrl Pts',(2.36039011602084,-1.,-3.05978266240056));
#38954=CARTESIAN_POINT('Ctrl Pts',(2.36628220107001,-1.,-3.06453964643152));
#38955=CARTESIAN_POINT('Ctrl Pts',(2.37218678163157,-1.,-3.06921275497472));
#38956=CARTESIAN_POINT('Ctrl Pts',(2.37809856205524,-1.,-3.07379777492133));
#38957=CARTESIAN_POINT('Ctrl Pts',(2.38402401216107,-1.,-3.07830597244301));
#38958=CARTESIAN_POINT('Ctrl Pts',(2.38997659219192,-1.,-3.08275773747083));
#38959=CARTESIAN_POINT('Ctrl Pts',(2.39597098250635,-1.,-3.08717489512919));
#38960=CARTESIAN_POINT('Ctrl Pts',(2.40201704423352,-1.,-3.09157266051115));
#38961=CARTESIAN_POINT('Ctrl Pts',(2.40811612696382,-1.,-3.09595472616093));
#38962=CARTESIAN_POINT('Ctrl Pts',(2.41426441798067,-1.,-3.10031775027683));
#38963=CARTESIAN_POINT('Ctrl Pts',(2.42045498612494,-1.,-3.10465410280902));
#38964=CARTESIAN_POINT('Ctrl Pts',(2.42668025870013,-1.,-3.10895518969592));
#38965=CARTESIAN_POINT('Ctrl Pts',(2.4329344968514,-1.,-3.11321477659012));
#38966=CARTESIAN_POINT('Ctrl Pts',(2.43921571477975,-1.,-3.11743156744182));
#38967=CARTESIAN_POINT('Ctrl Pts',(2.44552433364716,-1.,-3.12160740887768));
#38968=CARTESIAN_POINT('Ctrl Pts',(2.45186227369848,-1.,-3.12574608210849));
#38969=CARTESIAN_POINT('Ctrl Pts',(2.45823188859366,-1.,-3.12985188384372));
#38970=CARTESIAN_POINT('Ctrl Pts',(2.4646349433237,-1.,-3.13392826623902));
#38971=CARTESIAN_POINT('Ctrl Pts',(2.47107164236827,-1.,-3.13797654408931));
#38972=CARTESIAN_POINT('Ctrl Pts',(2.47754112428027,-1.,-3.14199655778845));
#38973=CARTESIAN_POINT('Ctrl Pts',(2.48404187418376,-1.,-3.1459872272388));
#38974=CARTESIAN_POINT('Ctrl Pts',(2.49057217131985,-1.,-3.14994715298903));
#38975=CARTESIAN_POINT('Ctrl Pts',(2.49713050858911,-1.,-3.15387518039064));
#38976=CARTESIAN_POINT('Ctrl Pts',(2.50371605688287,-1.,-3.15777102413998));
#38977=CARTESIAN_POINT('Ctrl Pts',(2.51032851007939,-1.,-3.16163506380211));
#38978=CARTESIAN_POINT('Ctrl Pts',(2.51696788755615,-1.,-3.16546808277069));
#38979=CARTESIAN_POINT('Ctrl Pts',(2.523634346718,-1.,-3.16927102130751));
#38980=CARTESIAN_POINT('Ctrl Pts',(2.5303280040691,-1.,-3.17304474093574));
#38981=CARTESIAN_POINT('Ctrl Pts',(2.53704871950871,-1.,-3.17678974135225));
#38982=CARTESIAN_POINT('Ctrl Pts',(2.54379612552948,-1.,-3.18050619750515));
#38983=CARTESIAN_POINT('Ctrl Pts',(2.55056972387638,-1.,-3.18419408529482));
#38984=CARTESIAN_POINT('Ctrl Pts',(2.55736896206016,-1.,-3.1878532811617));
#38985=CARTESIAN_POINT('Ctrl Pts',(2.56419331092909,-1.,-3.19148366395201));
#38986=CARTESIAN_POINT('Ctrl Pts',(2.57104235898053,-1.,-3.19508523784548));
#38987=CARTESIAN_POINT('Ctrl Pts',(2.577915819091,-1.,-3.19865814628955));
#38988=CARTESIAN_POINT('Ctrl Pts',(2.58481347777953,-1.,-3.20220261408685));
#38989=CARTESIAN_POINT('Ctrl Pts',(2.59173516023605,-1.,-3.20571891028879));
#38990=CARTESIAN_POINT('Ctrl Pts',(2.59868069194267,-1.,-3.2092073056959));
#38991=CARTESIAN_POINT('Ctrl Pts',(2.60564985359699,-1.,-3.21266802609297));
#38992=CARTESIAN_POINT('Ctrl Pts',(2.61264236718662,-1.,-3.21610123232465));
#38993=CARTESIAN_POINT('Ctrl Pts',(2.61965792832396,-1.,-3.21950704108654));
#38994=CARTESIAN_POINT('Ctrl Pts',(2.62669622735548,-1.,-3.222885536128));
#38995=CARTESIAN_POINT('Ctrl Pts',(2.63375697391438,-1.,-3.22623678292539));
#38996=CARTESIAN_POINT('Ctrl Pts',(2.64083992182478,-1.,-3.2295608435934));
#38997=CARTESIAN_POINT('Ctrl Pts',(2.64794488744246,-1.,-3.23285778738558));
#38998=CARTESIAN_POINT('Ctrl Pts',(2.6550717396303,-1.,-3.23612768065687));
#38999=CARTESIAN_POINT('Ctrl Pts',(2.6607906631973,-1.,-3.23872200036311));
#39000=CARTESIAN_POINT('Ctrl Pts',(2.66508964664767,-1.,-3.24065561087681));
#39001=CARTESIAN_POINT('Ctrl Pts',(2.66795998539861,-1.,-3.24193929584813));
#39002=CARTESIAN_POINT('Ctrl Pts',(2.66939624221984,-1.,-3.24257979115744));
#39003=CARTESIAN_POINT('',(2.78507268004356,-1.,-3.14378277984898));
#39004=CARTESIAN_POINT('',(2.66939624221984,-1.,-3.24257979115744));
#39005=CARTESIAN_POINT('',(2.58633475774921,-1.,-2.71539546306948));
#39006=CARTESIAN_POINT('Ctrl Pts',(2.78507268004356,-1.,-3.14378277984898));
#39007=CARTESIAN_POINT('Ctrl Pts',(2.7846647503589,-1.,-3.14226401018816));
#39008=CARTESIAN_POINT('Ctrl Pts',(2.78384588958165,-1.,-3.13922819749279));
#39009=CARTESIAN_POINT('Ctrl Pts',(2.78260859419319,-1.,-3.13467965833037));
#39010=CARTESIAN_POINT('Ctrl Pts',(2.78094085161413,-1.,-3.12862530318457));
#39011=CARTESIAN_POINT('Ctrl Pts',(2.77882610146731,-1.,-3.12107467037201));
#39012=CARTESIAN_POINT('Ctrl Pts',(2.77668121002545,-1.,-3.11354142303921));
#39013=CARTESIAN_POINT('Ctrl Pts',(2.77450609123362,-1.,-3.10602568032564));
#39014=CARTESIAN_POINT('Ctrl Pts',(2.77230064796057,-1.,-3.0985276127786));
#39015=CARTESIAN_POINT('Ctrl Pts',(2.7700647803451,-1.,-3.09104745382531));
#39016=CARTESIAN_POINT('Ctrl Pts',(2.76779837829373,-1.,-3.08358548001504));
#39017=CARTESIAN_POINT('Ctrl Pts',(2.76550131064852,-1.,-3.07614198408862));
#39018=CARTESIAN_POINT('Ctrl Pts',(2.76317341453493,-1.,-3.0687172484321));
#39019=CARTESIAN_POINT('Ctrl Pts',(2.76081448759882,-1.,-3.06131152247454));
#39020=CARTESIAN_POINT('Ctrl Pts',(2.75842427252931,-1.,-3.05392498749847));
#39021=CARTESIAN_POINT('Ctrl Pts',(2.75600247455925,-1.,-3.04655777351067));
#39022=CARTESIAN_POINT('Ctrl Pts',(2.75354880060314,-1.,-3.03921001107977));
#39023=CARTESIAN_POINT('Ctrl Pts',(2.75106299522979,-1.,-3.03188187589107));
#39024=CARTESIAN_POINT('Ctrl Pts',(2.7485448718414,-1.,-3.02457362909245));
#39025=CARTESIAN_POINT('Ctrl Pts',(2.74599436193625,-1.,-3.01728567646611));
#39026=CARTESIAN_POINT('Ctrl Pts',(2.74341150239887,-1.,-3.01001855960162));
#39027=CARTESIAN_POINT('Ctrl Pts',(2.74079632883931,-1.,-3.00277284351521));
#39028=CARTESIAN_POINT('Ctrl Pts',(2.73814878711641,-1.,-2.99554902409778));
#39029=CARTESIAN_POINT('Ctrl Pts',(2.73546864694536,-1.,-2.9883474369644));
#39030=CARTESIAN_POINT('Ctrl Pts',(2.73275539286497,-1.,-2.98116814232129));
#39031=CARTESIAN_POINT('Ctrl Pts',(2.73000819218414,-1.,-2.97401089032677));
#39032=CARTESIAN_POINT('Ctrl Pts',(2.72722614084076,-1.,-2.96687537842451));
#39033=CARTESIAN_POINT('Ctrl Pts',(2.72440846811729,-1.,-2.95976146492576));
#39034=CARTESIAN_POINT('Ctrl Pts',(2.72155475123364,-1.,-2.95266939280621));
#39035=CARTESIAN_POINT('Ctrl Pts',(2.71866514227965,-1.,-2.94560002559806));
#39036=CARTESIAN_POINT('Ctrl Pts',(2.7157405459259,-1.,-2.93855503247266));
#39037=CARTESIAN_POINT('Ctrl Pts',(2.71278207520817,-1.,-2.93153633192595));
#39038=CARTESIAN_POINT('Ctrl Pts',(2.70979055994754,-1.,-2.92454558914778));
#39039=CARTESIAN_POINT('Ctrl Pts',(2.70676602302518,-1.,-2.91758367994737));
#39040=CARTESIAN_POINT('Ctrl Pts',(2.70370719782113,-1.,-2.91065019668329));
#39041=CARTESIAN_POINT('Ctrl Pts',(2.70061095078692,-1.,-2.90374285605838));
#39042=CARTESIAN_POINT('Ctrl Pts',(2.69747340630625,-1.,-2.89685866123671));
#39043=CARTESIAN_POINT('Ctrl Pts',(2.69429113011374,-1.,-2.88999512410309));
#39044=CARTESIAN_POINT('Ctrl Pts',(2.69106236420198,-1.,-2.88315153980466));
#39045=CARTESIAN_POINT('Ctrl Pts',(2.68778807801686,-1.,-2.8763300724388));
#39046=CARTESIAN_POINT('Ctrl Pts',(2.68447353139599,-1.,-2.86953736547238));
#39047=CARTESIAN_POINT('Ctrl Pts',(2.68112602796308,-1.,-2.86278224277689));
#39048=CARTESIAN_POINT('Ctrl Pts',(2.67775201955724,-1.,-2.85607274378018));
#39049=CARTESIAN_POINT('Ctrl Pts',(2.67435421039677,-1.,-2.84941315703092));
#39050=CARTESIAN_POINT('Ctrl Pts',(2.67092916452125,-1.,-2.84280157191323));
#39051=CARTESIAN_POINT('Ctrl Pts',(2.66746339678107,-1.,-2.83622586853982));
#39052=CARTESIAN_POINT('Ctrl Pts',(2.6639376472693,-1.,-2.82966813308998));
#39053=CARTESIAN_POINT('Ctrl Pts',(2.66033388273461,-1.,-2.82311188135078));
#39054=CARTESIAN_POINT('Ctrl Pts',(2.65664198781344,-1.,-2.81654896073883));
#39055=CARTESIAN_POINT('Ctrl Pts',(2.65286529532208,-1.,-2.80998526078165));
#39056=CARTESIAN_POINT('Ctrl Pts',(2.64902988983337,-1.,-2.80345029781152));
#39057=CARTESIAN_POINT('Ctrl Pts',(2.64517667799319,-1.,-2.79698910670736));
#39058=CARTESIAN_POINT('Ctrl Pts',(2.64134450532584,-1.,-2.79064495573224));
#39059=CARTESIAN_POINT('Ctrl Pts',(2.637554714303,-1.,-2.78444351041571));
#39060=CARTESIAN_POINT('Ctrl Pts',(2.63379800904599,-1.,-2.77837943466449));
#39061=CARTESIAN_POINT('Ctrl Pts',(2.63001305229625,-1.,-2.77239433377921));
#39062=CARTESIAN_POINT('Ctrl Pts',(2.62609956506355,-1.,-2.76639078479021));
#39063=CARTESIAN_POINT('Ctrl Pts',(2.62195665834605,-1.,-2.76027271596686));
#39064=CARTESIAN_POINT('Ctrl Pts',(2.61751580407667,-1.,-2.7539802502603));
#39065=CARTESIAN_POINT('Ctrl Pts',(2.61277170105813,-1.,-2.74752219567252));
#39066=CARTESIAN_POINT('Ctrl Pts',(2.60782480638448,-1.,-2.7410211099909));
#39067=CARTESIAN_POINT('Ctrl Pts',(2.60287635688728,-1.,-2.73470730109615));
#39068=CARTESIAN_POINT('Ctrl Pts',(2.59817869034746,-1.,-2.7288648348152));
#39069=CARTESIAN_POINT('Ctrl Pts',(2.59399625537278,-1.,-2.72378896977134));
#39070=CARTESIAN_POINT('Ctrl Pts',(2.59056604771971,-1.,-2.71974308958086));
#39071=CARTESIAN_POINT('Ctrl Pts',(2.58823792682672,-1.,-2.71711860281815));
#39072=CARTESIAN_POINT('Ctrl Pts',(2.58706285424358,-1.,-2.71591054189786));
#39073=CARTESIAN_POINT('Ctrl Pts',(2.58656037976753,-1.,-2.71548946460575));
#39074=CARTESIAN_POINT('Ctrl Pts',(2.58638312917167,-1.,-2.71540296616024));
#39075=CARTESIAN_POINT('Ctrl Pts',(2.58633475774921,-1.,-2.71539546306948));
#39076=CARTESIAN_POINT('',(2.71539546306824,-1.,-2.58633475775051));
#39077=CARTESIAN_POINT('Origin',(0.,-1.,0.));
#39078=CARTESIAN_POINT('',(3.14378277984898,-1.,-2.78507268004356));
#39079=CARTESIAN_POINT('Ctrl Pts',(2.71539546306824,-1.,-2.58633475775051));
#39080=CARTESIAN_POINT('Ctrl Pts',(2.71540296615967,-1.,-2.58638312917291));
#39081=CARTESIAN_POINT('Ctrl Pts',(2.71548946460616,-1.,-2.58656037976884));
#39082=CARTESIAN_POINT('Ctrl Pts',(2.71591054189884,-1.,-2.58706285424469));
#39083=CARTESIAN_POINT('Ctrl Pts',(2.7171186028189,-1.,-2.58823792682724));
#39084=CARTESIAN_POINT('Ctrl Pts',(2.7197430895797,-1.,-2.59056604771863));
#39085=CARTESIAN_POINT('Ctrl Pts',(2.72378896977273,-1.,-2.59399625537407));
#39086=CARTESIAN_POINT('Ctrl Pts',(2.72886483481804,-1.,-2.5981786903501));
#39087=CARTESIAN_POINT('Ctrl Pts',(2.73470730109906,-1.,-2.60287635689));
#39088=CARTESIAN_POINT('Ctrl Pts',(2.74102110999284,-1.,-2.60782480638629));
#39089=CARTESIAN_POINT('Ctrl Pts',(2.74752219567307,-1.,-2.61277170105864));
#39090=CARTESIAN_POINT('Ctrl Pts',(2.75398025025967,-1.,-2.61751580407608));
#39091=CARTESIAN_POINT('Ctrl Pts',(2.76027271596564,-1.,-2.62195665834491));
#39092=CARTESIAN_POINT('Ctrl Pts',(2.76639078478898,-1.,-2.6260995650624));
#39093=CARTESIAN_POINT('Ctrl Pts',(2.77239433377839,-1.,-2.63001305229548));
#39094=CARTESIAN_POINT('Ctrl Pts',(2.77837943466423,-1.,-2.63379800904575));
#39095=CARTESIAN_POINT('Ctrl Pts',(2.78444351041594,-1.,-2.63755471430322));
#39096=CARTESIAN_POINT('Ctrl Pts',(2.79064495573275,-1.,-2.64134450532632));
#39097=CARTESIAN_POINT('Ctrl Pts',(2.7969891067079,-1.,-2.6451766779937));
#39098=CARTESIAN_POINT('Ctrl Pts',(2.80345029781191,-1.,-2.64902988983373));
#39099=CARTESIAN_POINT('Ctrl Pts',(2.80998526078179,-1.,-2.65286529532221));
#39100=CARTESIAN_POINT('Ctrl Pts',(2.81654896073874,-1.,-2.65664198781335));
#39101=CARTESIAN_POINT('Ctrl Pts',(2.82311188135053,-1.,-2.66033388273437));
#39102=CARTESIAN_POINT('Ctrl Pts',(2.82966813308969,-1.,-2.66393764726902));
#39103=CARTESIAN_POINT('Ctrl Pts',(2.8362258685396,-1.,-2.66746339678085));
#39104=CARTESIAN_POINT('Ctrl Pts',(2.84280157191314,-1.,-2.67092916452117));
#39105=CARTESIAN_POINT('Ctrl Pts',(2.84941315703096,-1.,-2.67435421039682));
#39106=CARTESIAN_POINT('Ctrl Pts',(2.85607274378031,-1.,-2.67775201955736));
#39107=CARTESIAN_POINT('Ctrl Pts',(2.86278224277705,-1.,-2.68112602796323));
#39108=CARTESIAN_POINT('Ctrl Pts',(2.8695373654725,-1.,-2.68447353139611));
#39109=CARTESIAN_POINT('Ctrl Pts',(2.87633007243885,-1.,-2.68778807801691));
#39110=CARTESIAN_POINT('Ctrl Pts',(2.88315153980464,-1.,-2.69106236420197));
#39111=CARTESIAN_POINT('Ctrl Pts',(2.88999512410304,-1.,-2.69429113011369));
#39112=CARTESIAN_POINT('Ctrl Pts',(2.89685866123668,-1.,-2.69747340630621));
#39113=CARTESIAN_POINT('Ctrl Pts',(2.90374285605839,-1.,-2.70061095078692));
#39114=CARTESIAN_POINT('Ctrl Pts',(2.91065019668331,-1.,-2.70370719782114));
#39115=CARTESIAN_POINT('Ctrl Pts',(2.91758367994738,-1.,-2.70676602302518));
#39116=CARTESIAN_POINT('Ctrl Pts',(2.92454558914774,-1.,-2.70979055994751));
#39117=CARTESIAN_POINT('Ctrl Pts',(2.93153633192583,-1.,-2.71278207520807));
#39118=CARTESIAN_POINT('Ctrl Pts',(2.93855503247248,-1.,-2.71574054592575));
#39119=CARTESIAN_POINT('Ctrl Pts',(2.94560002559789,-1.,-2.71866514227951));
#39120=CARTESIAN_POINT('Ctrl Pts',(2.95266939280617,-1.,-2.72155475123361));
#39121=CARTESIAN_POINT('Ctrl Pts',(2.95976146492595,-1.,-2.72440846811745));
#39122=CARTESIAN_POINT('Ctrl Pts',(2.96687537842492,-1.,-2.72722614084112));
#39123=CARTESIAN_POINT('Ctrl Pts',(2.97401089032729,-1.,-2.7300081921846));
#39124=CARTESIAN_POINT('Ctrl Pts',(2.98116814232175,-1.,-2.73275539286537));
#39125=CARTESIAN_POINT('Ctrl Pts',(2.98834743696455,-1.,-2.73546864694548));
#39126=CARTESIAN_POINT('Ctrl Pts',(2.99554902409741,-1.,-2.73814878711609));
#39127=CARTESIAN_POINT('Ctrl Pts',(3.00277284351431,-1.,-2.74079632883852));
#39128=CARTESIAN_POINT('Ctrl Pts',(3.01001855960041,-1.,-2.7434115023978));
#39129=CARTESIAN_POINT('Ctrl Pts',(3.01728567646502,-1.,-2.74599436193528));
#39130=CARTESIAN_POINT('Ctrl Pts',(3.02457362909199,-1.,-2.74854487184099));
#39131=CARTESIAN_POINT('Ctrl Pts',(3.03188187589168,-1.,-2.75106299523032));
#39132=CARTESIAN_POINT('Ctrl Pts',(3.03921001108158,-1.,-2.75354880060473));
#39133=CARTESIAN_POINT('Ctrl Pts',(3.04655777351333,-1.,-2.7560024745616));
#39134=CARTESIAN_POINT('Ctrl Pts',(3.05392498750112,-1.,-2.75842427253164));
#39135=CARTESIAN_POINT('Ctrl Pts',(3.06131152247599,-1.,-2.76081448760011));
#39136=CARTESIAN_POINT('Ctrl Pts',(3.06871724843121,-1.,-2.76317341453415));
#39137=CARTESIAN_POINT('Ctrl Pts',(3.07614198408488,-1.,-2.76550131064522));
#39138=CARTESIAN_POINT('Ctrl Pts',(3.08358548000904,-1.,-2.76779837828843));
#39139=CARTESIAN_POINT('Ctrl Pts',(3.09104745381882,-1.,-2.77006478033937));
#39140=CARTESIAN_POINT('Ctrl Pts',(3.09852761277432,-1.,-2.77230064795679));
#39141=CARTESIAN_POINT('Ctrl Pts',(3.10602568032641,-1.,-2.7745060912343));
#39142=CARTESIAN_POINT('Ctrl Pts',(3.11354142304692,-1.,-2.77668121003225));
#39143=CARTESIAN_POINT('Ctrl Pts',(3.12107467038623,-1.,-2.77882610147986));
#39144=CARTESIAN_POINT('Ctrl Pts',(3.12862530320194,-1.,-2.78094085162947));
#39145=CARTESIAN_POINT('Ctrl Pts',(3.1346796583452,-1.,-2.78260859420629));
#39146=CARTESIAN_POINT('Ctrl Pts',(3.13922819750185,-1.,-2.78384588958965));
#39147=CARTESIAN_POINT('Ctrl Pts',(3.14226401019149,-1.,-2.78466475036183));
#39148=CARTESIAN_POINT('Ctrl Pts',(3.14378277984898,-1.,-2.78507268004356));
#39149=CARTESIAN_POINT('',(3.24257979115744,-1.,-2.66939624221984));
#39150=CARTESIAN_POINT('',(3.14378277984898,-1.,-2.78507268004356));
#39151=CARTESIAN_POINT('',(2.97927412174279,-1.,-2.27737254473521));
#39152=CARTESIAN_POINT('Ctrl Pts',(3.24257979115744,-1.,-2.66939624221984));
#39153=CARTESIAN_POINT('Ctrl Pts',(3.24193929584471,-1.,-2.66795998539579));
#39154=CARTESIAN_POINT('Ctrl Pts',(3.24065561086749,-1.,-2.66508964663997));
#39155=CARTESIAN_POINT('Ctrl Pts',(3.23872200034785,-1.,-2.6607906631847));
#39156=CARTESIAN_POINT('Ctrl Pts',(3.236127680639,-1.,-2.65507173961555));
#39157=CARTESIAN_POINT('Ctrl Pts',(3.23285778737096,-1.,-2.64794488743038));
#39158=CARTESIAN_POINT('Ctrl Pts',(3.22956084358547,-1.,-2.64083992181823));
#39159=CARTESIAN_POINT('Ctrl Pts',(3.2262367829246,-1.,-2.63375697391372));
#39160=CARTESIAN_POINT('Ctrl Pts',(3.2228855361324,-1.,-2.62669622735912));
#39161=CARTESIAN_POINT('Ctrl Pts',(3.21950704109321,-1.,-2.61965792832947));
#39162=CARTESIAN_POINT('Ctrl Pts',(3.21610123233082,-1.,-2.61264236719171));
#39163=CARTESIAN_POINT('Ctrl Pts',(3.21266802609681,-1.,-2.60564985360017));
#39164=CARTESIAN_POINT('Ctrl Pts',(3.20920730569681,-1.,-2.59868069194342));
#39165=CARTESIAN_POINT('Ctrl Pts',(3.2057189102873,-1.,-2.59173516023481));
#39166=CARTESIAN_POINT('Ctrl Pts',(3.20220261408414,-1.,-2.58481347777729));
#39167=CARTESIAN_POINT('Ctrl Pts',(3.19865814628682,-1.,-2.57791581908875));
#39168=CARTESIAN_POINT('Ctrl Pts',(3.19508523784363,-1.,-2.57104235897899));
#39169=CARTESIAN_POINT('Ctrl Pts',(3.19148366395139,-1.,-2.56419331092858));
#39170=CARTESIAN_POINT('Ctrl Pts',(3.18785328116218,-1.,-2.55736896206056));
#39171=CARTESIAN_POINT('Ctrl Pts',(3.18419408529594,-1.,-2.55056972387731));
#39172=CARTESIAN_POINT('Ctrl Pts',(3.18050619750639,-1.,-2.54379612553051));
#39173=CARTESIAN_POINT('Ctrl Pts',(3.17678974135318,-1.,-2.53704871950948));
#39174=CARTESIAN_POINT('Ctrl Pts',(3.17304474093612,-1.,-2.53032800406941));
#39175=CARTESIAN_POINT('Ctrl Pts',(3.16927102130735,-1.,-2.52363434671788));
#39176=CARTESIAN_POINT('Ctrl Pts',(3.16546808277023,-1.,-2.51696788755577));
#39177=CARTESIAN_POINT('Ctrl Pts',(3.16163506380157,-1.,-2.51032851007894));
#39178=CARTESIAN_POINT('Ctrl Pts',(3.15777102413957,-1.,-2.50371605688252));
#39179=CARTESIAN_POINT('Ctrl Pts',(3.15387518039046,-1.,-2.49713050858896));
#39180=CARTESIAN_POINT('Ctrl Pts',(3.14994715298907,-1.,-2.49057217131988));
#39181=CARTESIAN_POINT('Ctrl Pts',(3.14598722723896,-1.,-2.4840418741839));
#39182=CARTESIAN_POINT('Ctrl Pts',(3.14199655778863,-1.,-2.47754112428043));
#39183=CARTESIAN_POINT('Ctrl Pts',(3.13797654408943,-1.,-2.47107164236838));
#39184=CARTESIAN_POINT('Ctrl Pts',(3.13392826623906,-1.,-2.46463494332374));
#39185=CARTESIAN_POINT('Ctrl Pts',(3.12985188384371,-1.,-2.45823188859366));
#39186=CARTESIAN_POINT('Ctrl Pts',(3.12574608210847,-1.,-2.45186227369846));
#39187=CARTESIAN_POINT('Ctrl Pts',(3.12160740887768,-1.,-2.44552433364715));
#39188=CARTESIAN_POINT('Ctrl Pts',(3.11743156744186,-1.,-2.43921571477977));
#39189=CARTESIAN_POINT('Ctrl Pts',(3.11321477659018,-1.,-2.43293449685144));
#39190=CARTESIAN_POINT('Ctrl Pts',(3.10895518969595,-1.,-2.42668025870015));
#39191=CARTESIAN_POINT('Ctrl Pts',(3.10465410280896,-1.,-2.42045498612489));
#39192=CARTESIAN_POINT('Ctrl Pts',(3.1003177502767,-1.,-2.41426441798057));
#39193=CARTESIAN_POINT('Ctrl Pts',(3.09595472616076,-1.,-2.40811612696369));
#39194=CARTESIAN_POINT('Ctrl Pts',(3.091572660511,-1.,-2.40201704423341));
#39195=CARTESIAN_POINT('Ctrl Pts',(3.08717489512914,-1.,-2.39597098250631));
#39196=CARTESIAN_POINT('Ctrl Pts',(3.08275773747093,-1.,-2.38997659219199));
#39197=CARTESIAN_POINT('Ctrl Pts',(3.07830597244326,-1.,-2.38402401216126));
#39198=CARTESIAN_POINT('Ctrl Pts',(3.07379777492165,-1.,-2.37809856205548));
#39199=CARTESIAN_POINT('Ctrl Pts',(3.069212754975,-1.,-2.37218678163178));
#39200=CARTESIAN_POINT('Ctrl Pts',(3.06453964643162,-1.,-2.36628220107009));
#39201=CARTESIAN_POINT('Ctrl Pts',(3.0597826624004,-1.,-2.36039011602072));
#39202=CARTESIAN_POINT('Ctrl Pts',(3.05497218368146,-1.,-2.35453559889474));
#39203=CARTESIAN_POINT('Ctrl Pts',(3.05015565829918,-1.,-2.34875673090771));
#39204=CARTESIAN_POINT('Ctrl Pts',(3.04537822217256,-1.,-2.34309017083977));
#39205=CARTESIAN_POINT('Ctrl Pts',(3.04066496998544,-1.,-2.33755792953706));
#39206=CARTESIAN_POINT('Ctrl Pts',(3.03600588555793,-1.,-2.33215619079829));
#39207=CARTESIAN_POINT('Ctrl Pts',(3.03133125185136,-1.,-2.32683687412097));
#39208=CARTESIAN_POINT('Ctrl Pts',(3.02652678416611,-1.,-2.32151944306402));
#39209=CARTESIAN_POINT('Ctrl Pts',(3.0214778066816,-1.,-2.31612479121631));
#39210=CARTESIAN_POINT('Ctrl Pts',(3.01610726819086,-1.,-2.31060449886629));
#39211=CARTESIAN_POINT('Ctrl Pts',(3.01041131063823,-1.,-2.30496809486482));
#39212=CARTESIAN_POINT('Ctrl Pts',(3.00450832658613,-1.,-2.29932091315775));
#39213=CARTESIAN_POINT('Ctrl Pts',(2.99863310339691,-1.,-2.29385894577754));
#39214=CARTESIAN_POINT('Ctrl Pts',(2.99307930984034,-1.,-2.28882328690362));
#39215=CARTESIAN_POINT('Ctrl Pts',(2.9881543273478,-1.,-2.28446419115919));
#39216=CARTESIAN_POINT('Ctrl Pts',(2.98413343613983,-1.,-2.28100472516679));
#39217=CARTESIAN_POINT('Ctrl Pts',(2.9814234180956,-1.,-2.27877674853766));
#39218=CARTESIAN_POINT('Ctrl Pts',(2.98007383024207,-1.,-2.27776738270289));
#39219=CARTESIAN_POINT('Ctrl Pts',(2.9795116710597,-1.,-2.27743009389684));
#39220=CARTESIAN_POINT('Ctrl Pts',(2.97932307137476,-1.,-2.27737238849287));
#39221=CARTESIAN_POINT('Ctrl Pts',(2.97927412174279,-1.,-2.27737254473521));
#39222=CARTESIAN_POINT('',(3.08655633322109,-1.,-2.12971124846838));
#39223=CARTESIAN_POINT('Origin',(0.,-1.,0.));
#39224=CARTESIAN_POINT('',(3.54075895182139,-1.,-2.25898783642071));
#39225=CARTESIAN_POINT('Ctrl Pts',(3.08655633322109,-1.,-2.12971124846838));
#39226=CARTESIAN_POINT('Ctrl Pts',(3.0865713108946,-1.,-2.1297578506162));
#39227=CARTESIAN_POINT('Ctrl Pts',(3.08668447250383,-1.,-2.12991938762497));
#39228=CARTESIAN_POINT('Ctrl Pts',(3.08717896996213,-1.,-2.13034980480519));
#39229=CARTESIAN_POINT('Ctrl Pts',(3.08855597949844,-1.,-2.13132142793056));
#39230=CARTESIAN_POINT('Ctrl Pts',(3.09151235281832,-1.,-2.13321032560805));
#39231=CARTESIAN_POINT('Ctrl Pts',(3.09604502421197,-1.,-2.13596538661154));
#39232=CARTESIAN_POINT('Ctrl Pts',(3.1017126739137,-1.,-2.13930228863968));
#39233=CARTESIAN_POINT('Ctrl Pts',(3.10821808669189,-1.,-2.14302815602195));
#39234=CARTESIAN_POINT('Ctrl Pts',(3.11522827017075,-1.,-2.1469279845768));
#39235=CARTESIAN_POINT('Ctrl Pts',(3.12242318152001,-1.,-2.15079698090627));
#39236=CARTESIAN_POINT('Ctrl Pts',(3.12954386795575,-1.,-2.15447241382872));
#39237=CARTESIAN_POINT('Ctrl Pts',(3.136453565629,-1.,-2.15787423530583));
#39238=CARTESIAN_POINT('Ctrl Pts',(3.14314440426882,-1.,-2.16100905914341));
#39239=CARTESIAN_POINT('Ctrl Pts',(3.14968624388961,-1.,-2.16393520288009));
#39240=CARTESIAN_POINT('Ctrl Pts',(3.15618975593627,-1.,-2.1667372844767));
#39241=CARTESIAN_POINT('Ctrl Pts',(3.16276685102999,-1.,-2.16949910801237));
#39242=CARTESIAN_POINT('Ctrl Pts',(3.16948480019555,-1.,-2.17227212063857));
#39243=CARTESIAN_POINT('Ctrl Pts',(3.17635032802584,-1.,-2.17506466903736));
#39244=CARTESIAN_POINT('Ctrl Pts',(3.18333474627851,-1.,-2.17785968847172));
#39245=CARTESIAN_POINT('Ctrl Pts',(3.19038924261589,-1.,-2.18062558031789));
#39246=CARTESIAN_POINT('Ctrl Pts',(3.197462937404,-1.,-2.18332898656595));
#39247=CARTESIAN_POINT('Ctrl Pts',(3.20452259717947,-1.,-2.18594876115914));
#39248=CARTESIAN_POINT('Ctrl Pts',(3.21156188355736,-1.,-2.18848253363878));
#39249=CARTESIAN_POINT('Ctrl Pts',(3.21859043114069,-1.,-2.1909390194865));
#39250=CARTESIAN_POINT('Ctrl Pts',(3.22562734221636,-1.,-2.19333345123531));
#39251=CARTESIAN_POINT('Ctrl Pts',(3.23269332296938,-1.,-2.19568204933172));
#39252=CARTESIAN_POINT('Ctrl Pts',(3.23980245361323,-1.,-2.19799623693263));
#39253=CARTESIAN_POINT('Ctrl Pts',(3.24695715874356,-1.,-2.20027910880993));
#39254=CARTESIAN_POINT('Ctrl Pts',(3.25415277957789,-1.,-2.20252866491554));
#39255=CARTESIAN_POINT('Ctrl Pts',(3.26138036637711,-1.,-2.20473979048682));
#39256=CARTESIAN_POINT('Ctrl Pts',(3.2686300613678,-1.,-2.20690665217741));
#39257=CARTESIAN_POINT('Ctrl Pts',(3.27589448005534,-1.,-2.20902509417425));
#39258=CARTESIAN_POINT('Ctrl Pts',(3.28317133333127,-1.,-2.21109449750638));
#39259=CARTESIAN_POINT('Ctrl Pts',(3.29046159238344,-1.,-2.21311648827391));
#39260=CARTESIAN_POINT('Ctrl Pts',(3.29776825193162,-1.,-2.2150940692337));
#39261=CARTESIAN_POINT('Ctrl Pts',(3.3050948781957,-1.,-2.21703059947837));
#39262=CARTESIAN_POINT('Ctrl Pts',(3.31244421655662,-1.,-2.21892881679083));
#39263=CARTESIAN_POINT('Ctrl Pts',(3.31981686778008,-1.,-2.22078990842768));
#39264=CARTESIAN_POINT('Ctrl Pts',(3.32721196326019,-1.,-2.22261398879623));
#39265=CARTESIAN_POINT('Ctrl Pts',(3.3346277284958,-1.,-2.224400498785));
#39266=CARTESIAN_POINT('Ctrl Pts',(3.34206209449371,-1.,-2.22614863918044));
#39267=CARTESIAN_POINT('Ctrl Pts',(3.34951327111117,-1.,-2.22785777756588));
#39268=CARTESIAN_POINT('Ctrl Pts',(3.35698038165529,-1.,-2.22952789881011));
#39269=CARTESIAN_POINT('Ctrl Pts',(3.36446325227908,-1.,-2.23115945849777));
#39270=CARTESIAN_POINT('Ctrl Pts',(3.37196214349356,-1.,-2.23275319569253));
#39271=CARTESIAN_POINT('Ctrl Pts',(3.37947749555649,-1.,-2.23430995599572));
#39272=CARTESIAN_POINT('Ctrl Pts',(3.38700968549522,-1.,-2.23583052276281));
#39273=CARTESIAN_POINT('Ctrl Pts',(3.39455873448088,-1.,-2.23731541452727));
#39274=CARTESIAN_POINT('Ctrl Pts',(3.40212434705511,-1.,-2.23876491124064));
#39275=CARTESIAN_POINT('Ctrl Pts',(3.40970604190205,-1.,-2.24017914395211));
#39276=CARTESIAN_POINT('Ctrl Pts',(3.41730325539119,-1.,-2.24155816587811));
#39277=CARTESIAN_POINT('Ctrl Pts',(3.42491544683075,-1.,-2.24290202531144));
#39278=CARTESIAN_POINT('Ctrl Pts',(3.43254222615007,-1.,-2.24421085338856));
#39279=CARTESIAN_POINT('Ctrl Pts',(3.44018336460619,-1.,-2.24548487526212));
#39280=CARTESIAN_POINT('Ctrl Pts',(3.44783872863448,-1.,-2.24672437070139));
#39281=CARTESIAN_POINT('Ctrl Pts',(3.45550823512213,-1.,-2.24792964960874));
#39282=CARTESIAN_POINT('Ctrl Pts',(3.46319180177474,-1.,-2.24910102345977));
#39283=CARTESIAN_POINT('Ctrl Pts',(3.47088928979467,-1.,-2.25023877475674));
#39284=CARTESIAN_POINT('Ctrl Pts',(3.47860048448015,-1.,-2.25134314238258));
#39285=CARTESIAN_POINT('Ctrl Pts',(3.48632513240231,-1.,-2.25241433138231));
#39286=CARTESIAN_POINT('Ctrl Pts',(3.49406296494309,-1.,-2.25345251709453));
#39287=CARTESIAN_POINT('Ctrl Pts',(3.50181372618058,-1.,-2.25445785151923));
#39288=CARTESIAN_POINT('Ctrl Pts',(3.50957720118209,-1.,-2.25543046980351));
#39289=CARTESIAN_POINT('Ctrl Pts',(3.51735323669213,-1.,-2.25637049456061));
#39290=CARTESIAN_POINT('Ctrl Pts',(3.52514172849666,-1.,-2.25727802942142));
#39291=CARTESIAN_POINT('Ctrl Pts',(3.53138243689932,-1.,-2.25797812951166));
#39292=CARTESIAN_POINT('Ctrl Pts',(3.53606853163247,-1.,-2.25848864344599));
#39293=CARTESIAN_POINT('Ctrl Pts',(3.5391950664771,-1.,-2.25882251694918));
#39294=CARTESIAN_POINT('Ctrl Pts',(3.54075895182139,-1.,-2.25898783642071));
#39295=CARTESIAN_POINT('',(3.62024382630768,-1.,-2.12928030988903));
#39296=CARTESIAN_POINT('',(3.54075895182139,-1.,-2.25898783642071));
#39297=CARTESIAN_POINT('',(3.29885386921513,-1.,-1.78327315618341));
#39298=CARTESIAN_POINT('Ctrl Pts',(3.62024382630768,-1.,-2.12928030988903));
#39299=CARTESIAN_POINT('Ctrl Pts',(3.61938653648716,-1.,-2.12796193131142));
#39300=CARTESIAN_POINT('Ctrl Pts',(3.61766963589442,-1.,-2.12532774376144));
#39301=CARTESIAN_POINT('Ctrl Pts',(3.61508732215187,-1.,-2.12138417125349));
#39302=CARTESIAN_POINT('Ctrl Pts',(3.61163030607452,-1.,-2.11614149813928));
#39303=CARTESIAN_POINT('Ctrl Pts',(3.60728578530968,-1.,-2.10961391333497));
#39304=CARTESIAN_POINT('Ctrl Pts',(3.60291797087849,-1.,-2.10311217727687));
#39305=CARTESIAN_POINT('Ctrl Pts',(3.59852681775396,-1.,-2.09663642986579));
#39306=CARTESIAN_POINT('Ctrl Pts',(3.5941122862608,-1.,-2.09018686331706));
#39307=CARTESIAN_POINT('Ctrl Pts',(3.58967435355834,-1.,-2.08376373049196));
#39308=CARTESIAN_POINT('Ctrl Pts',(3.58521300039988,-1.,-2.07736732842524));
#39309=CARTESIAN_POINT('Ctrl Pts',(3.58072819250872,-1.,-2.07099797606));
#39310=CARTESIAN_POINT('Ctrl Pts',(3.57621986224402,-1.,-2.06465599229234));
#39311=CARTESIAN_POINT('Ctrl Pts',(3.5716878942334,-1.,-2.05834167687425));
#39312=CARTESIAN_POINT('Ctrl Pts',(3.56713209977904,-1.,-2.05205528172911));
#39313=CARTESIAN_POINT('Ctrl Pts',(3.56255223871505,-1.,-2.04579702158876));
#39314=CARTESIAN_POINT('Ctrl Pts',(3.55794807264844,-1.,-2.03956711119976));
#39315=CARTESIAN_POINT('Ctrl Pts',(3.55331941293949,-1.,-2.03336579658133));
#39316=CARTESIAN_POINT('Ctrl Pts',(3.54866616282227,-1.,-2.02719338376175));
#39317=CARTESIAN_POINT('Ctrl Pts',(3.54398838254136,-1.,-2.02105027983104));
#39318=CARTESIAN_POINT('Ctrl Pts',(3.53928627453642,-1.,-2.01493698847351));
#39319=CARTESIAN_POINT('Ctrl Pts',(3.53456004727424,-1.,-2.00885403604746));
#39320=CARTESIAN_POINT('Ctrl Pts',(3.52980980250224,-1.,-2.00280191090366));
#39321=CARTESIAN_POINT('Ctrl Pts',(3.52503542491728,-1.,-1.99678100339296));
#39322=CARTESIAN_POINT('Ctrl Pts',(3.52023644289142,-1.,-1.99079153006112));
#39323=CARTESIAN_POINT('Ctrl Pts',(3.51541198728301,-1.,-1.9848335106103));
#39324=CARTESIAN_POINT('Ctrl Pts',(3.51056110478287,-1.,-1.97890693666288));
#39325=CARTESIAN_POINT('Ctrl Pts',(3.5056830186108,-1.,-1.97301191162968));
#39326=CARTESIAN_POINT('Ctrl Pts',(3.50077740176267,-1.,-1.96714879724052));
#39327=CARTESIAN_POINT('Ctrl Pts',(3.49584466573064,-1.,-1.961318367765));
#39328=CARTESIAN_POINT('Ctrl Pts',(3.49088618670987,-1.,-1.95552193112084));
#39329=CARTESIAN_POINT('Ctrl Pts',(3.48590361610814,-1.,-1.94976096795911));
#39330=CARTESIAN_POINT('Ctrl Pts',(3.48089825770416,-1.,-1.94403680554065));
#39331=CARTESIAN_POINT('Ctrl Pts',(3.47587040389915,-1.,-1.93835026973887));
#39332=CARTESIAN_POINT('Ctrl Pts',(3.47081872409781,-1.,-1.93270136427081));
#39333=CARTESIAN_POINT('Ctrl Pts',(3.46573953254084,-1.,-1.92708888591158));
#39334=CARTESIAN_POINT('Ctrl Pts',(3.46062821722485,-1.,-1.92151118213212));
#39335=CARTESIAN_POINT('Ctrl Pts',(3.4554807430995,-1.,-1.91596694784064));
#39336=CARTESIAN_POINT('Ctrl Pts',(3.45029522038888,-1.,-1.91045605593639));
#39337=CARTESIAN_POINT('Ctrl Pts',(3.44507323983367,-1.,-1.90498026502305));
#39338=CARTESIAN_POINT('Ctrl Pts',(3.4398218567809,-1.,-1.89954426803384));
#39339=CARTESIAN_POINT('Ctrl Pts',(3.43455074411571,-1.,-1.89415420002542));
#39340=CARTESIAN_POINT('Ctrl Pts',(3.42926852222158,-1.,-1.88881571322009));
#39341=CARTESIAN_POINT('Ctrl Pts',(3.42397908819736,-1.,-1.8835320506206));
#39342=CARTESIAN_POINT('Ctrl Pts',(3.41867858383771,-1.,-1.87830245689344));
#39343=CARTESIAN_POINT('Ctrl Pts',(3.41335043875209,-1.,-1.87311957248121));
#39344=CARTESIAN_POINT('Ctrl Pts',(3.40797080000549,-1.,-1.86797231196654));
#39345=CARTESIAN_POINT('Ctrl Pts',(3.40251742305476,-1.,-1.86285057051245));
#39346=CARTESIAN_POINT('Ctrl Pts',(3.39697816833067,-1.,-1.85774972037062));
#39347=CARTESIAN_POINT('Ctrl Pts',(3.39135802549398,-1.,-1.85267433291769));
#39348=CARTESIAN_POINT('Ctrl Pts',(3.38569092349592,-1.,-1.84764441927753));
#39349=CARTESIAN_POINT('Ctrl Pts',(3.38002968341157,-1.,-1.84269016931643));
#39350=CARTESIAN_POINT('Ctrl Pts',(3.37442462015853,-1.,-1.83784072967077));
#39351=CARTESIAN_POINT('Ctrl Pts',(3.36890396271836,-1.,-1.83311391452322));
#39352=CARTESIAN_POINT('Ctrl Pts',(3.36345722124158,-1.,-1.82850752153199));
#39353=CARTESIAN_POINT('Ctrl Pts',(3.35800801557424,-1.,-1.82398496829301));
#39354=CARTESIAN_POINT('Ctrl Pts',(3.35243086937598,-1.,-1.81948458796829));
#39355=CARTESIAN_POINT('Ctrl Pts',(3.34660014370673,-1.,-1.81494618732853));
#39356=CARTESIAN_POINT('Ctrl Pts',(3.34043216147606,-1.,-1.81033399625352));
#39357=CARTESIAN_POINT('Ctrl Pts',(3.33392460276808,-1.,-1.80565802981102));
#39358=CARTESIAN_POINT('Ctrl Pts',(3.32721088039578,-1.,-1.80100380443406));
#39359=CARTESIAN_POINT('Ctrl Pts',(3.3205535510082,-1.,-1.79652817033251));
#39360=CARTESIAN_POINT('Ctrl Pts',(3.31428038326424,-1.,-1.79242331349949));
#39361=CARTESIAN_POINT('Ctrl Pts',(3.30873412266788,-1.,-1.78888832245873));
#39362=CARTESIAN_POINT('Ctrl Pts',(3.30422155559112,-1.,-1.78610045419846));
#39363=CARTESIAN_POINT('Ctrl Pts',(3.30119637003393,-1.,-1.78432384788174));
#39364=CARTESIAN_POINT('Ctrl Pts',(3.299705498242,-1.,-1.78353803106924));
#39365=CARTESIAN_POINT('Ctrl Pts',(3.29909749657808,-1.,-1.78329283591905));
#39366=CARTESIAN_POINT('Ctrl Pts',(3.29890219175423,-1.,-1.78326534445518));
#39367=CARTESIAN_POINT('Ctrl Pts',(3.29885386921513,-1.,-1.78327315618341));
#39368=CARTESIAN_POINT('',(3.38171594275687,-1.,-1.62064718014256));
#39369=CARTESIAN_POINT('Origin',(0.,-1.,0.));
#39370=CARTESIAN_POINT('',(3.85054988729471,-1.,-1.67727921511438));
#39371=CARTESIAN_POINT('Ctrl Pts',(3.38171594275687,-1.,-1.62064718014256));
#39372=CARTESIAN_POINT('Ctrl Pts',(3.38173802621242,-1.,-1.62069086551626));
#39373=CARTESIAN_POINT('Ctrl Pts',(3.38187506457001,-1.,-1.62083271136059));
#39374=CARTESIAN_POINT('Ctrl Pts',(3.38243080602536,-1.,-1.62118047294574));
#39375=CARTESIAN_POINT('Ctrl Pts',(3.3839428576331,-1.,-1.62192472202795));
#39376=CARTESIAN_POINT('Ctrl Pts',(3.38715832178929,-1.,-1.62332788556183));
#39377=CARTESIAN_POINT('Ctrl Pts',(3.39206617497078,-1.,-1.62533996116793));
#39378=CARTESIAN_POINT('Ctrl Pts',(3.39818605298342,-1.,-1.62774916464571));
#39379=CARTESIAN_POINT('Ctrl Pts',(3.40519422740596,-1.,-1.63041148964996));
#39380=CARTESIAN_POINT('Ctrl Pts',(3.41272817148719,-1.,-1.63316667054156));
#39381=CARTESIAN_POINT('Ctrl Pts',(3.4204397459095,-1.,-1.63586250099804));
#39382=CARTESIAN_POINT('Ctrl Pts',(3.42804772926213,-1.,-1.6383787624689));
#39383=CARTESIAN_POINT('Ctrl Pts',(3.43540451921397,-1.,-1.64065778701952));
#39384=CARTESIAN_POINT('Ctrl Pts',(3.44250337701736,-1.,-1.64270733821042));
#39385=CARTESIAN_POINT('Ctrl Pts',(3.44942242546693,-1.,-1.64457408708059));
#39386=CARTESIAN_POINT('Ctrl Pts',(3.4562842106239,-1.,-1.64632429697506));
#39387=CARTESIAN_POINT('Ctrl Pts',(3.46321237515029,-1.,-1.64802323352752));
#39388=CARTESIAN_POINT('Ctrl Pts',(3.47028140996055,-1.,-1.64971118698285));
#39389=CARTESIAN_POINT('Ctrl Pts',(3.47749926256543,-1.,-1.65139534930353));
#39390=CARTESIAN_POINT('Ctrl Pts',(3.48483492840942,-1.,-1.65306335367762));
#39391=CARTESIAN_POINT('Ctrl Pts',(3.49223525300194,-1.,-1.65469162644476));
#39392=CARTESIAN_POINT('Ctrl Pts',(3.49964476477929,-1.,-1.65625517961583));
#39393=CARTESIAN_POINT('Ctrl Pts',(3.5070273314651,-1.,-1.65773832633617));
#39394=CARTESIAN_POINT('Ctrl Pts',(3.51437632188903,-1.,-1.65913971687324));
#39395=CARTESIAN_POINT('Ctrl Pts',(3.52170261543787,-1.,-1.66046645222266));
#39396=CARTESIAN_POINT('Ctrl Pts',(3.52902746211081,-1.,-1.66173058912365));
#39397=CARTESIAN_POINT('Ctrl Pts',(3.53637385060225,-1.,-1.66294490916113));
#39398=CARTESIAN_POINT('Ctrl Pts',(3.5437574747503,-1.,-1.66411849222334));
#39399=CARTESIAN_POINT('Ctrl Pts',(3.5511812134288,-1.,-1.66525401569004));
#39400=CARTESIAN_POINT('Ctrl Pts',(3.55864015233617,-1.,-1.66635023293121));
#39401=CARTESIAN_POINT('Ctrl Pts',(3.56612465179429,-1.,-1.66740349220308));
#39402=CARTESIAN_POINT('Ctrl Pts',(3.57362406285884,-1.,-1.66840957407299));
#39403=CARTESIAN_POINT('Ctrl Pts',(3.58113044183823,-1.,-1.66936552908228));
#39404=CARTESIAN_POINT('Ctrl Pts',(3.5886414309783,-1.,-1.67027110397602));
#39405=CARTESIAN_POINT('Ctrl Pts',(3.59615824388808,-1.,-1.67112775290706));
#39406=CARTESIAN_POINT('Ctrl Pts',(3.60368430815203,-1.,-1.67193797318598));
#39407=CARTESIAN_POINT('Ctrl Pts',(3.61122367156182,-1.,-1.67270452466968));
#39408=CARTESIAN_POINT('Ctrl Pts',(3.61877947398179,-1.,-1.67342968196223));
#39409=CARTESIAN_POINT('Ctrl Pts',(3.62635249450908,-1.,-1.67411452372265));
#39410=CARTESIAN_POINT('Ctrl Pts',(3.63394189312902,-1.,-1.67475929882962));
#39411=CARTESIAN_POINT('Ctrl Pts',(3.6415458297232,-1.,-1.6753637326484));
#39412=CARTESIAN_POINT('Ctrl Pts',(3.64916213574663,-1.,-1.6759273594669));
#39413=CARTESIAN_POINT('Ctrl Pts',(3.65678894416442,-1.,-1.67644983469459));
#39414=CARTESIAN_POINT('Ctrl Pts',(3.66442538671018,-1.,-1.67693128053153));
#39415=CARTESIAN_POINT('Ctrl Pts',(3.67207136294639,-1.,-1.67737217414901));
#39416=CARTESIAN_POINT('Ctrl Pts',(3.6797272457918,-1.,-1.67777320475872));
#39417=CARTESIAN_POINT('Ctrl Pts',(3.68739360236505,-1.,-1.67813513867973));
#39418=CARTESIAN_POINT('Ctrl Pts',(3.69507092759545,-1.,-1.67845869064304));
#39419=CARTESIAN_POINT('Ctrl Pts',(3.70275932350998,-1.,-1.6787443694862));
#39420=CARTESIAN_POINT('Ctrl Pts',(3.71045854208195,-1.,-1.67899249793398));
#39421=CARTESIAN_POINT('Ctrl Pts',(3.71816812842188,-1.,-1.6792032807165));
#39422=CARTESIAN_POINT('Ctrl Pts',(3.72588753416339,-1.,-1.67937685856627));
#39423=CARTESIAN_POINT('Ctrl Pts',(3.73361623282617,-1.,-1.67951336376434));
#39424=CARTESIAN_POINT('Ctrl Pts',(3.74135385965622,-1.,-1.67961298685316));
#39425=CARTESIAN_POINT('Ctrl Pts',(3.74910022394845,-1.,-1.67967598599665));
#39426=CARTESIAN_POINT('Ctrl Pts',(3.75685523754816,-1.,-1.67970265841379));
#39427=CARTESIAN_POINT('Ctrl Pts',(3.76461886684523,-1.,-1.67969332319322));
#39428=CARTESIAN_POINT('Ctrl Pts',(3.77239107928394,-1.,-1.67964830084946));
#39429=CARTESIAN_POINT('Ctrl Pts',(3.78017178196859,-1.,-1.67956789211943));
#39430=CARTESIAN_POINT('Ctrl Pts',(3.78796080021026,-1.,-1.67945236653175));
#39431=CARTESIAN_POINT('Ctrl Pts',(3.7957579157763,-1.,-1.67930196625204));
#39432=CARTESIAN_POINT('Ctrl Pts',(3.80356289078481,-1.,-1.67911690648128));
#39433=CARTESIAN_POINT('Ctrl Pts',(3.81137549624273,-1.,-1.67889737738311));
#39434=CARTESIAN_POINT('Ctrl Pts',(3.81919554100522,-1.,-1.67864354606363));
#39435=CARTESIAN_POINT('Ctrl Pts',(3.82702289288453,-1.,-1.67835555760094));
#39436=CARTESIAN_POINT('Ctrl Pts',(3.83485746516115,-1.,-1.67803353065273));
#39437=CARTESIAN_POINT('Ctrl Pts',(3.8411308598706,-1.,-1.67774874946867));
#39438=CARTESIAN_POINT('Ctrl Pts',(3.84583912297567,-1.,-1.67751991140661));
#39439=CARTESIAN_POINT('Ctrl Pts',(3.84897939431104,-1.,-1.6773605765671));
#39440=CARTESIAN_POINT('Ctrl Pts',(3.85054988729471,-1.,-1.67727921511438));
#39441=CARTESIAN_POINT('',(3.90876544355381,-1.,-1.53673442965256));
#39442=CARTESIAN_POINT('',(3.85054988729471,-1.,-1.67727921511438));
#39443=CARTESIAN_POINT('',(3.5372048861591,-1.,-1.24526366418208));
#39444=CARTESIAN_POINT('Ctrl Pts',(3.90876544355381,-1.,-1.53673442965256));
#39445=CARTESIAN_POINT('Ctrl Pts',(3.90771246854607,-1.,-1.53556639217742));
#39446=CARTESIAN_POINT('Ctrl Pts',(3.90560462812846,-1.,-1.53323321827311));
#39447=CARTESIAN_POINT('Ctrl Pts',(3.90243719629755,-1.,-1.5297421605556));
#39448=CARTESIAN_POINT('Ctrl Pts',(3.8982026070607,-1.,-1.52510482990784));
#39449=CARTESIAN_POINT('Ctrl Pts',(3.89289043531893,-1.,-1.51933724328609));
#39450=CARTESIAN_POINT('Ctrl Pts',(3.88755930032927,-1.,-1.51359883110181));
#39451=CARTESIAN_POINT('Ctrl Pts',(3.88220917950443,-1.,-1.50788973857719));
#39452=CARTESIAN_POINT('Ctrl Pts',(3.87684006372665,-1.,-1.50221016176766));
#39453=CARTESIAN_POINT('Ctrl Pts',(3.8714519699927,-1.,-1.4965603539944));
#39454=CARTESIAN_POINT('Ctrl Pts',(3.86604492575933,-1.,-1.49094061164604));
#39455=CARTESIAN_POINT('Ctrl Pts',(3.86061894706551,-1.,-1.48535125510102));
#39456=CARTESIAN_POINT('Ctrl Pts',(3.85517401698952,-1.,-1.47979260991063));
#39457=CARTESIAN_POINT('Ctrl Pts',(3.84971006847096,-1.,-1.47426499018467));
#39458=CARTESIAN_POINT('Ctrl Pts',(3.84422695454469,-1.,-1.46876867426375));
#39459=CARTESIAN_POINT('Ctrl Pts',(3.83872447159309,-1.,-1.46330391180621));
#39460=CARTESIAN_POINT('Ctrl Pts',(3.83320241775199,-1.,-1.45787095220763));
#39461=CARTESIAN_POINT('Ctrl Pts',(3.82766064519,-1.,-1.45247006796807));
#39462=CARTESIAN_POINT('Ctrl Pts',(3.82209910620591,-1.,-1.44710157648562));
#39463=CARTESIAN_POINT('Ctrl Pts',(3.8165179239855,-1.,-1.44176587041401));
#39464=CARTESIAN_POINT('Ctrl Pts',(3.81091737726965,-1.,-1.43646341556783));
#39465=CARTESIAN_POINT('Ctrl Pts',(3.80529775429916,-1.,-1.43119469921364));
#39466=CARTESIAN_POINT('Ctrl Pts',(3.79965923196365,-1.,-1.42596018777301));
#39467=CARTESIAN_POINT('Ctrl Pts',(3.7940017574439,-1.,-1.42076028482828));
#39468=CARTESIAN_POINT('Ctrl Pts',(3.78832489879369,-1.,-1.41559527803808));
#39469=CARTESIAN_POINT('Ctrl Pts',(3.78262780065406,-1.,-1.41046532282567));
#39470=CARTESIAN_POINT('Ctrl Pts',(3.77690952014209,-1.,-1.40537056004702));
#39471=CARTESIAN_POINT('Ctrl Pts',(3.77116930621804,-1.,-1.40031121335495));
#39472=CARTESIAN_POINT('Ctrl Pts',(3.76540689249078,-1.,-1.39528769118054));
#39473=CARTESIAN_POINT('Ctrl Pts',(3.75962280650875,-1.,-1.39030069388926));
#39474=CARTESIAN_POINT('Ctrl Pts',(3.75381861212728,-1.,-1.38535129801185));
#39475=CARTESIAN_POINT('Ctrl Pts',(3.74799617204744,-1.,-1.38044070763302));
#39476=CARTESIAN_POINT('Ctrl Pts',(3.7421569816256,-1.,-1.3755700297169));
#39477=CARTESIAN_POINT('Ctrl Pts',(3.73630145885809,-1.,-1.37074003422739));
#39478=CARTESIAN_POINT('Ctrl Pts',(3.73042829011293,-1.,-1.36595093298674));
#39479=CARTESIAN_POINT('Ctrl Pts',(3.72453364678279,-1.,-1.36120211416354));
#39480=CARTESIAN_POINT('Ctrl Pts',(3.71861271513318,-1.,-1.35649266705038));
#39481=CARTESIAN_POINT('Ctrl Pts',(3.71266130563061,-1.,-1.35182193384426));
#39482=CARTESIAN_POINT('Ctrl Pts',(3.7066775318825,-1.,-1.34719008463535));
#39483=CARTESIAN_POINT('Ctrl Pts',(3.70066324015112,-1.,-1.3425986075293));
#39484=CARTESIAN_POINT('Ctrl Pts',(3.69462613305692,-1.,-1.33805103398214));
#39485=CARTESIAN_POINT('Ctrl Pts',(3.68857672413013,-1.,-1.33355191034515));
#39486=CARTESIAN_POINT('Ctrl Pts',(3.68252441182534,-1.,-1.32910547072734));
#39487=CARTESIAN_POINT('Ctrl Pts',(3.67647355257906,-1.,-1.32471430856413));
#39488=CARTESIAN_POINT('Ctrl Pts',(3.67042021752668,-1.,-1.3203782813777));
#39489=CARTESIAN_POINT('Ctrl Pts',(3.66434688899822,-1.,-1.31609271239922));
#39490=CARTESIAN_POINT('Ctrl Pts',(3.65822827358655,-1.,-1.31185038411231));
#39491=CARTESIAN_POINT('Ctrl Pts',(3.65204081987101,-1.,-1.30764479590051));
#39492=CARTESIAN_POINT('Ctrl Pts',(3.64577181380125,-1.,-1.30347327603778));
#39493=CARTESIAN_POINT('Ctrl Pts',(3.6394268987279,-1.,-1.29933955906463));
#39494=CARTESIAN_POINT('Ctrl Pts',(3.63304271630995,-1.,-1.29525810207744));
#39495=CARTESIAN_POINT('Ctrl Pts',(3.62667616004299,-1.,-1.29125046021853));
#39496=CARTESIAN_POINT('Ctrl Pts',(3.62038148492295,-1.,-1.2873375502936));
#39497=CARTESIAN_POINT('Ctrl Pts',(3.61418935913793,-1.,-1.28353255117754));
#39498=CARTESIAN_POINT('Ctrl Pts',(3.60808907746372,-1.,-1.27983492861703));
#39499=CARTESIAN_POINT('Ctrl Pts',(3.60199947736404,-1.,-1.27622049908664));
#39500=CARTESIAN_POINT('Ctrl Pts',(3.59578698050164,-1.,-1.27264798379365));
#39501=CARTESIAN_POINT('Ctrl Pts',(3.5893180784647,-1.,-1.26907758484766));
#39502=CARTESIAN_POINT('Ctrl Pts',(3.58250452868699,-1.,-1.26548706249891));
#39503=CARTESIAN_POINT('Ctrl Pts',(3.5753456065164,-1.,-1.26188667142784));
#39504=CARTESIAN_POINT('Ctrl Pts',(3.56798645995025,-1.,-1.25834000485626));
#39505=CARTESIAN_POINT('Ctrl Pts',(3.56071094990825,-1.,-1.25496090899873));
#39506=CARTESIAN_POINT('Ctrl Pts',(3.5538728741862,-1.,-1.25188792940508));
#39507=CARTESIAN_POINT('Ctrl Pts',(3.54784190282889,-1.,-1.24926408627938));
#39508=CARTESIAN_POINT('Ctrl Pts',(3.54294877426113,-1.,-1.2472164623202));
#39509=CARTESIAN_POINT('Ctrl Pts',(3.53968291129942,-1.,-1.24593497225964));
#39510=CARTESIAN_POINT('Ctrl Pts',(3.53808746578052,-1.,-1.2453920538873));
#39511=CARTESIAN_POINT('Ctrl Pts',(3.53744859265385,-1.,-1.24524498991133));
#39512=CARTESIAN_POINT('Ctrl Pts',(3.53725139174402,-1.,-1.24524838931864));
#39513=CARTESIAN_POINT('Ctrl Pts',(3.5372048861591,-1.,-1.24526366418208));
#39514=CARTESIAN_POINT('',(3.59360648251021,-1.,-1.071677399622));
#39515=CARTESIAN_POINT('Origin',(0.,-1.,0.));
#39516=CARTESIAN_POINT('',(4.06552750530042,-1.,-1.05427041296137));
#39517=CARTESIAN_POINT('Ctrl Pts',(3.59360648251021,-1.,-1.071677399622));
#39518=CARTESIAN_POINT('Ctrl Pts',(3.59363512797985,-1.,-1.07171709254271));
#39519=CARTESIAN_POINT('Ctrl Pts',(3.59379266874663,-1.,-1.07183575450716));
#39520=CARTESIAN_POINT('Ctrl Pts',(3.59439597,-1.,-1.07209229745284));
#39521=CARTESIAN_POINT('Ctrl Pts',(3.59600583195037,-1.,-1.07259084660947));
#39522=CARTESIAN_POINT('Ctrl Pts',(3.59940121154383,-1.,-1.0734737254567));
#39523=CARTESIAN_POINT('Ctrl Pts',(3.6045633988796,-1.,-1.0746932716863));
#39524=CARTESIAN_POINT('Ctrl Pts',(3.61098481349577,-1.,-1.07611545402841));
#39525=CARTESIAN_POINT('Ctrl Pts',(3.61832318504957,-1.,-1.07764868137729));
#39526=CARTESIAN_POINT('Ctrl Pts',(3.62619537902616,-1.,-1.07919137290816));
#39527=CARTESIAN_POINT('Ctrl Pts',(3.63423373196602,-1.,-1.08064765719887));
#39528=CARTESIAN_POINT('Ctrl Pts',(3.64214167843595,-1.,-1.08194278850972));
#39529=CARTESIAN_POINT('Ctrl Pts',(3.64976441208197,-1.,-1.08304289898577));
#39530=CARTESIAN_POINT('Ctrl Pts',(3.65709649161004,-1.,-1.08395671077761));
#39531=CARTESIAN_POINT('Ctrl Pts',(3.66422237895256,-1.,-1.0847180992287));
#39532=CARTESIAN_POINT('Ctrl Pts',(3.67127347729632,-1.,-1.0853733414448));
#39533=CARTESIAN_POINT('Ctrl Pts',(3.67838211685148,-1.,-1.08596755755768));
#39534=CARTESIAN_POINT('Ctrl Pts',(3.68562817420864,-1.,-1.08652888882609));
#39535=CARTESIAN_POINT('Ctrl Pts',(3.69302062410229,-1.,-1.08706319540292));
#39536=CARTESIAN_POINT('Ctrl Pts',(3.70052690909884,-1.,-1.08756311291324));
#39537=CARTESIAN_POINT('Ctrl Pts',(3.70809084139476,-1.,-1.0880136731219));
#39538=CARTESIAN_POINT('Ctrl Pts',(3.71565372339063,-1.,-1.08839887334777));
#39539=CARTESIAN_POINT('Ctrl Pts',(3.72317741369364,-1.,-1.08870887220072));
#39540=CARTESIAN_POINT('Ctrl Pts',(3.73065515162949,-1.,-1.08894337390925));
#39541=CARTESIAN_POINT('Ctrl Pts',(3.73809879348209,-1.,-1.08910769013288));
#39542=CARTESIAN_POINT('Ctrl Pts',(3.74553121371745,-1.,-1.08921040494013));
#39543=CARTESIAN_POINT('Ctrl Pts',(3.75297711748138,-1.,-1.08926054632927));
#39544=CARTESIAN_POINT('Ctrl Pts',(3.76045342580226,-1.,-1.08926462734287));
#39545=CARTESIAN_POINT('Ctrl Pts',(3.76796340094469,-1.,-1.08922484204263));
#39546=CARTESIAN_POINT('Ctrl Pts',(3.7755019940944,-1.,-1.08914072791275));
#39547=CARTESIAN_POINT('Ctrl Pts',(3.78305911299511,-1.,-1.08901018614638));
#39548=CARTESIAN_POINT('Ctrl Pts',(3.79062357974401,-1.,-1.08883071512097));
#39549=CARTESIAN_POINT('Ctrl Pts',(3.79818708705252,-1.,-1.08860064435776));
#39550=CARTESIAN_POINT('Ctrl Pts',(3.80574726657656,-1.,-1.08832009255378));
#39551=CARTESIAN_POINT('Ctrl Pts',(3.81330554446324,-1.,-1.08799030610861));
#39552=CARTESIAN_POINT('Ctrl Pts',(3.82086569676321,-1.,-1.08761321539442));
#39553=CARTESIAN_POINT('Ctrl Pts',(3.82843215316985,-1.,-1.08719091307558));
#39554=CARTESIAN_POINT('Ctrl Pts',(3.83600837071702,-1.,-1.08672515456901));
#39555=CARTESIAN_POINT('Ctrl Pts',(3.84359528764934,-1.,-1.08621688337601));
#39556=CARTESIAN_POINT('Ctrl Pts',(3.85119211322732,-1.,-1.08566647671838));
#39557=CARTESIAN_POINT('Ctrl Pts',(3.85879698702511,-1.,-1.08507395120054));
#39558=CARTESIAN_POINT('Ctrl Pts',(3.86640769434269,-1.,-1.08443918607926));
#39559=CARTESIAN_POINT('Ctrl Pts',(3.87402233722563,-1.,-1.0837621330751));
#39560=CARTESIAN_POINT('Ctrl Pts',(3.88164007721365,-1.,-1.08304304871042));
#39561=CARTESIAN_POINT('Ctrl Pts',(3.88926088975182,-1.,-1.08228241999363));
#39562=CARTESIAN_POINT('Ctrl Pts',(3.89688525098408,-1.,-1.08148086931373));
#39563=CARTESIAN_POINT('Ctrl Pts',(3.90451384092564,-1.,-1.08063906483823));
#39564=CARTESIAN_POINT('Ctrl Pts',(3.91214726022096,-1.,-1.0797576350746));
#39565=CARTESIAN_POINT('Ctrl Pts',(3.91978568924062,-1.,-1.07883706663524));
#39566=CARTESIAN_POINT('Ctrl Pts',(3.92742893349684,-1.,-1.07787771707155));
#39567=CARTESIAN_POINT('Ctrl Pts',(3.93507657572743,-1.,-1.07687985975348));
#39568=CARTESIAN_POINT('Ctrl Pts',(3.94272809633271,-1.,-1.07584371946428));
#39569=CARTESIAN_POINT('Ctrl Pts',(3.95038299600754,-1.,-1.07476950921607));
#39570=CARTESIAN_POINT('Ctrl Pts',(3.95804094429606,-1.,-1.07365747426551));
#39571=CARTESIAN_POINT('Ctrl Pts',(3.96570179322681,-1.,-1.07250789943095));
#39572=CARTESIAN_POINT('Ctrl Pts',(3.97336550222571,-1.,-1.07132109206252));
#39573=CARTESIAN_POINT('Ctrl Pts',(3.98103208801289,-1.,-1.07009737257815));
#39574=CARTESIAN_POINT('Ctrl Pts',(3.98870156857298,-1.,-1.06883706263912));
#39575=CARTESIAN_POINT('Ctrl Pts',(3.99637389919958,-1.,-1.06754047381188));
#39576=CARTESIAN_POINT('Ctrl Pts',(4.00404894951804,-1.,-1.06620789963406));
#39577=CARTESIAN_POINT('Ctrl Pts',(4.0117265418656,-1.,-1.06483961342894));
#39578=CARTESIAN_POINT('Ctrl Pts',(4.0194064749539,-1.,-1.06343586496094));
#39579=CARTESIAN_POINT('Ctrl Pts',(4.02708855235732,-1.,-1.06199687787488));
#39580=CARTESIAN_POINT('Ctrl Pts',(4.03477261142549,-1.,-1.06052284712114));
#39581=CARTESIAN_POINT('Ctrl Pts',(4.04245854429333,-1.,-1.0590139366704));
#39582=CARTESIAN_POINT('Ctrl Pts',(4.05014628387112,-1.,-1.05747027728537));
#39583=CARTESIAN_POINT('Ctrl Pts',(4.05629789308941,-1.,-1.0562076270849));
#39584=CARTESIAN_POINT('Ctrl Pts',(4.06091239150293,-1.,-1.05524507177901));
#39585=CARTESIAN_POINT('Ctrl Pts',(4.06398907542679,-1.,-1.05459645194934));
#39586=CARTESIAN_POINT('Ctrl Pts',(4.06552750530042,-1.,-1.05427041296137));
#39587=CARTESIAN_POINT('',(4.10104028313088,-1.,-0.906349047628866));
#39588=CARTESIAN_POINT('',(4.06552750530042,-1.,-1.05427041296137));
#39589=CARTESIAN_POINT('',(3.68845817949586,-1.,-0.676591647975429));
#39590=CARTESIAN_POINT('Ctrl Pts',(4.10104028313088,-1.,-0.906349047628866));
#39591=CARTESIAN_POINT('Ctrl Pts',(4.09981755067523,-1.,-0.905360112215337));
#39592=CARTESIAN_POINT('Ctrl Pts',(4.09737067245935,-1.,-0.903385402441588));
#39593=CARTESIAN_POINT('Ctrl Pts',(4.09369611522387,-1.,-0.900432820941675));
#39594=CARTESIAN_POINT('Ctrl Pts',(4.08878822246833,-1.,-0.896515019231334));
#39595=CARTESIAN_POINT('Ctrl Pts',(4.08263920304799,-1.,-0.891649447916278));
#39596=CARTESIAN_POINT('Ctrl Pts',(4.07647601773635,-1.,-0.886815658358501));
#39597=CARTESIAN_POINT('Ctrl Pts',(4.07029866694192,-1.,-0.882013797525692));
#39598=CARTESIAN_POINT('Ctrl Pts',(4.06410717232905,-1.,-0.877244060485838));
#39599=CARTESIAN_POINT('Ctrl Pts',(4.0579015903134,-1.,-0.872506694782446));
#39600=CARTESIAN_POINT('Ctrl Pts',(4.05168199437909,-1.,-0.867801988859918));
#39601=CARTESIAN_POINT('Ctrl Pts',(4.04544845048584,-1.,-0.863130256643259));
#39602=CARTESIAN_POINT('Ctrl Pts',(4.03920099284773,-1.,-0.858491822322828));
#39603=CARTESIAN_POINT('Ctrl Pts',(4.03293960436756,-1.,-0.853887006631755));
#39604=CARTESIAN_POINT('Ctrl Pts',(4.02666418343164,-1.,-0.849316107474245));
#39605=CARTESIAN_POINT('Ctrl Pts',(4.02037456798441,-1.,-0.844779403287746));
#39606=CARTESIAN_POINT('Ctrl Pts',(4.01407059766103,-1.,-0.840277171975855));
#39607=CARTESIAN_POINT('Ctrl Pts',(4.00775216907856,-1.,-0.835809705809646));
#39608=CARTESIAN_POINT('Ctrl Pts',(4.00141928477507,-1.,-0.831377325741623));
#39609=CARTESIAN_POINT('Ctrl Pts',(3.99507212784431,-1.,-0.82698040032079));
#39610=CARTESIAN_POINT('Ctrl Pts',(3.98871104646485,-1.,-0.822619346022119));
#39611=CARTESIAN_POINT('Ctrl Pts',(3.98233640155404,-1.,-0.818294599022294));
#39612=CARTESIAN_POINT('Ctrl Pts',(3.97594844078811,-1.,-0.814006592328844));
#39613=CARTESIAN_POINT('Ctrl Pts',(3.96954717513232,-1.,-0.809755732818091));
#39614=CARTESIAN_POINT('Ctrl Pts',(3.96313222295815,-1.,-0.805542372178362));
#39615=CARTESIAN_POINT('Ctrl Pts',(3.95670276375108,-1.,-0.80136679772705));
#39616=CARTESIAN_POINT('Ctrl Pts',(3.95025788827136,-1.,-0.797229296085316));
#39617=CARTESIAN_POINT('Ctrl Pts',(3.94379688971283,-1.,-0.793130205640961));
#39618=CARTESIAN_POINT('Ctrl Pts',(3.93731956885676,-1.,-0.789069971469333));
#39619=CARTESIAN_POINT('Ctrl Pts',(3.93082655631789,-1.,-0.785049202786508));
#39620=CARTESIAN_POINT('Ctrl Pts',(3.92431956510441,-1.,-0.781068718228451));
#39621=CARTESIAN_POINT('Ctrl Pts',(3.9178006233448,-1.,-0.777129415664956));
#39622=CARTESIAN_POINT('Ctrl Pts',(3.91127138115243,-1.,-0.773232154506321));
#39623=CARTESIAN_POINT('Ctrl Pts',(3.90473237182633,-1.,-0.769377629847874));
#39624=CARTESIAN_POINT('Ctrl Pts',(3.89818233104378,-1.,-0.765566256401296));
#39625=CARTESIAN_POINT('Ctrl Pts',(3.89161738162245,-1.,-0.76179802879397));
#39626=CARTESIAN_POINT('Ctrl Pts',(3.88503262662689,-1.,-0.758072800564801));
#39627=CARTESIAN_POINT('Ctrl Pts',(3.87842382520065,-1.,-0.754390577396857));
#39628=CARTESIAN_POINT('Ctrl Pts',(3.87178914078374,-1.,-0.750751822383028));
#39629=CARTESIAN_POINT('Ctrl Pts',(3.86513062969889,-1.,-0.747157716488871));
#39630=CARTESIAN_POINT('Ctrl Pts',(3.85845645217594,-1.,-0.743610542737013));
#39631=CARTESIAN_POINT('Ctrl Pts',(3.85177770351215,-1.,-0.740113146827137));
#39632=CARTESIAN_POINT('Ctrl Pts',(3.84510432881213,-1.,-0.736668240497118));
#39633=CARTESIAN_POINT('Ctrl Pts',(3.83844103658009,-1.,-0.733277703756078));
#39634=CARTESIAN_POINT('Ctrl Pts',(3.83178392403383,-1.,-0.729942010490168));
#39635=CARTESIAN_POINT('Ctrl Pts',(3.82511495756713,-1.,-0.726659281876664));
#39636=CARTESIAN_POINT('Ctrl Pts',(3.81840802610835,-1.,-0.723426346019423));
#39637=CARTESIAN_POINT('Ctrl Pts',(3.81163885127344,-1.,-0.720240466589236));
#39638=CARTESIAN_POINT('Ctrl Pts',(3.80479445759309,-1.,-0.717100993669115));
#39639=CARTESIAN_POINT('Ctrl Pts',(3.79788100314975,-1.,-0.714010733006641));
#39640=CARTESIAN_POINT('Ctrl Pts',(3.79093694007094,-1.,-0.710978231689017));
#39641=CARTESIAN_POINT('Ctrl Pts',(3.78402183336605,-1.,-0.708015879375459));
#39642=CARTESIAN_POINT('Ctrl Pts',(3.77719254217129,-1.,-0.705135847999817));
#39643=CARTESIAN_POINT('Ctrl Pts',(3.77048141872872,-1.,-0.702346356621552));
#39644=CARTESIAN_POINT('Ctrl Pts',(3.76387780603759,-1.,-0.699648552230917));
#39645=CARTESIAN_POINT('Ctrl Pts',(3.75729775767023,-1.,-0.697031245659744));
#39646=CARTESIAN_POINT('Ctrl Pts',(3.75060288243455,-1.,-0.694474562581493));
#39647=CARTESIAN_POINT('Ctrl Pts',(3.74365508986712,-1.,-0.69196008040082));
#39648=CARTESIAN_POINT('Ctrl Pts',(3.73636374475077,-1.,-0.689479637354814));
#39649=CARTESIAN_POINT('Ctrl Pts',(3.72872973554051,-1.,-0.687043475232355));
#39650=CARTESIAN_POINT('Ctrl Pts',(3.7209063713926,-1.,-0.684691698167848));
#39651=CARTESIAN_POINT('Ctrl Pts',(3.71319182789943,-1.,-0.68249234510893));
#39652=CARTESIAN_POINT('Ctrl Pts',(3.70595722031785,-1.,-0.680526909710877));
#39653=CARTESIAN_POINT('Ctrl Pts',(3.69959004073005,-1.,-0.678878822226027));
#39654=CARTESIAN_POINT('Ctrl Pts',(3.69443683573598,-1.,-0.677621861865498));
#39655=CARTESIAN_POINT('Ctrl Pts',(3.69101071175464,-1.,-0.676867042599402));
#39656=CARTESIAN_POINT('Ctrl Pts',(3.68934997767243,-1.,-0.676580391119396));
#39657=CARTESIAN_POINT('Ctrl Pts',(3.68869596425969,-1.,-0.676535079520807));
#39658=CARTESIAN_POINT('Ctrl Pts',(3.68850172300477,-1.,-0.676569286094607));
#39659=CARTESIAN_POINT('Ctrl Pts',(3.68845817949586,-1.,-0.676591647975429));
#39660=CARTESIAN_POINT('',(3.71701050416802,-1.,-0.496319364829374));
#39661=CARTESIAN_POINT('Origin',(0.,-1.,0.));
#39662=CARTESIAN_POINT('',(4.18039834341342,-1.,-0.40530197431835));
#39663=CARTESIAN_POINT('Ctrl Pts',(3.71701050416802,-1.,-0.496319364829374));
#39664=CARTESIAN_POINT('Ctrl Pts',(3.71704500630521,-1.,-0.496354087925646));
#39665=CARTESIAN_POINT('Ctrl Pts',(3.71721917030465,-1.,-0.496446644158827));
#39666=CARTESIAN_POINT('Ctrl Pts',(3.71785517607694,-1.,-0.496605651526314));
#39667=CARTESIAN_POINT('Ctrl Pts',(3.7195232082259,-1.,-0.496846224822535));
#39668=CARTESIAN_POINT('Ctrl Pts',(3.72301489774241,-1.,-0.497187079575795));
#39669=CARTESIAN_POINT('Ctrl Pts',(3.72830430904794,-1.,-0.49758406715328));
#39670=CARTESIAN_POINT('Ctrl Pts',(3.73486914372834,-1.,-0.497984209510496));
#39671=CARTESIAN_POINT('Ctrl Pts',(3.74235701735109,-1.,-0.498350586058176));
#39672=CARTESIAN_POINT('Ctrl Pts',(3.75037362168103,-1.,-0.498642802042929));
#39673=CARTESIAN_POINT('Ctrl Pts',(3.75854082221127,-1.,-0.498823681615513));
#39674=CARTESIAN_POINT('Ctrl Pts',(3.76655401191144,-1.,-0.498865792335185));
#39675=CARTESIAN_POINT('Ctrl Pts',(3.77425499225089,-1.,-0.498759900365687));
#39676=CARTESIAN_POINT('Ctrl Pts',(3.78163975337189,-1.,-0.498515471679379));
#39677=CARTESIAN_POINT('Ctrl Pts',(3.78879701661152,-1.,-0.498152751800819));
#39678=CARTESIAN_POINT('Ctrl Pts',(3.79586380669959,-1.,-0.497696892100581));
#39679=CARTESIAN_POINT('Ctrl Pts',(3.80297788298545,-1.,-0.497171756201091));
#39680=CARTESIAN_POINT('Ctrl Pts',(3.81022254090909,-1.,-0.496592643443789));
#39681=CARTESIAN_POINT('Ctrl Pts',(3.81760756144099,-1.,-0.495963937875572));
#39682=CARTESIAN_POINT('Ctrl Pts',(3.82509963594156,-1.,-0.495283458893903));
#39683=CARTESIAN_POINT('Ctrl Pts',(3.8326409268245,-1.,-0.494545212256426));
#39684=CARTESIAN_POINT('Ctrl Pts',(3.84017095578438,-1.,-0.493742574629117));
#39685=CARTESIAN_POINT('Ctrl Pts',(3.84765051147965,-1.,-0.492871792414095));
#39686=CARTESIAN_POINT('Ctrl Pts',(3.85507287020223,-1.,-0.49193363108376));
#39687=CARTESIAN_POINT('Ctrl Pts',(3.86245057319215,-1.,-0.490931482170849));
#39688=CARTESIAN_POINT('Ctrl Pts',(3.86980755613694,-1.,-0.4898702457049));
#39689=CARTESIAN_POINT('Ctrl Pts',(3.87716963231115,-1.,-0.488754973798281));
#39690=CARTESIAN_POINT('Ctrl Pts',(3.88455453328156,-1.,-0.487589452275179));
#39691=CARTESIAN_POINT('Ctrl Pts',(3.89196582437574,-1.,-0.486375337854134));
#39692=CARTESIAN_POINT('Ctrl Pts',(3.89939844658529,-1.,-0.485112963522246));
#39693=CARTESIAN_POINT('Ctrl Pts',(3.90684210358063,-1.,-0.483801835089161));
#39694=CARTESIAN_POINT('Ctrl Pts',(3.91428536373749,-1.,-0.482441230340709));
#39695=CARTESIAN_POINT('Ctrl Pts',(3.92171976072334,-1.,-0.481030798910735));
#39696=CARTESIAN_POINT('Ctrl Pts',(3.92914297392067,-1.,-0.479571028525566));
#39697=CARTESIAN_POINT('Ctrl Pts',(3.93655660689819,-1.,-0.478062927140957));
#39698=CARTESIAN_POINT('Ctrl Pts',(3.94396469119385,-1.,-0.476507810658535));
#39699=CARTESIAN_POINT('Ctrl Pts',(3.95137192932898,-1.,-0.474907053021791));
#39700=CARTESIAN_POINT('Ctrl Pts',(3.95878201038332,-1.,-0.473261847236296));
#39701=CARTESIAN_POINT('Ctrl Pts',(3.96619600864626,-1.,-0.471572978413494));
#39702=CARTESIAN_POINT('Ctrl Pts',(3.97361320212413,-1.,-0.469840942829878));
#39703=CARTESIAN_POINT('Ctrl Pts',(3.98103175589349,-1.,-0.46806604792014));
#39704=CARTESIAN_POINT('Ctrl Pts',(3.98844946363258,-1.,-0.466248520883035));
#39705=CARTESIAN_POINT('Ctrl Pts',(3.99586444320134,-1.,-0.464388610938995));
#39706=CARTESIAN_POINT('Ctrl Pts',(4.00327590659129,-1.,-0.462486702616252));
#39707=CARTESIAN_POINT('Ctrl Pts',(4.01068390573469,-1.,-0.460543280768577));
#39708=CARTESIAN_POINT('Ctrl Pts',(4.01808900827647,-1.,-0.458558885637001));
#39709=CARTESIAN_POINT('Ctrl Pts',(4.02549199038414,-1.,-0.456534070784968));
#39710=CARTESIAN_POINT('Ctrl Pts',(4.03289354362745,-1.,-0.454469363020496));
#39711=CARTESIAN_POINT('Ctrl Pts',(4.0402939222793,-1.,-0.452365214748779));
#39712=CARTESIAN_POINT('Ctrl Pts',(4.0476929901797,-1.,-0.450222009543774));
#39713=CARTESIAN_POINT('Ctrl Pts',(4.05509037796815,-1.,-0.448040082683977));
#39714=CARTESIAN_POINT('Ctrl Pts',(4.06248560760596,-1.,-0.445819737468478));
#39715=CARTESIAN_POINT('Ctrl Pts',(4.0698782192577,-1.,-0.443561262395408));
#39716=CARTESIAN_POINT('Ctrl Pts',(4.07726792490256,-1.,-0.441264951396587));
#39717=CARTESIAN_POINT('Ctrl Pts',(4.08465462294625,-1.,-0.438931108931614));
#39718=CARTESIAN_POINT('Ctrl Pts',(4.09203832139439,-1.,-0.436560044913814));
#39719=CARTESIAN_POINT('Ctrl Pts',(4.09941908688567,-1.,-0.434152073200643));
#39720=CARTESIAN_POINT('Ctrl Pts',(4.10679698750219,-1.,-0.431707508679772));
#39721=CARTESIAN_POINT('Ctrl Pts',(4.1141720278277,-1.,-0.429226666075373));
#39722=CARTESIAN_POINT('Ctrl Pts',(4.1215441250121,-1.,-0.426709855706243));
#39723=CARTESIAN_POINT('Ctrl Pts',(4.1289131463371,-1.,-0.424157375323155));
#39724=CARTESIAN_POINT('Ctrl Pts',(4.13627893206433,-1.,-0.421569503103971));
#39725=CARTESIAN_POINT('Ctrl Pts',(4.14364132317223,-1.,-0.4189464906678));
#39726=CARTESIAN_POINT('Ctrl Pts',(4.15100018950989,-1.,-0.416288556008986));
#39727=CARTESIAN_POINT('Ctrl Pts',(4.1583554501909,-1.,-0.413595877953269));
#39728=CARTESIAN_POINT('Ctrl Pts',(4.16570705940731,-1.,-0.410868596148614));
#39729=CARTESIAN_POINT('Ctrl Pts',(4.17158541009947,-1.,-0.408659167570153));
#39730=CARTESIAN_POINT('Ctrl Pts',(4.17599251955585,-1.,-0.406986596326603));
#39731=CARTESIAN_POINT('Ctrl Pts',(4.17892985789908,-1.,-0.405864662679631));
#39732=CARTESIAN_POINT('Ctrl Pts',(4.18039834341342,-1.,-0.40530197431835));
#39733=CARTESIAN_POINT('',(4.1923339003649,-1.,-0.253646344052521));
#39734=CARTESIAN_POINT('',(4.18039834341342,-1.,-0.40530197431835));
#39735=CARTESIAN_POINT('',(3.74888939116255,-1.,-0.0912596999166826));
#39736=CARTESIAN_POINT('Ctrl Pts',(4.1923339003649,-1.,-0.253646344052521));
#39737=CARTESIAN_POINT('Ctrl Pts',(4.19097151819241,-1.,-0.252860861572566));
#39738=CARTESIAN_POINT('Ctrl Pts',(4.18824585244066,-1.,-0.251293239837693));
#39739=CARTESIAN_POINT('Ctrl Pts',(4.18415464959491,-1.,-0.248951836910964));
#39740=CARTESIAN_POINT('Ctrl Pts',(4.17869430192868,-1.,-0.245850033418584));
#39741=CARTESIAN_POINT('Ctrl Pts',(4.17185984409533,-1.,-0.242006283923912));
#39742=CARTESIAN_POINT('Ctrl Pts',(4.1650163665385,-1.,-0.238196140933977));
#39743=CARTESIAN_POINT('Ctrl Pts',(4.1581638926525,-1.,-0.234419749543143));
#39744=CARTESIAN_POINT('Ctrl Pts',(4.15130247435029,-1.,-0.230677299028738));
#39745=CARTESIAN_POINT('Ctrl Pts',(4.14443220607733,-1.,-0.226969025061244));
#39746=CARTESIAN_POINT('Ctrl Pts',(4.13755320553563,-1.,-0.223295201038384));
#39747=CARTESIAN_POINT('Ctrl Pts',(4.13066558698156,-1.,-0.219656126701852));
#39748=CARTESIAN_POINT('Ctrl Pts',(4.12376943492249,-1.,-0.216052116898425));
#39749=CARTESIAN_POINT('Ctrl Pts',(4.11686478264545,-1.,-0.212483491087068));
#39750=CARTESIAN_POINT('Ctrl Pts',(4.10995157639026,-1.,-0.208950559400172));
#39751=CARTESIAN_POINT('Ctrl Pts',(4.10302969965374,-1.,-0.205453622198233));
#39752=CARTESIAN_POINT('Ctrl Pts',(4.09609903751912,-1.,-0.201992979049985));
#39753=CARTESIAN_POINT('Ctrl Pts',(4.08915953359753,-1.,-0.198568934800811));
#39754=CARTESIAN_POINT('Ctrl Pts',(4.08221124060385,-1.,-0.195181806054714));
#39755=CARTESIAN_POINT('Ctrl Pts',(4.07525439703137,-1.,-0.191831928181081));
#39756=CARTESIAN_POINT('Ctrl Pts',(4.06828941192308,-1.,-0.188519658060256));
#39757=CARTESIAN_POINT('Ctrl Pts',(4.06131670998589,-1.,-0.185245370038948));
#39758=CARTESIAN_POINT('Ctrl Pts',(4.05433660358402,-1.,-0.18200945304855));
#39759=CARTESIAN_POINT('Ctrl Pts',(4.04734916719722,-1.,-0.178812307240716));
#39760=CARTESIAN_POINT('Ctrl Pts',(4.04035407891161,-1.,-0.175654339673758));
#39761=CARTESIAN_POINT('Ctrl Pts',(4.03335057326093,-1.,-0.172535962484467));
#39762=CARTESIAN_POINT('Ctrl Pts',(4.0263377970371,-1.,-0.169457601001653));
#39763=CARTESIAN_POINT('Ctrl Pts',(4.01931510507143,-1.,-0.166419700015848));
#39764=CARTESIAN_POINT('Ctrl Pts',(4.01228237022301,-1.,-0.163422730287459));
#39765=CARTESIAN_POINT('Ctrl Pts',(4.00524031064509,-1.,-0.160467194882219));
#39766=CARTESIAN_POINT('Ctrl Pts',(3.99819074631874,-1.,-0.15755363438381));
#39767=CARTESIAN_POINT('Ctrl Pts',(3.99113582086059,-1.,-0.154682618338563));
#39768=CARTESIAN_POINT('Ctrl Pts',(3.9840772985098,-1.,-0.151854737441406));
#39769=CARTESIAN_POINT('Ctrl Pts',(3.97701581473643,-1.,-0.149070594803544));
#39770=CARTESIAN_POINT('Ctrl Pts',(3.96995018565891,-1.,-0.146330797814514));
#39771=CARTESIAN_POINT('Ctrl Pts',(3.96287658098896,-1.,-0.143635947692791));
#39772=CARTESIAN_POINT('Ctrl Pts',(3.95579014116899,-1.,-0.140986665829937));
#39773=CARTESIAN_POINT('Ctrl Pts',(3.94868667844355,-1.,-0.138383621255159));
#39774=CARTESIAN_POINT('Ctrl Pts',(3.94156445130744,-1.,-0.135827558661188));
#39775=CARTESIAN_POINT('Ctrl Pts',(3.93442567551035,-1.,-0.13331932279419));
#39776=CARTESIAN_POINT('Ctrl Pts',(3.9272787679596,-1.,-0.130859892027799));
#39777=CARTESIAN_POINT('Ctrl Pts',(3.92013513251642,-1.,-0.128450341339528));
#39778=CARTESIAN_POINT('Ctrl Pts',(3.91300501605392,-1.,-0.126091793324137));
#39779=CARTESIAN_POINT('Ctrl Pts',(3.90589336320508,-1.,-0.123785368272378));
#39780=CARTESIAN_POINT('Ctrl Pts',(3.89879639336952,-1.,-0.121532144765723));
#39781=CARTESIAN_POINT('Ctrl Pts',(3.89169600105201,-1.,-0.119333088190418));
#39782=CARTESIAN_POINT('Ctrl Pts',(3.88456590045767,-1.,-0.117189150373144));
#39783=CARTESIAN_POINT('Ctrl Pts',(3.87738168405343,-1.,-0.11510142664947));
#39784=CARTESIAN_POINT('Ctrl Pts',(3.87013043445014,-1.,-0.113071304914562));
#39785=CARTESIAN_POINT('Ctrl Pts',(3.86281867282965,-1.,-0.111100593036261));
#39786=CARTESIAN_POINT('Ctrl Pts',(3.855485714969,-1.,-0.109191717634944));
#39787=CARTESIAN_POINT('Ctrl Pts',(3.84819233070317,-1.,-0.107347597812184));
#39788=CARTESIAN_POINT('Ctrl Pts',(3.84099658324803,-1.,-0.105571360916569));
#39789=CARTESIAN_POINT('Ctrl Pts',(3.83393171228002,-1.,-0.103866063811623));
#39790=CARTESIAN_POINT('Ctrl Pts',(3.82698737143255,-1.,-0.102234506488457));
#39791=CARTESIAN_POINT('Ctrl Pts',(3.82007889742625,-1.,-0.100678769650632));
#39792=CARTESIAN_POINT('Ctrl Pts',(3.81306649386461,-1.,-0.0992008728096518));
#39793=CARTESIAN_POINT('Ctrl Pts',(3.80581088847809,-1.,-0.0978042222906647));
#39794=CARTESIAN_POINT('Ctrl Pts',(3.79822128513845,-1.,-0.0964949352873135));
#39795=CARTESIAN_POINT('Ctrl Pts',(3.79030016353111,-1.,-0.0952829885100805));
#39796=CARTESIAN_POINT('Ctrl Pts',(3.782205218991,-1.,-0.0941840095090818));
#39797=CARTESIAN_POINT('Ctrl Pts',(3.77424159971059,-1.,-0.0932185546203182));
#39798=CARTESIAN_POINT('Ctrl Pts',(3.76678860031841,-1.,-0.0924090589602695));
#39799=CARTESIAN_POINT('Ctrl Pts',(3.76024199359303,-1.,-0.0917773084998339));
#39800=CARTESIAN_POINT('Ctrl Pts',(3.75495560118212,-1.,-0.0913419622736402));
#39801=CARTESIAN_POINT('Ctrl Pts',(3.75145357872422,-1.,-0.091132399957443));
#39802=CARTESIAN_POINT('Ctrl Pts',(3.74976844886346,-1.,-0.0911090736805514));
#39803=CARTESIAN_POINT('Ctrl Pts',(3.74911539914542,-1.,-0.0911666301812821));
#39804=CARTESIAN_POINT('Ctrl Pts',(3.74892890040974,-1.,-0.0912308016421984));
#39805=CARTESIAN_POINT('Ctrl Pts',(3.74888939116255,-1.,-0.0912596999166826));
#39806=CARTESIAN_POINT('',(3.74888939116259,-1.,0.0912596999148864));
#39807=CARTESIAN_POINT('Origin',(0.,-1.,0.));
#39808=CARTESIAN_POINT('',(4.1923339003649,-1.,0.253646344052522));
#39809=CARTESIAN_POINT('Ctrl Pts',(3.74888939116259,-1.,0.0912596999148864));
#39810=CARTESIAN_POINT('Ctrl Pts',(3.74892890041021,-1.,0.0912308016409238));
#39811=CARTESIAN_POINT('Ctrl Pts',(3.74911539914664,-1.,0.091166630180643));
#39812=CARTESIAN_POINT('Ctrl Pts',(3.74976844886495,-1.,0.0911090736804577));
#39813=CARTESIAN_POINT('Ctrl Pts',(3.75145357872511,-1.,0.0911323999576149));
#39814=CARTESIAN_POINT('Ctrl Pts',(3.75495560118053,-1.,0.0913419622735858));
#39815=CARTESIAN_POINT('Ctrl Pts',(3.76024199359493,-1.,0.0917773084999013));
#39816=CARTESIAN_POINT('Ctrl Pts',(3.76678860032228,-1.,0.092409058960406));
#39817=CARTESIAN_POINT('Ctrl Pts',(3.77424159971456,-1.,0.093218554620458));
#39818=CARTESIAN_POINT('Ctrl Pts',(3.78220521899366,-1.,0.0941840095091749));
#39819=CARTESIAN_POINT('Ctrl Pts',(3.79030016353186,-1.,0.0952829885101074));
#39820=CARTESIAN_POINT('Ctrl Pts',(3.7982212851376,-1.,0.0964949352872849));
#39821=CARTESIAN_POINT('Ctrl Pts',(3.80581088847642,-1.,0.097804222290608));
#39822=CARTESIAN_POINT('Ctrl Pts',(3.81306649386293,-1.,0.0992008728095949));
#39823=CARTESIAN_POINT('Ctrl Pts',(3.82007889742512,-1.,0.100678769650595));
#39824=CARTESIAN_POINT('Ctrl Pts',(3.8269873714322,-1.,0.102234506488446));
#39825=CARTESIAN_POINT('Ctrl Pts',(3.83393171228034,-1.,0.103866063811635));
#39826=CARTESIAN_POINT('Ctrl Pts',(3.84099658324873,-1.,0.105571360916594));
#39827=CARTESIAN_POINT('Ctrl Pts',(3.84819233070391,-1.,0.107347597812209));
#39828=CARTESIAN_POINT('Ctrl Pts',(3.85548571496953,-1.,0.109191717634961));
#39829=CARTESIAN_POINT('Ctrl Pts',(3.86281867282984,-1.,0.111100593036267));
#39830=CARTESIAN_POINT('Ctrl Pts',(3.87013043445001,-1.,0.113071304914559));
#39831=CARTESIAN_POINT('Ctrl Pts',(3.87738168405308,-1.,0.115101426649461));
#39832=CARTESIAN_POINT('Ctrl Pts',(3.88456590045726,-1.,0.117189150373135));
#39833=CARTESIAN_POINT('Ctrl Pts',(3.8916960010517,-1.,0.119333088190411));
#39834=CARTESIAN_POINT('Ctrl Pts',(3.89879639336939,-1.,0.121532144765722));
#39835=CARTESIAN_POINT('Ctrl Pts',(3.90589336320515,-1.,0.12378536827238));
#39836=CARTESIAN_POINT('Ctrl Pts',(3.91300501605411,-1.,0.126091793324141));
#39837=CARTESIAN_POINT('Ctrl Pts',(3.92013513251664,-1.,0.128450341339533));
#39838=CARTESIAN_POINT('Ctrl Pts',(3.92727876795977,-1.,0.130859892027802));
#39839=CARTESIAN_POINT('Ctrl Pts',(3.93442567551042,-1.,0.133319322794191));
#39840=CARTESIAN_POINT('Ctrl Pts',(3.94156445130741,-1.,0.135827558661189));
#39841=CARTESIAN_POINT('Ctrl Pts',(3.94868667844347,-1.,0.138383621255161));
#39842=CARTESIAN_POINT('Ctrl Pts',(3.95579014116894,-1.,0.140986665829942));
#39843=CARTESIAN_POINT('Ctrl Pts',(3.96287658098896,-1.,0.143635947692799));
#39844=CARTESIAN_POINT('Ctrl Pts',(3.96995018565893,-1.,0.146330797814521));
#39845=CARTESIAN_POINT('Ctrl Pts',(3.97701581473644,-1.,0.149070594803545));
#39846=CARTESIAN_POINT('Ctrl Pts',(3.98407729850975,-1.,0.151854737441399));
#39847=CARTESIAN_POINT('Ctrl Pts',(3.99113582086043,-1.,0.154682618338548));
#39848=CARTESIAN_POINT('Ctrl Pts',(3.9981907463185,-1.,0.15755363438379));
#39849=CARTESIAN_POINT('Ctrl Pts',(4.00524031064487,-1.,0.160467194882203));
#39850=CARTESIAN_POINT('Ctrl Pts',(4.01228237022296,-1.,0.163422730287457));
#39851=CARTESIAN_POINT('Ctrl Pts',(4.01931510507167,-1.,0.166419700015866));
#39852=CARTESIAN_POINT('Ctrl Pts',(4.02633779703764,-1.,0.169457601001692));
#39853=CARTESIAN_POINT('Ctrl Pts',(4.03335057326163,-1.,0.172535962484515));
#39854=CARTESIAN_POINT('Ctrl Pts',(4.04035407891222,-1.,0.175654339673798));
#39855=CARTESIAN_POINT('Ctrl Pts',(4.04734916719741,-1.,0.178812307240729));
#39856=CARTESIAN_POINT('Ctrl Pts',(4.05433660358353,-1.,0.18200945304852));
#39857=CARTESIAN_POINT('Ctrl Pts',(4.06131670998469,-1.,0.185245370038874));
#39858=CARTESIAN_POINT('Ctrl Pts',(4.06828941192148,-1.,0.188519658060156));
#39859=CARTESIAN_POINT('Ctrl Pts',(4.07525439702992,-1.,0.191831928180991));
#39860=CARTESIAN_POINT('Ctrl Pts',(4.08221124060322,-1.,0.195181806054676));
#39861=CARTESIAN_POINT('Ctrl Pts',(4.08915953359833,-1.,0.198568934800862));
#39862=CARTESIAN_POINT('Ctrl Pts',(4.09609903752152,-1.,0.201992979050136));
#39863=CARTESIAN_POINT('Ctrl Pts',(4.10302969965728,-1.,0.205453622198455));
#39864=CARTESIAN_POINT('Ctrl Pts',(4.10995157639377,-1.,0.208950559400393));
#39865=CARTESIAN_POINT('Ctrl Pts',(4.11686478264739,-1.,0.21248349108719));
#39866=CARTESIAN_POINT('Ctrl Pts',(4.12376943492132,-1.,0.216052116898353));
#39867=CARTESIAN_POINT('Ctrl Pts',(4.13066558697658,-1.,0.219656126701542));
#39868=CARTESIAN_POINT('Ctrl Pts',(4.13755320552764,-1.,0.223295201037886));
#39869=CARTESIAN_POINT('Ctrl Pts',(4.14443220606869,-1.,0.226969025060706));
#39870=CARTESIAN_POINT('Ctrl Pts',(4.15130247434459,-1.,0.230677299028384));
#39871=CARTESIAN_POINT('Ctrl Pts',(4.15816389265352,-1.,0.234419749543208));
#39872=CARTESIAN_POINT('Ctrl Pts',(4.16501636654877,-1.,0.238196140934617));
#39873=CARTESIAN_POINT('Ctrl Pts',(4.17185984411426,-1.,0.242006283925089));
#39874=CARTESIAN_POINT('Ctrl Pts',(4.1786943019518,-1.,0.24585003342002));
#39875=CARTESIAN_POINT('Ctrl Pts',(4.18415464961466,-1.,0.248951836912189));
#39876=CARTESIAN_POINT('Ctrl Pts',(4.18824585245272,-1.,0.251293239838441));
#39877=CARTESIAN_POINT('Ctrl Pts',(4.19097151819684,-1.,0.252860861572841));
#39878=CARTESIAN_POINT('Ctrl Pts',(4.1923339003649,-1.,0.253646344052522));
#39879=CARTESIAN_POINT('',(4.18039834341342,-1.,0.405301974318351));
#39880=CARTESIAN_POINT('',(4.1923339003649,-1.,0.253646344052522));
#39881=CARTESIAN_POINT('Ctrl Pts',(4.18039834341342,-1.,0.405301974318351));
#39882=CARTESIAN_POINT('Ctrl Pts',(4.17892985789466,-1.,0.40586466267921));
#39883=CARTESIAN_POINT('Ctrl Pts',(4.17599251954382,-1.,0.406986596325455));
#39884=CARTESIAN_POINT('Ctrl Pts',(4.17158541007977,-1.,0.408659167568273));
#39885=CARTESIAN_POINT('Ctrl Pts',(4.16570705938425,-1.,0.410868596146415));
#39886=CARTESIAN_POINT('Ctrl Pts',(4.15835545017202,-1.,0.413595877951471));
#39887=CARTESIAN_POINT('Ctrl Pts',(4.15100018949965,-1.,0.416288556008012));
#39888=CARTESIAN_POINT('Ctrl Pts',(4.14364132317121,-1.,0.418946490667703));
#39889=CARTESIAN_POINT('Ctrl Pts',(4.13627893207002,-1.,0.421569503104513));
#39890=CARTESIAN_POINT('Ctrl Pts',(4.12891314634572,-1.,0.424157375323976));
#39891=CARTESIAN_POINT('Ctrl Pts',(4.12154412502007,-1.,0.426709855707001));
#39892=CARTESIAN_POINT('Ctrl Pts',(4.11417202783267,-1.,0.429226666075845));
#39893=CARTESIAN_POINT('Ctrl Pts',(4.10679698750336,-1.,0.431707508679884));
#39894=CARTESIAN_POINT('Ctrl Pts',(4.09941908688373,-1.,0.434152073200461));
#39895=CARTESIAN_POINT('Ctrl Pts',(4.09203832139089,-1.,0.436560044913483));
#39896=CARTESIAN_POINT('Ctrl Pts',(4.08465462294273,-1.,0.43893110893128));
#39897=CARTESIAN_POINT('Ctrl Pts',(4.07726792490016,-1.,0.441264951396361));
#39898=CARTESIAN_POINT('Ctrl Pts',(4.0698782192569,-1.,0.443561262395333));
#39899=CARTESIAN_POINT('Ctrl Pts',(4.06248560760659,-1.,0.445819737468538));
#39900=CARTESIAN_POINT('Ctrl Pts',(4.0550903779696,-1.,0.448040082684115));
#39901=CARTESIAN_POINT('Ctrl Pts',(4.0476929901813,-1.,0.450222009543927));
#39902=CARTESIAN_POINT('Ctrl Pts',(4.04029392228049,-1.,0.452365214748893));
#39903=CARTESIAN_POINT('Ctrl Pts',(4.03289354362794,-1.,0.454469363020542));
#39904=CARTESIAN_POINT('Ctrl Pts',(4.02549199038394,-1.,0.456534070784951));
#39905=CARTESIAN_POINT('Ctrl Pts',(4.01808900827587,-1.,0.458558885636946));
#39906=CARTESIAN_POINT('Ctrl Pts',(4.01068390573399,-1.,0.460543280768515));
#39907=CARTESIAN_POINT('Ctrl Pts',(4.00327590659075,-1.,0.462486702616205));
#39908=CARTESIAN_POINT('Ctrl Pts',(3.9958644432011,-1.,0.464388610938976));
#39909=CARTESIAN_POINT('Ctrl Pts',(3.98844946363262,-1.,0.46624852088304));
#39910=CARTESIAN_POINT('Ctrl Pts',(3.98103175589371,-1.,0.468066047920158));
#39911=CARTESIAN_POINT('Ctrl Pts',(3.97361320212436,-1.,0.469840942829896));
#39912=CARTESIAN_POINT('Ctrl Pts',(3.96619600864643,-1.,0.471572978413504));
#39913=CARTESIAN_POINT('Ctrl Pts',(3.95878201038338,-1.,0.473261847236298));
#39914=CARTESIAN_POINT('Ctrl Pts',(3.95137192932897,-1.,0.474907053021791));
#39915=CARTESIAN_POINT('Ctrl Pts',(3.94396469119383,-1.,0.476507810658538));
#39916=CARTESIAN_POINT('Ctrl Pts',(3.93655660689819,-1.,0.478062927140965));
#39917=CARTESIAN_POINT('Ctrl Pts',(3.92914297392071,-1.,0.479571028525579));
#39918=CARTESIAN_POINT('Ctrl Pts',(3.92171976072341,-1.,0.481030798910749));
#39919=CARTESIAN_POINT('Ctrl Pts',(3.91428536373751,-1.,0.482441230340714));
#39920=CARTESIAN_POINT('Ctrl Pts',(3.90684210358056,-1.,0.48380183508915));
#39921=CARTESIAN_POINT('Ctrl Pts',(3.89939844658513,-1.,0.485112963522223));
#39922=CARTESIAN_POINT('Ctrl Pts',(3.89196582437552,-1.,0.486375337854104));
#39923=CARTESIAN_POINT('Ctrl Pts',(3.88455453328138,-1.,0.487589452275155));
#39924=CARTESIAN_POINT('Ctrl Pts',(3.87716963231109,-1.,0.488754973798274));
#39925=CARTESIAN_POINT('Ctrl Pts',(3.86980755613707,-1.,0.489870245704918));
#39926=CARTESIAN_POINT('Ctrl Pts',(3.86245057319246,-1.,0.490931482170891));
#39927=CARTESIAN_POINT('Ctrl Pts',(3.85507287020263,-1.,0.491933631083814));
#39928=CARTESIAN_POINT('Ctrl Pts',(3.84765051147999,-1.,0.492871792414141));
#39929=CARTESIAN_POINT('Ctrl Pts',(3.84017095578451,-1.,0.493742574629135));
#39930=CARTESIAN_POINT('Ctrl Pts',(3.83264092682431,-1.,0.494545212256402));
#39931=CARTESIAN_POINT('Ctrl Pts',(3.82509963594103,-1.,0.495283458893838));
#39932=CARTESIAN_POINT('Ctrl Pts',(3.81760756144025,-1.,0.49596393787548));
#39933=CARTESIAN_POINT('Ctrl Pts',(3.81022254090839,-1.,0.496592643443704));
#39934=CARTESIAN_POINT('Ctrl Pts',(3.80297788298514,-1.,0.497171756201052));
#39935=CARTESIAN_POINT('Ctrl Pts',(3.79586380669994,-1.,0.497696892100625));
#39936=CARTESIAN_POINT('Ctrl Pts',(3.78879701661264,-1.,0.498152751800959));
#39937=CARTESIAN_POINT('Ctrl Pts',(3.78163975337356,-1.,0.498515471679585));
#39938=CARTESIAN_POINT('Ctrl Pts',(3.77425499225255,-1.,0.498759900365892));
#39939=CARTESIAN_POINT('Ctrl Pts',(3.76655401191229,-1.,0.498865792335291));
#39940=CARTESIAN_POINT('Ctrl Pts',(3.75854082221053,-1.,0.498823681615422));
#39941=CARTESIAN_POINT('Ctrl Pts',(3.75037362167839,-1.,0.498642802042606));
#39942=CARTESIAN_POINT('Ctrl Pts',(3.74235701734714,-1.,0.498350586057693));
#39943=CARTESIAN_POINT('Ctrl Pts',(3.73486914372449,-1.,0.497984209510025));
#39944=CARTESIAN_POINT('Ctrl Pts',(3.72830430904606,-1.,0.49758406715305));
#39945=CARTESIAN_POINT('Ctrl Pts',(3.72301489774398,-1.,0.497187079575988));
#39946=CARTESIAN_POINT('Ctrl Pts',(3.71952320822499,-1.,0.496846224822564));
#39947=CARTESIAN_POINT('Ctrl Pts',(3.71785517607549,-1.,0.496605651525989));
#39948=CARTESIAN_POINT('Ctrl Pts',(3.71721917030355,-1.,0.496446644158006));
#39949=CARTESIAN_POINT('Ctrl Pts',(3.71704500630494,-1.,0.496354087924313));
#39950=CARTESIAN_POINT('Ctrl Pts',(3.71701050416825,-1.,0.496319364827592));
#39951=CARTESIAN_POINT('Origin',(0.,-1.,0.));
#39952=CARTESIAN_POINT('Origin',(0.,0.,0.));
#39953=CARTESIAN_POINT('Origin',(0.,2.2,0.));
#39954=CARTESIAN_POINT('Origin',(0.,1.,0.));
#39955=CARTESIAN_POINT('',(-1.99383466746626,2.2,0.15691819145569));
#39956=CARTESIAN_POINT('Origin',(0.,2.2,0.));
#39957=CARTESIAN_POINT('',(-1.99383466746626,1.,0.15691819145569));
#39958=CARTESIAN_POINT('',(-1.99383466746626,1.,0.15691819145569));
#39959=CARTESIAN_POINT('Origin',(0.,1.,0.));
#39960=CARTESIAN_POINT('Origin',(0.,2.2,0.));
#39961=CARTESIAN_POINT('Ctrl Pts',(4.1923339003649,-1.,0.253646344052522));
#39962=CARTESIAN_POINT('Ctrl Pts',(4.1923339003649,1.,0.253646344052522));
#39963=CARTESIAN_POINT('Ctrl Pts',(4.19097151819684,-1.,0.252860861572841));
#39964=CARTESIAN_POINT('Ctrl Pts',(4.19097151819684,1.,0.252860861572841));
#39965=CARTESIAN_POINT('Ctrl Pts',(4.18824585245272,-1.,0.251293239838441));
#39966=CARTESIAN_POINT('Ctrl Pts',(4.18824585245272,1.,0.251293239838441));
#39967=CARTESIAN_POINT('Ctrl Pts',(4.18415464961466,-1.,0.248951836912189));
#39968=CARTESIAN_POINT('Ctrl Pts',(4.18415464961466,1.,0.248951836912189));
#39969=CARTESIAN_POINT('Ctrl Pts',(4.1786943019518,-1.,0.24585003342002));
#39970=CARTESIAN_POINT('Ctrl Pts',(4.1786943019518,1.,0.24585003342002));
#39971=CARTESIAN_POINT('Ctrl Pts',(4.17185984411426,-1.,0.242006283925089));
#39972=CARTESIAN_POINT('Ctrl Pts',(4.17185984411426,1.,0.242006283925089));
#39973=CARTESIAN_POINT('Ctrl Pts',(4.16501636654877,-1.,0.238196140934617));
#39974=CARTESIAN_POINT('Ctrl Pts',(4.16501636654877,1.,0.238196140934617));
#39975=CARTESIAN_POINT('Ctrl Pts',(4.15816389265352,-1.,0.234419749543208));
#39976=CARTESIAN_POINT('Ctrl Pts',(4.15816389265352,1.,0.234419749543208));
#39977=CARTESIAN_POINT('Ctrl Pts',(4.15130247434459,-1.,0.230677299028384));
#39978=CARTESIAN_POINT('Ctrl Pts',(4.15130247434459,1.,0.230677299028384));
#39979=CARTESIAN_POINT('Ctrl Pts',(4.14443220606869,-1.,0.226969025060706));
#39980=CARTESIAN_POINT('Ctrl Pts',(4.14443220606869,1.,0.226969025060706));
#39981=CARTESIAN_POINT('Ctrl Pts',(4.13755320552764,-1.,0.223295201037886));
#39982=CARTESIAN_POINT('Ctrl Pts',(4.13755320552764,1.,0.223295201037886));
#39983=CARTESIAN_POINT('Ctrl Pts',(4.13066558697658,-1.,0.219656126701542));
#39984=CARTESIAN_POINT('Ctrl Pts',(4.13066558697658,1.,0.219656126701542));
#39985=CARTESIAN_POINT('Ctrl Pts',(4.12376943492132,-1.,0.216052116898353));
#39986=CARTESIAN_POINT('Ctrl Pts',(4.12376943492132,1.,0.216052116898353));
#39987=CARTESIAN_POINT('Ctrl Pts',(4.11686478264739,-1.,0.21248349108719));
#39988=CARTESIAN_POINT('Ctrl Pts',(4.11686478264739,1.,0.21248349108719));
#39989=CARTESIAN_POINT('Ctrl Pts',(4.10995157639377,-1.,0.208950559400393));
#39990=CARTESIAN_POINT('Ctrl Pts',(4.10995157639377,1.,0.208950559400393));
#39991=CARTESIAN_POINT('Ctrl Pts',(4.10302969965728,-1.,0.205453622198455));
#39992=CARTESIAN_POINT('Ctrl Pts',(4.10302969965728,1.,0.205453622198455));
#39993=CARTESIAN_POINT('Ctrl Pts',(4.09609903752152,-1.,0.201992979050136));
#39994=CARTESIAN_POINT('Ctrl Pts',(4.09609903752152,1.,0.201992979050136));
#39995=CARTESIAN_POINT('Ctrl Pts',(4.08915953359833,-1.,0.198568934800862));
#39996=CARTESIAN_POINT('Ctrl Pts',(4.08915953359833,1.,0.198568934800862));
#39997=CARTESIAN_POINT('Ctrl Pts',(4.08221124060322,-1.,0.195181806054676));
#39998=CARTESIAN_POINT('Ctrl Pts',(4.08221124060322,1.,0.195181806054676));
#39999=CARTESIAN_POINT('Ctrl Pts',(4.07525439702992,-1.,0.191831928180991));
#40000=CARTESIAN_POINT('Ctrl Pts',(4.07525439702992,1.,0.191831928180991));
#40001=CARTESIAN_POINT('Ctrl Pts',(4.06828941192148,-1.,0.188519658060156));
#40002=CARTESIAN_POINT('Ctrl Pts',(4.06828941192148,1.,0.188519658060156));
#40003=CARTESIAN_POINT('Ctrl Pts',(4.06131670998469,-1.,0.185245370038874));
#40004=CARTESIAN_POINT('Ctrl Pts',(4.06131670998469,1.,0.185245370038874));
#40005=CARTESIAN_POINT('Ctrl Pts',(4.05433660358353,-1.,0.18200945304852));
#40006=CARTESIAN_POINT('Ctrl Pts',(4.05433660358353,1.,0.18200945304852));
#40007=CARTESIAN_POINT('Ctrl Pts',(4.04734916719741,-1.,0.178812307240729));
#40008=CARTESIAN_POINT('Ctrl Pts',(4.04734916719741,1.,0.178812307240729));
#40009=CARTESIAN_POINT('Ctrl Pts',(4.04035407891222,-1.,0.175654339673798));
#40010=CARTESIAN_POINT('Ctrl Pts',(4.04035407891222,1.,0.175654339673798));
#40011=CARTESIAN_POINT('Ctrl Pts',(4.03335057326163,-1.,0.172535962484515));
#40012=CARTESIAN_POINT('Ctrl Pts',(4.03335057326163,1.,0.172535962484515));
#40013=CARTESIAN_POINT('Ctrl Pts',(4.02633779703764,-1.,0.169457601001692));
#40014=CARTESIAN_POINT('Ctrl Pts',(4.02633779703764,1.,0.169457601001692));
#40015=CARTESIAN_POINT('Ctrl Pts',(4.01931510507167,-1.,0.166419700015866));
#40016=CARTESIAN_POINT('Ctrl Pts',(4.01931510507167,1.,0.166419700015866));
#40017=CARTESIAN_POINT('Ctrl Pts',(4.01228237022296,-1.,0.163422730287457));
#40018=CARTESIAN_POINT('Ctrl Pts',(4.01228237022296,1.,0.163422730287457));
#40019=CARTESIAN_POINT('Ctrl Pts',(4.00524031064487,-1.,0.160467194882203));
#40020=CARTESIAN_POINT('Ctrl Pts',(4.00524031064487,1.,0.160467194882203));
#40021=CARTESIAN_POINT('Ctrl Pts',(3.9981907463185,-1.,0.15755363438379));
#40022=CARTESIAN_POINT('Ctrl Pts',(3.9981907463185,1.,0.15755363438379));
#40023=CARTESIAN_POINT('Ctrl Pts',(3.99113582086043,-1.,0.154682618338548));
#40024=CARTESIAN_POINT('Ctrl Pts',(3.99113582086043,1.,0.154682618338548));
#40025=CARTESIAN_POINT('Ctrl Pts',(3.98407729850975,-1.,0.151854737441399));
#40026=CARTESIAN_POINT('Ctrl Pts',(3.98407729850975,1.,0.151854737441399));
#40027=CARTESIAN_POINT('Ctrl Pts',(3.97701581473644,-1.,0.149070594803545));
#40028=CARTESIAN_POINT('Ctrl Pts',(3.97701581473644,1.,0.149070594803545));
#40029=CARTESIAN_POINT('Ctrl Pts',(3.96995018565893,-1.,0.146330797814521));
#40030=CARTESIAN_POINT('Ctrl Pts',(3.96995018565893,1.,0.146330797814521));
#40031=CARTESIAN_POINT('Ctrl Pts',(3.96287658098896,-1.,0.143635947692799));
#40032=CARTESIAN_POINT('Ctrl Pts',(3.96287658098896,1.,0.143635947692799));
#40033=CARTESIAN_POINT('Ctrl Pts',(3.95579014116894,-1.,0.140986665829942));
#40034=CARTESIAN_POINT('Ctrl Pts',(3.95579014116894,1.,0.140986665829942));
#40035=CARTESIAN_POINT('Ctrl Pts',(3.94868667844347,-1.,0.138383621255161));
#40036=CARTESIAN_POINT('Ctrl Pts',(3.94868667844347,1.,0.138383621255161));
#40037=CARTESIAN_POINT('Ctrl Pts',(3.94156445130741,-1.,0.135827558661189));
#40038=CARTESIAN_POINT('Ctrl Pts',(3.94156445130741,1.,0.135827558661189));
#40039=CARTESIAN_POINT('Ctrl Pts',(3.93442567551042,-1.,0.133319322794191));
#40040=CARTESIAN_POINT('Ctrl Pts',(3.93442567551042,1.,0.133319322794191));
#40041=CARTESIAN_POINT('Ctrl Pts',(3.92727876795977,-1.,0.130859892027802));
#40042=CARTESIAN_POINT('Ctrl Pts',(3.92727876795977,1.,0.130859892027802));
#40043=CARTESIAN_POINT('Ctrl Pts',(3.92013513251664,-1.,0.128450341339533));
#40044=CARTESIAN_POINT('Ctrl Pts',(3.92013513251664,1.,0.128450341339533));
#40045=CARTESIAN_POINT('Ctrl Pts',(3.91300501605411,-1.,0.126091793324141));
#40046=CARTESIAN_POINT('Ctrl Pts',(3.91300501605411,1.,0.126091793324141));
#40047=CARTESIAN_POINT('Ctrl Pts',(3.90589336320515,-1.,0.12378536827238));
#40048=CARTESIAN_POINT('Ctrl Pts',(3.90589336320515,1.,0.12378536827238));
#40049=CARTESIAN_POINT('Ctrl Pts',(3.89879639336939,-1.,0.121532144765722));
#40050=CARTESIAN_POINT('Ctrl Pts',(3.89879639336939,1.,0.121532144765722));
#40051=CARTESIAN_POINT('Ctrl Pts',(3.8916960010517,-1.,0.119333088190411));
#40052=CARTESIAN_POINT('Ctrl Pts',(3.8916960010517,1.,0.119333088190411));
#40053=CARTESIAN_POINT('Ctrl Pts',(3.88456590045726,-1.,0.117189150373135));
#40054=CARTESIAN_POINT('Ctrl Pts',(3.88456590045726,1.,0.117189150373135));
#40055=CARTESIAN_POINT('Ctrl Pts',(3.87738168405308,-1.,0.115101426649461));
#40056=CARTESIAN_POINT('Ctrl Pts',(3.87738168405308,1.,0.115101426649461));
#40057=CARTESIAN_POINT('Ctrl Pts',(3.87013043445001,-1.,0.113071304914559));
#40058=CARTESIAN_POINT('Ctrl Pts',(3.87013043445001,1.,0.113071304914559));
#40059=CARTESIAN_POINT('Ctrl Pts',(3.86281867282984,-1.,0.111100593036267));
#40060=CARTESIAN_POINT('Ctrl Pts',(3.86281867282984,1.,0.111100593036267));
#40061=CARTESIAN_POINT('Ctrl Pts',(3.85548571496953,-1.,0.109191717634961));
#40062=CARTESIAN_POINT('Ctrl Pts',(3.85548571496953,1.,0.109191717634961));
#40063=CARTESIAN_POINT('Ctrl Pts',(3.84819233070391,-1.,0.107347597812209));
#40064=CARTESIAN_POINT('Ctrl Pts',(3.84819233070391,1.,0.107347597812209));
#40065=CARTESIAN_POINT('Ctrl Pts',(3.84099658324873,-1.,0.105571360916594));
#40066=CARTESIAN_POINT('Ctrl Pts',(3.84099658324873,1.,0.105571360916594));
#40067=CARTESIAN_POINT('Ctrl Pts',(3.83393171228034,-1.,0.103866063811635));
#40068=CARTESIAN_POINT('Ctrl Pts',(3.83393171228034,1.,0.103866063811635));
#40069=CARTESIAN_POINT('Ctrl Pts',(3.8269873714322,-1.,0.102234506488446));
#40070=CARTESIAN_POINT('Ctrl Pts',(3.8269873714322,1.,0.102234506488446));
#40071=CARTESIAN_POINT('Ctrl Pts',(3.82007889742512,-1.,0.100678769650595));
#40072=CARTESIAN_POINT('Ctrl Pts',(3.82007889742512,1.,0.100678769650595));
#40073=CARTESIAN_POINT('Ctrl Pts',(3.81306649386293,-1.,0.0992008728095949));
#40074=CARTESIAN_POINT('Ctrl Pts',(3.81306649386293,1.,0.0992008728095949));
#40075=CARTESIAN_POINT('Ctrl Pts',(3.80581088847642,-1.,0.097804222290608));
#40076=CARTESIAN_POINT('Ctrl Pts',(3.80581088847642,1.,0.097804222290608));
#40077=CARTESIAN_POINT('Ctrl Pts',(3.7982212851376,-1.,0.0964949352872849));
#40078=CARTESIAN_POINT('Ctrl Pts',(3.7982212851376,1.,0.0964949352872849));
#40079=CARTESIAN_POINT('Ctrl Pts',(3.79030016353186,-1.,0.0952829885101074));
#40080=CARTESIAN_POINT('Ctrl Pts',(3.79030016353186,1.,0.0952829885101074));
#40081=CARTESIAN_POINT('Ctrl Pts',(3.78220521899366,-1.,0.0941840095091749));
#40082=CARTESIAN_POINT('Ctrl Pts',(3.78220521899366,1.,0.0941840095091749));
#40083=CARTESIAN_POINT('Ctrl Pts',(3.77424159971456,-1.,0.093218554620458));
#40084=CARTESIAN_POINT('Ctrl Pts',(3.77424159971456,1.,0.093218554620458));
#40085=CARTESIAN_POINT('Ctrl Pts',(3.76678860032228,-1.,0.092409058960406));
#40086=CARTESIAN_POINT('Ctrl Pts',(3.76678860032228,1.,0.092409058960406));
#40087=CARTESIAN_POINT('Ctrl Pts',(3.76024199359493,-1.,0.0917773084999013));
#40088=CARTESIAN_POINT('Ctrl Pts',(3.76024199359493,1.,0.0917773084999013));
#40089=CARTESIAN_POINT('Ctrl Pts',(3.75495560118053,-1.,0.0913419622735858));
#40090=CARTESIAN_POINT('Ctrl Pts',(3.75495560118053,1.,0.0913419622735858));
#40091=CARTESIAN_POINT('Ctrl Pts',(3.75116949194125,-1.,0.0911154000996411));
#40092=CARTESIAN_POINT('Ctrl Pts',(3.75116949194125,1.,0.0911154000996411));
#40093=CARTESIAN_POINT('Ctrl Pts',(3.74943097853257,-1.,0.0911057547504666));
#40094=CARTESIAN_POINT('Ctrl Pts',(3.74943097853257,1.,0.0911057547504666));
#40095=CARTESIAN_POINT('Ctrl Pts',(3.7488701717383,-1.,0.0911958743733931));
#40096=CARTESIAN_POINT('Ctrl Pts',(3.7488701717383,1.,0.0911958743733931));
#40097=CARTESIAN_POINT('Ctrl Pts',(3.74882632118923,-1.,0.0912992005792096));
#40098=CARTESIAN_POINT('Ctrl Pts',(3.74882632118923,1.,0.0912992005792096));
#40099=CARTESIAN_POINT('Ctrl Pts',(3.74888690736767,-1.,0.0913616755937434));
#40100=CARTESIAN_POINT('Ctrl Pts',(3.74888690736767,1.,0.0913616755937434));
#40101=CARTESIAN_POINT('',(3.74888939116259,1.,0.0912596999148864));
#40102=CARTESIAN_POINT('Ctrl Pts',(3.74888939116259,1.,0.0912596999148864));
#40103=CARTESIAN_POINT('Ctrl Pts',(3.74888939116259,0.666666666666667,0.0912596999148864));
#40104=CARTESIAN_POINT('Ctrl Pts',(3.74888939116259,0.333333333333333,0.0912596999148864));
#40105=CARTESIAN_POINT('Ctrl Pts',(3.74888939116259,-0.333333333333333,
0.0912596999148864));
#40106=CARTESIAN_POINT('Ctrl Pts',(3.74888939116259,-0.666666666666667,
0.0912596999148867));
#40107=CARTESIAN_POINT('Ctrl Pts',(3.74888939116259,-1.,0.0912596999148867));
#40108=CARTESIAN_POINT('',(4.1923339003649,1.,0.253646344052522));
#40109=CARTESIAN_POINT('Ctrl Pts',(4.1923339003649,1.,0.253646344052522));
#40110=CARTESIAN_POINT('Ctrl Pts',(4.19097151819684,1.,0.252860861572841));
#40111=CARTESIAN_POINT('Ctrl Pts',(4.18824585245272,1.,0.251293239838441));
#40112=CARTESIAN_POINT('Ctrl Pts',(4.18415464961466,1.,0.248951836912189));
#40113=CARTESIAN_POINT('Ctrl Pts',(4.1786943019518,1.,0.24585003342002));
#40114=CARTESIAN_POINT('Ctrl Pts',(4.17185984411426,1.,0.242006283925089));
#40115=CARTESIAN_POINT('Ctrl Pts',(4.16501636654877,1.,0.238196140934617));
#40116=CARTESIAN_POINT('Ctrl Pts',(4.15816389265352,1.,0.234419749543208));
#40117=CARTESIAN_POINT('Ctrl Pts',(4.15130247434459,1.,0.230677299028384));
#40118=CARTESIAN_POINT('Ctrl Pts',(4.14443220606869,1.,0.226969025060706));
#40119=CARTESIAN_POINT('Ctrl Pts',(4.13755320552764,1.,0.223295201037886));
#40120=CARTESIAN_POINT('Ctrl Pts',(4.13066558697658,1.,0.219656126701542));
#40121=CARTESIAN_POINT('Ctrl Pts',(4.12376943492132,1.,0.216052116898353));
#40122=CARTESIAN_POINT('Ctrl Pts',(4.11686478264739,1.,0.21248349108719));
#40123=CARTESIAN_POINT('Ctrl Pts',(4.10995157639377,1.,0.208950559400393));
#40124=CARTESIAN_POINT('Ctrl Pts',(4.10302969965728,1.,0.205453622198455));
#40125=CARTESIAN_POINT('Ctrl Pts',(4.09609903752152,1.,0.201992979050136));
#40126=CARTESIAN_POINT('Ctrl Pts',(4.08915953359833,1.,0.198568934800862));
#40127=CARTESIAN_POINT('Ctrl Pts',(4.08221124060322,1.,0.195181806054676));
#40128=CARTESIAN_POINT('Ctrl Pts',(4.07525439702992,1.,0.191831928180991));
#40129=CARTESIAN_POINT('Ctrl Pts',(4.06828941192148,1.,0.188519658060156));
#40130=CARTESIAN_POINT('Ctrl Pts',(4.06131670998469,1.,0.185245370038874));
#40131=CARTESIAN_POINT('Ctrl Pts',(4.05433660358353,1.,0.18200945304852));
#40132=CARTESIAN_POINT('Ctrl Pts',(4.04734916719741,1.,0.178812307240729));
#40133=CARTESIAN_POINT('Ctrl Pts',(4.04035407891222,1.,0.175654339673798));
#40134=CARTESIAN_POINT('Ctrl Pts',(4.03335057326163,1.,0.172535962484515));
#40135=CARTESIAN_POINT('Ctrl Pts',(4.02633779703764,1.,0.169457601001692));
#40136=CARTESIAN_POINT('Ctrl Pts',(4.01931510507167,1.,0.166419700015866));
#40137=CARTESIAN_POINT('Ctrl Pts',(4.01228237022296,1.,0.163422730287457));
#40138=CARTESIAN_POINT('Ctrl Pts',(4.00524031064487,1.,0.160467194882203));
#40139=CARTESIAN_POINT('Ctrl Pts',(3.9981907463185,1.,0.15755363438379));
#40140=CARTESIAN_POINT('Ctrl Pts',(3.99113582086043,1.,0.154682618338548));
#40141=CARTESIAN_POINT('Ctrl Pts',(3.98407729850975,1.,0.151854737441399));
#40142=CARTESIAN_POINT('Ctrl Pts',(3.97701581473644,1.,0.149070594803545));
#40143=CARTESIAN_POINT('Ctrl Pts',(3.96995018565893,1.,0.146330797814521));
#40144=CARTESIAN_POINT('Ctrl Pts',(3.96287658098896,1.,0.143635947692799));
#40145=CARTESIAN_POINT('Ctrl Pts',(3.95579014116894,1.,0.140986665829942));
#40146=CARTESIAN_POINT('Ctrl Pts',(3.94868667844347,1.,0.138383621255161));
#40147=CARTESIAN_POINT('Ctrl Pts',(3.94156445130741,1.,0.135827558661189));
#40148=CARTESIAN_POINT('Ctrl Pts',(3.93442567551042,1.,0.133319322794191));
#40149=CARTESIAN_POINT('Ctrl Pts',(3.92727876795977,1.,0.130859892027802));
#40150=CARTESIAN_POINT('Ctrl Pts',(3.92013513251664,1.,0.128450341339533));
#40151=CARTESIAN_POINT('Ctrl Pts',(3.91300501605411,1.,0.126091793324141));
#40152=CARTESIAN_POINT('Ctrl Pts',(3.90589336320515,1.,0.12378536827238));
#40153=CARTESIAN_POINT('Ctrl Pts',(3.89879639336939,1.,0.121532144765722));
#40154=CARTESIAN_POINT('Ctrl Pts',(3.8916960010517,1.,0.119333088190411));
#40155=CARTESIAN_POINT('Ctrl Pts',(3.88456590045726,1.,0.117189150373135));
#40156=CARTESIAN_POINT('Ctrl Pts',(3.87738168405308,1.,0.115101426649461));
#40157=CARTESIAN_POINT('Ctrl Pts',(3.87013043445001,1.,0.113071304914559));
#40158=CARTESIAN_POINT('Ctrl Pts',(3.86281867282984,1.,0.111100593036267));
#40159=CARTESIAN_POINT('Ctrl Pts',(3.85548571496953,1.,0.109191717634961));
#40160=CARTESIAN_POINT('Ctrl Pts',(3.84819233070391,1.,0.107347597812209));
#40161=CARTESIAN_POINT('Ctrl Pts',(3.84099658324873,1.,0.105571360916594));
#40162=CARTESIAN_POINT('Ctrl Pts',(3.83393171228034,1.,0.103866063811635));
#40163=CARTESIAN_POINT('Ctrl Pts',(3.8269873714322,1.,0.102234506488446));
#40164=CARTESIAN_POINT('Ctrl Pts',(3.82007889742512,1.,0.100678769650595));
#40165=CARTESIAN_POINT('Ctrl Pts',(3.81306649386293,1.,0.0992008728095949));
#40166=CARTESIAN_POINT('Ctrl Pts',(3.80581088847642,1.,0.097804222290608));
#40167=CARTESIAN_POINT('Ctrl Pts',(3.7982212851376,1.,0.0964949352872849));
#40168=CARTESIAN_POINT('Ctrl Pts',(3.79030016353186,1.,0.0952829885101074));
#40169=CARTESIAN_POINT('Ctrl Pts',(3.78220521899366,1.,0.0941840095091749));
#40170=CARTESIAN_POINT('Ctrl Pts',(3.77424159971456,1.,0.093218554620458));
#40171=CARTESIAN_POINT('Ctrl Pts',(3.76678860032228,1.,0.092409058960406));
#40172=CARTESIAN_POINT('Ctrl Pts',(3.76024199359493,1.,0.0917773084999013));
#40173=CARTESIAN_POINT('Ctrl Pts',(3.75495560118053,1.,0.0913419622735858));
#40174=CARTESIAN_POINT('Ctrl Pts',(3.75145357872511,1.,0.0911323999576148));
#40175=CARTESIAN_POINT('Ctrl Pts',(3.74976844886495,1.,0.0911090736804576));
#40176=CARTESIAN_POINT('Ctrl Pts',(3.74911539914664,1.,0.091166630180643));
#40177=CARTESIAN_POINT('Ctrl Pts',(3.74892890041021,1.,0.0912308016409239));
#40178=CARTESIAN_POINT('Ctrl Pts',(3.74888939116259,1.,0.0912596999148865));
#40179=CARTESIAN_POINT('',(4.1923339003649,0.,0.253646344052522));
#40180=CARTESIAN_POINT('Ctrl Pts',(3.71702400346349,-1.,0.496218256089213));
#40181=CARTESIAN_POINT('Ctrl Pts',(3.71702400346349,1.,0.496218256089213));
#40182=CARTESIAN_POINT('Ctrl Pts',(3.7169543899574,-1.,0.496270484166409));
#40183=CARTESIAN_POINT('Ctrl Pts',(3.7169543899574,1.,0.496270484166409));
#40184=CARTESIAN_POINT('Ctrl Pts',(3.71698153685602,-1.,0.49637939799264));
#40185=CARTESIAN_POINT('Ctrl Pts',(3.71698153685602,1.,0.49637939799264));
#40186=CARTESIAN_POINT('Ctrl Pts',(3.71752134137482,-1.,0.496556137604533));
#40187=CARTESIAN_POINT('Ctrl Pts',(3.71752134137482,1.,0.496556137604533));
#40188=CARTESIAN_POINT('Ctrl Pts',(3.71923995966302,-1.,0.496818574420596));
#40189=CARTESIAN_POINT('Ctrl Pts',(3.71923995966302,1.,0.496818574420596));
#40190=CARTESIAN_POINT('Ctrl Pts',(3.72301489774398,-1.,0.497187079575988));
#40191=CARTESIAN_POINT('Ctrl Pts',(3.72301489774398,1.,0.497187079575988));
#40192=CARTESIAN_POINT('Ctrl Pts',(3.72830430904606,-1.,0.49758406715305));
#40193=CARTESIAN_POINT('Ctrl Pts',(3.72830430904606,1.,0.49758406715305));
#40194=CARTESIAN_POINT('Ctrl Pts',(3.73486914372449,-1.,0.497984209510025));
#40195=CARTESIAN_POINT('Ctrl Pts',(3.73486914372449,1.,0.497984209510025));
#40196=CARTESIAN_POINT('Ctrl Pts',(3.74235701734714,-1.,0.498350586057693));
#40197=CARTESIAN_POINT('Ctrl Pts',(3.74235701734714,1.,0.498350586057693));
#40198=CARTESIAN_POINT('Ctrl Pts',(3.75037362167839,-1.,0.498642802042606));
#40199=CARTESIAN_POINT('Ctrl Pts',(3.75037362167839,1.,0.498642802042606));
#40200=CARTESIAN_POINT('Ctrl Pts',(3.75854082221053,-1.,0.498823681615422));
#40201=CARTESIAN_POINT('Ctrl Pts',(3.75854082221053,1.,0.498823681615422));
#40202=CARTESIAN_POINT('Ctrl Pts',(3.76655401191229,-1.,0.498865792335291));
#40203=CARTESIAN_POINT('Ctrl Pts',(3.76655401191229,1.,0.498865792335291));
#40204=CARTESIAN_POINT('Ctrl Pts',(3.77425499225255,-1.,0.498759900365892));
#40205=CARTESIAN_POINT('Ctrl Pts',(3.77425499225255,1.,0.498759900365892));
#40206=CARTESIAN_POINT('Ctrl Pts',(3.78163975337356,-1.,0.498515471679585));
#40207=CARTESIAN_POINT('Ctrl Pts',(3.78163975337356,1.,0.498515471679585));
#40208=CARTESIAN_POINT('Ctrl Pts',(3.78879701661264,-1.,0.498152751800959));
#40209=CARTESIAN_POINT('Ctrl Pts',(3.78879701661264,1.,0.498152751800959));
#40210=CARTESIAN_POINT('Ctrl Pts',(3.79586380669994,-1.,0.497696892100625));
#40211=CARTESIAN_POINT('Ctrl Pts',(3.79586380669994,1.,0.497696892100625));
#40212=CARTESIAN_POINT('Ctrl Pts',(3.80297788298514,-1.,0.497171756201052));
#40213=CARTESIAN_POINT('Ctrl Pts',(3.80297788298514,1.,0.497171756201052));
#40214=CARTESIAN_POINT('Ctrl Pts',(3.81022254090839,-1.,0.496592643443704));
#40215=CARTESIAN_POINT('Ctrl Pts',(3.81022254090839,1.,0.496592643443704));
#40216=CARTESIAN_POINT('Ctrl Pts',(3.81760756144025,-1.,0.49596393787548));
#40217=CARTESIAN_POINT('Ctrl Pts',(3.81760756144025,1.,0.49596393787548));
#40218=CARTESIAN_POINT('Ctrl Pts',(3.82509963594103,-1.,0.495283458893838));
#40219=CARTESIAN_POINT('Ctrl Pts',(3.82509963594103,1.,0.495283458893838));
#40220=CARTESIAN_POINT('Ctrl Pts',(3.83264092682431,-1.,0.494545212256402));
#40221=CARTESIAN_POINT('Ctrl Pts',(3.83264092682431,1.,0.494545212256402));
#40222=CARTESIAN_POINT('Ctrl Pts',(3.84017095578451,-1.,0.493742574629135));
#40223=CARTESIAN_POINT('Ctrl Pts',(3.84017095578451,1.,0.493742574629135));
#40224=CARTESIAN_POINT('Ctrl Pts',(3.84765051147999,-1.,0.492871792414141));
#40225=CARTESIAN_POINT('Ctrl Pts',(3.84765051147999,1.,0.492871792414141));
#40226=CARTESIAN_POINT('Ctrl Pts',(3.85507287020263,-1.,0.491933631083814));
#40227=CARTESIAN_POINT('Ctrl Pts',(3.85507287020263,1.,0.491933631083814));
#40228=CARTESIAN_POINT('Ctrl Pts',(3.86245057319246,-1.,0.490931482170891));
#40229=CARTESIAN_POINT('Ctrl Pts',(3.86245057319246,1.,0.490931482170891));
#40230=CARTESIAN_POINT('Ctrl Pts',(3.86980755613707,-1.,0.489870245704918));
#40231=CARTESIAN_POINT('Ctrl Pts',(3.86980755613707,1.,0.489870245704918));
#40232=CARTESIAN_POINT('Ctrl Pts',(3.87716963231109,-1.,0.488754973798274));
#40233=CARTESIAN_POINT('Ctrl Pts',(3.87716963231109,1.,0.488754973798274));
#40234=CARTESIAN_POINT('Ctrl Pts',(3.88455453328138,-1.,0.487589452275155));
#40235=CARTESIAN_POINT('Ctrl Pts',(3.88455453328138,1.,0.487589452275155));
#40236=CARTESIAN_POINT('Ctrl Pts',(3.89196582437552,-1.,0.486375337854104));
#40237=CARTESIAN_POINT('Ctrl Pts',(3.89196582437552,1.,0.486375337854104));
#40238=CARTESIAN_POINT('Ctrl Pts',(3.89939844658513,-1.,0.485112963522223));
#40239=CARTESIAN_POINT('Ctrl Pts',(3.89939844658513,1.,0.485112963522223));
#40240=CARTESIAN_POINT('Ctrl Pts',(3.90684210358056,-1.,0.48380183508915));
#40241=CARTESIAN_POINT('Ctrl Pts',(3.90684210358056,1.,0.48380183508915));
#40242=CARTESIAN_POINT('Ctrl Pts',(3.91428536373751,-1.,0.482441230340714));
#40243=CARTESIAN_POINT('Ctrl Pts',(3.91428536373751,1.,0.482441230340714));
#40244=CARTESIAN_POINT('Ctrl Pts',(3.92171976072341,-1.,0.481030798910749));
#40245=CARTESIAN_POINT('Ctrl Pts',(3.92171976072341,1.,0.481030798910749));
#40246=CARTESIAN_POINT('Ctrl Pts',(3.92914297392071,-1.,0.479571028525579));
#40247=CARTESIAN_POINT('Ctrl Pts',(3.92914297392071,1.,0.479571028525579));
#40248=CARTESIAN_POINT('Ctrl Pts',(3.93655660689819,-1.,0.478062927140965));
#40249=CARTESIAN_POINT('Ctrl Pts',(3.93655660689819,1.,0.478062927140965));
#40250=CARTESIAN_POINT('Ctrl Pts',(3.94396469119383,-1.,0.476507810658538));
#40251=CARTESIAN_POINT('Ctrl Pts',(3.94396469119383,1.,0.476507810658538));
#40252=CARTESIAN_POINT('Ctrl Pts',(3.95137192932897,-1.,0.474907053021791));
#40253=CARTESIAN_POINT('Ctrl Pts',(3.95137192932897,1.,0.474907053021791));
#40254=CARTESIAN_POINT('Ctrl Pts',(3.95878201038338,-1.,0.473261847236298));
#40255=CARTESIAN_POINT('Ctrl Pts',(3.95878201038338,1.,0.473261847236298));
#40256=CARTESIAN_POINT('Ctrl Pts',(3.96619600864643,-1.,0.471572978413504));
#40257=CARTESIAN_POINT('Ctrl Pts',(3.96619600864643,1.,0.471572978413504));
#40258=CARTESIAN_POINT('Ctrl Pts',(3.97361320212436,-1.,0.469840942829896));
#40259=CARTESIAN_POINT('Ctrl Pts',(3.97361320212436,1.,0.469840942829896));
#40260=CARTESIAN_POINT('Ctrl Pts',(3.98103175589371,-1.,0.468066047920158));
#40261=CARTESIAN_POINT('Ctrl Pts',(3.98103175589371,1.,0.468066047920158));
#40262=CARTESIAN_POINT('Ctrl Pts',(3.98844946363262,-1.,0.46624852088304));
#40263=CARTESIAN_POINT('Ctrl Pts',(3.98844946363262,1.,0.46624852088304));
#40264=CARTESIAN_POINT('Ctrl Pts',(3.9958644432011,-1.,0.464388610938976));
#40265=CARTESIAN_POINT('Ctrl Pts',(3.9958644432011,1.,0.464388610938976));
#40266=CARTESIAN_POINT('Ctrl Pts',(4.00327590659075,-1.,0.462486702616205));
#40267=CARTESIAN_POINT('Ctrl Pts',(4.00327590659075,1.,0.462486702616205));
#40268=CARTESIAN_POINT('Ctrl Pts',(4.01068390573399,-1.,0.460543280768515));
#40269=CARTESIAN_POINT('Ctrl Pts',(4.01068390573399,1.,0.460543280768515));
#40270=CARTESIAN_POINT('Ctrl Pts',(4.01808900827587,-1.,0.458558885636946));
#40271=CARTESIAN_POINT('Ctrl Pts',(4.01808900827587,1.,0.458558885636946));
#40272=CARTESIAN_POINT('Ctrl Pts',(4.02549199038394,-1.,0.456534070784951));
#40273=CARTESIAN_POINT('Ctrl Pts',(4.02549199038394,1.,0.456534070784951));
#40274=CARTESIAN_POINT('Ctrl Pts',(4.03289354362794,-1.,0.454469363020542));
#40275=CARTESIAN_POINT('Ctrl Pts',(4.03289354362794,1.,0.454469363020542));
#40276=CARTESIAN_POINT('Ctrl Pts',(4.04029392228049,-1.,0.452365214748893));
#40277=CARTESIAN_POINT('Ctrl Pts',(4.04029392228049,1.,0.452365214748893));
#40278=CARTESIAN_POINT('Ctrl Pts',(4.0476929901813,-1.,0.450222009543927));
#40279=CARTESIAN_POINT('Ctrl Pts',(4.0476929901813,1.,0.450222009543927));
#40280=CARTESIAN_POINT('Ctrl Pts',(4.0550903779696,-1.,0.448040082684115));
#40281=CARTESIAN_POINT('Ctrl Pts',(4.0550903779696,1.,0.448040082684115));
#40282=CARTESIAN_POINT('Ctrl Pts',(4.06248560760659,-1.,0.445819737468538));
#40283=CARTESIAN_POINT('Ctrl Pts',(4.06248560760659,1.,0.445819737468538));
#40284=CARTESIAN_POINT('Ctrl Pts',(4.0698782192569,-1.,0.443561262395333));
#40285=CARTESIAN_POINT('Ctrl Pts',(4.0698782192569,1.,0.443561262395333));
#40286=CARTESIAN_POINT('Ctrl Pts',(4.07726792490016,-1.,0.441264951396361));
#40287=CARTESIAN_POINT('Ctrl Pts',(4.07726792490016,1.,0.441264951396361));
#40288=CARTESIAN_POINT('Ctrl Pts',(4.08465462294273,-1.,0.43893110893128));
#40289=CARTESIAN_POINT('Ctrl Pts',(4.08465462294273,1.,0.43893110893128));
#40290=CARTESIAN_POINT('Ctrl Pts',(4.09203832139089,-1.,0.436560044913483));
#40291=CARTESIAN_POINT('Ctrl Pts',(4.09203832139089,1.,0.436560044913483));
#40292=CARTESIAN_POINT('Ctrl Pts',(4.09941908688373,-1.,0.434152073200461));
#40293=CARTESIAN_POINT('Ctrl Pts',(4.09941908688373,1.,0.434152073200461));
#40294=CARTESIAN_POINT('Ctrl Pts',(4.10679698750336,-1.,0.431707508679884));
#40295=CARTESIAN_POINT('Ctrl Pts',(4.10679698750336,1.,0.431707508679884));
#40296=CARTESIAN_POINT('Ctrl Pts',(4.11417202783267,-1.,0.429226666075845));
#40297=CARTESIAN_POINT('Ctrl Pts',(4.11417202783267,1.,0.429226666075845));
#40298=CARTESIAN_POINT('Ctrl Pts',(4.12154412502007,-1.,0.426709855707001));
#40299=CARTESIAN_POINT('Ctrl Pts',(4.12154412502007,1.,0.426709855707001));
#40300=CARTESIAN_POINT('Ctrl Pts',(4.12891314634572,-1.,0.424157375323976));
#40301=CARTESIAN_POINT('Ctrl Pts',(4.12891314634572,1.,0.424157375323976));
#40302=CARTESIAN_POINT('Ctrl Pts',(4.13627893207002,-1.,0.421569503104513));
#40303=CARTESIAN_POINT('Ctrl Pts',(4.13627893207002,1.,0.421569503104513));
#40304=CARTESIAN_POINT('Ctrl Pts',(4.14364132317121,-1.,0.418946490667703));
#40305=CARTESIAN_POINT('Ctrl Pts',(4.14364132317121,1.,0.418946490667703));
#40306=CARTESIAN_POINT('Ctrl Pts',(4.15100018949965,-1.,0.416288556008012));
#40307=CARTESIAN_POINT('Ctrl Pts',(4.15100018949965,1.,0.416288556008012));
#40308=CARTESIAN_POINT('Ctrl Pts',(4.15835545017202,-1.,0.413595877951471));
#40309=CARTESIAN_POINT('Ctrl Pts',(4.15835545017202,1.,0.413595877951471));
#40310=CARTESIAN_POINT('Ctrl Pts',(4.16570705938425,-1.,0.410868596146415));
#40311=CARTESIAN_POINT('Ctrl Pts',(4.16570705938425,1.,0.410868596146415));
#40312=CARTESIAN_POINT('Ctrl Pts',(4.17158541007977,-1.,0.408659167568273));
#40313=CARTESIAN_POINT('Ctrl Pts',(4.17158541007977,1.,0.408659167568273));
#40314=CARTESIAN_POINT('Ctrl Pts',(4.17599251954382,-1.,0.406986596325455));
#40315=CARTESIAN_POINT('Ctrl Pts',(4.17599251954382,1.,0.406986596325455));
#40316=CARTESIAN_POINT('Ctrl Pts',(4.17892985789466,-1.,0.40586466267921));
#40317=CARTESIAN_POINT('Ctrl Pts',(4.17892985789466,1.,0.40586466267921));
#40318=CARTESIAN_POINT('Ctrl Pts',(4.18039834341342,-1.,0.405301974318351));
#40319=CARTESIAN_POINT('Ctrl Pts',(4.18039834341342,1.,0.405301974318351));
#40320=CARTESIAN_POINT('',(3.71701050416825,1.,0.496319364827592));
#40321=CARTESIAN_POINT('Ctrl Pts',(3.71701050416825,-1.,0.496319364827593));
#40322=CARTESIAN_POINT('Ctrl Pts',(3.71701050416825,-0.666666666666667,
0.496319364827593));
#40323=CARTESIAN_POINT('Ctrl Pts',(3.71701050416825,-0.333333333333333,
0.496319364827593));
#40324=CARTESIAN_POINT('Ctrl Pts',(3.71701050416825,0.333333333333333,0.496319364827593));
#40325=CARTESIAN_POINT('Ctrl Pts',(3.71701050416825,0.666666666666667,0.496319364827593));
#40326=CARTESIAN_POINT('Ctrl Pts',(3.71701050416825,1.,0.496319364827593));
#40327=CARTESIAN_POINT('',(4.18039834341342,1.,0.405301974318351));
#40328=CARTESIAN_POINT('',(4.18039834341342,0.,0.405301974318351));
#40329=CARTESIAN_POINT('Ctrl Pts',(3.71701050416825,1.,0.496319364827592));
#40330=CARTESIAN_POINT('Ctrl Pts',(3.71704500630494,1.,0.496354087924312));
#40331=CARTESIAN_POINT('Ctrl Pts',(3.71721917030355,1.,0.496446644158006));
#40332=CARTESIAN_POINT('Ctrl Pts',(3.71785517607548,1.,0.496605651525989));
#40333=CARTESIAN_POINT('Ctrl Pts',(3.71952320822499,1.,0.496846224822564));
#40334=CARTESIAN_POINT('Ctrl Pts',(3.72301489774398,1.,0.497187079575988));
#40335=CARTESIAN_POINT('Ctrl Pts',(3.72830430904606,1.,0.49758406715305));
#40336=CARTESIAN_POINT('Ctrl Pts',(3.73486914372449,1.,0.497984209510025));
#40337=CARTESIAN_POINT('Ctrl Pts',(3.74235701734714,1.,0.498350586057693));
#40338=CARTESIAN_POINT('Ctrl Pts',(3.75037362167839,1.,0.498642802042606));
#40339=CARTESIAN_POINT('Ctrl Pts',(3.75854082221053,1.,0.498823681615422));
#40340=CARTESIAN_POINT('Ctrl Pts',(3.76655401191229,1.,0.498865792335291));
#40341=CARTESIAN_POINT('Ctrl Pts',(3.77425499225255,1.,0.498759900365892));
#40342=CARTESIAN_POINT('Ctrl Pts',(3.78163975337356,1.,0.498515471679585));
#40343=CARTESIAN_POINT('Ctrl Pts',(3.78879701661264,1.,0.498152751800959));
#40344=CARTESIAN_POINT('Ctrl Pts',(3.79586380669994,1.,0.497696892100625));
#40345=CARTESIAN_POINT('Ctrl Pts',(3.80297788298514,1.,0.497171756201052));
#40346=CARTESIAN_POINT('Ctrl Pts',(3.81022254090839,1.,0.496592643443704));
#40347=CARTESIAN_POINT('Ctrl Pts',(3.81760756144025,1.,0.49596393787548));
#40348=CARTESIAN_POINT('Ctrl Pts',(3.82509963594103,1.,0.495283458893838));
#40349=CARTESIAN_POINT('Ctrl Pts',(3.83264092682431,1.,0.494545212256402));
#40350=CARTESIAN_POINT('Ctrl Pts',(3.84017095578451,1.,0.493742574629135));
#40351=CARTESIAN_POINT('Ctrl Pts',(3.84765051147999,1.,0.492871792414141));
#40352=CARTESIAN_POINT('Ctrl Pts',(3.85507287020263,1.,0.491933631083814));
#40353=CARTESIAN_POINT('Ctrl Pts',(3.86245057319246,1.,0.490931482170891));
#40354=CARTESIAN_POINT('Ctrl Pts',(3.86980755613707,1.,0.489870245704918));
#40355=CARTESIAN_POINT('Ctrl Pts',(3.87716963231109,1.,0.488754973798274));
#40356=CARTESIAN_POINT('Ctrl Pts',(3.88455453328138,1.,0.487589452275155));
#40357=CARTESIAN_POINT('Ctrl Pts',(3.89196582437552,1.,0.486375337854104));
#40358=CARTESIAN_POINT('Ctrl Pts',(3.89939844658513,1.,0.485112963522223));
#40359=CARTESIAN_POINT('Ctrl Pts',(3.90684210358056,1.,0.48380183508915));
#40360=CARTESIAN_POINT('Ctrl Pts',(3.91428536373751,1.,0.482441230340714));
#40361=CARTESIAN_POINT('Ctrl Pts',(3.92171976072341,1.,0.481030798910749));
#40362=CARTESIAN_POINT('Ctrl Pts',(3.92914297392071,1.,0.479571028525579));
#40363=CARTESIAN_POINT('Ctrl Pts',(3.93655660689819,1.,0.478062927140965));
#40364=CARTESIAN_POINT('Ctrl Pts',(3.94396469119383,1.,0.476507810658538));
#40365=CARTESIAN_POINT('Ctrl Pts',(3.95137192932897,1.,0.474907053021791));
#40366=CARTESIAN_POINT('Ctrl Pts',(3.95878201038338,1.,0.473261847236298));
#40367=CARTESIAN_POINT('Ctrl Pts',(3.96619600864643,1.,0.471572978413504));
#40368=CARTESIAN_POINT('Ctrl Pts',(3.97361320212436,1.,0.469840942829896));
#40369=CARTESIAN_POINT('Ctrl Pts',(3.98103175589371,1.,0.468066047920158));
#40370=CARTESIAN_POINT('Ctrl Pts',(3.98844946363262,1.,0.46624852088304));
#40371=CARTESIAN_POINT('Ctrl Pts',(3.9958644432011,1.,0.464388610938976));
#40372=CARTESIAN_POINT('Ctrl Pts',(4.00327590659075,1.,0.462486702616205));
#40373=CARTESIAN_POINT('Ctrl Pts',(4.01068390573399,1.,0.460543280768515));
#40374=CARTESIAN_POINT('Ctrl Pts',(4.01808900827587,1.,0.458558885636946));
#40375=CARTESIAN_POINT('Ctrl Pts',(4.02549199038394,1.,0.456534070784951));
#40376=CARTESIAN_POINT('Ctrl Pts',(4.03289354362794,1.,0.454469363020542));
#40377=CARTESIAN_POINT('Ctrl Pts',(4.04029392228049,1.,0.452365214748893));
#40378=CARTESIAN_POINT('Ctrl Pts',(4.0476929901813,1.,0.450222009543927));
#40379=CARTESIAN_POINT('Ctrl Pts',(4.0550903779696,1.,0.448040082684115));
#40380=CARTESIAN_POINT('Ctrl Pts',(4.06248560760659,1.,0.445819737468538));
#40381=CARTESIAN_POINT('Ctrl Pts',(4.0698782192569,1.,0.443561262395333));
#40382=CARTESIAN_POINT('Ctrl Pts',(4.07726792490016,1.,0.441264951396361));
#40383=CARTESIAN_POINT('Ctrl Pts',(4.08465462294273,1.,0.43893110893128));
#40384=CARTESIAN_POINT('Ctrl Pts',(4.09203832139089,1.,0.436560044913483));
#40385=CARTESIAN_POINT('Ctrl Pts',(4.09941908688373,1.,0.434152073200461));
#40386=CARTESIAN_POINT('Ctrl Pts',(4.10679698750336,1.,0.431707508679884));
#40387=CARTESIAN_POINT('Ctrl Pts',(4.11417202783267,1.,0.429226666075845));
#40388=CARTESIAN_POINT('Ctrl Pts',(4.12154412502007,1.,0.426709855707001));
#40389=CARTESIAN_POINT('Ctrl Pts',(4.12891314634572,1.,0.424157375323976));
#40390=CARTESIAN_POINT('Ctrl Pts',(4.13627893207002,1.,0.421569503104513));
#40391=CARTESIAN_POINT('Ctrl Pts',(4.14364132317121,1.,0.418946490667703));
#40392=CARTESIAN_POINT('Ctrl Pts',(4.15100018949965,1.,0.416288556008012));
#40393=CARTESIAN_POINT('Ctrl Pts',(4.15835545017202,1.,0.413595877951471));
#40394=CARTESIAN_POINT('Ctrl Pts',(4.16570705938425,1.,0.410868596146415));
#40395=CARTESIAN_POINT('Ctrl Pts',(4.17158541007977,1.,0.408659167568273));
#40396=CARTESIAN_POINT('Ctrl Pts',(4.17599251954382,1.,0.406986596325455));
#40397=CARTESIAN_POINT('Ctrl Pts',(4.17892985789466,1.,0.40586466267921));
#40398=CARTESIAN_POINT('Ctrl Pts',(4.18039834341342,1.,0.405301974318351));
#40399=CARTESIAN_POINT('Origin',(4.18039834341342,0.,0.405301974318351));
#40400=CARTESIAN_POINT('',(4.1923339003649,1.,0.253646344052522));
#40401=CARTESIAN_POINT('Origin',(0.,0.,0.));
#40402=CARTESIAN_POINT('',(3.68845817949618,1.,0.676591647973661));
#40403=CARTESIAN_POINT('Origin',(0.,1.,0.));
#40404=CARTESIAN_POINT('Ctrl Pts',(3.68845817949618,1.,0.676591647973661));
#40405=CARTESIAN_POINT('Ctrl Pts',(3.68845817949618,0.666666666666667,0.676591647973661));
#40406=CARTESIAN_POINT('Ctrl Pts',(3.68845817949618,0.333333333333333,0.676591647973661));
#40407=CARTESIAN_POINT('Ctrl Pts',(3.68845817949618,-0.333333333333333,
0.676591647973661));
#40408=CARTESIAN_POINT('Ctrl Pts',(3.68845817949618,-0.666666666666667,
0.676591647973662));
#40409=CARTESIAN_POINT('Ctrl Pts',(3.68845817949618,-1.,0.676591647973662));
#40410=CARTESIAN_POINT('Ctrl Pts',(4.10104028313088,-1.,0.906349047628867));
#40411=CARTESIAN_POINT('Ctrl Pts',(4.10104028313088,1.,0.906349047628867));
#40412=CARTESIAN_POINT('Ctrl Pts',(4.09981755067956,-1.,0.905360112216302));
#40413=CARTESIAN_POINT('Ctrl Pts',(4.09981755067956,1.,0.905360112216302));
#40414=CARTESIAN_POINT('Ctrl Pts',(4.09737067247114,-1.,0.903385402444213));
#40415=CARTESIAN_POINT('Ctrl Pts',(4.09737067247114,1.,0.903385402444213));
#40416=CARTESIAN_POINT('Ctrl Pts',(4.09369611524319,-1.,0.900432820945976));
#40417=CARTESIAN_POINT('Ctrl Pts',(4.09369611524319,1.,0.900432820945976));
#40418=CARTESIAN_POINT('Ctrl Pts',(4.08878822249095,-1.,0.896515019236369));
#40419=CARTESIAN_POINT('Ctrl Pts',(4.08878822249095,1.,0.896515019236369));
#40420=CARTESIAN_POINT('Ctrl Pts',(4.08263920306651,-1.,0.891649447920402));
#40421=CARTESIAN_POINT('Ctrl Pts',(4.08263920306651,1.,0.891649447920402));
#40422=CARTESIAN_POINT('Ctrl Pts',(4.07647601774639,-1.,0.886815658360739));
#40423=CARTESIAN_POINT('Ctrl Pts',(4.07647601774639,1.,0.886815658360739));
#40424=CARTESIAN_POINT('Ctrl Pts',(4.07029866694292,-1.,0.882013797525917));
#40425=CARTESIAN_POINT('Ctrl Pts',(4.07029866694292,1.,0.882013797525917));
#40426=CARTESIAN_POINT('Ctrl Pts',(4.06410717232347,-1.,0.877244060484596));
#40427=CARTESIAN_POINT('Ctrl Pts',(4.06410717232347,1.,0.877244060484596));
#40428=CARTESIAN_POINT('Ctrl Pts',(4.05790159030495,-1.,0.872506694780564));
#40429=CARTESIAN_POINT('Ctrl Pts',(4.05790159030495,1.,0.872506694780564));
#40430=CARTESIAN_POINT('Ctrl Pts',(4.05168199437128,-1.,0.867801988858176));
#40431=CARTESIAN_POINT('Ctrl Pts',(4.05168199437128,1.,0.867801988858176));
#40432=CARTESIAN_POINT('Ctrl Pts',(4.04544845048097,-1.,0.863130256642174));
#40433=CARTESIAN_POINT('Ctrl Pts',(4.04544845048097,1.,0.863130256642174));
#40434=CARTESIAN_POINT('Ctrl Pts',(4.03920099284658,-1.,0.858491822322572));
#40435=CARTESIAN_POINT('Ctrl Pts',(4.03920099284658,1.,0.858491822322572));
#40436=CARTESIAN_POINT('Ctrl Pts',(4.03293960436945,-1.,0.853887006632179));
#40437=CARTESIAN_POINT('Ctrl Pts',(4.03293960436945,1.,0.853887006632179));
#40438=CARTESIAN_POINT('Ctrl Pts',(4.02666418343508,-1.,0.849316107475013));
#40439=CARTESIAN_POINT('Ctrl Pts',(4.02666418343508,1.,0.849316107475013));
#40440=CARTESIAN_POINT('Ctrl Pts',(4.02037456798787,-1.,0.844779403288517));
#40441=CARTESIAN_POINT('Ctrl Pts',(4.02037456798787,1.,0.844779403288517));
#40442=CARTESIAN_POINT('Ctrl Pts',(4.01407059766338,-1.,0.840277171976381));
#40443=CARTESIAN_POINT('Ctrl Pts',(4.01407059766338,1.,0.840277171976381));
#40444=CARTESIAN_POINT('Ctrl Pts',(4.00775216907934,-1.,0.835809705809822));
#40445=CARTESIAN_POINT('Ctrl Pts',(4.00775216907934,1.,0.835809705809822));
#40446=CARTESIAN_POINT('Ctrl Pts',(4.00141928477447,-1.,0.831377325741487));
#40447=CARTESIAN_POINT('Ctrl Pts',(4.00141928477447,1.,0.831377325741487));
#40448=CARTESIAN_POINT('Ctrl Pts',(3.99507212784289,-1.,0.826980400320474));
#40449=CARTESIAN_POINT('Ctrl Pts',(3.99507212784289,1.,0.826980400320474));
#40450=CARTESIAN_POINT('Ctrl Pts',(3.98871104646328,-1.,0.82261934602177));
#40451=CARTESIAN_POINT('Ctrl Pts',(3.98871104646328,1.,0.82261934602177));
#40452=CARTESIAN_POINT('Ctrl Pts',(3.98233640155287,-1.,0.818294599022034));
#40453=CARTESIAN_POINT('Ctrl Pts',(3.98233640155287,1.,0.818294599022034));
#40454=CARTESIAN_POINT('Ctrl Pts',(3.97594844078763,-1.,0.814006592328738));
#40455=CARTESIAN_POINT('Ctrl Pts',(3.97594844078763,1.,0.814006592328738));
#40456=CARTESIAN_POINT('Ctrl Pts',(3.96954717513251,-1.,0.809755732818134));
#40457=CARTESIAN_POINT('Ctrl Pts',(3.96954717513251,1.,0.809755732818134));
#40458=CARTESIAN_POINT('Ctrl Pts',(3.96313222295874,-1.,0.805542372178496));
#40459=CARTESIAN_POINT('Ctrl Pts',(3.96313222295874,1.,0.805542372178496));
#40460=CARTESIAN_POINT('Ctrl Pts',(3.95670276375176,-1.,0.801366797727206));
#40461=CARTESIAN_POINT('Ctrl Pts',(3.95670276375176,1.,0.801366797727206));
#40462=CARTESIAN_POINT('Ctrl Pts',(3.95025788827189,-1.,0.797229296085439));
#40463=CARTESIAN_POINT('Ctrl Pts',(3.95025788827189,1.,0.797229296085439));
#40464=CARTESIAN_POINT('Ctrl Pts',(3.94379688971307,-1.,0.793130205641017));
#40465=CARTESIAN_POINT('Ctrl Pts',(3.94379688971307,1.,0.793130205641017));
#40466=CARTESIAN_POINT('Ctrl Pts',(3.93731956885671,-1.,0.789069971469324));
#40467=CARTESIAN_POINT('Ctrl Pts',(3.93731956885671,1.,0.789069971469324));
#40468=CARTESIAN_POINT('Ctrl Pts',(3.93082655631768,-1.,0.785049202786459));
#40469=CARTESIAN_POINT('Ctrl Pts',(3.93082655631768,1.,0.785049202786459));
#40470=CARTESIAN_POINT('Ctrl Pts',(3.92431956510418,-1.,0.781068718228395));
#40471=CARTESIAN_POINT('Ctrl Pts',(3.92431956510418,1.,0.781068718228395));
#40472=CARTESIAN_POINT('Ctrl Pts',(3.91780062334464,-1.,0.777129415664915));
#40473=CARTESIAN_POINT('Ctrl Pts',(3.91780062334464,1.,0.777129415664915));
#40474=CARTESIAN_POINT('Ctrl Pts',(3.91127138115238,-1.,0.773232154506306));
#40475=CARTESIAN_POINT('Ctrl Pts',(3.91127138115238,1.,0.773232154506306));
#40476=CARTESIAN_POINT('Ctrl Pts',(3.90473237182634,-1.,0.769377629847877));
#40477=CARTESIAN_POINT('Ctrl Pts',(3.90473237182634,1.,0.769377629847877));
#40478=CARTESIAN_POINT('Ctrl Pts',(3.89818233104381,-1.,0.765566256401307));
#40479=CARTESIAN_POINT('Ctrl Pts',(3.89818233104381,1.,0.765566256401307));
#40480=CARTESIAN_POINT('Ctrl Pts',(3.89161738162245,-1.,0.761798028793978));
#40481=CARTESIAN_POINT('Ctrl Pts',(3.89161738162245,1.,0.761798028793978));
#40482=CARTESIAN_POINT('Ctrl Pts',(3.88503262662684,-1.,0.758072800564799));
#40483=CARTESIAN_POINT('Ctrl Pts',(3.88503262662684,1.,0.758072800564799));
#40484=CARTESIAN_POINT('Ctrl Pts',(3.87842382520058,-1.,0.754390577396847));
#40485=CARTESIAN_POINT('Ctrl Pts',(3.87842382520058,1.,0.754390577396847));
#40486=CARTESIAN_POINT('Ctrl Pts',(3.87178914078372,-1.,0.750751822383024));
#40487=CARTESIAN_POINT('Ctrl Pts',(3.87178914078372,1.,0.750751822383024));
#40488=CARTESIAN_POINT('Ctrl Pts',(3.86513062969896,-1.,0.747157716488884));
#40489=CARTESIAN_POINT('Ctrl Pts',(3.86513062969896,1.,0.747157716488884));
#40490=CARTESIAN_POINT('Ctrl Pts',(3.85845645217611,-1.,0.743610542737042));
#40491=CARTESIAN_POINT('Ctrl Pts',(3.85845645217611,1.,0.743610542737042));
#40492=CARTESIAN_POINT('Ctrl Pts',(3.85177770351237,-1.,0.740113146827177));
#40493=CARTESIAN_POINT('Ctrl Pts',(3.85177770351237,1.,0.740113146827177));
#40494=CARTESIAN_POINT('Ctrl Pts',(3.84510432881231,-1.,0.736668240497151));
#40495=CARTESIAN_POINT('Ctrl Pts',(3.84510432881231,1.,0.736668240497151));
#40496=CARTESIAN_POINT('Ctrl Pts',(3.83844103658016,-1.,0.733277703756091));
#40497=CARTESIAN_POINT('Ctrl Pts',(3.83844103658016,1.,0.733277703756091));
#40498=CARTESIAN_POINT('Ctrl Pts',(3.8317839240337,-1.,0.729942010490146));
#40499=CARTESIAN_POINT('Ctrl Pts',(3.8317839240337,1.,0.729942010490146));
#40500=CARTESIAN_POINT('Ctrl Pts',(3.82511495756682,-1.,0.726659281876608));
#40501=CARTESIAN_POINT('Ctrl Pts',(3.82511495756682,1.,0.726659281876608));
#40502=CARTESIAN_POINT('Ctrl Pts',(3.81840802610795,-1.,0.72342634601935));
#40503=CARTESIAN_POINT('Ctrl Pts',(3.81840802610795,1.,0.72342634601935));
#40504=CARTESIAN_POINT('Ctrl Pts',(3.81163885127309,-1.,0.720240466589173));
#40505=CARTESIAN_POINT('Ctrl Pts',(3.81163885127309,1.,0.720240466589173));
#40506=CARTESIAN_POINT('Ctrl Pts',(3.80479445759296,-1.,0.717100993669091));
#40507=CARTESIAN_POINT('Ctrl Pts',(3.80479445759296,1.,0.717100993669091));
#40508=CARTESIAN_POINT('Ctrl Pts',(3.79788100314994,-1.,0.714010733006678));
#40509=CARTESIAN_POINT('Ctrl Pts',(3.79788100314994,1.,0.714010733006678));
#40510=CARTESIAN_POINT('Ctrl Pts',(3.79093694007146,-1.,0.710978231689118));
#40511=CARTESIAN_POINT('Ctrl Pts',(3.79093694007146,1.,0.710978231689118));
#40512=CARTESIAN_POINT('Ctrl Pts',(3.78402183336678,-1.,0.7080158793756));
#40513=CARTESIAN_POINT('Ctrl Pts',(3.78402183336678,1.,0.7080158793756));
#40514=CARTESIAN_POINT('Ctrl Pts',(3.77719254217197,-1.,0.70513584799995));
#40515=CARTESIAN_POINT('Ctrl Pts',(3.77719254217197,1.,0.70513584799995));
#40516=CARTESIAN_POINT('Ctrl Pts',(3.77048141872904,-1.,0.702346356621614));
#40517=CARTESIAN_POINT('Ctrl Pts',(3.77048141872904,1.,0.702346356621614));
#40518=CARTESIAN_POINT('Ctrl Pts',(3.76387780603725,-1.,0.699648552230851));
#40519=CARTESIAN_POINT('Ctrl Pts',(3.76387780603725,1.,0.699648552230851));
#40520=CARTESIAN_POINT('Ctrl Pts',(3.75729775766913,-1.,0.69703124565953));
#40521=CARTESIAN_POINT('Ctrl Pts',(3.75729775766913,1.,0.69703124565953));
#40522=CARTESIAN_POINT('Ctrl Pts',(3.7506028824329,-1.,0.694474562581174));
#40523=CARTESIAN_POINT('Ctrl Pts',(3.7506028824329,1.,0.694474562581174));
#40524=CARTESIAN_POINT('Ctrl Pts',(3.74365508986548,-1.,0.691960080400503));
#40525=CARTESIAN_POINT('Ctrl Pts',(3.74365508986548,1.,0.691960080400503));
#40526=CARTESIAN_POINT('Ctrl Pts',(3.73636374474993,-1.,0.689479637354652));
#40527=CARTESIAN_POINT('Ctrl Pts',(3.73636374474993,1.,0.689479637354652));
#40528=CARTESIAN_POINT('Ctrl Pts',(3.72872973554125,-1.,0.687043475232499));
#40529=CARTESIAN_POINT('Ctrl Pts',(3.72872973554125,1.,0.687043475232499));
#40530=CARTESIAN_POINT('Ctrl Pts',(3.7209063713952,-1.,0.684691698168356));
#40531=CARTESIAN_POINT('Ctrl Pts',(3.7209063713952,1.,0.684691698168356));
#40532=CARTESIAN_POINT('Ctrl Pts',(3.71319182790334,-1.,0.68249234510969));
#40533=CARTESIAN_POINT('Ctrl Pts',(3.71319182790334,1.,0.68249234510969));
#40534=CARTESIAN_POINT('Ctrl Pts',(3.70595722032165,-1.,0.680526909711618));
#40535=CARTESIAN_POINT('Ctrl Pts',(3.70595722032165,1.,0.680526909711618));
#40536=CARTESIAN_POINT('Ctrl Pts',(3.69959004073192,-1.,0.67887882222639));
#40537=CARTESIAN_POINT('Ctrl Pts',(3.69959004073192,1.,0.67887882222639));
#40538=CARTESIAN_POINT('Ctrl Pts',(3.69443683573443,-1.,0.677621861865197));
#40539=CARTESIAN_POINT('Ctrl Pts',(3.69443683573443,1.,0.677621861865197));
#40540=CARTESIAN_POINT('Ctrl Pts',(3.69073278191505,-1.,0.676805811074141));
#40541=CARTESIAN_POINT('Ctrl Pts',(3.69073278191505,1.,0.676805811074141));
#40542=CARTESIAN_POINT('Ctrl Pts',(3.68901718135636,-1.,0.676524321060167));
#40543=CARTESIAN_POINT('Ctrl Pts',(3.68901718135636,1.,0.676524321060167));
#40544=CARTESIAN_POINT('Ctrl Pts',(3.68844918120934,-1.,0.676525601650139));
#40545=CARTESIAN_POINT('Ctrl Pts',(3.68844918120934,1.,0.676525601650139));
#40546=CARTESIAN_POINT('Ctrl Pts',(3.68838970675356,-1.,0.676620796001717));
#40547=CARTESIAN_POINT('Ctrl Pts',(3.68838970675356,1.,0.676620796001717));
#40548=CARTESIAN_POINT('Ctrl Pts',(3.68843977377012,-1.,0.676691979611562));
#40549=CARTESIAN_POINT('Ctrl Pts',(3.68843977377012,1.,0.676691979611562));
#40550=CARTESIAN_POINT('',(4.10104028313088,1.,0.906349047628867));
#40551=CARTESIAN_POINT('Ctrl Pts',(4.10104028313088,1.,0.906349047628867));
#40552=CARTESIAN_POINT('Ctrl Pts',(4.09981755067956,1.,0.905360112216302));
#40553=CARTESIAN_POINT('Ctrl Pts',(4.09737067247114,1.,0.903385402444213));
#40554=CARTESIAN_POINT('Ctrl Pts',(4.09369611524319,1.,0.900432820945976));
#40555=CARTESIAN_POINT('Ctrl Pts',(4.08878822249095,1.,0.896515019236369));
#40556=CARTESIAN_POINT('Ctrl Pts',(4.08263920306651,1.,0.891649447920402));
#40557=CARTESIAN_POINT('Ctrl Pts',(4.07647601774639,1.,0.886815658360739));
#40558=CARTESIAN_POINT('Ctrl Pts',(4.07029866694292,1.,0.882013797525917));
#40559=CARTESIAN_POINT('Ctrl Pts',(4.06410717232347,1.,0.877244060484596));
#40560=CARTESIAN_POINT('Ctrl Pts',(4.05790159030495,1.,0.872506694780564));
#40561=CARTESIAN_POINT('Ctrl Pts',(4.05168199437128,1.,0.867801988858176));
#40562=CARTESIAN_POINT('Ctrl Pts',(4.04544845048097,1.,0.863130256642174));
#40563=CARTESIAN_POINT('Ctrl Pts',(4.03920099284658,1.,0.858491822322572));
#40564=CARTESIAN_POINT('Ctrl Pts',(4.03293960436945,1.,0.853887006632179));
#40565=CARTESIAN_POINT('Ctrl Pts',(4.02666418343508,1.,0.849316107475013));
#40566=CARTESIAN_POINT('Ctrl Pts',(4.02037456798787,1.,0.844779403288517));
#40567=CARTESIAN_POINT('Ctrl Pts',(4.01407059766338,1.,0.840277171976381));
#40568=CARTESIAN_POINT('Ctrl Pts',(4.00775216907934,1.,0.835809705809822));
#40569=CARTESIAN_POINT('Ctrl Pts',(4.00141928477447,1.,0.831377325741487));
#40570=CARTESIAN_POINT('Ctrl Pts',(3.99507212784289,1.,0.826980400320474));
#40571=CARTESIAN_POINT('Ctrl Pts',(3.98871104646328,1.,0.82261934602177));
#40572=CARTESIAN_POINT('Ctrl Pts',(3.98233640155287,1.,0.818294599022034));
#40573=CARTESIAN_POINT('Ctrl Pts',(3.97594844078763,1.,0.814006592328738));
#40574=CARTESIAN_POINT('Ctrl Pts',(3.96954717513251,1.,0.809755732818134));
#40575=CARTESIAN_POINT('Ctrl Pts',(3.96313222295874,1.,0.805542372178496));
#40576=CARTESIAN_POINT('Ctrl Pts',(3.95670276375176,1.,0.801366797727206));
#40577=CARTESIAN_POINT('Ctrl Pts',(3.95025788827189,1.,0.797229296085439));
#40578=CARTESIAN_POINT('Ctrl Pts',(3.94379688971307,1.,0.793130205641017));
#40579=CARTESIAN_POINT('Ctrl Pts',(3.93731956885671,1.,0.789069971469324));
#40580=CARTESIAN_POINT('Ctrl Pts',(3.93082655631768,1.,0.785049202786459));
#40581=CARTESIAN_POINT('Ctrl Pts',(3.92431956510418,1.,0.781068718228395));
#40582=CARTESIAN_POINT('Ctrl Pts',(3.91780062334464,1.,0.777129415664915));
#40583=CARTESIAN_POINT('Ctrl Pts',(3.91127138115238,1.,0.773232154506306));
#40584=CARTESIAN_POINT('Ctrl Pts',(3.90473237182634,1.,0.769377629847877));
#40585=CARTESIAN_POINT('Ctrl Pts',(3.89818233104381,1.,0.765566256401307));
#40586=CARTESIAN_POINT('Ctrl Pts',(3.89161738162245,1.,0.761798028793978));
#40587=CARTESIAN_POINT('Ctrl Pts',(3.88503262662684,1.,0.758072800564799));
#40588=CARTESIAN_POINT('Ctrl Pts',(3.87842382520058,1.,0.754390577396847));
#40589=CARTESIAN_POINT('Ctrl Pts',(3.87178914078372,1.,0.750751822383024));
#40590=CARTESIAN_POINT('Ctrl Pts',(3.86513062969896,1.,0.747157716488884));
#40591=CARTESIAN_POINT('Ctrl Pts',(3.85845645217611,1.,0.743610542737042));
#40592=CARTESIAN_POINT('Ctrl Pts',(3.85177770351237,1.,0.740113146827177));
#40593=CARTESIAN_POINT('Ctrl Pts',(3.84510432881231,1.,0.736668240497151));
#40594=CARTESIAN_POINT('Ctrl Pts',(3.83844103658016,1.,0.733277703756091));
#40595=CARTESIAN_POINT('Ctrl Pts',(3.8317839240337,1.,0.729942010490146));
#40596=CARTESIAN_POINT('Ctrl Pts',(3.82511495756682,1.,0.726659281876608));
#40597=CARTESIAN_POINT('Ctrl Pts',(3.81840802610795,1.,0.72342634601935));
#40598=CARTESIAN_POINT('Ctrl Pts',(3.81163885127309,1.,0.720240466589173));
#40599=CARTESIAN_POINT('Ctrl Pts',(3.80479445759296,1.,0.717100993669091));
#40600=CARTESIAN_POINT('Ctrl Pts',(3.79788100314994,1.,0.714010733006678));
#40601=CARTESIAN_POINT('Ctrl Pts',(3.79093694007146,1.,0.710978231689118));
#40602=CARTESIAN_POINT('Ctrl Pts',(3.78402183336678,1.,0.7080158793756));
#40603=CARTESIAN_POINT('Ctrl Pts',(3.77719254217197,1.,0.70513584799995));
#40604=CARTESIAN_POINT('Ctrl Pts',(3.77048141872904,1.,0.702346356621614));
#40605=CARTESIAN_POINT('Ctrl Pts',(3.76387780603725,1.,0.699648552230851));
#40606=CARTESIAN_POINT('Ctrl Pts',(3.75729775766913,1.,0.69703124565953));
#40607=CARTESIAN_POINT('Ctrl Pts',(3.7506028824329,1.,0.694474562581174));
#40608=CARTESIAN_POINT('Ctrl Pts',(3.74365508986548,1.,0.691960080400503));
#40609=CARTESIAN_POINT('Ctrl Pts',(3.73636374474993,1.,0.689479637354652));
#40610=CARTESIAN_POINT('Ctrl Pts',(3.72872973554125,1.,0.687043475232499));
#40611=CARTESIAN_POINT('Ctrl Pts',(3.7209063713952,1.,0.684691698168356));
#40612=CARTESIAN_POINT('Ctrl Pts',(3.71319182790334,1.,0.68249234510969));
#40613=CARTESIAN_POINT('Ctrl Pts',(3.70595722032165,1.,0.680526909711618));
#40614=CARTESIAN_POINT('Ctrl Pts',(3.69959004073192,1.,0.67887882222639));
#40615=CARTESIAN_POINT('Ctrl Pts',(3.69443683573443,1.,0.677621861865197));
#40616=CARTESIAN_POINT('Ctrl Pts',(3.6910107117555,1.,0.676867042599712));
#40617=CARTESIAN_POINT('Ctrl Pts',(3.68934997767391,1.,0.676580391119535));
#40618=CARTESIAN_POINT('Ctrl Pts',(3.68869596426099,1.,0.676535079520366));
#40619=CARTESIAN_POINT('Ctrl Pts',(3.68850172300543,1.,0.67656928609342));
#40620=CARTESIAN_POINT('Ctrl Pts',(3.68845817949618,1.,0.676591647973661));
#40621=CARTESIAN_POINT('',(4.10104028313088,0.,0.906349047628867));
#40622=CARTESIAN_POINT('Ctrl Pts',(3.59363563249864,-1.,1.07157964745328));
#40623=CARTESIAN_POINT('Ctrl Pts',(3.59363563249864,1.,1.07157964745328));
#40624=CARTESIAN_POINT('Ctrl Pts',(3.59355870577901,-1.,1.07162034256459));
#40625=CARTESIAN_POINT('Ctrl Pts',(3.59355870577901,1.,1.07162034256459));
#40626=CARTESIAN_POINT('Ctrl Pts',(3.59356848057812,-1.,1.07173216219145));
#40627=CARTESIAN_POINT('Ctrl Pts',(3.59356848057812,1.,1.07173216219145));
#40628=CARTESIAN_POINT('Ctrl Pts',(3.5940739910409,-1.,1.07199116987656));
#40629=CARTESIAN_POINT('Ctrl Pts',(3.5940739910409,1.,1.07199116987656));
#40630=CARTESIAN_POINT('Ctrl Pts',(3.59573039612316,-1.,1.07251922679245));
#40631=CARTESIAN_POINT('Ctrl Pts',(3.59573039612316,1.,1.07251922679245));
#40632=CARTESIAN_POINT('Ctrl Pts',(3.59940121154535,-1.,1.07347372545714));
#40633=CARTESIAN_POINT('Ctrl Pts',(3.59940121154535,1.,1.07347372545714));
#40634=CARTESIAN_POINT('Ctrl Pts',(3.60456339887778,-1.,1.07469327168578));
#40635=CARTESIAN_POINT('Ctrl Pts',(3.60456339887778,1.,1.07469327168578));
#40636=CARTESIAN_POINT('Ctrl Pts',(3.61098481349204,-1.,1.07611545402734));
#40637=CARTESIAN_POINT('Ctrl Pts',(3.61098481349204,1.,1.07611545402734));
#40638=CARTESIAN_POINT('Ctrl Pts',(3.61832318504574,-1.,1.07764868137619));
#40639=CARTESIAN_POINT('Ctrl Pts',(3.61832318504574,1.,1.07764868137619));
#40640=CARTESIAN_POINT('Ctrl Pts',(3.62619537902361,-1.,1.07919137290742));
#40641=CARTESIAN_POINT('Ctrl Pts',(3.62619537902361,1.,1.07919137290742));
#40642=CARTESIAN_POINT('Ctrl Pts',(3.63423373196529,-1.,1.08064765719867));
#40643=CARTESIAN_POINT('Ctrl Pts',(3.63423373196529,1.,1.08064765719867));
#40644=CARTESIAN_POINT('Ctrl Pts',(3.64214167843677,-1.,1.08194278850996));
#40645=CARTESIAN_POINT('Ctrl Pts',(3.64214167843677,1.,1.08194278850996));
#40646=CARTESIAN_POINT('Ctrl Pts',(3.64976441208358,-1.,1.08304289898623));
#40647=CARTESIAN_POINT('Ctrl Pts',(3.64976441208358,1.,1.08304289898623));
#40648=CARTESIAN_POINT('Ctrl Pts',(3.65709649161166,-1.,1.08395671077807));
#40649=CARTESIAN_POINT('Ctrl Pts',(3.65709649161166,1.,1.08395671077807));
#40650=CARTESIAN_POINT('Ctrl Pts',(3.66422237895365,-1.,1.08471809922901));
#40651=CARTESIAN_POINT('Ctrl Pts',(3.66422237895365,1.,1.08471809922901));
#40652=CARTESIAN_POINT('Ctrl Pts',(3.67127347729666,-1.,1.0853733414449));
#40653=CARTESIAN_POINT('Ctrl Pts',(3.67127347729666,1.,1.0853733414449));
#40654=CARTESIAN_POINT('Ctrl Pts',(3.67838211685117,-1.,1.0859675575576));
#40655=CARTESIAN_POINT('Ctrl Pts',(3.67838211685117,1.,1.0859675575576));
#40656=CARTESIAN_POINT('Ctrl Pts',(3.68562817420797,-1.,1.0865288888259));
#40657=CARTESIAN_POINT('Ctrl Pts',(3.68562817420797,1.,1.0865288888259));
#40658=CARTESIAN_POINT('Ctrl Pts',(3.69302062410157,-1.,1.08706319540271));
#40659=CARTESIAN_POINT('Ctrl Pts',(3.69302062410157,1.,1.08706319540271));
#40660=CARTESIAN_POINT('Ctrl Pts',(3.70052690909833,-1.,1.08756311291309));
#40661=CARTESIAN_POINT('Ctrl Pts',(3.70052690909833,1.,1.08756311291309));
#40662=CARTESIAN_POINT('Ctrl Pts',(3.70809084139457,-1.,1.08801367312185));
#40663=CARTESIAN_POINT('Ctrl Pts',(3.70809084139457,1.,1.08801367312185));
#40664=CARTESIAN_POINT('Ctrl Pts',(3.71565372339075,-1.,1.0883988733478));
#40665=CARTESIAN_POINT('Ctrl Pts',(3.71565372339075,1.,1.0883988733478));
#40666=CARTESIAN_POINT('Ctrl Pts',(3.72317741369398,-1.,1.08870887220082));
#40667=CARTESIAN_POINT('Ctrl Pts',(3.72317741369398,1.,1.08870887220082));
#40668=CARTESIAN_POINT('Ctrl Pts',(3.73065515162988,-1.,1.08894337390937));
#40669=CARTESIAN_POINT('Ctrl Pts',(3.73065515162988,1.,1.08894337390937));
#40670=CARTESIAN_POINT('Ctrl Pts',(3.73809879348239,-1.,1.08910769013298));
#40671=CARTESIAN_POINT('Ctrl Pts',(3.73809879348239,1.,1.08910769013298));
#40672=CARTESIAN_POINT('Ctrl Pts',(3.74553121371757,-1.,1.08921040494017));
#40673=CARTESIAN_POINT('Ctrl Pts',(3.74553121371757,1.,1.08921040494017));
#40674=CARTESIAN_POINT('Ctrl Pts',(3.75297711748132,-1.,1.08926054632925));
#40675=CARTESIAN_POINT('Ctrl Pts',(3.75297711748132,1.,1.08926054632925));
#40676=CARTESIAN_POINT('Ctrl Pts',(3.76045342580208,-1.,1.08926462734282));
#40677=CARTESIAN_POINT('Ctrl Pts',(3.76045342580208,1.,1.08926462734282));
#40678=CARTESIAN_POINT('Ctrl Pts',(3.76796340094448,-1.,1.08922484204256));
#40679=CARTESIAN_POINT('Ctrl Pts',(3.76796340094448,1.,1.08922484204256));
#40680=CARTESIAN_POINT('Ctrl Pts',(3.77550199409424,-1.,1.0891407279127));
#40681=CARTESIAN_POINT('Ctrl Pts',(3.77550199409424,1.,1.0891407279127));
#40682=CARTESIAN_POINT('Ctrl Pts',(3.78305911299504,-1.,1.08901018614636));
#40683=CARTESIAN_POINT('Ctrl Pts',(3.78305911299504,1.,1.08901018614636));
#40684=CARTESIAN_POINT('Ctrl Pts',(3.79062357974404,-1.,1.08883071512098));
#40685=CARTESIAN_POINT('Ctrl Pts',(3.79062357974404,1.,1.08883071512098));
#40686=CARTESIAN_POINT('Ctrl Pts',(3.79818708705259,-1.,1.08860064435778));
#40687=CARTESIAN_POINT('Ctrl Pts',(3.79818708705259,1.,1.08860064435778));
#40688=CARTESIAN_POINT('Ctrl Pts',(3.8057472665766,-1.,1.0883200925538));
#40689=CARTESIAN_POINT('Ctrl Pts',(3.8057472665766,1.,1.0883200925538));
#40690=CARTESIAN_POINT('Ctrl Pts',(3.81330554446323,-1.,1.08799030610862));
#40691=CARTESIAN_POINT('Ctrl Pts',(3.81330554446323,1.,1.08799030610862));
#40692=CARTESIAN_POINT('Ctrl Pts',(3.82086569676319,-1.,1.08761321539442));
#40693=CARTESIAN_POINT('Ctrl Pts',(3.82086569676319,1.,1.08761321539442));
#40694=CARTESIAN_POINT('Ctrl Pts',(3.82843215316984,-1.,1.08719091307558));
#40695=CARTESIAN_POINT('Ctrl Pts',(3.82843215316984,1.,1.08719091307558));
#40696=CARTESIAN_POINT('Ctrl Pts',(3.83600837071708,-1.,1.08672515456902));
#40697=CARTESIAN_POINT('Ctrl Pts',(3.83600837071708,1.,1.08672515456902));
#40698=CARTESIAN_POINT('Ctrl Pts',(3.8435952876495,-1.,1.08621688337604));
#40699=CARTESIAN_POINT('Ctrl Pts',(3.8435952876495,1.,1.08621688337604));
#40700=CARTESIAN_POINT('Ctrl Pts',(3.85119211322755,-1.,1.08566647671844));
#40701=CARTESIAN_POINT('Ctrl Pts',(3.85119211322755,1.,1.08566647671844));
#40702=CARTESIAN_POINT('Ctrl Pts',(3.85879698702532,-1.,1.08507395120059));
#40703=CARTESIAN_POINT('Ctrl Pts',(3.85879698702532,1.,1.08507395120059));
#40704=CARTESIAN_POINT('Ctrl Pts',(3.86640769434274,-1.,1.08443918607927));
#40705=CARTESIAN_POINT('Ctrl Pts',(3.86640769434274,1.,1.08443918607927));
#40706=CARTESIAN_POINT('Ctrl Pts',(3.8740223372254,-1.,1.08376213307504));
#40707=CARTESIAN_POINT('Ctrl Pts',(3.8740223372254,1.,1.08376213307504));
#40708=CARTESIAN_POINT('Ctrl Pts',(3.88164007721312,-1.,1.08304304871029));
#40709=CARTESIAN_POINT('Ctrl Pts',(3.88164007721312,1.,1.08304304871029));
#40710=CARTESIAN_POINT('Ctrl Pts',(3.88926088975114,-1.,1.08228241999346));
#40711=CARTESIAN_POINT('Ctrl Pts',(3.88926088975114,1.,1.08228241999346));
#40712=CARTESIAN_POINT('Ctrl Pts',(3.8968852509835,-1.,1.08148086931358));
#40713=CARTESIAN_POINT('Ctrl Pts',(3.8968852509835,1.,1.08148086931358));
#40714=CARTESIAN_POINT('Ctrl Pts',(3.90451384092545,-1.,1.08063906483818));
#40715=CARTESIAN_POINT('Ctrl Pts',(3.90451384092545,1.,1.08063906483818));
#40716=CARTESIAN_POINT('Ctrl Pts',(3.91214726022143,-1.,1.07975763507473));
#40717=CARTESIAN_POINT('Ctrl Pts',(3.91214726022143,1.,1.07975763507473));
#40718=CARTESIAN_POINT('Ctrl Pts',(3.91978568924178,-1.,1.07883706663554));
#40719=CARTESIAN_POINT('Ctrl Pts',(3.91978568924178,1.,1.07883706663554));
#40720=CARTESIAN_POINT('Ctrl Pts',(3.9274289334984,-1.,1.07787771707195));
#40721=CARTESIAN_POINT('Ctrl Pts',(3.9274289334984,1.,1.07787771707195));
#40722=CARTESIAN_POINT('Ctrl Pts',(3.93507657572883,-1.,1.07687985975384));
#40723=CARTESIAN_POINT('Ctrl Pts',(3.93507657572883,1.,1.07687985975384));
#40724=CARTESIAN_POINT('Ctrl Pts',(3.94272809633331,-1.,1.07584371946443));
#40725=CARTESIAN_POINT('Ctrl Pts',(3.94272809633331,1.,1.07584371946443));
#40726=CARTESIAN_POINT('Ctrl Pts',(3.95038299600676,-1.,1.07476950921587));
#40727=CARTESIAN_POINT('Ctrl Pts',(3.95038299600676,1.,1.07476950921587));
#40728=CARTESIAN_POINT('Ctrl Pts',(3.95804094429373,-1.,1.07365747426491));
#40729=CARTESIAN_POINT('Ctrl Pts',(3.95804094429373,1.,1.07365747426491));
#40730=CARTESIAN_POINT('Ctrl Pts',(3.96570179322338,-1.,1.07250789943007));
#40731=CARTESIAN_POINT('Ctrl Pts',(3.96570179322338,1.,1.07250789943007));
#40732=CARTESIAN_POINT('Ctrl Pts',(3.9733655022223,-1.,1.07132109206164));
#40733=CARTESIAN_POINT('Ctrl Pts',(3.9733655022223,1.,1.07132109206164));
#40734=CARTESIAN_POINT('Ctrl Pts',(3.98103208801101,-1.,1.07009737257767));
#40735=CARTESIAN_POINT('Ctrl Pts',(3.98103208801101,1.,1.07009737257767));
#40736=CARTESIAN_POINT('Ctrl Pts',(3.98870156857412,-1.,1.06883706263942));
#40737=CARTESIAN_POINT('Ctrl Pts',(3.98870156857412,1.,1.06883706263942));
#40738=CARTESIAN_POINT('Ctrl Pts',(3.99637389920441,-1.,1.06754047381312));
#40739=CARTESIAN_POINT('Ctrl Pts',(3.99637389920441,1.,1.06754047381312));
#40740=CARTESIAN_POINT('Ctrl Pts',(4.00404894952579,-1.,1.06620789963606));
#40741=CARTESIAN_POINT('Ctrl Pts',(4.00404894952579,1.,1.06620789963606));
#40742=CARTESIAN_POINT('Ctrl Pts',(4.01172654187398,-1.,1.0648396134311));
#40743=CARTESIAN_POINT('Ctrl Pts',(4.01172654187398,1.,1.0648396134311));
#40744=CARTESIAN_POINT('Ctrl Pts',(4.01940647495943,-1.,1.06343586496236));
#40745=CARTESIAN_POINT('Ctrl Pts',(4.01940647495943,1.,1.06343586496236));
#40746=CARTESIAN_POINT('Ctrl Pts',(4.02708855235633,-1.,1.06199687787462));
#40747=CARTESIAN_POINT('Ctrl Pts',(4.02708855235633,1.,1.06199687787462));
#40748=CARTESIAN_POINT('Ctrl Pts',(4.03477261141553,-1.,1.06052284711857));
#40749=CARTESIAN_POINT('Ctrl Pts',(4.03477261141553,1.,1.06052284711857));
#40750=CARTESIAN_POINT('Ctrl Pts',(4.04245854427496,-1.,1.05901393666567));
#40751=CARTESIAN_POINT('Ctrl Pts',(4.04245854427496,1.,1.05901393666567));
#40752=CARTESIAN_POINT('Ctrl Pts',(4.05014628384869,-1.,1.05747027727959));
#40753=CARTESIAN_POINT('Ctrl Pts',(4.05014628384869,1.,1.05747027727959));
#40754=CARTESIAN_POINT('Ctrl Pts',(4.05629789307025,-1.,1.05620762707996));
#40755=CARTESIAN_POINT('Ctrl Pts',(4.05629789307025,1.,1.05620762707996));
#40756=CARTESIAN_POINT('Ctrl Pts',(4.06091239149123,-1.,1.055245071776));
#40757=CARTESIAN_POINT('Ctrl Pts',(4.06091239149123,1.,1.055245071776));
#40758=CARTESIAN_POINT('Ctrl Pts',(4.06398907542249,-1.,1.05459645194823));
#40759=CARTESIAN_POINT('Ctrl Pts',(4.06398907542249,1.,1.05459645194823));
#40760=CARTESIAN_POINT('Ctrl Pts',(4.06552750530042,-1.,1.05427041296137));
#40761=CARTESIAN_POINT('Ctrl Pts',(4.06552750530042,1.,1.05427041296137));
#40762=CARTESIAN_POINT('',(3.59360648251073,1.,1.07167739962028));
#40763=CARTESIAN_POINT('Ctrl Pts',(3.59360648251073,-1.,1.07167739962028));
#40764=CARTESIAN_POINT('Ctrl Pts',(3.59360648251073,-0.666666666666667,
1.07167739962028));
#40765=CARTESIAN_POINT('Ctrl Pts',(3.59360648251073,-0.333333333333333,
1.07167739962028));
#40766=CARTESIAN_POINT('Ctrl Pts',(3.59360648251073,0.333333333333333,1.07167739962028));
#40767=CARTESIAN_POINT('Ctrl Pts',(3.59360648251073,0.666666666666667,1.07167739962028));
#40768=CARTESIAN_POINT('Ctrl Pts',(3.59360648251073,1.,1.07167739962028));
#40769=CARTESIAN_POINT('',(4.06552750530042,1.,1.05427041296137));
#40770=CARTESIAN_POINT('',(4.06552750530042,0.,1.05427041296137));
#40771=CARTESIAN_POINT('Ctrl Pts',(3.59360648251073,1.,1.07167739962028));
#40772=CARTESIAN_POINT('Ctrl Pts',(3.5936351279798,1.,1.07171709254135));
#40773=CARTESIAN_POINT('Ctrl Pts',(3.59379266874567,1.,1.07183575450617));
#40774=CARTESIAN_POINT('Ctrl Pts',(3.59439596999862,1.,1.07209229745229));
#40775=CARTESIAN_POINT('Ctrl Pts',(3.59600583194946,1.,1.07259084660936));
#40776=CARTESIAN_POINT('Ctrl Pts',(3.59940121154535,1.,1.07347372545714));
#40777=CARTESIAN_POINT('Ctrl Pts',(3.60456339887778,1.,1.07469327168578));
#40778=CARTESIAN_POINT('Ctrl Pts',(3.61098481349204,1.,1.07611545402734));
#40779=CARTESIAN_POINT('Ctrl Pts',(3.61832318504574,1.,1.07764868137619));
#40780=CARTESIAN_POINT('Ctrl Pts',(3.62619537902361,1.,1.07919137290742));
#40781=CARTESIAN_POINT('Ctrl Pts',(3.63423373196529,1.,1.08064765719867));
#40782=CARTESIAN_POINT('Ctrl Pts',(3.64214167843677,1.,1.08194278850996));
#40783=CARTESIAN_POINT('Ctrl Pts',(3.64976441208358,1.,1.08304289898623));
#40784=CARTESIAN_POINT('Ctrl Pts',(3.65709649161166,1.,1.08395671077807));
#40785=CARTESIAN_POINT('Ctrl Pts',(3.66422237895365,1.,1.08471809922901));
#40786=CARTESIAN_POINT('Ctrl Pts',(3.67127347729666,1.,1.0853733414449));
#40787=CARTESIAN_POINT('Ctrl Pts',(3.67838211685117,1.,1.0859675575576));
#40788=CARTESIAN_POINT('Ctrl Pts',(3.68562817420797,1.,1.0865288888259));
#40789=CARTESIAN_POINT('Ctrl Pts',(3.69302062410157,1.,1.08706319540271));
#40790=CARTESIAN_POINT('Ctrl Pts',(3.70052690909833,1.,1.08756311291309));
#40791=CARTESIAN_POINT('Ctrl Pts',(3.70809084139457,1.,1.08801367312185));
#40792=CARTESIAN_POINT('Ctrl Pts',(3.71565372339075,1.,1.0883988733478));
#40793=CARTESIAN_POINT('Ctrl Pts',(3.72317741369398,1.,1.08870887220082));
#40794=CARTESIAN_POINT('Ctrl Pts',(3.73065515162988,1.,1.08894337390937));
#40795=CARTESIAN_POINT('Ctrl Pts',(3.73809879348239,1.,1.08910769013298));
#40796=CARTESIAN_POINT('Ctrl Pts',(3.74553121371757,1.,1.08921040494017));
#40797=CARTESIAN_POINT('Ctrl Pts',(3.75297711748132,1.,1.08926054632925));
#40798=CARTESIAN_POINT('Ctrl Pts',(3.76045342580208,1.,1.08926462734282));
#40799=CARTESIAN_POINT('Ctrl Pts',(3.76796340094448,1.,1.08922484204256));
#40800=CARTESIAN_POINT('Ctrl Pts',(3.77550199409424,1.,1.0891407279127));
#40801=CARTESIAN_POINT('Ctrl Pts',(3.78305911299504,1.,1.08901018614636));
#40802=CARTESIAN_POINT('Ctrl Pts',(3.79062357974404,1.,1.08883071512098));
#40803=CARTESIAN_POINT('Ctrl Pts',(3.79818708705259,1.,1.08860064435778));
#40804=CARTESIAN_POINT('Ctrl Pts',(3.8057472665766,1.,1.0883200925538));
#40805=CARTESIAN_POINT('Ctrl Pts',(3.81330554446323,1.,1.08799030610862));
#40806=CARTESIAN_POINT('Ctrl Pts',(3.82086569676319,1.,1.08761321539442));
#40807=CARTESIAN_POINT('Ctrl Pts',(3.82843215316984,1.,1.08719091307558));
#40808=CARTESIAN_POINT('Ctrl Pts',(3.83600837071708,1.,1.08672515456902));
#40809=CARTESIAN_POINT('Ctrl Pts',(3.8435952876495,1.,1.08621688337604));
#40810=CARTESIAN_POINT('Ctrl Pts',(3.85119211322755,1.,1.08566647671844));
#40811=CARTESIAN_POINT('Ctrl Pts',(3.85879698702532,1.,1.08507395120059));
#40812=CARTESIAN_POINT('Ctrl Pts',(3.86640769434274,1.,1.08443918607927));
#40813=CARTESIAN_POINT('Ctrl Pts',(3.8740223372254,1.,1.08376213307504));
#40814=CARTESIAN_POINT('Ctrl Pts',(3.88164007721312,1.,1.08304304871029));
#40815=CARTESIAN_POINT('Ctrl Pts',(3.88926088975114,1.,1.08228241999346));
#40816=CARTESIAN_POINT('Ctrl Pts',(3.8968852509835,1.,1.08148086931358));
#40817=CARTESIAN_POINT('Ctrl Pts',(3.90451384092545,1.,1.08063906483818));
#40818=CARTESIAN_POINT('Ctrl Pts',(3.91214726022143,1.,1.07975763507473));
#40819=CARTESIAN_POINT('Ctrl Pts',(3.91978568924178,1.,1.07883706663554));
#40820=CARTESIAN_POINT('Ctrl Pts',(3.9274289334984,1.,1.07787771707195));
#40821=CARTESIAN_POINT('Ctrl Pts',(3.93507657572883,1.,1.07687985975384));
#40822=CARTESIAN_POINT('Ctrl Pts',(3.94272809633331,1.,1.07584371946443));
#40823=CARTESIAN_POINT('Ctrl Pts',(3.95038299600676,1.,1.07476950921587));
#40824=CARTESIAN_POINT('Ctrl Pts',(3.95804094429373,1.,1.07365747426491));
#40825=CARTESIAN_POINT('Ctrl Pts',(3.96570179322338,1.,1.07250789943007));
#40826=CARTESIAN_POINT('Ctrl Pts',(3.9733655022223,1.,1.07132109206164));
#40827=CARTESIAN_POINT('Ctrl Pts',(3.98103208801101,1.,1.07009737257767));
#40828=CARTESIAN_POINT('Ctrl Pts',(3.98870156857412,1.,1.06883706263942));
#40829=CARTESIAN_POINT('Ctrl Pts',(3.99637389920441,1.,1.06754047381312));
#40830=CARTESIAN_POINT('Ctrl Pts',(4.00404894952579,1.,1.06620789963606));
#40831=CARTESIAN_POINT('Ctrl Pts',(4.01172654187398,1.,1.0648396134311));
#40832=CARTESIAN_POINT('Ctrl Pts',(4.01940647495943,1.,1.06343586496236));
#40833=CARTESIAN_POINT('Ctrl Pts',(4.02708855235633,1.,1.06199687787462));
#40834=CARTESIAN_POINT('Ctrl Pts',(4.03477261141553,1.,1.06052284711857));
#40835=CARTESIAN_POINT('Ctrl Pts',(4.04245854427496,1.,1.05901393666567));
#40836=CARTESIAN_POINT('Ctrl Pts',(4.05014628384869,1.,1.05747027727959));
#40837=CARTESIAN_POINT('Ctrl Pts',(4.05629789307025,1.,1.05620762707996));
#40838=CARTESIAN_POINT('Ctrl Pts',(4.06091239149123,1.,1.055245071776));
#40839=CARTESIAN_POINT('Ctrl Pts',(4.06398907542249,1.,1.05459645194823));
#40840=CARTESIAN_POINT('Ctrl Pts',(4.06552750530042,1.,1.05427041296137));
#40841=CARTESIAN_POINT('Origin',(4.06552750530042,0.,1.05427041296137));
#40842=CARTESIAN_POINT('',(4.10104028313088,1.,0.906349047628867));
#40843=CARTESIAN_POINT('Origin',(0.,0.,0.));
#40844=CARTESIAN_POINT('',(3.5372048861597,1.,1.24526366418038));
#40845=CARTESIAN_POINT('Origin',(0.,1.,0.));
#40846=CARTESIAN_POINT('Ctrl Pts',(3.5372048861597,1.,1.24526366418038));
#40847=CARTESIAN_POINT('Ctrl Pts',(3.5372048861597,0.666666666666667,1.24526366418038));
#40848=CARTESIAN_POINT('Ctrl Pts',(3.5372048861597,0.333333333333333,1.24526366418038));
#40849=CARTESIAN_POINT('Ctrl Pts',(3.5372048861597,-0.333333333333333,1.24526366418038));
#40850=CARTESIAN_POINT('Ctrl Pts',(3.5372048861597,-0.666666666666667,1.24526366418038));
#40851=CARTESIAN_POINT('Ctrl Pts',(3.5372048861597,-1.,1.24526366418038));
#40852=CARTESIAN_POINT('Ctrl Pts',(3.90876544355381,-1.,1.53673442965256));
#40853=CARTESIAN_POINT('Ctrl Pts',(3.90876544355381,1.,1.53673442965256));
#40854=CARTESIAN_POINT('Ctrl Pts',(3.90771246855019,-1.,1.53556639217905));
#40855=CARTESIAN_POINT('Ctrl Pts',(3.90771246855019,1.,1.53556639217905));
#40856=CARTESIAN_POINT('Ctrl Pts',(3.90560462813969,-1.,1.53323321827755));
#40857=CARTESIAN_POINT('Ctrl Pts',(3.90560462813969,1.,1.53323321827755));
#40858=CARTESIAN_POINT('Ctrl Pts',(3.90243719631596,-1.,1.52974216056287));
#40859=CARTESIAN_POINT('Ctrl Pts',(3.90243719631596,1.,1.52974216056287));
#40860=CARTESIAN_POINT('Ctrl Pts',(3.89820260708225,-1.,1.52510482991635));
#40861=CARTESIAN_POINT('Ctrl Pts',(3.89820260708225,1.,1.52510482991635));
#40862=CARTESIAN_POINT('Ctrl Pts',(3.89289043533657,-1.,1.51933724329306));
#40863=CARTESIAN_POINT('Ctrl Pts',(3.89289043533657,1.,1.51933724329306));
#40864=CARTESIAN_POINT('Ctrl Pts',(3.88755930033884,-1.,1.51359883110559));
#40865=CARTESIAN_POINT('Ctrl Pts',(3.88755930033884,1.,1.51359883110559));
#40866=CARTESIAN_POINT('Ctrl Pts',(3.88220917950538,-1.,1.50788973857757));
#40867=CARTESIAN_POINT('Ctrl Pts',(3.88220917950538,1.,1.50788973857757));
#40868=CARTESIAN_POINT('Ctrl Pts',(3.87684006372134,-1.,1.50221016176556));
#40869=CARTESIAN_POINT('Ctrl Pts',(3.87684006372134,1.,1.50221016176556));
#40870=CARTESIAN_POINT('Ctrl Pts',(3.87145196998465,-1.,1.49656035399122));
#40871=CARTESIAN_POINT('Ctrl Pts',(3.87145196998465,1.,1.49656035399122));
#40872=CARTESIAN_POINT('Ctrl Pts',(3.86604492575189,-1.,1.4909406116431));
#40873=CARTESIAN_POINT('Ctrl Pts',(3.86604492575189,1.,1.4909406116431));
#40874=CARTESIAN_POINT('Ctrl Pts',(3.86061894706087,-1.,1.48535125509919));
#40875=CARTESIAN_POINT('Ctrl Pts',(3.86061894706087,1.,1.48535125509919));
#40876=CARTESIAN_POINT('Ctrl Pts',(3.85517401698843,-1.,1.4797926099102));
#40877=CARTESIAN_POINT('Ctrl Pts',(3.85517401698843,1.,1.4797926099102));
#40878=CARTESIAN_POINT('Ctrl Pts',(3.84971006847277,-1.,1.47426499018538));
#40879=CARTESIAN_POINT('Ctrl Pts',(3.84971006847277,1.,1.47426499018538));
#40880=CARTESIAN_POINT('Ctrl Pts',(3.84422695454796,-1.,1.46876867426504));
#40881=CARTESIAN_POINT('Ctrl Pts',(3.84422695454796,1.,1.46876867426504));
#40882=CARTESIAN_POINT('Ctrl Pts',(3.83872447159639,-1.,1.46330391180752));
#40883=CARTESIAN_POINT('Ctrl Pts',(3.83872447159639,1.,1.46330391180752));
#40884=CARTESIAN_POINT('Ctrl Pts',(3.83320241775423,-1.,1.45787095220852));
#40885=CARTESIAN_POINT('Ctrl Pts',(3.83320241775423,1.,1.45787095220852));
#40886=CARTESIAN_POINT('Ctrl Pts',(3.82766064519074,-1.,1.45247006796836));
#40887=CARTESIAN_POINT('Ctrl Pts',(3.82766064519074,1.,1.45247006796836));
#40888=CARTESIAN_POINT('Ctrl Pts',(3.82209910620533,-1.,1.44710157648539));
#40889=CARTESIAN_POINT('Ctrl Pts',(3.82209910620533,1.,1.44710157648539));
#40890=CARTESIAN_POINT('Ctrl Pts',(3.81651792398414,-1.,1.44176587041347));
#40891=CARTESIAN_POINT('Ctrl Pts',(3.81651792398414,1.,1.44176587041347));
#40892=CARTESIAN_POINT('Ctrl Pts',(3.81091737726815,-1.,1.43646341556724));
#40893=CARTESIAN_POINT('Ctrl Pts',(3.81091737726815,1.,1.43646341556724));
#40894=CARTESIAN_POINT('Ctrl Pts',(3.80529775429805,-1.,1.4311946992132));
#40895=CARTESIAN_POINT('Ctrl Pts',(3.80529775429805,1.,1.4311946992132));
#40896=CARTESIAN_POINT('Ctrl Pts',(3.7996592319632,-1.,1.42596018777283));
#40897=CARTESIAN_POINT('Ctrl Pts',(3.7996592319632,1.,1.42596018777283));
#40898=CARTESIAN_POINT('Ctrl Pts',(3.79400175744408,-1.,1.42076028482836));
#40899=CARTESIAN_POINT('Ctrl Pts',(3.79400175744408,1.,1.42076028482836));
#40900=CARTESIAN_POINT('Ctrl Pts',(3.78832489879426,-1.,1.4155952780383));
#40901=CARTESIAN_POINT('Ctrl Pts',(3.78832489879426,1.,1.4155952780383));
#40902=CARTESIAN_POINT('Ctrl Pts',(3.78262780065471,-1.,1.41046532282593));
#40903=CARTESIAN_POINT('Ctrl Pts',(3.78262780065471,1.,1.41046532282593));
#40904=CARTESIAN_POINT('Ctrl Pts',(3.77690952014259,-1.,1.40537056004722));
#40905=CARTESIAN_POINT('Ctrl Pts',(3.77690952014259,1.,1.40537056004722));
#40906=CARTESIAN_POINT('Ctrl Pts',(3.77116930621827,-1.,1.40031121335505));
#40907=CARTESIAN_POINT('Ctrl Pts',(3.77116930621827,1.,1.40031121335505));
#40908=CARTESIAN_POINT('Ctrl Pts',(3.76540689249074,-1.,1.39528769118052));
#40909=CARTESIAN_POINT('Ctrl Pts',(3.76540689249074,1.,1.39528769118052));
#40910=CARTESIAN_POINT('Ctrl Pts',(3.75962280650855,-1.,1.39030069388918));
#40911=CARTESIAN_POINT('Ctrl Pts',(3.75962280650855,1.,1.39030069388918));
#40912=CARTESIAN_POINT('Ctrl Pts',(3.75381861212707,-1.,1.38535129801176));
#40913=CARTESIAN_POINT('Ctrl Pts',(3.75381861212707,1.,1.38535129801176));
#40914=CARTESIAN_POINT('Ctrl Pts',(3.74799617204729,-1.,1.38044070763295));
#40915=CARTESIAN_POINT('Ctrl Pts',(3.74799617204729,1.,1.38044070763295));
#40916=CARTESIAN_POINT('Ctrl Pts',(3.74215698162555,-1.,1.37557002971687));
#40917=CARTESIAN_POINT('Ctrl Pts',(3.74215698162555,1.,1.37557002971687));
#40918=CARTESIAN_POINT('Ctrl Pts',(3.7363014588581,-1.,1.37074003422739));
#40919=CARTESIAN_POINT('Ctrl Pts',(3.7363014588581,1.,1.37074003422739));
#40920=CARTESIAN_POINT('Ctrl Pts',(3.73042829011295,-1.,1.36595093298676));
#40921=CARTESIAN_POINT('Ctrl Pts',(3.73042829011295,1.,1.36595093298676));
#40922=CARTESIAN_POINT('Ctrl Pts',(3.72453364678279,-1.,1.36120211416354));
#40923=CARTESIAN_POINT('Ctrl Pts',(3.72453364678279,1.,1.36120211416354));
#40924=CARTESIAN_POINT('Ctrl Pts',(3.71861271513313,-1.,1.35649266705037));
#40925=CARTESIAN_POINT('Ctrl Pts',(3.71861271513313,1.,1.35649266705037));
#40926=CARTESIAN_POINT('Ctrl Pts',(3.71266130563054,-1.,1.35182193384424));
#40927=CARTESIAN_POINT('Ctrl Pts',(3.71266130563054,1.,1.35182193384424));
#40928=CARTESIAN_POINT('Ctrl Pts',(3.70667753188248,-1.,1.34719008463534));
#40929=CARTESIAN_POINT('Ctrl Pts',(3.70667753188248,1.,1.34719008463534));
#40930=CARTESIAN_POINT('Ctrl Pts',(3.70066324015119,-1.,1.34259860752933));
#40931=CARTESIAN_POINT('Ctrl Pts',(3.70066324015119,1.,1.34259860752933));
#40932=CARTESIAN_POINT('Ctrl Pts',(3.69462613305708,-1.,1.3380510339822));
#40933=CARTESIAN_POINT('Ctrl Pts',(3.69462613305708,1.,1.3380510339822));
#40934=CARTESIAN_POINT('Ctrl Pts',(3.68857672413033,-1.,1.33355191034523));
#40935=CARTESIAN_POINT('Ctrl Pts',(3.68857672413033,1.,1.33355191034523));
#40936=CARTESIAN_POINT('Ctrl Pts',(3.68252441182551,-1.,1.3291054707274));
#40937=CARTESIAN_POINT('Ctrl Pts',(3.68252441182551,1.,1.3291054707274));
#40938=CARTESIAN_POINT('Ctrl Pts',(3.67647355257912,-1.,1.32471430856415));
#40939=CARTESIAN_POINT('Ctrl Pts',(3.67647355257912,1.,1.32471430856415));
#40940=CARTESIAN_POINT('Ctrl Pts',(3.67042021752656,-1.,1.32037828137766));
#40941=CARTESIAN_POINT('Ctrl Pts',(3.67042021752656,1.,1.32037828137766));
#40942=CARTESIAN_POINT('Ctrl Pts',(3.66434688899793,-1.,1.31609271239911));
#40943=CARTESIAN_POINT('Ctrl Pts',(3.66434688899793,1.,1.31609271239911));
#40944=CARTESIAN_POINT('Ctrl Pts',(3.65822827358617,-1.,1.31185038411218));
#40945=CARTESIAN_POINT('Ctrl Pts',(3.65822827358617,1.,1.31185038411218));
#40946=CARTESIAN_POINT('Ctrl Pts',(3.65204081987068,-1.,1.30764479590039));
#40947=CARTESIAN_POINT('Ctrl Pts',(3.65204081987068,1.,1.30764479590039));
#40948=CARTESIAN_POINT('Ctrl Pts',(3.64577181380113,-1.,1.30347327603774));
#40949=CARTESIAN_POINT('Ctrl Pts',(3.64577181380113,1.,1.30347327603774));
#40950=CARTESIAN_POINT('Ctrl Pts',(3.63942689872808,-1.,1.2993395590647));
#40951=CARTESIAN_POINT('Ctrl Pts',(3.63942689872808,1.,1.2993395590647));
#40952=CARTESIAN_POINT('Ctrl Pts',(3.63304271631046,-1.,1.29525810207762));
#40953=CARTESIAN_POINT('Ctrl Pts',(3.63304271631046,1.,1.29525810207762));
#40954=CARTESIAN_POINT('Ctrl Pts',(3.62667616004369,-1.,1.29125046021878));
#40955=CARTESIAN_POINT('Ctrl Pts',(3.62667616004369,1.,1.29125046021878));
#40956=CARTESIAN_POINT('Ctrl Pts',(3.6203814849236,-1.,1.28733755029384));
#40957=CARTESIAN_POINT('Ctrl Pts',(3.6203814849236,1.,1.28733755029384));
#40958=CARTESIAN_POINT('Ctrl Pts',(3.61418935913823,-1.,1.28353255117765));
#40959=CARTESIAN_POINT('Ctrl Pts',(3.61418935913823,1.,1.28353255117765));
#40960=CARTESIAN_POINT('Ctrl Pts',(3.60808907746339,-1.,1.27983492861691));
#40961=CARTESIAN_POINT('Ctrl Pts',(3.60808907746339,1.,1.27983492861691));
#40962=CARTESIAN_POINT('Ctrl Pts',(3.60199947736298,-1.,1.27622049908625));
#40963=CARTESIAN_POINT('Ctrl Pts',(3.60199947736298,1.,1.27622049908625));
#40964=CARTESIAN_POINT('Ctrl Pts',(3.59578698050006,-1.,1.27264798379307));
#40965=CARTESIAN_POINT('Ctrl Pts',(3.59578698050006,1.,1.27264798379307));
#40966=CARTESIAN_POINT('Ctrl Pts',(3.58931807846313,-1.,1.26907758484709));
#40967=CARTESIAN_POINT('Ctrl Pts',(3.58931807846313,1.,1.26907758484709));
#40968=CARTESIAN_POINT('Ctrl Pts',(3.58250452868618,-1.,1.26548706249862));
#40969=CARTESIAN_POINT('Ctrl Pts',(3.58250452868618,1.,1.26548706249862));
#40970=CARTESIAN_POINT('Ctrl Pts',(3.5753456065171,-1.,1.2618866714281));
#40971=CARTESIAN_POINT('Ctrl Pts',(3.5753456065171,1.,1.2618866714281));
#40972=CARTESIAN_POINT('Ctrl Pts',(3.56798645995275,-1.,1.25834000485716));
#40973=CARTESIAN_POINT('Ctrl Pts',(3.56798645995275,1.,1.25834000485716));
#40974=CARTESIAN_POINT('Ctrl Pts',(3.56071094991199,-1.,1.25496090900009));
#40975=CARTESIAN_POINT('Ctrl Pts',(3.56071094991199,1.,1.25496090900009));
#40976=CARTESIAN_POINT('Ctrl Pts',(3.55387287418985,-1.,1.2518879294064));
#40977=CARTESIAN_POINT('Ctrl Pts',(3.55387287418985,1.,1.2518879294064));
#40978=CARTESIAN_POINT('Ctrl Pts',(3.54784190283068,-1.,1.24926408628003));
#40979=CARTESIAN_POINT('Ctrl Pts',(3.54784190283068,1.,1.24926408628003));
#40980=CARTESIAN_POINT('Ctrl Pts',(3.54294877425964,-1.,1.24721646231966));
#40981=CARTESIAN_POINT('Ctrl Pts',(3.54294877425964,1.,1.24721646231966));
#40982=CARTESIAN_POINT('Ctrl Pts',(3.53941798195825,-1.,1.24583101679029));
#40983=CARTESIAN_POINT('Ctrl Pts',(3.53941798195825,1.,1.24583101679029));
#40984=CARTESIAN_POINT('Ctrl Pts',(3.53776753802906,-1.,1.24528461332987));
#40985=CARTESIAN_POINT('Ctrl Pts',(3.53776753802906,1.,1.24528461332987));
#40986=CARTESIAN_POINT('Ctrl Pts',(3.53720633057798,-1.,1.24519702335451));
#40987=CARTESIAN_POINT('Ctrl Pts',(3.53720633057798,1.,1.24519702335451));
#40988=CARTESIAN_POINT('Ctrl Pts',(3.53713269667399,-1.,1.24528174185098));
#40989=CARTESIAN_POINT('Ctrl Pts',(3.53713269667399,1.,1.24528174185098));
#40990=CARTESIAN_POINT('Ctrl Pts',(3.53717101171257,-1.,1.24535988127942));
#40991=CARTESIAN_POINT('Ctrl Pts',(3.53717101171257,1.,1.24535988127942));
#40992=CARTESIAN_POINT('',(3.90876544355381,1.,1.53673442965256));
#40993=CARTESIAN_POINT('Ctrl Pts',(3.90876544355381,1.,1.53673442965256));
#40994=CARTESIAN_POINT('Ctrl Pts',(3.90771246855019,1.,1.53556639217905));
#40995=CARTESIAN_POINT('Ctrl Pts',(3.90560462813969,1.,1.53323321827755));
#40996=CARTESIAN_POINT('Ctrl Pts',(3.90243719631596,1.,1.52974216056287));
#40997=CARTESIAN_POINT('Ctrl Pts',(3.89820260708225,1.,1.52510482991635));
#40998=CARTESIAN_POINT('Ctrl Pts',(3.89289043533657,1.,1.51933724329306));
#40999=CARTESIAN_POINT('Ctrl Pts',(3.88755930033884,1.,1.51359883110559));
#41000=CARTESIAN_POINT('Ctrl Pts',(3.88220917950538,1.,1.50788973857757));
#41001=CARTESIAN_POINT('Ctrl Pts',(3.87684006372134,1.,1.50221016176556));
#41002=CARTESIAN_POINT('Ctrl Pts',(3.87145196998465,1.,1.49656035399122));
#41003=CARTESIAN_POINT('Ctrl Pts',(3.86604492575189,1.,1.4909406116431));
#41004=CARTESIAN_POINT('Ctrl Pts',(3.86061894706087,1.,1.48535125509919));
#41005=CARTESIAN_POINT('Ctrl Pts',(3.85517401698843,1.,1.4797926099102));
#41006=CARTESIAN_POINT('Ctrl Pts',(3.84971006847277,1.,1.47426499018538));
#41007=CARTESIAN_POINT('Ctrl Pts',(3.84422695454796,1.,1.46876867426504));
#41008=CARTESIAN_POINT('Ctrl Pts',(3.83872447159639,1.,1.46330391180752));
#41009=CARTESIAN_POINT('Ctrl Pts',(3.83320241775423,1.,1.45787095220852));
#41010=CARTESIAN_POINT('Ctrl Pts',(3.82766064519074,1.,1.45247006796836));
#41011=CARTESIAN_POINT('Ctrl Pts',(3.82209910620533,1.,1.44710157648539));
#41012=CARTESIAN_POINT('Ctrl Pts',(3.81651792398414,1.,1.44176587041347));
#41013=CARTESIAN_POINT('Ctrl Pts',(3.81091737726815,1.,1.43646341556724));
#41014=CARTESIAN_POINT('Ctrl Pts',(3.80529775429805,1.,1.4311946992132));
#41015=CARTESIAN_POINT('Ctrl Pts',(3.7996592319632,1.,1.42596018777283));
#41016=CARTESIAN_POINT('Ctrl Pts',(3.79400175744408,1.,1.42076028482836));
#41017=CARTESIAN_POINT('Ctrl Pts',(3.78832489879426,1.,1.4155952780383));
#41018=CARTESIAN_POINT('Ctrl Pts',(3.78262780065471,1.,1.41046532282593));
#41019=CARTESIAN_POINT('Ctrl Pts',(3.77690952014259,1.,1.40537056004722));
#41020=CARTESIAN_POINT('Ctrl Pts',(3.77116930621827,1.,1.40031121335505));
#41021=CARTESIAN_POINT('Ctrl Pts',(3.76540689249074,1.,1.39528769118052));
#41022=CARTESIAN_POINT('Ctrl Pts',(3.75962280650855,1.,1.39030069388918));
#41023=CARTESIAN_POINT('Ctrl Pts',(3.75381861212707,1.,1.38535129801176));
#41024=CARTESIAN_POINT('Ctrl Pts',(3.74799617204729,1.,1.38044070763295));
#41025=CARTESIAN_POINT('Ctrl Pts',(3.74215698162555,1.,1.37557002971687));
#41026=CARTESIAN_POINT('Ctrl Pts',(3.7363014588581,1.,1.37074003422739));
#41027=CARTESIAN_POINT('Ctrl Pts',(3.73042829011295,1.,1.36595093298676));
#41028=CARTESIAN_POINT('Ctrl Pts',(3.72453364678279,1.,1.36120211416354));
#41029=CARTESIAN_POINT('Ctrl Pts',(3.71861271513313,1.,1.35649266705037));
#41030=CARTESIAN_POINT('Ctrl Pts',(3.71266130563054,1.,1.35182193384424));
#41031=CARTESIAN_POINT('Ctrl Pts',(3.70667753188248,1.,1.34719008463534));
#41032=CARTESIAN_POINT('Ctrl Pts',(3.70066324015119,1.,1.34259860752933));
#41033=CARTESIAN_POINT('Ctrl Pts',(3.69462613305708,1.,1.3380510339822));
#41034=CARTESIAN_POINT('Ctrl Pts',(3.68857672413033,1.,1.33355191034523));
#41035=CARTESIAN_POINT('Ctrl Pts',(3.68252441182551,1.,1.3291054707274));
#41036=CARTESIAN_POINT('Ctrl Pts',(3.67647355257912,1.,1.32471430856415));
#41037=CARTESIAN_POINT('Ctrl Pts',(3.67042021752656,1.,1.32037828137766));
#41038=CARTESIAN_POINT('Ctrl Pts',(3.66434688899793,1.,1.31609271239911));
#41039=CARTESIAN_POINT('Ctrl Pts',(3.65822827358617,1.,1.31185038411218));
#41040=CARTESIAN_POINT('Ctrl Pts',(3.65204081987068,1.,1.30764479590039));
#41041=CARTESIAN_POINT('Ctrl Pts',(3.64577181380113,1.,1.30347327603774));
#41042=CARTESIAN_POINT('Ctrl Pts',(3.63942689872808,1.,1.2993395590647));
#41043=CARTESIAN_POINT('Ctrl Pts',(3.63304271631046,1.,1.29525810207762));
#41044=CARTESIAN_POINT('Ctrl Pts',(3.62667616004369,1.,1.29125046021878));
#41045=CARTESIAN_POINT('Ctrl Pts',(3.6203814849236,1.,1.28733755029384));
#41046=CARTESIAN_POINT('Ctrl Pts',(3.61418935913823,1.,1.28353255117765));
#41047=CARTESIAN_POINT('Ctrl Pts',(3.60808907746339,1.,1.27983492861691));
#41048=CARTESIAN_POINT('Ctrl Pts',(3.60199947736298,1.,1.27622049908625));
#41049=CARTESIAN_POINT('Ctrl Pts',(3.59578698050006,1.,1.27264798379307));
#41050=CARTESIAN_POINT('Ctrl Pts',(3.58931807846313,1.,1.26907758484709));
#41051=CARTESIAN_POINT('Ctrl Pts',(3.58250452868618,1.,1.26548706249862));
#41052=CARTESIAN_POINT('Ctrl Pts',(3.5753456065171,1.,1.2618866714281));
#41053=CARTESIAN_POINT('Ctrl Pts',(3.56798645995275,1.,1.25834000485716));
#41054=CARTESIAN_POINT('Ctrl Pts',(3.56071094991199,1.,1.25496090900009));
#41055=CARTESIAN_POINT('Ctrl Pts',(3.55387287418985,1.,1.2518879294064));
#41056=CARTESIAN_POINT('Ctrl Pts',(3.54784190283068,1.,1.24926408628003));
#41057=CARTESIAN_POINT('Ctrl Pts',(3.54294877425964,1.,1.24721646231966));
#41058=CARTESIAN_POINT('Ctrl Pts',(3.53968291130022,1.,1.24593497226008));
#41059=CARTESIAN_POINT('Ctrl Pts',(3.53808746578196,1.,1.24539205388767));
#41060=CARTESIAN_POINT('Ctrl Pts',(3.5374485926552,1.,1.2452449899111));
#41061=CARTESIAN_POINT('Ctrl Pts',(3.53725139174486,1.,1.24524838931757));
#41062=CARTESIAN_POINT('Ctrl Pts',(3.5372048861597,1.,1.24526366418038));
#41063=CARTESIAN_POINT('',(3.90876544355381,0.,1.53673442965256));
#41064=CARTESIAN_POINT('Ctrl Pts',(3.38176002566879,-1.,1.62055519152809));
#41065=CARTESIAN_POINT('Ctrl Pts',(3.38176002566879,1.,1.62055519152809));
#41066=CARTESIAN_POINT('Ctrl Pts',(3.38167767992676,-1.,1.62058335162482));
#41067=CARTESIAN_POINT('Ctrl Pts',(3.38167767992676,1.,1.62058335162482));
#41068=CARTESIAN_POINT('Ctrl Pts',(3.38166984193836,-1.,1.62069532368199));
#41069=CARTESIAN_POINT('Ctrl Pts',(3.38166984193836,1.,1.62069532368199));
#41070=CARTESIAN_POINT('Ctrl Pts',(3.38212861099983,-1.,1.62103022181151));
#41071=CARTESIAN_POINT('Ctrl Pts',(3.38212861099983,1.,1.62103022181151));
#41072=CARTESIAN_POINT('Ctrl Pts',(3.38368201668574,-1.,1.62181089631344));
#41073=CARTESIAN_POINT('Ctrl Pts',(3.38368201668574,1.,1.62181089631344));
#41074=CARTESIAN_POINT('Ctrl Pts',(3.38715832179072,-1.,1.6233278855625));
#41075=CARTESIAN_POINT('Ctrl Pts',(3.38715832179072,1.,1.6233278855625));
#41076=CARTESIAN_POINT('Ctrl Pts',(3.39206617496906,-1.,1.62533996116713));
#41077=CARTESIAN_POINT('Ctrl Pts',(3.39206617496906,1.,1.62533996116713));
#41078=CARTESIAN_POINT('Ctrl Pts',(3.39818605297991,-1.,1.62774916464408));
#41079=CARTESIAN_POINT('Ctrl Pts',(3.39818605297991,1.,1.62774916464408));
#41080=CARTESIAN_POINT('Ctrl Pts',(3.40519422740235,-1.,1.63041148964828));
#41081=CARTESIAN_POINT('Ctrl Pts',(3.40519422740235,1.,1.63041148964828));
#41082=CARTESIAN_POINT('Ctrl Pts',(3.41272817148478,-1.,1.63316667054044));
#41083=CARTESIAN_POINT('Ctrl Pts',(3.41272817148478,1.,1.63316667054044));
#41084=CARTESIAN_POINT('Ctrl Pts',(3.42043974590882,-1.,1.63586250099773));
#41085=CARTESIAN_POINT('Ctrl Pts',(3.42043974590882,1.,1.63586250099773));
#41086=CARTESIAN_POINT('Ctrl Pts',(3.42804772926291,-1.,1.63837876246926));
#41087=CARTESIAN_POINT('Ctrl Pts',(3.42804772926291,1.,1.63837876246926));
#41088=CARTESIAN_POINT('Ctrl Pts',(3.43540451921548,-1.,1.64065778702023));
#41089=CARTESIAN_POINT('Ctrl Pts',(3.43540451921548,1.,1.64065778702023));
#41090=CARTESIAN_POINT('Ctrl Pts',(3.44250337701888,-1.,1.64270733821113));
#41091=CARTESIAN_POINT('Ctrl Pts',(3.44250337701888,1.,1.64270733821113));
#41092=CARTESIAN_POINT('Ctrl Pts',(3.44942242546795,-1.,1.64457408708107));
#41093=CARTESIAN_POINT('Ctrl Pts',(3.44942242546795,1.,1.64457408708107));
#41094=CARTESIAN_POINT('Ctrl Pts',(3.45628421062422,-1.,1.64632429697521));
#41095=CARTESIAN_POINT('Ctrl Pts',(3.45628421062422,1.,1.64632429697521));
#41096=CARTESIAN_POINT('Ctrl Pts',(3.46321237515,-1.,1.64802323352738));
#41097=CARTESIAN_POINT('Ctrl Pts',(3.46321237515,1.,1.64802323352738));
#41098=CARTESIAN_POINT('Ctrl Pts',(3.47028140995992,-1.,1.64971118698256));
#41099=CARTESIAN_POINT('Ctrl Pts',(3.47028140995992,1.,1.64971118698256));
#41100=CARTESIAN_POINT('Ctrl Pts',(3.47749926256476,-1.,1.65139534930322));
#41101=CARTESIAN_POINT('Ctrl Pts',(3.47749926256476,1.,1.65139534930322));
#41102=CARTESIAN_POINT('Ctrl Pts',(3.48483492840894,-1.,1.65306335367739));
#41103=CARTESIAN_POINT('Ctrl Pts',(3.48483492840894,1.,1.65306335367739));
#41104=CARTESIAN_POINT('Ctrl Pts',(3.49223525300176,-1.,1.65469162644468));
#41105=CARTESIAN_POINT('Ctrl Pts',(3.49223525300176,1.,1.65469162644468));
#41106=CARTESIAN_POINT('Ctrl Pts',(3.4996447647794,-1.,1.65625517961588));
#41107=CARTESIAN_POINT('Ctrl Pts',(3.4996447647794,1.,1.65625517961588));
#41108=CARTESIAN_POINT('Ctrl Pts',(3.50702733146542,-1.,1.65773832633632));
#41109=CARTESIAN_POINT('Ctrl Pts',(3.50702733146542,1.,1.65773832633632));
#41110=CARTESIAN_POINT('Ctrl Pts',(3.5143763218894,-1.,1.65913971687342));
#41111=CARTESIAN_POINT('Ctrl Pts',(3.5143763218894,1.,1.65913971687342));
#41112=CARTESIAN_POINT('Ctrl Pts',(3.52170261543815,-1.,1.66046645222279));
#41113=CARTESIAN_POINT('Ctrl Pts',(3.52170261543815,1.,1.66046645222279));
#41114=CARTESIAN_POINT('Ctrl Pts',(3.52902746211093,-1.,1.66173058912371));
#41115=CARTESIAN_POINT('Ctrl Pts',(3.52902746211093,1.,1.66173058912371));
#41116=CARTESIAN_POINT('Ctrl Pts',(3.5363738506022,-1.,1.66294490916111));
#41117=CARTESIAN_POINT('Ctrl Pts',(3.5363738506022,1.,1.66294490916111));
#41118=CARTESIAN_POINT('Ctrl Pts',(3.54375747475014,-1.,1.66411849222326));
#41119=CARTESIAN_POINT('Ctrl Pts',(3.54375747475014,1.,1.66411849222326));
#41120=CARTESIAN_POINT('Ctrl Pts',(3.55118121342861,-1.,1.66525401568994));
#41121=CARTESIAN_POINT('Ctrl Pts',(3.55118121342861,1.,1.66525401568994));
#41122=CARTESIAN_POINT('Ctrl Pts',(3.55864015233602,-1.,1.66635023293114));
#41123=CARTESIAN_POINT('Ctrl Pts',(3.55864015233602,1.,1.66635023293114));
#41124=CARTESIAN_POINT('Ctrl Pts',(3.56612465179422,-1.,1.66740349220305));
#41125=CARTESIAN_POINT('Ctrl Pts',(3.56612465179422,1.,1.66740349220305));
#41126=CARTESIAN_POINT('Ctrl Pts',(3.57362406285887,-1.,1.668409574073));
#41127=CARTESIAN_POINT('Ctrl Pts',(3.57362406285887,1.,1.668409574073));
#41128=CARTESIAN_POINT('Ctrl Pts',(3.58113044183829,-1.,1.66936552908232));
#41129=CARTESIAN_POINT('Ctrl Pts',(3.58113044183829,1.,1.66936552908232));
#41130=CARTESIAN_POINT('Ctrl Pts',(3.58864143097834,-1.,1.67027110397604));
#41131=CARTESIAN_POINT('Ctrl Pts',(3.58864143097834,1.,1.67027110397604));
#41132=CARTESIAN_POINT('Ctrl Pts',(3.59615824388807,-1.,1.67112775290707));
#41133=CARTESIAN_POINT('Ctrl Pts',(3.59615824388807,1.,1.67112775290707));
#41134=CARTESIAN_POINT('Ctrl Pts',(3.603684308152,-1.,1.67193797318597));
#41135=CARTESIAN_POINT('Ctrl Pts',(3.603684308152,1.,1.67193797318597));
#41136=CARTESIAN_POINT('Ctrl Pts',(3.61122367156181,-1.,1.67270452466968));
#41137=CARTESIAN_POINT('Ctrl Pts',(3.61122367156181,1.,1.67270452466968));
#41138=CARTESIAN_POINT('Ctrl Pts',(3.61877947398184,-1.,1.67342968196224));
#41139=CARTESIAN_POINT('Ctrl Pts',(3.61877947398184,1.,1.67342968196224));
#41140=CARTESIAN_POINT('Ctrl Pts',(3.62635249450923,-1.,1.67411452372271));
#41141=CARTESIAN_POINT('Ctrl Pts',(3.62635249450923,1.,1.67411452372271));
#41142=CARTESIAN_POINT('Ctrl Pts',(3.63394189312924,-1.,1.67475929882971));
#41143=CARTESIAN_POINT('Ctrl Pts',(3.63394189312924,1.,1.67475929882971));
#41144=CARTESIAN_POINT('Ctrl Pts',(3.6415458297234,-1.,1.67536373264848));
#41145=CARTESIAN_POINT('Ctrl Pts',(3.6415458297234,1.,1.67536373264848));
#41146=CARTESIAN_POINT('Ctrl Pts',(3.64916213574667,-1.,1.67592735946692));
#41147=CARTESIAN_POINT('Ctrl Pts',(3.64916213574667,1.,1.67592735946692));
#41148=CARTESIAN_POINT('Ctrl Pts',(3.6567889441642,-1.,1.6764498346945));
#41149=CARTESIAN_POINT('Ctrl Pts',(3.6567889441642,1.,1.6764498346945));
#41150=CARTESIAN_POINT('Ctrl Pts',(3.66442538670968,-1.,1.67693128053132));
#41151=CARTESIAN_POINT('Ctrl Pts',(3.66442538670968,1.,1.67693128053132));
#41152=CARTESIAN_POINT('Ctrl Pts',(3.67207136294575,-1.,1.67737217414874));
#41153=CARTESIAN_POINT('Ctrl Pts',(3.67207136294575,1.,1.67737217414874));
#41154=CARTESIAN_POINT('Ctrl Pts',(3.67972724579124,-1.,1.67777320475848));
#41155=CARTESIAN_POINT('Ctrl Pts',(3.67972724579124,1.,1.67777320475848));
#41156=CARTESIAN_POINT('Ctrl Pts',(3.68739360236487,-1.,1.67813513867965));
#41157=CARTESIAN_POINT('Ctrl Pts',(3.68739360236487,1.,1.67813513867965));
#41158=CARTESIAN_POINT('Ctrl Pts',(3.6950709275959,-1.,1.67845869064323));
#41159=CARTESIAN_POINT('Ctrl Pts',(3.6950709275959,1.,1.67845869064323));
#41160=CARTESIAN_POINT('Ctrl Pts',(3.70275932351108,-1.,1.67874436948667));
#41161=CARTESIAN_POINT('Ctrl Pts',(3.70275932351108,1.,1.67874436948667));
#41162=CARTESIAN_POINT('Ctrl Pts',(3.71045854208343,-1.,1.67899249793462));
#41163=CARTESIAN_POINT('Ctrl Pts',(3.71045854208343,1.,1.67899249793462));
#41164=CARTESIAN_POINT('Ctrl Pts',(3.71816812842322,-1.,1.67920328071708));
#41165=CARTESIAN_POINT('Ctrl Pts',(3.71816812842322,1.,1.67920328071708));
#41166=CARTESIAN_POINT('Ctrl Pts',(3.72588753416396,-1.,1.67937685856652));
#41167=CARTESIAN_POINT('Ctrl Pts',(3.72588753416396,1.,1.67937685856652));
#41168=CARTESIAN_POINT('Ctrl Pts',(3.73361623282543,-1.,1.67951336376402));
#41169=CARTESIAN_POINT('Ctrl Pts',(3.73361623282543,1.,1.67951336376402));
#41170=CARTESIAN_POINT('Ctrl Pts',(3.74135385965401,-1.,1.6796129868522));
#41171=CARTESIAN_POINT('Ctrl Pts',(3.74135385965401,1.,1.6796129868522));
#41172=CARTESIAN_POINT('Ctrl Pts',(3.7491002239452,-1.,1.67967598599525));
#41173=CARTESIAN_POINT('Ctrl Pts',(3.7491002239452,1.,1.67967598599525));
#41174=CARTESIAN_POINT('Ctrl Pts',(3.75685523754493,-1.,1.67970265841239));
#41175=CARTESIAN_POINT('Ctrl Pts',(3.75685523754493,1.,1.67970265841239));
#41176=CARTESIAN_POINT('Ctrl Pts',(3.76461886684344,-1.,1.67969332319245));
#41177=CARTESIAN_POINT('Ctrl Pts',(3.76461886684344,1.,1.67969332319245));
#41178=CARTESIAN_POINT('Ctrl Pts',(3.77239107928502,-1.,1.67964830084993));
#41179=CARTESIAN_POINT('Ctrl Pts',(3.77239107928502,1.,1.67964830084993));
#41180=CARTESIAN_POINT('Ctrl Pts',(3.78017178197317,-1.,1.67956789212141));
#41181=CARTESIAN_POINT('Ctrl Pts',(3.78017178197317,1.,1.67956789212141));
#41182=CARTESIAN_POINT('Ctrl Pts',(3.7879608002176,-1.,1.67945236653493));
#41183=CARTESIAN_POINT('Ctrl Pts',(3.7879608002176,1.,1.67945236653493));
#41184=CARTESIAN_POINT('Ctrl Pts',(3.79575791578424,-1.,1.67930196625548));
#41185=CARTESIAN_POINT('Ctrl Pts',(3.79575791578424,1.,1.67930196625548));
#41186=CARTESIAN_POINT('Ctrl Pts',(3.80356289079005,-1.,1.67911690648355));
#41187=CARTESIAN_POINT('Ctrl Pts',(3.80356289079005,1.,1.67911690648355));
#41188=CARTESIAN_POINT('Ctrl Pts',(3.81137549624178,-1.,1.6788973773827));
#41189=CARTESIAN_POINT('Ctrl Pts',(3.81137549624178,1.,1.6788973773827));
#41190=CARTESIAN_POINT('Ctrl Pts',(3.81919554099578,-1.,1.67864354605954));
#41191=CARTESIAN_POINT('Ctrl Pts',(3.81919554099578,1.,1.67864354605954));
#41192=CARTESIAN_POINT('Ctrl Pts',(3.82702289286713,-1.,1.6783555575934));
#41193=CARTESIAN_POINT('Ctrl Pts',(3.82702289286713,1.,1.6783555575934));
#41194=CARTESIAN_POINT('Ctrl Pts',(3.83485746513989,-1.,1.67803353064351));
#41195=CARTESIAN_POINT('Ctrl Pts',(3.83485746513989,1.,1.67803353064351));
#41196=CARTESIAN_POINT('Ctrl Pts',(3.84113085985244,-1.,1.67774874946079));
#41197=CARTESIAN_POINT('Ctrl Pts',(3.84113085985244,1.,1.67774874946079));
#41198=CARTESIAN_POINT('Ctrl Pts',(3.84583912296459,-1.,1.6775199114018));
#41199=CARTESIAN_POINT('Ctrl Pts',(3.84583912296459,1.,1.6775199114018));
#41200=CARTESIAN_POINT('Ctrl Pts',(3.84897939430696,-1.,1.67736057656533));
#41201=CARTESIAN_POINT('Ctrl Pts',(3.84897939430696,1.,1.67736057656533));
#41202=CARTESIAN_POINT('Ctrl Pts',(3.85054988729471,-1.,1.67727921511438));
#41203=CARTESIAN_POINT('Ctrl Pts',(3.85054988729471,1.,1.67727921511438));
#41204=CARTESIAN_POINT('',(3.38171594275765,1.,1.62064718014094));
#41205=CARTESIAN_POINT('Ctrl Pts',(3.38171594275765,-1.,1.62064718014094));
#41206=CARTESIAN_POINT('Ctrl Pts',(3.38171594275765,-0.666666666666667,
1.62064718014094));
#41207=CARTESIAN_POINT('Ctrl Pts',(3.38171594275765,-0.333333333333333,
1.62064718014094));
#41208=CARTESIAN_POINT('Ctrl Pts',(3.38171594275765,0.333333333333333,1.62064718014094));
#41209=CARTESIAN_POINT('Ctrl Pts',(3.38171594275765,0.666666666666667,1.62064718014093));
#41210=CARTESIAN_POINT('Ctrl Pts',(3.38171594275765,1.,1.62064718014093));
#41211=CARTESIAN_POINT('',(3.85054988729471,1.,1.67727921511438));
#41212=CARTESIAN_POINT('',(3.85054988729471,0.,1.67727921511438));
#41213=CARTESIAN_POINT('Ctrl Pts',(3.38171594275765,1.,1.62064718014094));
#41214=CARTESIAN_POINT('Ctrl Pts',(3.38173802621259,1.,1.62069086551492));
#41215=CARTESIAN_POINT('Ctrl Pts',(3.38187506456922,1.,1.62083271135947));
#41216=CARTESIAN_POINT('Ctrl Pts',(3.38243080602408,1.,1.62118047294498));
#41217=CARTESIAN_POINT('Ctrl Pts',(3.38394285763222,1.,1.62192472202769));
#41218=CARTESIAN_POINT('Ctrl Pts',(3.38715832179072,1.,1.6233278855625));
#41219=CARTESIAN_POINT('Ctrl Pts',(3.39206617496906,1.,1.62533996116713));
#41220=CARTESIAN_POINT('Ctrl Pts',(3.39818605297991,1.,1.62774916464408));
#41221=CARTESIAN_POINT('Ctrl Pts',(3.40519422740235,1.,1.63041148964828));
#41222=CARTESIAN_POINT('Ctrl Pts',(3.41272817148478,1.,1.63316667054044));
#41223=CARTESIAN_POINT('Ctrl Pts',(3.42043974590882,1.,1.63586250099773));
#41224=CARTESIAN_POINT('Ctrl Pts',(3.42804772926291,1.,1.63837876246926));
#41225=CARTESIAN_POINT('Ctrl Pts',(3.43540451921548,1.,1.64065778702023));
#41226=CARTESIAN_POINT('Ctrl Pts',(3.44250337701888,1.,1.64270733821113));
#41227=CARTESIAN_POINT('Ctrl Pts',(3.44942242546795,1.,1.64457408708107));
#41228=CARTESIAN_POINT('Ctrl Pts',(3.45628421062422,1.,1.64632429697521));
#41229=CARTESIAN_POINT('Ctrl Pts',(3.46321237515,1.,1.64802323352738));
#41230=CARTESIAN_POINT('Ctrl Pts',(3.47028140995992,1.,1.64971118698256));
#41231=CARTESIAN_POINT('Ctrl Pts',(3.47749926256476,1.,1.65139534930322));
#41232=CARTESIAN_POINT('Ctrl Pts',(3.48483492840894,1.,1.65306335367739));
#41233=CARTESIAN_POINT('Ctrl Pts',(3.49223525300176,1.,1.65469162644468));
#41234=CARTESIAN_POINT('Ctrl Pts',(3.4996447647794,1.,1.65625517961588));
#41235=CARTESIAN_POINT('Ctrl Pts',(3.50702733146542,1.,1.65773832633632));
#41236=CARTESIAN_POINT('Ctrl Pts',(3.5143763218894,1.,1.65913971687342));
#41237=CARTESIAN_POINT('Ctrl Pts',(3.52170261543815,1.,1.66046645222279));
#41238=CARTESIAN_POINT('Ctrl Pts',(3.52902746211093,1.,1.66173058912371));
#41239=CARTESIAN_POINT('Ctrl Pts',(3.5363738506022,1.,1.66294490916111));
#41240=CARTESIAN_POINT('Ctrl Pts',(3.54375747475014,1.,1.66411849222326));
#41241=CARTESIAN_POINT('Ctrl Pts',(3.55118121342861,1.,1.66525401568994));
#41242=CARTESIAN_POINT('Ctrl Pts',(3.55864015233602,1.,1.66635023293114));
#41243=CARTESIAN_POINT('Ctrl Pts',(3.56612465179422,1.,1.66740349220305));
#41244=CARTESIAN_POINT('Ctrl Pts',(3.57362406285887,1.,1.668409574073));
#41245=CARTESIAN_POINT('Ctrl Pts',(3.58113044183829,1.,1.66936552908232));
#41246=CARTESIAN_POINT('Ctrl Pts',(3.58864143097834,1.,1.67027110397604));
#41247=CARTESIAN_POINT('Ctrl Pts',(3.59615824388807,1.,1.67112775290707));
#41248=CARTESIAN_POINT('Ctrl Pts',(3.603684308152,1.,1.67193797318597));
#41249=CARTESIAN_POINT('Ctrl Pts',(3.61122367156181,1.,1.67270452466968));
#41250=CARTESIAN_POINT('Ctrl Pts',(3.61877947398184,1.,1.67342968196224));
#41251=CARTESIAN_POINT('Ctrl Pts',(3.62635249450923,1.,1.67411452372271));
#41252=CARTESIAN_POINT('Ctrl Pts',(3.63394189312924,1.,1.67475929882971));
#41253=CARTESIAN_POINT('Ctrl Pts',(3.6415458297234,1.,1.67536373264848));
#41254=CARTESIAN_POINT('Ctrl Pts',(3.64916213574667,1.,1.67592735946692));
#41255=CARTESIAN_POINT('Ctrl Pts',(3.6567889441642,1.,1.6764498346945));
#41256=CARTESIAN_POINT('Ctrl Pts',(3.66442538670968,1.,1.67693128053132));
#41257=CARTESIAN_POINT('Ctrl Pts',(3.67207136294575,1.,1.67737217414874));
#41258=CARTESIAN_POINT('Ctrl Pts',(3.67972724579124,1.,1.67777320475848));
#41259=CARTESIAN_POINT('Ctrl Pts',(3.68739360236487,1.,1.67813513867965));
#41260=CARTESIAN_POINT('Ctrl Pts',(3.6950709275959,1.,1.67845869064323));
#41261=CARTESIAN_POINT('Ctrl Pts',(3.70275932351108,1.,1.67874436948667));
#41262=CARTESIAN_POINT('Ctrl Pts',(3.71045854208343,1.,1.67899249793462));
#41263=CARTESIAN_POINT('Ctrl Pts',(3.71816812842322,1.,1.67920328071708));
#41264=CARTESIAN_POINT('Ctrl Pts',(3.72588753416396,1.,1.67937685856652));
#41265=CARTESIAN_POINT('Ctrl Pts',(3.73361623282543,1.,1.67951336376402));
#41266=CARTESIAN_POINT('Ctrl Pts',(3.74135385965401,1.,1.6796129868522));
#41267=CARTESIAN_POINT('Ctrl Pts',(3.7491002239452,1.,1.67967598599525));
#41268=CARTESIAN_POINT('Ctrl Pts',(3.75685523754493,1.,1.67970265841239));
#41269=CARTESIAN_POINT('Ctrl Pts',(3.76461886684344,1.,1.67969332319245));
#41270=CARTESIAN_POINT('Ctrl Pts',(3.77239107928502,1.,1.67964830084993));
#41271=CARTESIAN_POINT('Ctrl Pts',(3.78017178197317,1.,1.67956789212141));
#41272=CARTESIAN_POINT('Ctrl Pts',(3.7879608002176,1.,1.67945236653493));
#41273=CARTESIAN_POINT('Ctrl Pts',(3.79575791578424,1.,1.67930196625548));
#41274=CARTESIAN_POINT('Ctrl Pts',(3.80356289079005,1.,1.67911690648355));
#41275=CARTESIAN_POINT('Ctrl Pts',(3.81137549624178,1.,1.6788973773827));
#41276=CARTESIAN_POINT('Ctrl Pts',(3.81919554099578,1.,1.67864354605954));
#41277=CARTESIAN_POINT('Ctrl Pts',(3.82702289286713,1.,1.6783555575934));
#41278=CARTESIAN_POINT('Ctrl Pts',(3.83485746513989,1.,1.67803353064351));
#41279=CARTESIAN_POINT('Ctrl Pts',(3.84113085985244,1.,1.67774874946079));
#41280=CARTESIAN_POINT('Ctrl Pts',(3.84583912296459,1.,1.6775199114018));
#41281=CARTESIAN_POINT('Ctrl Pts',(3.84897939430696,1.,1.67736057656533));
#41282=CARTESIAN_POINT('Ctrl Pts',(3.85054988729471,1.,1.67727921511438));
#41283=CARTESIAN_POINT('Origin',(3.85054988729471,0.,1.67727921511438));
#41284=CARTESIAN_POINT('',(3.90876544355381,1.,1.53673442965256));
#41285=CARTESIAN_POINT('Origin',(0.,0.,0.));
#41286=CARTESIAN_POINT('',(3.29885386921599,1.,1.78327315618183));
#41287=CARTESIAN_POINT('Origin',(0.,1.,0.));
#41288=CARTESIAN_POINT('Ctrl Pts',(3.29885386921599,1.,1.78327315618183));
#41289=CARTESIAN_POINT('Ctrl Pts',(3.29885386921599,0.666666666666667,1.78327315618183));
#41290=CARTESIAN_POINT('Ctrl Pts',(3.29885386921599,0.333333333333333,1.78327315618183));
#41291=CARTESIAN_POINT('Ctrl Pts',(3.29885386921599,-0.333333333333333,
1.78327315618183));
#41292=CARTESIAN_POINT('Ctrl Pts',(3.29885386921599,-0.666666666666667,
1.78327315618183));
#41293=CARTESIAN_POINT('Ctrl Pts',(3.29885386921599,-1.,1.78327315618183));
#41294=CARTESIAN_POINT('Ctrl Pts',(3.62024382630768,-1.,2.12928030988903));
#41295=CARTESIAN_POINT('Ctrl Pts',(3.62024382630768,1.,2.12928030988903));
#41296=CARTESIAN_POINT('Ctrl Pts',(3.61938653649098,-1.,2.12796193131368));
#41297=CARTESIAN_POINT('Ctrl Pts',(3.61938653649098,1.,2.12796193131368));
#41298=CARTESIAN_POINT('Ctrl Pts',(3.61766963590482,-1.,2.12532774376758));
#41299=CARTESIAN_POINT('Ctrl Pts',(3.61766963590482,1.,2.12532774376758));
#41300=CARTESIAN_POINT('Ctrl Pts',(3.61508732216891,-1.,2.12138417126355));
#41301=CARTESIAN_POINT('Ctrl Pts',(3.61508732216891,1.,2.12138417126355));
#41302=CARTESIAN_POINT('Ctrl Pts',(3.61163030609447,-1.,2.11614149815106));
#41303=CARTESIAN_POINT('Ctrl Pts',(3.61163030609447,1.,2.11614149815106));
#41304=CARTESIAN_POINT('Ctrl Pts',(3.60728578532601,-1.,2.10961391334462));
#41305=CARTESIAN_POINT('Ctrl Pts',(3.60728578532601,1.,2.10961391334462));
#41306=CARTESIAN_POINT('Ctrl Pts',(3.60291797088734,-1.,2.1031121772821));
#41307=CARTESIAN_POINT('Ctrl Pts',(3.60291797088734,1.,2.1031121772821));
#41308=CARTESIAN_POINT('Ctrl Pts',(3.59852681775485,-1.,2.09663642986631));
#41309=CARTESIAN_POINT('Ctrl Pts',(3.59852681775485,1.,2.09663642986631));
#41310=CARTESIAN_POINT('Ctrl Pts',(3.59411228625588,-1.,2.09018686331416));
#41311=CARTESIAN_POINT('Ctrl Pts',(3.59411228625588,1.,2.09018686331416));
#41312=CARTESIAN_POINT('Ctrl Pts',(3.58967435355088,-1.,2.08376373048756));
#41313=CARTESIAN_POINT('Ctrl Pts',(3.58967435355088,1.,2.08376373048756));
#41314=CARTESIAN_POINT('Ctrl Pts',(3.58521300039299,-1.,2.07736732842117));
#41315=CARTESIAN_POINT('Ctrl Pts',(3.58521300039299,1.,2.07736732842117));
#41316=CARTESIAN_POINT('Ctrl Pts',(3.58072819250442,-1.,2.07099797605747));
#41317=CARTESIAN_POINT('Ctrl Pts',(3.58072819250442,1.,2.07099797605747));
#41318=CARTESIAN_POINT('Ctrl Pts',(3.576219862243,-1.,2.06465599229174));
#41319=CARTESIAN_POINT('Ctrl Pts',(3.576219862243,1.,2.06465599229174));
#41320=CARTESIAN_POINT('Ctrl Pts',(3.57168789423507,-1.,2.05834167687524));
#41321=CARTESIAN_POINT('Ctrl Pts',(3.57168789423507,1.,2.05834167687524));
#41322=CARTESIAN_POINT('Ctrl Pts',(3.56713209978207,-1.,2.05205528173091));
#41323=CARTESIAN_POINT('Ctrl Pts',(3.56713209978207,1.,2.05205528173091));
#41324=CARTESIAN_POINT('Ctrl Pts',(3.5625522387181,-1.,2.04579702159056));
#41325=CARTESIAN_POINT('Ctrl Pts',(3.5625522387181,1.,2.04579702159056));
#41326=CARTESIAN_POINT('Ctrl Pts',(3.55794807265052,-1.,2.03956711120099));
#41327=CARTESIAN_POINT('Ctrl Pts',(3.55794807265052,1.,2.03956711120099));
#41328=CARTESIAN_POINT('Ctrl Pts',(3.55331941294018,-1.,2.03336579658174));
#41329=CARTESIAN_POINT('Ctrl Pts',(3.55331941294018,1.,2.03336579658174));
#41330=CARTESIAN_POINT('Ctrl Pts',(3.54866616282173,-1.,2.02719338376144));
#41331=CARTESIAN_POINT('Ctrl Pts',(3.54866616282173,1.,2.02719338376144));
#41332=CARTESIAN_POINT('Ctrl Pts',(3.54398838254011,-1.,2.0210502798303));
#41333=CARTESIAN_POINT('Ctrl Pts',(3.54398838254011,1.,2.0210502798303));
#41334=CARTESIAN_POINT('Ctrl Pts',(3.53928627453503,-1.,2.0149369884727));
#41335=CARTESIAN_POINT('Ctrl Pts',(3.53928627453503,1.,2.0149369884727));
#41336=CARTESIAN_POINT('Ctrl Pts',(3.53456004727321,-1.,2.00885403604685));
#41337=CARTESIAN_POINT('Ctrl Pts',(3.53456004727321,1.,2.00885403604685));
#41338=CARTESIAN_POINT('Ctrl Pts',(3.52980980250181,-1.,2.00280191090341));
#41339=CARTESIAN_POINT('Ctrl Pts',(3.52980980250181,1.,2.00280191090341));
#41340=CARTESIAN_POINT('Ctrl Pts',(3.52503542491745,-1.,1.99678100339306));
#41341=CARTESIAN_POINT('Ctrl Pts',(3.52503542491745,1.,1.99678100339306));
#41342=CARTESIAN_POINT('Ctrl Pts',(3.52023644289195,-1.,1.99079153006143));
#41343=CARTESIAN_POINT('Ctrl Pts',(3.52023644289195,1.,1.99079153006143));
#41344=CARTESIAN_POINT('Ctrl Pts',(3.51541198728362,-1.,1.98483351061066));
#41345=CARTESIAN_POINT('Ctrl Pts',(3.51541198728362,1.,1.98483351061066));
#41346=CARTESIAN_POINT('Ctrl Pts',(3.51056110478334,-1.,1.97890693666316));
#41347=CARTESIAN_POINT('Ctrl Pts',(3.51056110478334,1.,1.97890693666316));
#41348=CARTESIAN_POINT('Ctrl Pts',(3.505683018611,-1.,1.9730119116298));
#41349=CARTESIAN_POINT('Ctrl Pts',(3.505683018611,1.,1.9730119116298));
#41350=CARTESIAN_POINT('Ctrl Pts',(3.50077740176262,-1.,1.9671487972405));
#41351=CARTESIAN_POINT('Ctrl Pts',(3.50077740176262,1.,1.9671487972405));
#41352=CARTESIAN_POINT('Ctrl Pts',(3.49584466573045,-1.,1.96131836776489));
#41353=CARTESIAN_POINT('Ctrl Pts',(3.49584466573045,1.,1.96131836776489));
#41354=CARTESIAN_POINT('Ctrl Pts',(3.49088618670967,-1.,1.95552193112071));
#41355=CARTESIAN_POINT('Ctrl Pts',(3.49088618670967,1.,1.95552193112071));
#41356=CARTESIAN_POINT('Ctrl Pts',(3.485903616108,-1.,1.94976096795902));
#41357=CARTESIAN_POINT('Ctrl Pts',(3.485903616108,1.,1.94976096795902));
#41358=CARTESIAN_POINT('Ctrl Pts',(3.48089825770411,-1.,1.94403680554062));
#41359=CARTESIAN_POINT('Ctrl Pts',(3.48089825770411,1.,1.94403680554062));
#41360=CARTESIAN_POINT('Ctrl Pts',(3.47587040389916,-1.,1.93835026973888));
#41361=CARTESIAN_POINT('Ctrl Pts',(3.47587040389916,1.,1.93835026973888));
#41362=CARTESIAN_POINT('Ctrl Pts',(3.47081872409783,-1.,1.93270136427083));
#41363=CARTESIAN_POINT('Ctrl Pts',(3.47081872409783,1.,1.93270136427083));
#41364=CARTESIAN_POINT('Ctrl Pts',(3.46573953254084,-1.,1.92708888591159));
#41365=CARTESIAN_POINT('Ctrl Pts',(3.46573953254084,1.,1.92708888591159));
#41366=CARTESIAN_POINT('Ctrl Pts',(3.4606282172248,-1.,1.9215111821321));
#41367=CARTESIAN_POINT('Ctrl Pts',(3.4606282172248,1.,1.9215111821321));
#41368=CARTESIAN_POINT('Ctrl Pts',(3.45548074309943,-1.,1.9159669478406));
#41369=CARTESIAN_POINT('Ctrl Pts',(3.45548074309943,1.,1.9159669478406));
#41370=CARTESIAN_POINT('Ctrl Pts',(3.45029522038885,-1.,1.91045605593638));
#41371=CARTESIAN_POINT('Ctrl Pts',(3.45029522038885,1.,1.91045605593638));
#41372=CARTESIAN_POINT('Ctrl Pts',(3.44507323983374,-1.,1.90498026502308));
#41373=CARTESIAN_POINT('Ctrl Pts',(3.44507323983374,1.,1.90498026502308));
#41374=CARTESIAN_POINT('Ctrl Pts',(3.43982185678105,-1.,1.89954426803392));
#41375=CARTESIAN_POINT('Ctrl Pts',(3.43982185678105,1.,1.89954426803392));
#41376=CARTESIAN_POINT('Ctrl Pts',(3.43455074411591,-1.,1.89415420002553));
#41377=CARTESIAN_POINT('Ctrl Pts',(3.43455074411591,1.,1.89415420002553));
#41378=CARTESIAN_POINT('Ctrl Pts',(3.42926852222174,-1.,1.88881571322018));
#41379=CARTESIAN_POINT('Ctrl Pts',(3.42926852222174,1.,1.88881571322018));
#41380=CARTESIAN_POINT('Ctrl Pts',(3.42397908819741,-1.,1.88353205062063));
#41381=CARTESIAN_POINT('Ctrl Pts',(3.42397908819741,1.,1.88353205062063));
#41382=CARTESIAN_POINT('Ctrl Pts',(3.4186785838376,-1.,1.87830245689338));
#41383=CARTESIAN_POINT('Ctrl Pts',(3.4186785838376,1.,1.87830245689338));
#41384=CARTESIAN_POINT('Ctrl Pts',(3.41335043875182,-1.,1.87311957248106));
#41385=CARTESIAN_POINT('Ctrl Pts',(3.41335043875182,1.,1.87311957248106));
#41386=CARTESIAN_POINT('Ctrl Pts',(3.40797080000513,-1.,1.86797231196635));
#41387=CARTESIAN_POINT('Ctrl Pts',(3.40797080000513,1.,1.86797231196635));
#41388=CARTESIAN_POINT('Ctrl Pts',(3.40251742305445,-1.,1.86285057051228));
#41389=CARTESIAN_POINT('Ctrl Pts',(3.40251742305445,1.,1.86285057051228));
#41390=CARTESIAN_POINT('Ctrl Pts',(3.39697816833056,-1.,1.85774972037055));
#41391=CARTESIAN_POINT('Ctrl Pts',(3.39697816833056,1.,1.85774972037055));
#41392=CARTESIAN_POINT('Ctrl Pts',(3.39135802549415,-1.,1.85267433291778));
#41393=CARTESIAN_POINT('Ctrl Pts',(3.39135802549415,1.,1.85267433291778));
#41394=CARTESIAN_POINT('Ctrl Pts',(3.38569092349639,-1.,1.84764441927778));
#41395=CARTESIAN_POINT('Ctrl Pts',(3.38569092349639,1.,1.84764441927778));
#41396=CARTESIAN_POINT('Ctrl Pts',(3.38002968341222,-1.,1.84269016931679));
#41397=CARTESIAN_POINT('Ctrl Pts',(3.38002968341222,1.,1.84269016931679));
#41398=CARTESIAN_POINT('Ctrl Pts',(3.37442462015914,-1.,1.83784072967111));
#41399=CARTESIAN_POINT('Ctrl Pts',(3.37442462015914,1.,1.83784072967111));
#41400=CARTESIAN_POINT('Ctrl Pts',(3.36890396271864,-1.,1.83311391452338));
#41401=CARTESIAN_POINT('Ctrl Pts',(3.36890396271864,1.,1.83311391452338));
#41402=CARTESIAN_POINT('Ctrl Pts',(3.36345722124127,-1.,1.82850752153182));
#41403=CARTESIAN_POINT('Ctrl Pts',(3.36345722124127,1.,1.82850752153182));
#41404=CARTESIAN_POINT('Ctrl Pts',(3.35800801557326,-1.,1.82398496829247));
#41405=CARTESIAN_POINT('Ctrl Pts',(3.35800801557326,1.,1.82398496829247));
#41406=CARTESIAN_POINT('Ctrl Pts',(3.35243086937451,-1.,1.81948458796748));
#41407=CARTESIAN_POINT('Ctrl Pts',(3.35243086937451,1.,1.81948458796748));
#41408=CARTESIAN_POINT('Ctrl Pts',(3.34660014370527,-1.,1.81494618732772));
#41409=CARTESIAN_POINT('Ctrl Pts',(3.34660014370527,1.,1.81494618732772));
#41410=CARTESIAN_POINT('Ctrl Pts',(3.34043216147532,-1.,1.81033399625311));
#41411=CARTESIAN_POINT('Ctrl Pts',(3.34043216147532,1.,1.81033399625311));
#41412=CARTESIAN_POINT('Ctrl Pts',(3.33392460276874,-1.,1.80565802981139));
#41413=CARTESIAN_POINT('Ctrl Pts',(3.33392460276874,1.,1.80565802981139));
#41414=CARTESIAN_POINT('Ctrl Pts',(3.3272108803981,-1.,1.80100380443535));
#41415=CARTESIAN_POINT('Ctrl Pts',(3.3272108803981,1.,1.80100380443535));
#41416=CARTESIAN_POINT('Ctrl Pts',(3.32055355101168,-1.,1.79652817033444));
#41417=CARTESIAN_POINT('Ctrl Pts',(3.32055355101168,1.,1.79652817033444));
#41418=CARTESIAN_POINT('Ctrl Pts',(3.31428038326763,-1.,1.79242331350137));
#41419=CARTESIAN_POINT('Ctrl Pts',(3.31428038326763,1.,1.79242331350137));
#41420=CARTESIAN_POINT('Ctrl Pts',(3.30873412266954,-1.,1.78888832245965));
#41421=CARTESIAN_POINT('Ctrl Pts',(3.30873412266954,1.,1.78888832245965));
#41422=CARTESIAN_POINT('Ctrl Pts',(3.30422155558973,-1.,1.78610045419769));
#41423=CARTESIAN_POINT('Ctrl Pts',(3.30422155558973,1.,1.78610045419769));
#41424=CARTESIAN_POINT('Ctrl Pts',(3.30095096463082,-1.,1.78417972819697));
#41425=CARTESIAN_POINT('Ctrl Pts',(3.30095096463082,1.,1.78417972819697));
#41426=CARTESIAN_POINT('Ctrl Pts',(3.29940631673818,-1.,1.78338186555671));
#41427=CARTESIAN_POINT('Ctrl Pts',(3.29940631673818,1.,1.78338186555671));
#41428=CARTESIAN_POINT('Ctrl Pts',(3.29886572077303,-1.,1.78320756177191));
#41429=CARTESIAN_POINT('Ctrl Pts',(3.29886572077303,1.,1.78320756177191));
#41430=CARTESIAN_POINT('Ctrl Pts',(3.29877974053191,-1.,1.78327971836273));
#41431=CARTESIAN_POINT('Ctrl Pts',(3.29877974053191,1.,1.78327971836273));
#41432=CARTESIAN_POINT('Ctrl Pts',(3.2988053601491,-1.,1.7833628895577));
#41433=CARTESIAN_POINT('Ctrl Pts',(3.2988053601491,1.,1.7833628895577));
#41434=CARTESIAN_POINT('',(3.62024382630768,1.,2.12928030988903));
#41435=CARTESIAN_POINT('Ctrl Pts',(3.62024382630768,1.,2.12928030988903));
#41436=CARTESIAN_POINT('Ctrl Pts',(3.61938653649098,1.,2.12796193131368));
#41437=CARTESIAN_POINT('Ctrl Pts',(3.61766963590482,1.,2.12532774376758));
#41438=CARTESIAN_POINT('Ctrl Pts',(3.61508732216891,1.,2.12138417126355));
#41439=CARTESIAN_POINT('Ctrl Pts',(3.61163030609447,1.,2.11614149815106));
#41440=CARTESIAN_POINT('Ctrl Pts',(3.60728578532601,1.,2.10961391334462));
#41441=CARTESIAN_POINT('Ctrl Pts',(3.60291797088734,1.,2.1031121772821));
#41442=CARTESIAN_POINT('Ctrl Pts',(3.59852681775485,1.,2.09663642986631));
#41443=CARTESIAN_POINT('Ctrl Pts',(3.59411228625588,1.,2.09018686331416));
#41444=CARTESIAN_POINT('Ctrl Pts',(3.58967435355088,1.,2.08376373048756));
#41445=CARTESIAN_POINT('Ctrl Pts',(3.58521300039299,1.,2.07736732842117));
#41446=CARTESIAN_POINT('Ctrl Pts',(3.58072819250442,1.,2.07099797605747));
#41447=CARTESIAN_POINT('Ctrl Pts',(3.576219862243,1.,2.06465599229174));
#41448=CARTESIAN_POINT('Ctrl Pts',(3.57168789423507,1.,2.05834167687524));
#41449=CARTESIAN_POINT('Ctrl Pts',(3.56713209978207,1.,2.05205528173091));
#41450=CARTESIAN_POINT('Ctrl Pts',(3.5625522387181,1.,2.04579702159056));
#41451=CARTESIAN_POINT('Ctrl Pts',(3.55794807265052,1.,2.03956711120099));
#41452=CARTESIAN_POINT('Ctrl Pts',(3.55331941294018,1.,2.03336579658174));
#41453=CARTESIAN_POINT('Ctrl Pts',(3.54866616282173,1.,2.02719338376144));
#41454=CARTESIAN_POINT('Ctrl Pts',(3.54398838254011,1.,2.0210502798303));
#41455=CARTESIAN_POINT('Ctrl Pts',(3.53928627453503,1.,2.0149369884727));
#41456=CARTESIAN_POINT('Ctrl Pts',(3.53456004727321,1.,2.00885403604685));
#41457=CARTESIAN_POINT('Ctrl Pts',(3.52980980250181,1.,2.00280191090341));
#41458=CARTESIAN_POINT('Ctrl Pts',(3.52503542491745,1.,1.99678100339306));
#41459=CARTESIAN_POINT('Ctrl Pts',(3.52023644289195,1.,1.99079153006143));
#41460=CARTESIAN_POINT('Ctrl Pts',(3.51541198728362,1.,1.98483351061066));
#41461=CARTESIAN_POINT('Ctrl Pts',(3.51056110478334,1.,1.97890693666316));
#41462=CARTESIAN_POINT('Ctrl Pts',(3.505683018611,1.,1.9730119116298));
#41463=CARTESIAN_POINT('Ctrl Pts',(3.50077740176262,1.,1.9671487972405));
#41464=CARTESIAN_POINT('Ctrl Pts',(3.49584466573045,1.,1.96131836776489));
#41465=CARTESIAN_POINT('Ctrl Pts',(3.49088618670967,1.,1.95552193112071));
#41466=CARTESIAN_POINT('Ctrl Pts',(3.485903616108,1.,1.94976096795902));
#41467=CARTESIAN_POINT('Ctrl Pts',(3.48089825770411,1.,1.94403680554062));
#41468=CARTESIAN_POINT('Ctrl Pts',(3.47587040389916,1.,1.93835026973888));
#41469=CARTESIAN_POINT('Ctrl Pts',(3.47081872409783,1.,1.93270136427083));
#41470=CARTESIAN_POINT('Ctrl Pts',(3.46573953254084,1.,1.92708888591159));
#41471=CARTESIAN_POINT('Ctrl Pts',(3.4606282172248,1.,1.9215111821321));
#41472=CARTESIAN_POINT('Ctrl Pts',(3.45548074309943,1.,1.9159669478406));
#41473=CARTESIAN_POINT('Ctrl Pts',(3.45029522038885,1.,1.91045605593638));
#41474=CARTESIAN_POINT('Ctrl Pts',(3.44507323983374,1.,1.90498026502308));
#41475=CARTESIAN_POINT('Ctrl Pts',(3.43982185678105,1.,1.89954426803392));
#41476=CARTESIAN_POINT('Ctrl Pts',(3.43455074411591,1.,1.89415420002553));
#41477=CARTESIAN_POINT('Ctrl Pts',(3.42926852222174,1.,1.88881571322018));
#41478=CARTESIAN_POINT('Ctrl Pts',(3.42397908819741,1.,1.88353205062063));
#41479=CARTESIAN_POINT('Ctrl Pts',(3.4186785838376,1.,1.87830245689338));
#41480=CARTESIAN_POINT('Ctrl Pts',(3.41335043875182,1.,1.87311957248106));
#41481=CARTESIAN_POINT('Ctrl Pts',(3.40797080000513,1.,1.86797231196635));
#41482=CARTESIAN_POINT('Ctrl Pts',(3.40251742305445,1.,1.86285057051228));
#41483=CARTESIAN_POINT('Ctrl Pts',(3.39697816833056,1.,1.85774972037055));
#41484=CARTESIAN_POINT('Ctrl Pts',(3.39135802549415,1.,1.85267433291778));
#41485=CARTESIAN_POINT('Ctrl Pts',(3.38569092349639,1.,1.84764441927778));
#41486=CARTESIAN_POINT('Ctrl Pts',(3.38002968341222,1.,1.84269016931679));
#41487=CARTESIAN_POINT('Ctrl Pts',(3.37442462015914,1.,1.83784072967111));
#41488=CARTESIAN_POINT('Ctrl Pts',(3.36890396271864,1.,1.83311391452338));
#41489=CARTESIAN_POINT('Ctrl Pts',(3.36345722124127,1.,1.82850752153182));
#41490=CARTESIAN_POINT('Ctrl Pts',(3.35800801557326,1.,1.82398496829247));
#41491=CARTESIAN_POINT('Ctrl Pts',(3.35243086937451,1.,1.81948458796748));
#41492=CARTESIAN_POINT('Ctrl Pts',(3.34660014370527,1.,1.81494618732772));
#41493=CARTESIAN_POINT('Ctrl Pts',(3.34043216147532,1.,1.81033399625311));
#41494=CARTESIAN_POINT('Ctrl Pts',(3.33392460276874,1.,1.80565802981139));
#41495=CARTESIAN_POINT('Ctrl Pts',(3.3272108803981,1.,1.80100380443535));
#41496=CARTESIAN_POINT('Ctrl Pts',(3.32055355101168,1.,1.79652817033444));
#41497=CARTESIAN_POINT('Ctrl Pts',(3.31428038326763,1.,1.79242331350137));
#41498=CARTESIAN_POINT('Ctrl Pts',(3.30873412266954,1.,1.78888832245965));
#41499=CARTESIAN_POINT('Ctrl Pts',(3.30422155558973,1.,1.78610045419769));
#41500=CARTESIAN_POINT('Ctrl Pts',(3.30119637003466,1.,1.78432384788231));
#41501=CARTESIAN_POINT('Ctrl Pts',(3.29970549824337,1.,1.78353803106983));
#41502=CARTESIAN_POINT('Ctrl Pts',(3.29909749657945,1.,1.78329283591903));
#41503=CARTESIAN_POINT('Ctrl Pts',(3.29890219175522,1.,1.78326534445426));
#41504=CARTESIAN_POINT('Ctrl Pts',(3.29885386921599,1.,1.78327315618183));
#41505=CARTESIAN_POINT('',(3.62024382630768,0.,2.12928030988903));
#41506=CARTESIAN_POINT('Ctrl Pts',(3.08661426358891,-1.,2.12962728847315));
#41507=CARTESIAN_POINT('Ctrl Pts',(3.08661426358891,1.,2.12962728847315));
#41508=CARTESIAN_POINT('Ctrl Pts',(3.08652852644995,-1.,2.12964222016025));
#41509=CARTESIAN_POINT('Ctrl Pts',(3.08652852644995,1.,2.12964222016025));
#41510=CARTESIAN_POINT('Ctrl Pts',(3.08650326867133,-1.,2.12975158752407));
#41511=CARTESIAN_POINT('Ctrl Pts',(3.08650326867133,1.,2.12975158752407));
#41512=CARTESIAN_POINT('Ctrl Pts',(3.08690399991463,-1.,2.1301541297946));
#41513=CARTESIAN_POINT('Ctrl Pts',(3.08690399991463,1.,2.1301541297946));
#41514=CARTESIAN_POINT('Ctrl Pts',(3.08831615620074,-1.,2.13116819908542));
#41515=CARTESIAN_POINT('Ctrl Pts',(3.08831615620074,1.,2.13116819908542));
#41516=CARTESIAN_POINT('Ctrl Pts',(3.09151235281963,-1.,2.13321032560894));
#41517=CARTESIAN_POINT('Ctrl Pts',(3.09151235281963,1.,2.13321032560894));
#41518=CARTESIAN_POINT('Ctrl Pts',(3.0960450242104,-1.,2.13596538661048));
#41519=CARTESIAN_POINT('Ctrl Pts',(3.0960450242104,1.,2.13596538661048));
#41520=CARTESIAN_POINT('Ctrl Pts',(3.10171267391049,-1.,2.13930228863751));
#41521=CARTESIAN_POINT('Ctrl Pts',(3.10171267391049,1.,2.13930228863751));
#41522=CARTESIAN_POINT('Ctrl Pts',(3.10821808668859,-1.,2.14302815601973));
#41523=CARTESIAN_POINT('Ctrl Pts',(3.10821808668859,1.,2.14302815601973));
#41524=CARTESIAN_POINT('Ctrl Pts',(3.11522827016855,-1.,2.14692798457532));
#41525=CARTESIAN_POINT('Ctrl Pts',(3.11522827016855,1.,2.14692798457532));
#41526=CARTESIAN_POINT('Ctrl Pts',(3.12242318151938,-1.,2.15079698090585));
#41527=CARTESIAN_POINT('Ctrl Pts',(3.12242318151938,1.,2.15079698090585));
#41528=CARTESIAN_POINT('Ctrl Pts',(3.12954386795646,-1.,2.1544724138292));
#41529=CARTESIAN_POINT('Ctrl Pts',(3.12954386795646,1.,2.1544724138292));
#41530=CARTESIAN_POINT('Ctrl Pts',(3.13645356563038,-1.,2.15787423530676));
#41531=CARTESIAN_POINT('Ctrl Pts',(3.13645356563038,1.,2.15787423530676));
#41532=CARTESIAN_POINT('Ctrl Pts',(3.14314440427022,-1.,2.16100905914435));
#41533=CARTESIAN_POINT('Ctrl Pts',(3.14314440427022,1.,2.16100905914435));
#41534=CARTESIAN_POINT('Ctrl Pts',(3.14968624389054,-1.,2.16393520288072));
#41535=CARTESIAN_POINT('Ctrl Pts',(3.14968624389054,1.,2.16393520288072));
#41536=CARTESIAN_POINT('Ctrl Pts',(3.15618975593656,-1.,2.1667372844769));
#41537=CARTESIAN_POINT('Ctrl Pts',(3.15618975593656,1.,2.1667372844769));
#41538=CARTESIAN_POINT('Ctrl Pts',(3.16276685102972,-1.,2.16949910801219));
#41539=CARTESIAN_POINT('Ctrl Pts',(3.16276685102972,1.,2.16949910801219));
#41540=CARTESIAN_POINT('Ctrl Pts',(3.16948480019497,-1.,2.17227212063817));
#41541=CARTESIAN_POINT('Ctrl Pts',(3.16948480019497,1.,2.17227212063817));
#41542=CARTESIAN_POINT('Ctrl Pts',(3.17635032802523,-1.,2.17506466903694));
#41543=CARTESIAN_POINT('Ctrl Pts',(3.17635032802523,1.,2.17506466903694));
#41544=CARTESIAN_POINT('Ctrl Pts',(3.18333474627807,-1.,2.17785968847142));
#41545=CARTESIAN_POINT('Ctrl Pts',(3.18333474627807,1.,2.17785968847142));
#41546=CARTESIAN_POINT('Ctrl Pts',(3.19038924261573,-1.,2.18062558031778));
#41547=CARTESIAN_POINT('Ctrl Pts',(3.19038924261573,1.,2.18062558031778));
#41548=CARTESIAN_POINT('Ctrl Pts',(3.19746293740411,-1.,2.18332898656602));
#41549=CARTESIAN_POINT('Ctrl Pts',(3.19746293740411,1.,2.18332898656602));
#41550=CARTESIAN_POINT('Ctrl Pts',(3.20452259717976,-1.,2.18594876115934));
#41551=CARTESIAN_POINT('Ctrl Pts',(3.20452259717976,1.,2.18594876115934));
#41552=CARTESIAN_POINT('Ctrl Pts',(3.21156188355769,-1.,2.18848253363901));
#41553=CARTESIAN_POINT('Ctrl Pts',(3.21156188355769,1.,2.18848253363901));
#41554=CARTESIAN_POINT('Ctrl Pts',(3.21859043114095,-1.,2.19093901948667));
#41555=CARTESIAN_POINT('Ctrl Pts',(3.21859043114095,1.,2.19093901948667));
#41556=CARTESIAN_POINT('Ctrl Pts',(3.22562734221646,-1.,2.19333345123538));
#41557=CARTESIAN_POINT('Ctrl Pts',(3.22562734221646,1.,2.19333345123538));
#41558=CARTESIAN_POINT('Ctrl Pts',(3.23269332296933,-1.,2.19568204933168));
#41559=CARTESIAN_POINT('Ctrl Pts',(3.23269332296933,1.,2.19568204933168));
#41560=CARTESIAN_POINT('Ctrl Pts',(3.23980245361308,-1.,2.19799623693253));
#41561=CARTESIAN_POINT('Ctrl Pts',(3.23980245361308,1.,2.19799623693253));
#41562=CARTESIAN_POINT('Ctrl Pts',(3.24695715874338,-1.,2.20027910880981));
#41563=CARTESIAN_POINT('Ctrl Pts',(3.24695715874338,1.,2.20027910880981));
#41564=CARTESIAN_POINT('Ctrl Pts',(3.25415277957775,-1.,2.20252866491545));
#41565=CARTESIAN_POINT('Ctrl Pts',(3.25415277957775,1.,2.20252866491545));
#41566=CARTESIAN_POINT('Ctrl Pts',(3.26138036637705,-1.,2.20473979048678));
#41567=CARTESIAN_POINT('Ctrl Pts',(3.26138036637705,1.,2.20473979048678));
#41568=CARTESIAN_POINT('Ctrl Pts',(3.26863006136782,-1.,2.20690665217743));
#41569=CARTESIAN_POINT('Ctrl Pts',(3.26863006136782,1.,2.20690665217743));
#41570=CARTESIAN_POINT('Ctrl Pts',(3.2758944800554,-1.,2.2090250941743));
#41571=CARTESIAN_POINT('Ctrl Pts',(3.2758944800554,1.,2.2090250941743));
#41572=CARTESIAN_POINT('Ctrl Pts',(3.28317133333131,-1.,2.21109449750641));
#41573=CARTESIAN_POINT('Ctrl Pts',(3.28317133333131,1.,2.21109449750641));
#41574=CARTESIAN_POINT('Ctrl Pts',(3.29046159238343,-1.,2.21311648827391));
#41575=CARTESIAN_POINT('Ctrl Pts',(3.29046159238343,1.,2.21311648827391));
#41576=CARTESIAN_POINT('Ctrl Pts',(3.29776825193159,-1.,2.21509406923369));
#41577=CARTESIAN_POINT('Ctrl Pts',(3.29776825193159,1.,2.21509406923369));
#41578=CARTESIAN_POINT('Ctrl Pts',(3.30509487819569,-1.,2.21703059947836));
#41579=CARTESIAN_POINT('Ctrl Pts',(3.30509487819569,1.,2.21703059947836));
#41580=CARTESIAN_POINT('Ctrl Pts',(3.31244421655666,-1.,2.21892881679086));
#41581=CARTESIAN_POINT('Ctrl Pts',(3.31244421655666,1.,2.21892881679086));
#41582=CARTESIAN_POINT('Ctrl Pts',(3.31981686778022,-1.,2.22078990842776));
#41583=CARTESIAN_POINT('Ctrl Pts',(3.31981686778022,1.,2.22078990842776));
#41584=CARTESIAN_POINT('Ctrl Pts',(3.3272119632604,-1.,2.22261398879635));
#41585=CARTESIAN_POINT('Ctrl Pts',(3.3272119632604,1.,2.22261398879635));
#41586=CARTESIAN_POINT('Ctrl Pts',(3.33462772849598,-1.,2.22440049878511));
#41587=CARTESIAN_POINT('Ctrl Pts',(3.33462772849598,1.,2.22440049878511));
#41588=CARTESIAN_POINT('Ctrl Pts',(3.34206209449375,-1.,2.22614863918047));
#41589=CARTESIAN_POINT('Ctrl Pts',(3.34206209449375,1.,2.22614863918047));
#41590=CARTESIAN_POINT('Ctrl Pts',(3.34951327111096,-1.,2.22785777756576));
#41591=CARTESIAN_POINT('Ctrl Pts',(3.34951327111096,1.,2.22785777756576));
#41592=CARTESIAN_POINT('Ctrl Pts',(3.35698038165483,-1.,2.22952789880983));
#41593=CARTESIAN_POINT('Ctrl Pts',(3.35698038165483,1.,2.22952789880983));
#41594=CARTESIAN_POINT('Ctrl Pts',(3.36446325227848,-1.,2.23115945849739));
#41595=CARTESIAN_POINT('Ctrl Pts',(3.36446325227848,1.,2.23115945849739));
#41596=CARTESIAN_POINT('Ctrl Pts',(3.37196214349304,-1.,2.23275319569221));
#41597=CARTESIAN_POINT('Ctrl Pts',(3.37196214349304,1.,2.23275319569221));
#41598=CARTESIAN_POINT('Ctrl Pts',(3.37947749555632,-1.,2.23430995599561));
#41599=CARTESIAN_POINT('Ctrl Pts',(3.37947749555632,1.,2.23430995599561));
#41600=CARTESIAN_POINT('Ctrl Pts',(3.38700968549563,-1.,2.23583052276308));
#41601=CARTESIAN_POINT('Ctrl Pts',(3.38700968549563,1.,2.23583052276308));
#41602=CARTESIAN_POINT('Ctrl Pts',(3.39455873448189,-1.,2.23731541452791));
#41603=CARTESIAN_POINT('Ctrl Pts',(3.39455873448189,1.,2.23731541452791));
#41604=CARTESIAN_POINT('Ctrl Pts',(3.40212434705647,-1.,2.23876491124151));
#41605=CARTESIAN_POINT('Ctrl Pts',(3.40212434705647,1.,2.23876491124151));
#41606=CARTESIAN_POINT('Ctrl Pts',(3.40970604190328,-1.,2.24017914395289));
#41607=CARTESIAN_POINT('Ctrl Pts',(3.40970604190328,1.,2.24017914395289));
#41608=CARTESIAN_POINT('Ctrl Pts',(3.41730325539172,-1.,2.24155816587844));
#41609=CARTESIAN_POINT('Ctrl Pts',(3.41730325539172,1.,2.24155816587844));
#41610=CARTESIAN_POINT('Ctrl Pts',(3.42491544683008,-1.,2.24290202531101));
#41611=CARTESIAN_POINT('Ctrl Pts',(3.42491544683008,1.,2.24290202531101));
#41612=CARTESIAN_POINT('Ctrl Pts',(3.43254222614803,-1.,2.24421085338727));
#41613=CARTESIAN_POINT('Ctrl Pts',(3.43254222614803,1.,2.24421085338727));
#41614=CARTESIAN_POINT('Ctrl Pts',(3.4401833646032,-1.,2.24548487526022));
#41615=CARTESIAN_POINT('Ctrl Pts',(3.4401833646032,1.,2.24548487526022));
#41616=CARTESIAN_POINT('Ctrl Pts',(3.44783872863151,-1.,2.2467243706995));
#41617=CARTESIAN_POINT('Ctrl Pts',(3.44783872863151,1.,2.2467243706995));
#41618=CARTESIAN_POINT('Ctrl Pts',(3.45550823512049,-1.,2.2479296496077));
#41619=CARTESIAN_POINT('Ctrl Pts',(3.45550823512049,1.,2.2479296496077));
#41620=CARTESIAN_POINT('Ctrl Pts',(3.46319180177573,-1.,2.2491010234604));
#41621=CARTESIAN_POINT('Ctrl Pts',(3.46319180177573,1.,2.2491010234604));
#41622=CARTESIAN_POINT('Ctrl Pts',(3.47088928979888,-1.,2.25023877475942));
#41623=CARTESIAN_POINT('Ctrl Pts',(3.47088928979888,1.,2.25023877475942));
#41624=CARTESIAN_POINT('Ctrl Pts',(3.47860048448691,-1.,2.25134314238687));
#41625=CARTESIAN_POINT('Ctrl Pts',(3.47860048448691,1.,2.25134314238687));
#41626=CARTESIAN_POINT('Ctrl Pts',(3.48632513240961,-1.,2.25241433138695));
#41627=CARTESIAN_POINT('Ctrl Pts',(3.48632513240961,1.,2.25241433138695));
#41628=CARTESIAN_POINT('Ctrl Pts',(3.49406296494791,-1.,2.2534525170976));
#41629=CARTESIAN_POINT('Ctrl Pts',(3.49406296494791,1.,2.2534525170976));
#41630=CARTESIAN_POINT('Ctrl Pts',(3.50181372617971,-1.,2.25445785151868));
#41631=CARTESIAN_POINT('Ctrl Pts',(3.50181372617971,1.,2.25445785151868));
#41632=CARTESIAN_POINT('Ctrl Pts',(3.50957720117341,-1.,2.255430469798));
#41633=CARTESIAN_POINT('Ctrl Pts',(3.50957720117341,1.,2.255430469798));
#41634=CARTESIAN_POINT('Ctrl Pts',(3.51735323667612,-1.,2.25637049455044));
#41635=CARTESIAN_POINT('Ctrl Pts',(3.51735323667612,1.,2.25637049455044));
#41636=CARTESIAN_POINT('Ctrl Pts',(3.52514172847711,-1.,2.25727802940898));
#41637=CARTESIAN_POINT('Ctrl Pts',(3.52514172847711,1.,2.25727802940898));
#41638=CARTESIAN_POINT('Ctrl Pts',(3.53138243688262,-1.,2.25797812950104));
#41639=CARTESIAN_POINT('Ctrl Pts',(3.53138243688262,1.,2.25797812950104));
#41640=CARTESIAN_POINT('Ctrl Pts',(3.53606853162228,-1.,2.25848864343951));
#41641=CARTESIAN_POINT('Ctrl Pts',(3.53606853162228,1.,2.25848864343951));
#41642=CARTESIAN_POINT('Ctrl Pts',(3.53919506647335,-1.,2.2588225169468));
#41643=CARTESIAN_POINT('Ctrl Pts',(3.53919506647335,1.,2.2588225169468));
#41644=CARTESIAN_POINT('Ctrl Pts',(3.54075895182139,-1.,2.25898783642071));
#41645=CARTESIAN_POINT('Ctrl Pts',(3.54075895182139,1.,2.25898783642071));
#41646=CARTESIAN_POINT('',(3.08655633322212,1.,2.1297112484669));
#41647=CARTESIAN_POINT('Ctrl Pts',(3.08655633322211,-1.,2.1297112484669));
#41648=CARTESIAN_POINT('Ctrl Pts',(3.08655633322211,-0.666666666666667,
2.1297112484669));
#41649=CARTESIAN_POINT('Ctrl Pts',(3.08655633322211,-0.333333333333333,
2.1297112484669));
#41650=CARTESIAN_POINT('Ctrl Pts',(3.08655633322211,0.333333333333333,2.1297112484669));
#41651=CARTESIAN_POINT('Ctrl Pts',(3.08655633322212,0.666666666666667,2.1297112484669));
#41652=CARTESIAN_POINT('Ctrl Pts',(3.08655633322212,1.,2.1297112484669));
#41653=CARTESIAN_POINT('',(3.54075895182139,1.,2.25898783642071));
#41654=CARTESIAN_POINT('',(3.54075895182139,0.,2.25898783642071));
#41655=CARTESIAN_POINT('Ctrl Pts',(3.08655633322212,1.,2.1297112484669));
#41656=CARTESIAN_POINT('Ctrl Pts',(3.08657131089497,1.,2.1297578506149));
#41657=CARTESIAN_POINT('Ctrl Pts',(3.08668447250322,1.,2.12991938762374));
#41658=CARTESIAN_POINT('Ctrl Pts',(3.08717896996098,1.,2.13034980480424));
#41659=CARTESIAN_POINT('Ctrl Pts',(3.08855597949761,1.,2.13132142793017));
#41660=CARTESIAN_POINT('Ctrl Pts',(3.09151235281963,1.,2.13321032560894));
#41661=CARTESIAN_POINT('Ctrl Pts',(3.0960450242104,1.,2.13596538661048));
#41662=CARTESIAN_POINT('Ctrl Pts',(3.10171267391049,1.,2.13930228863751));
#41663=CARTESIAN_POINT('Ctrl Pts',(3.10821808668859,1.,2.14302815601973));
#41664=CARTESIAN_POINT('Ctrl Pts',(3.11522827016855,1.,2.14692798457532));
#41665=CARTESIAN_POINT('Ctrl Pts',(3.12242318151938,1.,2.15079698090585));
#41666=CARTESIAN_POINT('Ctrl Pts',(3.12954386795646,1.,2.1544724138292));
#41667=CARTESIAN_POINT('Ctrl Pts',(3.13645356563038,1.,2.15787423530676));
#41668=CARTESIAN_POINT('Ctrl Pts',(3.14314440427022,1.,2.16100905914435));
#41669=CARTESIAN_POINT('Ctrl Pts',(3.14968624389054,1.,2.16393520288072));
#41670=CARTESIAN_POINT('Ctrl Pts',(3.15618975593656,1.,2.1667372844769));
#41671=CARTESIAN_POINT('Ctrl Pts',(3.16276685102972,1.,2.16949910801219));
#41672=CARTESIAN_POINT('Ctrl Pts',(3.16948480019497,1.,2.17227212063817));
#41673=CARTESIAN_POINT('Ctrl Pts',(3.17635032802523,1.,2.17506466903694));
#41674=CARTESIAN_POINT('Ctrl Pts',(3.18333474627807,1.,2.17785968847142));
#41675=CARTESIAN_POINT('Ctrl Pts',(3.19038924261573,1.,2.18062558031778));
#41676=CARTESIAN_POINT('Ctrl Pts',(3.19746293740411,1.,2.18332898656602));
#41677=CARTESIAN_POINT('Ctrl Pts',(3.20452259717976,1.,2.18594876115934));
#41678=CARTESIAN_POINT('Ctrl Pts',(3.21156188355769,1.,2.18848253363901));
#41679=CARTESIAN_POINT('Ctrl Pts',(3.21859043114095,1.,2.19093901948667));
#41680=CARTESIAN_POINT('Ctrl Pts',(3.22562734221646,1.,2.19333345123538));
#41681=CARTESIAN_POINT('Ctrl Pts',(3.23269332296933,1.,2.19568204933168));
#41682=CARTESIAN_POINT('Ctrl Pts',(3.23980245361308,1.,2.19799623693253));
#41683=CARTESIAN_POINT('Ctrl Pts',(3.24695715874338,1.,2.20027910880981));
#41684=CARTESIAN_POINT('Ctrl Pts',(3.25415277957775,1.,2.20252866491545));
#41685=CARTESIAN_POINT('Ctrl Pts',(3.26138036637705,1.,2.20473979048678));
#41686=CARTESIAN_POINT('Ctrl Pts',(3.26863006136782,1.,2.20690665217743));
#41687=CARTESIAN_POINT('Ctrl Pts',(3.2758944800554,1.,2.2090250941743));
#41688=CARTESIAN_POINT('Ctrl Pts',(3.28317133333131,1.,2.21109449750641));
#41689=CARTESIAN_POINT('Ctrl Pts',(3.29046159238343,1.,2.21311648827391));
#41690=CARTESIAN_POINT('Ctrl Pts',(3.29776825193159,1.,2.21509406923369));
#41691=CARTESIAN_POINT('Ctrl Pts',(3.30509487819569,1.,2.21703059947836));
#41692=CARTESIAN_POINT('Ctrl Pts',(3.31244421655666,1.,2.21892881679086));
#41693=CARTESIAN_POINT('Ctrl Pts',(3.31981686778022,1.,2.22078990842776));
#41694=CARTESIAN_POINT('Ctrl Pts',(3.3272119632604,1.,2.22261398879635));
#41695=CARTESIAN_POINT('Ctrl Pts',(3.33462772849598,1.,2.22440049878511));
#41696=CARTESIAN_POINT('Ctrl Pts',(3.34206209449375,1.,2.22614863918047));
#41697=CARTESIAN_POINT('Ctrl Pts',(3.34951327111096,1.,2.22785777756576));
#41698=CARTESIAN_POINT('Ctrl Pts',(3.35698038165483,1.,2.22952789880983));
#41699=CARTESIAN_POINT('Ctrl Pts',(3.36446325227848,1.,2.23115945849739));
#41700=CARTESIAN_POINT('Ctrl Pts',(3.37196214349304,1.,2.23275319569221));
#41701=CARTESIAN_POINT('Ctrl Pts',(3.37947749555632,1.,2.23430995599561));
#41702=CARTESIAN_POINT('Ctrl Pts',(3.38700968549563,1.,2.23583052276308));
#41703=CARTESIAN_POINT('Ctrl Pts',(3.39455873448189,1.,2.23731541452791));
#41704=CARTESIAN_POINT('Ctrl Pts',(3.40212434705647,1.,2.23876491124151));
#41705=CARTESIAN_POINT('Ctrl Pts',(3.40970604190328,1.,2.24017914395289));
#41706=CARTESIAN_POINT('Ctrl Pts',(3.41730325539172,1.,2.24155816587844));
#41707=CARTESIAN_POINT('Ctrl Pts',(3.42491544683008,1.,2.24290202531101));
#41708=CARTESIAN_POINT('Ctrl Pts',(3.43254222614803,1.,2.24421085338727));
#41709=CARTESIAN_POINT('Ctrl Pts',(3.4401833646032,1.,2.24548487526022));
#41710=CARTESIAN_POINT('Ctrl Pts',(3.44783872863151,1.,2.2467243706995));
#41711=CARTESIAN_POINT('Ctrl Pts',(3.45550823512049,1.,2.2479296496077));
#41712=CARTESIAN_POINT('Ctrl Pts',(3.46319180177573,1.,2.2491010234604));
#41713=CARTESIAN_POINT('Ctrl Pts',(3.47088928979888,1.,2.25023877475942));
#41714=CARTESIAN_POINT('Ctrl Pts',(3.47860048448691,1.,2.25134314238687));
#41715=CARTESIAN_POINT('Ctrl Pts',(3.48632513240961,1.,2.25241433138695));
#41716=CARTESIAN_POINT('Ctrl Pts',(3.49406296494791,1.,2.2534525170976));
#41717=CARTESIAN_POINT('Ctrl Pts',(3.50181372617971,1.,2.25445785151868));
#41718=CARTESIAN_POINT('Ctrl Pts',(3.50957720117341,1.,2.255430469798));
#41719=CARTESIAN_POINT('Ctrl Pts',(3.51735323667612,1.,2.25637049455044));
#41720=CARTESIAN_POINT('Ctrl Pts',(3.52514172847711,1.,2.25727802940898));
#41721=CARTESIAN_POINT('Ctrl Pts',(3.53138243688262,1.,2.25797812950104));
#41722=CARTESIAN_POINT('Ctrl Pts',(3.53606853162228,1.,2.25848864343951));
#41723=CARTESIAN_POINT('Ctrl Pts',(3.53919506647335,1.,2.2588225169468));
#41724=CARTESIAN_POINT('Ctrl Pts',(3.54075895182139,1.,2.25898783642071));
#41725=CARTESIAN_POINT('Origin',(3.54075895182139,0.,2.25898783642071));
#41726=CARTESIAN_POINT('',(3.62024382630768,1.,2.12928030988903));
#41727=CARTESIAN_POINT('Origin',(0.,0.,0.));
#41728=CARTESIAN_POINT('',(2.97927412174388,1.,2.27737254473378));
#41729=CARTESIAN_POINT('Origin',(0.,1.,0.));
#41730=CARTESIAN_POINT('Ctrl Pts',(2.97927412174388,1.,2.27737254473378));
#41731=CARTESIAN_POINT('Ctrl Pts',(2.97927412174388,0.666666666666667,2.27737254473378));
#41732=CARTESIAN_POINT('Ctrl Pts',(2.97927412174388,0.333333333333333,2.27737254473378));
#41733=CARTESIAN_POINT('Ctrl Pts',(2.97927412174388,-0.333333333333333,
2.27737254473378));
#41734=CARTESIAN_POINT('Ctrl Pts',(2.97927412174388,-0.666666666666667,
2.27737254473378));
#41735=CARTESIAN_POINT('Ctrl Pts',(2.97927412174388,-1.,2.27737254473378));
#41736=CARTESIAN_POINT('Ctrl Pts',(3.24257979115744,-1.,2.66939624221984));
#41737=CARTESIAN_POINT('Ctrl Pts',(3.24257979115744,1.,2.66939624221984));
#41738=CARTESIAN_POINT('Ctrl Pts',(3.24193929584813,-1.,2.66795998539861));
#41739=CARTESIAN_POINT('Ctrl Pts',(3.24193929584813,1.,2.66795998539861));
#41740=CARTESIAN_POINT('Ctrl Pts',(3.24065561087681,-1.,2.66508964664767));
#41741=CARTESIAN_POINT('Ctrl Pts',(3.24065561087681,1.,2.66508964664767));
#41742=CARTESIAN_POINT('Ctrl Pts',(3.23872200036311,-1.,2.6607906631973));
#41743=CARTESIAN_POINT('Ctrl Pts',(3.23872200036311,1.,2.6607906631973));
#41744=CARTESIAN_POINT('Ctrl Pts',(3.23612768065687,-1.,2.6550717396303));
#41745=CARTESIAN_POINT('Ctrl Pts',(3.23612768065687,1.,2.6550717396303));
#41746=CARTESIAN_POINT('Ctrl Pts',(3.23285778738558,-1.,2.64794488744246));
#41747=CARTESIAN_POINT('Ctrl Pts',(3.23285778738558,1.,2.64794488744246));
#41748=CARTESIAN_POINT('Ctrl Pts',(3.2295608435934,-1.,2.64083992182478));
#41749=CARTESIAN_POINT('Ctrl Pts',(3.2295608435934,1.,2.64083992182478));
#41750=CARTESIAN_POINT('Ctrl Pts',(3.22623678292539,-1.,2.63375697391438));
#41751=CARTESIAN_POINT('Ctrl Pts',(3.22623678292539,1.,2.63375697391438));
#41752=CARTESIAN_POINT('Ctrl Pts',(3.222885536128,-1.,2.62669622735548));
#41753=CARTESIAN_POINT('Ctrl Pts',(3.222885536128,1.,2.62669622735548));
#41754=CARTESIAN_POINT('Ctrl Pts',(3.21950704108654,-1.,2.61965792832396));
#41755=CARTESIAN_POINT('Ctrl Pts',(3.21950704108654,1.,2.61965792832396));
#41756=CARTESIAN_POINT('Ctrl Pts',(3.21610123232465,-1.,2.61264236718662));
#41757=CARTESIAN_POINT('Ctrl Pts',(3.21610123232465,1.,2.61264236718662));
#41758=CARTESIAN_POINT('Ctrl Pts',(3.21266802609297,-1.,2.60564985359699));
#41759=CARTESIAN_POINT('Ctrl Pts',(3.21266802609297,1.,2.60564985359699));
#41760=CARTESIAN_POINT('Ctrl Pts',(3.2092073056959,-1.,2.59868069194267));
#41761=CARTESIAN_POINT('Ctrl Pts',(3.2092073056959,1.,2.59868069194267));
#41762=CARTESIAN_POINT('Ctrl Pts',(3.20571891028879,-1.,2.59173516023605));
#41763=CARTESIAN_POINT('Ctrl Pts',(3.20571891028879,1.,2.59173516023605));
#41764=CARTESIAN_POINT('Ctrl Pts',(3.20220261408685,-1.,2.58481347777953));
#41765=CARTESIAN_POINT('Ctrl Pts',(3.20220261408685,1.,2.58481347777953));
#41766=CARTESIAN_POINT('Ctrl Pts',(3.19865814628955,-1.,2.577915819091));
#41767=CARTESIAN_POINT('Ctrl Pts',(3.19865814628955,1.,2.577915819091));
#41768=CARTESIAN_POINT('Ctrl Pts',(3.19508523784548,-1.,2.57104235898053));
#41769=CARTESIAN_POINT('Ctrl Pts',(3.19508523784548,1.,2.57104235898053));
#41770=CARTESIAN_POINT('Ctrl Pts',(3.19148366395201,-1.,2.56419331092909));
#41771=CARTESIAN_POINT('Ctrl Pts',(3.19148366395201,1.,2.56419331092909));
#41772=CARTESIAN_POINT('Ctrl Pts',(3.1878532811617,-1.,2.55736896206016));
#41773=CARTESIAN_POINT('Ctrl Pts',(3.1878532811617,1.,2.55736896206016));
#41774=CARTESIAN_POINT('Ctrl Pts',(3.18419408529482,-1.,2.55056972387638));
#41775=CARTESIAN_POINT('Ctrl Pts',(3.18419408529482,1.,2.55056972387638));
#41776=CARTESIAN_POINT('Ctrl Pts',(3.18050619750515,-1.,2.54379612552948));
#41777=CARTESIAN_POINT('Ctrl Pts',(3.18050619750515,1.,2.54379612552948));
#41778=CARTESIAN_POINT('Ctrl Pts',(3.17678974135225,-1.,2.53704871950871));
#41779=CARTESIAN_POINT('Ctrl Pts',(3.17678974135225,1.,2.53704871950871));
#41780=CARTESIAN_POINT('Ctrl Pts',(3.17304474093574,-1.,2.5303280040691));
#41781=CARTESIAN_POINT('Ctrl Pts',(3.17304474093574,1.,2.5303280040691));
#41782=CARTESIAN_POINT('Ctrl Pts',(3.1692710213075,-1.,2.523634346718));
#41783=CARTESIAN_POINT('Ctrl Pts',(3.1692710213075,1.,2.523634346718));
#41784=CARTESIAN_POINT('Ctrl Pts',(3.16546808277069,-1.,2.51696788755616));
#41785=CARTESIAN_POINT('Ctrl Pts',(3.16546808277069,1.,2.51696788755616));
#41786=CARTESIAN_POINT('Ctrl Pts',(3.16163506380211,-1.,2.51032851007939));
#41787=CARTESIAN_POINT('Ctrl Pts',(3.16163506380211,1.,2.51032851007939));
#41788=CARTESIAN_POINT('Ctrl Pts',(3.15777102413998,-1.,2.50371605688287));
#41789=CARTESIAN_POINT('Ctrl Pts',(3.15777102413998,1.,2.50371605688287));
#41790=CARTESIAN_POINT('Ctrl Pts',(3.15387518039064,-1.,2.49713050858911));
#41791=CARTESIAN_POINT('Ctrl Pts',(3.15387518039064,1.,2.49713050858911));
#41792=CARTESIAN_POINT('Ctrl Pts',(3.14994715298903,-1.,2.49057217131985));
#41793=CARTESIAN_POINT('Ctrl Pts',(3.14994715298903,1.,2.49057217131985));
#41794=CARTESIAN_POINT('Ctrl Pts',(3.14598722723879,-1.,2.48404187418376));
#41795=CARTESIAN_POINT('Ctrl Pts',(3.14598722723879,1.,2.48404187418376));
#41796=CARTESIAN_POINT('Ctrl Pts',(3.14199655778845,-1.,2.47754112428028));
#41797=CARTESIAN_POINT('Ctrl Pts',(3.14199655778845,1.,2.47754112428028));
#41798=CARTESIAN_POINT('Ctrl Pts',(3.13797654408931,-1.,2.47107164236827));
#41799=CARTESIAN_POINT('Ctrl Pts',(3.13797654408931,1.,2.47107164236827));
#41800=CARTESIAN_POINT('Ctrl Pts',(3.13392826623902,-1.,2.4646349433237));
#41801=CARTESIAN_POINT('Ctrl Pts',(3.13392826623902,1.,2.4646349433237));
#41802=CARTESIAN_POINT('Ctrl Pts',(3.12985188384372,-1.,2.45823188859367));
#41803=CARTESIAN_POINT('Ctrl Pts',(3.12985188384372,1.,2.45823188859367));
#41804=CARTESIAN_POINT('Ctrl Pts',(3.12574608210849,-1.,2.45186227369848));
#41805=CARTESIAN_POINT('Ctrl Pts',(3.12574608210849,1.,2.45186227369848));
#41806=CARTESIAN_POINT('Ctrl Pts',(3.12160740887768,-1.,2.44552433364716));
#41807=CARTESIAN_POINT('Ctrl Pts',(3.12160740887768,1.,2.44552433364716));
#41808=CARTESIAN_POINT('Ctrl Pts',(3.11743156744182,-1.,2.43921571477975));
#41809=CARTESIAN_POINT('Ctrl Pts',(3.11743156744182,1.,2.43921571477975));
#41810=CARTESIAN_POINT('Ctrl Pts',(3.11321477659012,-1.,2.4329344968514));
#41811=CARTESIAN_POINT('Ctrl Pts',(3.11321477659012,1.,2.4329344968514));
#41812=CARTESIAN_POINT('Ctrl Pts',(3.10895518969592,-1.,2.42668025870013));
#41813=CARTESIAN_POINT('Ctrl Pts',(3.10895518969592,1.,2.42668025870013));
#41814=CARTESIAN_POINT('Ctrl Pts',(3.10465410280902,-1.,2.42045498612494));
#41815=CARTESIAN_POINT('Ctrl Pts',(3.10465410280902,1.,2.42045498612494));
#41816=CARTESIAN_POINT('Ctrl Pts',(3.10031775027683,-1.,2.41426441798067));
#41817=CARTESIAN_POINT('Ctrl Pts',(3.10031775027683,1.,2.41426441798067));
#41818=CARTESIAN_POINT('Ctrl Pts',(3.09595472616093,-1.,2.40811612696382));
#41819=CARTESIAN_POINT('Ctrl Pts',(3.09595472616093,1.,2.40811612696382));
#41820=CARTESIAN_POINT('Ctrl Pts',(3.09157266051115,-1.,2.40201704423352));
#41821=CARTESIAN_POINT('Ctrl Pts',(3.09157266051115,1.,2.40201704423352));
#41822=CARTESIAN_POINT('Ctrl Pts',(3.08717489512919,-1.,2.39597098250635));
#41823=CARTESIAN_POINT('Ctrl Pts',(3.08717489512919,1.,2.39597098250635));
#41824=CARTESIAN_POINT('Ctrl Pts',(3.08275773747083,-1.,2.38997659219192));
#41825=CARTESIAN_POINT('Ctrl Pts',(3.08275773747083,1.,2.38997659219192));
#41826=CARTESIAN_POINT('Ctrl Pts',(3.07830597244301,-1.,2.38402401216107));
#41827=CARTESIAN_POINT('Ctrl Pts',(3.07830597244301,1.,2.38402401216107));
#41828=CARTESIAN_POINT('Ctrl Pts',(3.07379777492133,-1.,2.37809856205524));
#41829=CARTESIAN_POINT('Ctrl Pts',(3.07379777492133,1.,2.37809856205524));
#41830=CARTESIAN_POINT('Ctrl Pts',(3.06921275497472,-1.,2.37218678163157));
#41831=CARTESIAN_POINT('Ctrl Pts',(3.06921275497472,1.,2.37218678163157));
#41832=CARTESIAN_POINT('Ctrl Pts',(3.06453964643152,-1.,2.36628220107001));
#41833=CARTESIAN_POINT('Ctrl Pts',(3.06453964643152,1.,2.36628220107001));
#41834=CARTESIAN_POINT('Ctrl Pts',(3.05978266240056,-1.,2.36039011602084));
#41835=CARTESIAN_POINT('Ctrl Pts',(3.05978266240056,1.,2.36039011602084));
#41836=CARTESIAN_POINT('Ctrl Pts',(3.05497218368188,-1.,2.35453559889506));
#41837=CARTESIAN_POINT('Ctrl Pts',(3.05497218368188,1.,2.35453559889506));
#41838=CARTESIAN_POINT('Ctrl Pts',(3.05015565829976,-1.,2.34875673090816));
#41839=CARTESIAN_POINT('Ctrl Pts',(3.05015565829976,1.,2.34875673090816));
#41840=CARTESIAN_POINT('Ctrl Pts',(3.04537822217311,-1.,2.3430901708402));
#41841=CARTESIAN_POINT('Ctrl Pts',(3.04537822217311,1.,2.3430901708402));
#41842=CARTESIAN_POINT('Ctrl Pts',(3.04066496998569,-1.,2.33755792953726));
#41843=CARTESIAN_POINT('Ctrl Pts',(3.04066496998569,1.,2.33755792953726));
#41844=CARTESIAN_POINT('Ctrl Pts',(3.03600588555765,-1.,2.33215619079807));
#41845=CARTESIAN_POINT('Ctrl Pts',(3.03600588555765,1.,2.33215619079807));
#41846=CARTESIAN_POINT('Ctrl Pts',(3.03133125185047,-1.,2.32683687412027));
#41847=CARTESIAN_POINT('Ctrl Pts',(3.03133125185047,1.,2.32683687412027));
#41848=CARTESIAN_POINT('Ctrl Pts',(3.02652678416478,-1.,2.32151944306299));
#41849=CARTESIAN_POINT('Ctrl Pts',(3.02652678416478,1.,2.32151944306299));
#41850=CARTESIAN_POINT('Ctrl Pts',(3.02147780668029,-1.,2.31612479121528));
#41851=CARTESIAN_POINT('Ctrl Pts',(3.02147780668029,1.,2.31612479121528));
#41852=CARTESIAN_POINT('Ctrl Pts',(3.01610726819019,-1.,2.31060449886577));
#41853=CARTESIAN_POINT('Ctrl Pts',(3.01610726819019,1.,2.31060449886577));
#41854=CARTESIAN_POINT('Ctrl Pts',(3.01041131063882,-1.,2.30496809486529));
#41855=CARTESIAN_POINT('Ctrl Pts',(3.01041131063882,1.,2.30496809486529));
#41856=CARTESIAN_POINT('Ctrl Pts',(3.00450832658822,-1.,2.29932091315939));
#41857=CARTESIAN_POINT('Ctrl Pts',(3.00450832658822,1.,2.29932091315939));
#41858=CARTESIAN_POINT('Ctrl Pts',(2.99863310340004,-1.,2.29385894577999));
#41859=CARTESIAN_POINT('Ctrl Pts',(2.99863310340004,1.,2.29385894577999));
#41860=CARTESIAN_POINT('Ctrl Pts',(2.9930793098434,-1.,2.28882328690601));
#41861=CARTESIAN_POINT('Ctrl Pts',(2.9930793098434,1.,2.28882328690601));
#41862=CARTESIAN_POINT('Ctrl Pts',(2.98815432734929,-1.,2.28446419116036));
#41863=CARTESIAN_POINT('Ctrl Pts',(2.98815432734929,1.,2.28446419116036));
#41864=CARTESIAN_POINT('Ctrl Pts',(2.98413343613858,-1.,2.28100472516582));
#41865=CARTESIAN_POINT('Ctrl Pts',(2.98413343613858,1.,2.28100472516582));
#41866=CARTESIAN_POINT('Ctrl Pts',(2.98120357932601,-1.,2.2785960133424));
#41867=CARTESIAN_POINT('Ctrl Pts',(2.98120357932601,1.,2.2785960133424));
#41868=CARTESIAN_POINT('Ctrl Pts',(2.97980276182744,-1.,2.27756633754846));
#41869=CARTESIAN_POINT('Ctrl Pts',(2.97980276182744,1.,2.27756633754846));
#41870=CARTESIAN_POINT('Ctrl Pts',(2.97929608861502,-1.,2.27730961189188));
#41871=CARTESIAN_POINT('Ctrl Pts',(2.97929608861502,1.,2.27730961189188));
#41872=CARTESIAN_POINT('Ctrl Pts',(2.97919987915565,-1.,2.2773674298423));
#41873=CARTESIAN_POINT('Ctrl Pts',(2.97919987915565,1.,2.2773674298423));
#41874=CARTESIAN_POINT('Ctrl Pts',(2.97921217251145,-1.,2.27745358485296));
#41875=CARTESIAN_POINT('Ctrl Pts',(2.97921217251145,1.,2.27745358485296));
#41876=CARTESIAN_POINT('',(3.24257979115744,1.,2.66939624221984));
#41877=CARTESIAN_POINT('Ctrl Pts',(3.24257979115744,1.,2.66939624221984));
#41878=CARTESIAN_POINT('Ctrl Pts',(3.24193929584813,1.,2.66795998539861));
#41879=CARTESIAN_POINT('Ctrl Pts',(3.24065561087681,1.,2.66508964664767));
#41880=CARTESIAN_POINT('Ctrl Pts',(3.23872200036311,1.,2.6607906631973));
#41881=CARTESIAN_POINT('Ctrl Pts',(3.23612768065687,1.,2.6550717396303));
#41882=CARTESIAN_POINT('Ctrl Pts',(3.23285778738558,1.,2.64794488744246));
#41883=CARTESIAN_POINT('Ctrl Pts',(3.2295608435934,1.,2.64083992182478));
#41884=CARTESIAN_POINT('Ctrl Pts',(3.22623678292539,1.,2.63375697391438));
#41885=CARTESIAN_POINT('Ctrl Pts',(3.222885536128,1.,2.62669622735548));
#41886=CARTESIAN_POINT('Ctrl Pts',(3.21950704108654,1.,2.61965792832396));
#41887=CARTESIAN_POINT('Ctrl Pts',(3.21610123232465,1.,2.61264236718662));
#41888=CARTESIAN_POINT('Ctrl Pts',(3.21266802609297,1.,2.60564985359699));
#41889=CARTESIAN_POINT('Ctrl Pts',(3.2092073056959,1.,2.59868069194267));
#41890=CARTESIAN_POINT('Ctrl Pts',(3.20571891028879,1.,2.59173516023605));
#41891=CARTESIAN_POINT('Ctrl Pts',(3.20220261408685,1.,2.58481347777953));
#41892=CARTESIAN_POINT('Ctrl Pts',(3.19865814628955,1.,2.577915819091));
#41893=CARTESIAN_POINT('Ctrl Pts',(3.19508523784548,1.,2.57104235898053));
#41894=CARTESIAN_POINT('Ctrl Pts',(3.19148366395201,1.,2.56419331092909));
#41895=CARTESIAN_POINT('Ctrl Pts',(3.1878532811617,1.,2.55736896206016));
#41896=CARTESIAN_POINT('Ctrl Pts',(3.18419408529482,1.,2.55056972387638));
#41897=CARTESIAN_POINT('Ctrl Pts',(3.18050619750515,1.,2.54379612552948));
#41898=CARTESIAN_POINT('Ctrl Pts',(3.17678974135225,1.,2.53704871950871));
#41899=CARTESIAN_POINT('Ctrl Pts',(3.17304474093574,1.,2.5303280040691));
#41900=CARTESIAN_POINT('Ctrl Pts',(3.1692710213075,1.,2.523634346718));
#41901=CARTESIAN_POINT('Ctrl Pts',(3.16546808277069,1.,2.51696788755616));
#41902=CARTESIAN_POINT('Ctrl Pts',(3.16163506380211,1.,2.51032851007939));
#41903=CARTESIAN_POINT('Ctrl Pts',(3.15777102413998,1.,2.50371605688287));
#41904=CARTESIAN_POINT('Ctrl Pts',(3.15387518039064,1.,2.49713050858911));
#41905=CARTESIAN_POINT('Ctrl Pts',(3.14994715298903,1.,2.49057217131985));
#41906=CARTESIAN_POINT('Ctrl Pts',(3.14598722723879,1.,2.48404187418376));
#41907=CARTESIAN_POINT('Ctrl Pts',(3.14199655778845,1.,2.47754112428028));
#41908=CARTESIAN_POINT('Ctrl Pts',(3.13797654408931,1.,2.47107164236827));
#41909=CARTESIAN_POINT('Ctrl Pts',(3.13392826623902,1.,2.4646349433237));
#41910=CARTESIAN_POINT('Ctrl Pts',(3.12985188384372,1.,2.45823188859367));
#41911=CARTESIAN_POINT('Ctrl Pts',(3.12574608210849,1.,2.45186227369848));
#41912=CARTESIAN_POINT('Ctrl Pts',(3.12160740887768,1.,2.44552433364716));
#41913=CARTESIAN_POINT('Ctrl Pts',(3.11743156744182,1.,2.43921571477975));
#41914=CARTESIAN_POINT('Ctrl Pts',(3.11321477659012,1.,2.4329344968514));
#41915=CARTESIAN_POINT('Ctrl Pts',(3.10895518969592,1.,2.42668025870013));
#41916=CARTESIAN_POINT('Ctrl Pts',(3.10465410280902,1.,2.42045498612494));
#41917=CARTESIAN_POINT('Ctrl Pts',(3.10031775027683,1.,2.41426441798067));
#41918=CARTESIAN_POINT('Ctrl Pts',(3.09595472616093,1.,2.40811612696382));
#41919=CARTESIAN_POINT('Ctrl Pts',(3.09157266051115,1.,2.40201704423352));
#41920=CARTESIAN_POINT('Ctrl Pts',(3.08717489512919,1.,2.39597098250635));
#41921=CARTESIAN_POINT('Ctrl Pts',(3.08275773747083,1.,2.38997659219192));
#41922=CARTESIAN_POINT('Ctrl Pts',(3.07830597244301,1.,2.38402401216107));
#41923=CARTESIAN_POINT('Ctrl Pts',(3.07379777492133,1.,2.37809856205524));
#41924=CARTESIAN_POINT('Ctrl Pts',(3.06921275497472,1.,2.37218678163157));
#41925=CARTESIAN_POINT('Ctrl Pts',(3.06453964643152,1.,2.36628220107001));
#41926=CARTESIAN_POINT('Ctrl Pts',(3.05978266240056,1.,2.36039011602084));
#41927=CARTESIAN_POINT('Ctrl Pts',(3.05497218368188,1.,2.35453559889506));
#41928=CARTESIAN_POINT('Ctrl Pts',(3.05015565829976,1.,2.34875673090816));
#41929=CARTESIAN_POINT('Ctrl Pts',(3.04537822217311,1.,2.3430901708402));
#41930=CARTESIAN_POINT('Ctrl Pts',(3.04066496998569,1.,2.33755792953726));
#41931=CARTESIAN_POINT('Ctrl Pts',(3.03600588555765,1.,2.33215619079807));
#41932=CARTESIAN_POINT('Ctrl Pts',(3.03133125185047,1.,2.32683687412027));
#41933=CARTESIAN_POINT('Ctrl Pts',(3.02652678416478,1.,2.32151944306299));
#41934=CARTESIAN_POINT('Ctrl Pts',(3.02147780668029,1.,2.31612479121528));
#41935=CARTESIAN_POINT('Ctrl Pts',(3.01610726819019,1.,2.31060449886577));
#41936=CARTESIAN_POINT('Ctrl Pts',(3.01041131063882,1.,2.30496809486529));
#41937=CARTESIAN_POINT('Ctrl Pts',(3.00450832658822,1.,2.29932091315939));
#41938=CARTESIAN_POINT('Ctrl Pts',(2.99863310340004,1.,2.29385894577999));
#41939=CARTESIAN_POINT('Ctrl Pts',(2.9930793098434,1.,2.28882328690601));
#41940=CARTESIAN_POINT('Ctrl Pts',(2.98815432734929,1.,2.28446419116036));
#41941=CARTESIAN_POINT('Ctrl Pts',(2.98413343613858,1.,2.28100472516582));
#41942=CARTESIAN_POINT('Ctrl Pts',(2.98142341809623,1.,2.27877674853833));
#41943=CARTESIAN_POINT('Ctrl Pts',(2.98007383024333,1.,2.27776738270369));
#41944=CARTESIAN_POINT('Ctrl Pts',(2.97951167106106,1.,2.27743009389704));
#41945=CARTESIAN_POINT('Ctrl Pts',(2.97932307137589,1.,2.27737238849212));
#41946=CARTESIAN_POINT('Ctrl Pts',(2.97927412174388,1.,2.27737254473378));
#41947=CARTESIAN_POINT('',(3.24257979115744,0.,2.66939624221984));
#41948=CARTESIAN_POINT('Ctrl Pts',(2.71546581445404,-1.,2.58626089374824));
#41949=CARTESIAN_POINT('Ctrl Pts',(2.71546581445404,1.,2.58626089374824));
#41950=CARTESIAN_POINT('Ctrl Pts',(2.71537879705104,-1.,2.58626222935804));
#41951=CARTESIAN_POINT('Ctrl Pts',(2.71537879705104,1.,2.58626222935804));
#41952=CARTESIAN_POINT('Ctrl Pts',(2.71533674141254,-1.,2.58636629904103));
#41953=CARTESIAN_POINT('Ctrl Pts',(2.71533674141254,1.,2.58636629904103));
#41954=CARTESIAN_POINT('Ctrl Pts',(2.71566956750452,-1.,2.5868265735259));
#41955=CARTESIAN_POINT('Ctrl Pts',(2.71566956750452,1.,2.5868265735259));
#41956=CARTESIAN_POINT('Ctrl Pts',(2.71690570241638,-1.,2.58804906785417));
#41957=CARTESIAN_POINT('Ctrl Pts',(2.71690570241638,1.,2.58804906785417));
#41958=CARTESIAN_POINT('Ctrl Pts',(2.71974308958086,-1.,2.59056604771971));
#41959=CARTESIAN_POINT('Ctrl Pts',(2.71974308958086,1.,2.59056604771971));
#41960=CARTESIAN_POINT('Ctrl Pts',(2.72378896977134,-1.,2.59399625537278));
#41961=CARTESIAN_POINT('Ctrl Pts',(2.72378896977134,1.,2.59399625537278));
#41962=CARTESIAN_POINT('Ctrl Pts',(2.7288648348152,-1.,2.59817869034746));
#41963=CARTESIAN_POINT('Ctrl Pts',(2.7288648348152,1.,2.59817869034746));
#41964=CARTESIAN_POINT('Ctrl Pts',(2.73470730109615,-1.,2.60287635688728));
#41965=CARTESIAN_POINT('Ctrl Pts',(2.73470730109615,1.,2.60287635688728));
#41966=CARTESIAN_POINT('Ctrl Pts',(2.7410211099909,-1.,2.60782480638448));
#41967=CARTESIAN_POINT('Ctrl Pts',(2.7410211099909,1.,2.60782480638448));
#41968=CARTESIAN_POINT('Ctrl Pts',(2.74752219567252,-1.,2.61277170105813));
#41969=CARTESIAN_POINT('Ctrl Pts',(2.74752219567252,1.,2.61277170105813));
#41970=CARTESIAN_POINT('Ctrl Pts',(2.7539802502603,-1.,2.61751580407667));
#41971=CARTESIAN_POINT('Ctrl Pts',(2.7539802502603,1.,2.61751580407667));
#41972=CARTESIAN_POINT('Ctrl Pts',(2.76027271596686,-1.,2.62195665834605));
#41973=CARTESIAN_POINT('Ctrl Pts',(2.76027271596686,1.,2.62195665834605));
#41974=CARTESIAN_POINT('Ctrl Pts',(2.7663907847902,-1.,2.62609956506355));
#41975=CARTESIAN_POINT('Ctrl Pts',(2.7663907847902,1.,2.62609956506355));
#41976=CARTESIAN_POINT('Ctrl Pts',(2.77239433377921,-1.,2.63001305229625));
#41977=CARTESIAN_POINT('Ctrl Pts',(2.77239433377921,1.,2.63001305229625));
#41978=CARTESIAN_POINT('Ctrl Pts',(2.77837943466449,-1.,2.63379800904599));
#41979=CARTESIAN_POINT('Ctrl Pts',(2.77837943466449,1.,2.63379800904599));
#41980=CARTESIAN_POINT('Ctrl Pts',(2.78444351041571,-1.,2.637554714303));
#41981=CARTESIAN_POINT('Ctrl Pts',(2.78444351041571,1.,2.637554714303));
#41982=CARTESIAN_POINT('Ctrl Pts',(2.79064495573224,-1.,2.64134450532584));
#41983=CARTESIAN_POINT('Ctrl Pts',(2.79064495573224,1.,2.64134450532584));
#41984=CARTESIAN_POINT('Ctrl Pts',(2.79698910670736,-1.,2.6451766779932));
#41985=CARTESIAN_POINT('Ctrl Pts',(2.79698910670736,1.,2.6451766779932));
#41986=CARTESIAN_POINT('Ctrl Pts',(2.80345029781152,-1.,2.64902988983337));
#41987=CARTESIAN_POINT('Ctrl Pts',(2.80345029781152,1.,2.64902988983337));
#41988=CARTESIAN_POINT('Ctrl Pts',(2.80998526078165,-1.,2.65286529532208));
#41989=CARTESIAN_POINT('Ctrl Pts',(2.80998526078165,1.,2.65286529532208));
#41990=CARTESIAN_POINT('Ctrl Pts',(2.81654896073883,-1.,2.65664198781344));
#41991=CARTESIAN_POINT('Ctrl Pts',(2.81654896073883,1.,2.65664198781344));
#41992=CARTESIAN_POINT('Ctrl Pts',(2.82311188135078,-1.,2.66033388273461));
#41993=CARTESIAN_POINT('Ctrl Pts',(2.82311188135078,1.,2.66033388273461));
#41994=CARTESIAN_POINT('Ctrl Pts',(2.82966813308998,-1.,2.6639376472693));
#41995=CARTESIAN_POINT('Ctrl Pts',(2.82966813308998,1.,2.6639376472693));
#41996=CARTESIAN_POINT('Ctrl Pts',(2.83622586853982,-1.,2.66746339678107));
#41997=CARTESIAN_POINT('Ctrl Pts',(2.83622586853982,1.,2.66746339678107));
#41998=CARTESIAN_POINT('Ctrl Pts',(2.84280157191323,-1.,2.67092916452125));
#41999=CARTESIAN_POINT('Ctrl Pts',(2.84280157191323,1.,2.67092916452125));
#42000=CARTESIAN_POINT('Ctrl Pts',(2.84941315703092,-1.,2.67435421039677));
#42001=CARTESIAN_POINT('Ctrl Pts',(2.84941315703092,1.,2.67435421039677));
#42002=CARTESIAN_POINT('Ctrl Pts',(2.85607274378017,-1.,2.67775201955724));
#42003=CARTESIAN_POINT('Ctrl Pts',(2.85607274378017,1.,2.67775201955724));
#42004=CARTESIAN_POINT('Ctrl Pts',(2.86278224277689,-1.,2.68112602796308));
#42005=CARTESIAN_POINT('Ctrl Pts',(2.86278224277689,1.,2.68112602796308));
#42006=CARTESIAN_POINT('Ctrl Pts',(2.86953736547238,-1.,2.68447353139599));
#42007=CARTESIAN_POINT('Ctrl Pts',(2.86953736547238,1.,2.68447353139599));
#42008=CARTESIAN_POINT('Ctrl Pts',(2.8763300724388,-1.,2.68778807801686));
#42009=CARTESIAN_POINT('Ctrl Pts',(2.8763300724388,1.,2.68778807801686));
#42010=CARTESIAN_POINT('Ctrl Pts',(2.88315153980466,-1.,2.69106236420198));
#42011=CARTESIAN_POINT('Ctrl Pts',(2.88315153980466,1.,2.69106236420198));
#42012=CARTESIAN_POINT('Ctrl Pts',(2.88999512410309,-1.,2.69429113011374));
#42013=CARTESIAN_POINT('Ctrl Pts',(2.88999512410309,1.,2.69429113011374));
#42014=CARTESIAN_POINT('Ctrl Pts',(2.89685866123671,-1.,2.69747340630625));
#42015=CARTESIAN_POINT('Ctrl Pts',(2.89685866123671,1.,2.69747340630625));
#42016=CARTESIAN_POINT('Ctrl Pts',(2.90374285605838,-1.,2.70061095078692));
#42017=CARTESIAN_POINT('Ctrl Pts',(2.90374285605838,1.,2.70061095078692));
#42018=CARTESIAN_POINT('Ctrl Pts',(2.91065019668329,-1.,2.70370719782113));
#42019=CARTESIAN_POINT('Ctrl Pts',(2.91065019668329,1.,2.70370719782113));
#42020=CARTESIAN_POINT('Ctrl Pts',(2.91758367994737,-1.,2.70676602302518));
#42021=CARTESIAN_POINT('Ctrl Pts',(2.91758367994737,1.,2.70676602302518));
#42022=CARTESIAN_POINT('Ctrl Pts',(2.92454558914778,-1.,2.70979055994754));
#42023=CARTESIAN_POINT('Ctrl Pts',(2.92454558914778,1.,2.70979055994754));
#42024=CARTESIAN_POINT('Ctrl Pts',(2.93153633192595,-1.,2.71278207520817));
#42025=CARTESIAN_POINT('Ctrl Pts',(2.93153633192595,1.,2.71278207520817));
#42026=CARTESIAN_POINT('Ctrl Pts',(2.93855503247266,-1.,2.71574054592591));
#42027=CARTESIAN_POINT('Ctrl Pts',(2.93855503247266,1.,2.71574054592591));
#42028=CARTESIAN_POINT('Ctrl Pts',(2.94560002559805,-1.,2.71866514227965));
#42029=CARTESIAN_POINT('Ctrl Pts',(2.94560002559805,1.,2.71866514227965));
#42030=CARTESIAN_POINT('Ctrl Pts',(2.95266939280621,-1.,2.72155475123364));
#42031=CARTESIAN_POINT('Ctrl Pts',(2.95266939280621,1.,2.72155475123364));
#42032=CARTESIAN_POINT('Ctrl Pts',(2.95976146492576,-1.,2.72440846811729));
#42033=CARTESIAN_POINT('Ctrl Pts',(2.95976146492576,1.,2.72440846811729));
#42034=CARTESIAN_POINT('Ctrl Pts',(2.96687537842451,-1.,2.72722614084076));
#42035=CARTESIAN_POINT('Ctrl Pts',(2.96687537842451,1.,2.72722614084076));
#42036=CARTESIAN_POINT('Ctrl Pts',(2.97401089032676,-1.,2.73000819218414));
#42037=CARTESIAN_POINT('Ctrl Pts',(2.97401089032676,1.,2.73000819218414));
#42038=CARTESIAN_POINT('Ctrl Pts',(2.98116814232129,-1.,2.73275539286497));
#42039=CARTESIAN_POINT('Ctrl Pts',(2.98116814232129,1.,2.73275539286497));
#42040=CARTESIAN_POINT('Ctrl Pts',(2.9883474369644,-1.,2.73546864694536));
#42041=CARTESIAN_POINT('Ctrl Pts',(2.9883474369644,1.,2.73546864694536));
#42042=CARTESIAN_POINT('Ctrl Pts',(2.99554902409778,-1.,2.73814878711641));
#42043=CARTESIAN_POINT('Ctrl Pts',(2.99554902409778,1.,2.73814878711641));
#42044=CARTESIAN_POINT('Ctrl Pts',(3.00277284351521,-1.,2.74079632883931));
#42045=CARTESIAN_POINT('Ctrl Pts',(3.00277284351521,1.,2.74079632883931));
#42046=CARTESIAN_POINT('Ctrl Pts',(3.01001855960162,-1.,2.74341150239887));
#42047=CARTESIAN_POINT('Ctrl Pts',(3.01001855960162,1.,2.74341150239887));
#42048=CARTESIAN_POINT('Ctrl Pts',(3.01728567646611,-1.,2.74599436193625));
#42049=CARTESIAN_POINT('Ctrl Pts',(3.01728567646611,1.,2.74599436193625));
#42050=CARTESIAN_POINT('Ctrl Pts',(3.02457362909245,-1.,2.7485448718414));
#42051=CARTESIAN_POINT('Ctrl Pts',(3.02457362909245,1.,2.7485448718414));
#42052=CARTESIAN_POINT('Ctrl Pts',(3.03188187589107,-1.,2.75106299522979));
#42053=CARTESIAN_POINT('Ctrl Pts',(3.03188187589107,1.,2.75106299522979));
#42054=CARTESIAN_POINT('Ctrl Pts',(3.03921001107977,-1.,2.75354880060314));
#42055=CARTESIAN_POINT('Ctrl Pts',(3.03921001107977,1.,2.75354880060314));
#42056=CARTESIAN_POINT('Ctrl Pts',(3.04655777351067,-1.,2.75600247455925));
#42057=CARTESIAN_POINT('Ctrl Pts',(3.04655777351067,1.,2.75600247455925));
#42058=CARTESIAN_POINT('Ctrl Pts',(3.05392498749847,-1.,2.75842427252931));
#42059=CARTESIAN_POINT('Ctrl Pts',(3.05392498749847,1.,2.75842427252931));
#42060=CARTESIAN_POINT('Ctrl Pts',(3.06131152247454,-1.,2.76081448759882));
#42061=CARTESIAN_POINT('Ctrl Pts',(3.06131152247454,1.,2.76081448759882));
#42062=CARTESIAN_POINT('Ctrl Pts',(3.0687172484321,-1.,2.76317341453493));
#42063=CARTESIAN_POINT('Ctrl Pts',(3.0687172484321,1.,2.76317341453493));
#42064=CARTESIAN_POINT('Ctrl Pts',(3.07614198408862,-1.,2.76550131064852));
#42065=CARTESIAN_POINT('Ctrl Pts',(3.07614198408862,1.,2.76550131064852));
#42066=CARTESIAN_POINT('Ctrl Pts',(3.08358548001503,-1.,2.76779837829373));
#42067=CARTESIAN_POINT('Ctrl Pts',(3.08358548001503,1.,2.76779837829373));
#42068=CARTESIAN_POINT('Ctrl Pts',(3.0910474538253,-1.,2.7700647803451));
#42069=CARTESIAN_POINT('Ctrl Pts',(3.0910474538253,1.,2.7700647803451));
#42070=CARTESIAN_POINT('Ctrl Pts',(3.0985276127786,-1.,2.77230064796057));
#42071=CARTESIAN_POINT('Ctrl Pts',(3.0985276127786,1.,2.77230064796057));
#42072=CARTESIAN_POINT('Ctrl Pts',(3.10602568032564,-1.,2.77450609123362));
#42073=CARTESIAN_POINT('Ctrl Pts',(3.10602568032564,1.,2.77450609123362));
#42074=CARTESIAN_POINT('Ctrl Pts',(3.11354142303921,-1.,2.77668121002545));
#42075=CARTESIAN_POINT('Ctrl Pts',(3.11354142303921,1.,2.77668121002545));
#42076=CARTESIAN_POINT('Ctrl Pts',(3.12107467037201,-1.,2.77882610146731));
#42077=CARTESIAN_POINT('Ctrl Pts',(3.12107467037201,1.,2.77882610146731));
#42078=CARTESIAN_POINT('Ctrl Pts',(3.12862530318457,-1.,2.78094085161413));
#42079=CARTESIAN_POINT('Ctrl Pts',(3.12862530318457,1.,2.78094085161413));
#42080=CARTESIAN_POINT('Ctrl Pts',(3.13467965833037,-1.,2.78260859419319));
#42081=CARTESIAN_POINT('Ctrl Pts',(3.13467965833037,1.,2.78260859419319));
#42082=CARTESIAN_POINT('Ctrl Pts',(3.13922819749279,-1.,2.78384588958166));
#42083=CARTESIAN_POINT('Ctrl Pts',(3.13922819749279,1.,2.78384588958166));
#42084=CARTESIAN_POINT('Ctrl Pts',(3.14226401018816,-1.,2.7846647503589));
#42085=CARTESIAN_POINT('Ctrl Pts',(3.14226401018816,1.,2.7846647503589));
#42086=CARTESIAN_POINT('Ctrl Pts',(3.14378277984898,-1.,2.78507268004356));
#42087=CARTESIAN_POINT('Ctrl Pts',(3.14378277984898,1.,2.78507268004356));
#42088=CARTESIAN_POINT('',(2.71539546306948,1.,2.58633475774921));
#42089=CARTESIAN_POINT('Ctrl Pts',(2.71539546306948,-1.,2.58633475774921));
#42090=CARTESIAN_POINT('Ctrl Pts',(2.71539546306948,-0.666666666666667,
2.58633475774921));
#42091=CARTESIAN_POINT('Ctrl Pts',(2.71539546306948,-0.333333333333333,
2.58633475774921));
#42092=CARTESIAN_POINT('Ctrl Pts',(2.71539546306948,0.333333333333333,2.58633475774921));
#42093=CARTESIAN_POINT('Ctrl Pts',(2.71539546306948,0.666666666666667,2.58633475774921));
#42094=CARTESIAN_POINT('Ctrl Pts',(2.71539546306948,1.,2.58633475774921));
#42095=CARTESIAN_POINT('',(3.14378277984898,1.,2.78507268004356));
#42096=CARTESIAN_POINT('',(3.14378277984898,0.,2.78507268004356));
#42097=CARTESIAN_POINT('Ctrl Pts',(2.71539546306948,1.,2.58633475774921));
#42098=CARTESIAN_POINT('Ctrl Pts',(2.71540296616024,1.,2.58638312917167));
#42099=CARTESIAN_POINT('Ctrl Pts',(2.71548946460575,1.,2.58656037976753));
#42100=CARTESIAN_POINT('Ctrl Pts',(2.71591054189786,1.,2.58706285424358));
#42101=CARTESIAN_POINT('Ctrl Pts',(2.71711860281815,1.,2.58823792682672));
#42102=CARTESIAN_POINT('Ctrl Pts',(2.71974308958086,1.,2.59056604771971));
#42103=CARTESIAN_POINT('Ctrl Pts',(2.72378896977134,1.,2.59399625537278));
#42104=CARTESIAN_POINT('Ctrl Pts',(2.7288648348152,1.,2.59817869034746));
#42105=CARTESIAN_POINT('Ctrl Pts',(2.73470730109615,1.,2.60287635688728));
#42106=CARTESIAN_POINT('Ctrl Pts',(2.7410211099909,1.,2.60782480638448));
#42107=CARTESIAN_POINT('Ctrl Pts',(2.74752219567252,1.,2.61277170105813));
#42108=CARTESIAN_POINT('Ctrl Pts',(2.7539802502603,1.,2.61751580407667));
#42109=CARTESIAN_POINT('Ctrl Pts',(2.76027271596686,1.,2.62195665834605));
#42110=CARTESIAN_POINT('Ctrl Pts',(2.7663907847902,1.,2.62609956506355));
#42111=CARTESIAN_POINT('Ctrl Pts',(2.77239433377921,1.,2.63001305229625));
#42112=CARTESIAN_POINT('Ctrl Pts',(2.77837943466449,1.,2.63379800904599));
#42113=CARTESIAN_POINT('Ctrl Pts',(2.78444351041571,1.,2.637554714303));
#42114=CARTESIAN_POINT('Ctrl Pts',(2.79064495573224,1.,2.64134450532584));
#42115=CARTESIAN_POINT('Ctrl Pts',(2.79698910670736,1.,2.6451766779932));
#42116=CARTESIAN_POINT('Ctrl Pts',(2.80345029781152,1.,2.64902988983337));
#42117=CARTESIAN_POINT('Ctrl Pts',(2.80998526078165,1.,2.65286529532208));
#42118=CARTESIAN_POINT('Ctrl Pts',(2.81654896073883,1.,2.65664198781344));
#42119=CARTESIAN_POINT('Ctrl Pts',(2.82311188135078,1.,2.66033388273461));
#42120=CARTESIAN_POINT('Ctrl Pts',(2.82966813308998,1.,2.6639376472693));
#42121=CARTESIAN_POINT('Ctrl Pts',(2.83622586853982,1.,2.66746339678107));
#42122=CARTESIAN_POINT('Ctrl Pts',(2.84280157191323,1.,2.67092916452125));
#42123=CARTESIAN_POINT('Ctrl Pts',(2.84941315703092,1.,2.67435421039677));
#42124=CARTESIAN_POINT('Ctrl Pts',(2.85607274378017,1.,2.67775201955724));
#42125=CARTESIAN_POINT('Ctrl Pts',(2.86278224277689,1.,2.68112602796308));
#42126=CARTESIAN_POINT('Ctrl Pts',(2.86953736547238,1.,2.68447353139599));
#42127=CARTESIAN_POINT('Ctrl Pts',(2.8763300724388,1.,2.68778807801686));
#42128=CARTESIAN_POINT('Ctrl Pts',(2.88315153980466,1.,2.69106236420198));
#42129=CARTESIAN_POINT('Ctrl Pts',(2.88999512410309,1.,2.69429113011374));
#42130=CARTESIAN_POINT('Ctrl Pts',(2.89685866123671,1.,2.69747340630625));
#42131=CARTESIAN_POINT('Ctrl Pts',(2.90374285605838,1.,2.70061095078692));
#42132=CARTESIAN_POINT('Ctrl Pts',(2.91065019668329,1.,2.70370719782113));
#42133=CARTESIAN_POINT('Ctrl Pts',(2.91758367994737,1.,2.70676602302518));
#42134=CARTESIAN_POINT('Ctrl Pts',(2.92454558914778,1.,2.70979055994754));
#42135=CARTESIAN_POINT('Ctrl Pts',(2.93153633192595,1.,2.71278207520817));
#42136=CARTESIAN_POINT('Ctrl Pts',(2.93855503247266,1.,2.71574054592591));
#42137=CARTESIAN_POINT('Ctrl Pts',(2.94560002559805,1.,2.71866514227965));
#42138=CARTESIAN_POINT('Ctrl Pts',(2.95266939280621,1.,2.72155475123364));
#42139=CARTESIAN_POINT('Ctrl Pts',(2.95976146492576,1.,2.72440846811729));
#42140=CARTESIAN_POINT('Ctrl Pts',(2.96687537842451,1.,2.72722614084076));
#42141=CARTESIAN_POINT('Ctrl Pts',(2.97401089032676,1.,2.73000819218414));
#42142=CARTESIAN_POINT('Ctrl Pts',(2.98116814232129,1.,2.73275539286497));
#42143=CARTESIAN_POINT('Ctrl Pts',(2.9883474369644,1.,2.73546864694536));
#42144=CARTESIAN_POINT('Ctrl Pts',(2.99554902409778,1.,2.73814878711641));
#42145=CARTESIAN_POINT('Ctrl Pts',(3.00277284351521,1.,2.74079632883931));
#42146=CARTESIAN_POINT('Ctrl Pts',(3.01001855960162,1.,2.74341150239887));
#42147=CARTESIAN_POINT('Ctrl Pts',(3.01728567646611,1.,2.74599436193625));
#42148=CARTESIAN_POINT('Ctrl Pts',(3.02457362909245,1.,2.7485448718414));
#42149=CARTESIAN_POINT('Ctrl Pts',(3.03188187589107,1.,2.75106299522979));
#42150=CARTESIAN_POINT('Ctrl Pts',(3.03921001107977,1.,2.75354880060314));
#42151=CARTESIAN_POINT('Ctrl Pts',(3.04655777351067,1.,2.75600247455925));
#42152=CARTESIAN_POINT('Ctrl Pts',(3.05392498749847,1.,2.75842427252931));
#42153=CARTESIAN_POINT('Ctrl Pts',(3.06131152247454,1.,2.76081448759882));
#42154=CARTESIAN_POINT('Ctrl Pts',(3.0687172484321,1.,2.76317341453493));
#42155=CARTESIAN_POINT('Ctrl Pts',(3.07614198408862,1.,2.76550131064852));
#42156=CARTESIAN_POINT('Ctrl Pts',(3.08358548001503,1.,2.76779837829373));
#42157=CARTESIAN_POINT('Ctrl Pts',(3.0910474538253,1.,2.7700647803451));
#42158=CARTESIAN_POINT('Ctrl Pts',(3.0985276127786,1.,2.77230064796057));
#42159=CARTESIAN_POINT('Ctrl Pts',(3.10602568032564,1.,2.77450609123362));
#42160=CARTESIAN_POINT('Ctrl Pts',(3.11354142303921,1.,2.77668121002545));
#42161=CARTESIAN_POINT('Ctrl Pts',(3.12107467037201,1.,2.77882610146731));
#42162=CARTESIAN_POINT('Ctrl Pts',(3.12862530318457,1.,2.78094085161413));
#42163=CARTESIAN_POINT('Ctrl Pts',(3.13467965833037,1.,2.78260859419319));
#42164=CARTESIAN_POINT('Ctrl Pts',(3.13922819749279,1.,2.78384588958166));
#42165=CARTESIAN_POINT('Ctrl Pts',(3.14226401018816,1.,2.7846647503589));
#42166=CARTESIAN_POINT('Ctrl Pts',(3.14378277984898,1.,2.78507268004356));
#42167=CARTESIAN_POINT('Origin',(3.14378277984898,0.,2.78507268004356));
#42168=CARTESIAN_POINT('',(3.24257979115744,1.,2.66939624221984));
#42169=CARTESIAN_POINT('Origin',(0.,0.,0.));
#42170=CARTESIAN_POINT('',(2.58633475775051,1.,2.71539546306824));
#42171=CARTESIAN_POINT('Origin',(0.,1.,0.));
#42172=CARTESIAN_POINT('Ctrl Pts',(2.58633475775051,1.,2.71539546306824));
#42173=CARTESIAN_POINT('Ctrl Pts',(2.58633475775051,0.666666666666667,2.71539546306824));
#42174=CARTESIAN_POINT('Ctrl Pts',(2.58633475775051,0.333333333333333,2.71539546306824));
#42175=CARTESIAN_POINT('Ctrl Pts',(2.58633475775051,-0.333333333333333,
2.71539546306824));
#42176=CARTESIAN_POINT('Ctrl Pts',(2.58633475775051,-0.666666666666667,
2.71539546306824));
#42177=CARTESIAN_POINT('Ctrl Pts',(2.58633475775051,-1.,2.71539546306824));
#42178=CARTESIAN_POINT('Ctrl Pts',(2.78507268004355,-1.,3.14378277984898));
#42179=CARTESIAN_POINT('Ctrl Pts',(2.78507268004355,1.,3.14378277984898));
#42180=CARTESIAN_POINT('Ctrl Pts',(2.78466475036183,-1.,3.14226401019149));
#42181=CARTESIAN_POINT('Ctrl Pts',(2.78466475036183,1.,3.14226401019149));
#42182=CARTESIAN_POINT('Ctrl Pts',(2.78384588958965,-1.,3.13922819750185));
#42183=CARTESIAN_POINT('Ctrl Pts',(2.78384588958965,1.,3.13922819750185));
#42184=CARTESIAN_POINT('Ctrl Pts',(2.78260859420629,-1.,3.1346796583452));
#42185=CARTESIAN_POINT('Ctrl Pts',(2.78260859420629,1.,3.1346796583452));
#42186=CARTESIAN_POINT('Ctrl Pts',(2.78094085162947,-1.,3.12862530320194));
#42187=CARTESIAN_POINT('Ctrl Pts',(2.78094085162947,1.,3.12862530320194));
#42188=CARTESIAN_POINT('Ctrl Pts',(2.77882610147986,-1.,3.12107467038623));
#42189=CARTESIAN_POINT('Ctrl Pts',(2.77882610147986,1.,3.12107467038623));
#42190=CARTESIAN_POINT('Ctrl Pts',(2.77668121003225,-1.,3.11354142304692));
#42191=CARTESIAN_POINT('Ctrl Pts',(2.77668121003225,1.,3.11354142304692));
#42192=CARTESIAN_POINT('Ctrl Pts',(2.7745060912343,-1.,3.10602568032641));
#42193=CARTESIAN_POINT('Ctrl Pts',(2.7745060912343,1.,3.10602568032641));
#42194=CARTESIAN_POINT('Ctrl Pts',(2.77230064795679,-1.,3.09852761277432));
#42195=CARTESIAN_POINT('Ctrl Pts',(2.77230064795679,1.,3.09852761277432));
#42196=CARTESIAN_POINT('Ctrl Pts',(2.77006478033937,-1.,3.09104745381882));
#42197=CARTESIAN_POINT('Ctrl Pts',(2.77006478033937,1.,3.09104745381882));
#42198=CARTESIAN_POINT('Ctrl Pts',(2.76779837828843,-1.,3.08358548000904));
#42199=CARTESIAN_POINT('Ctrl Pts',(2.76779837828843,1.,3.08358548000904));
#42200=CARTESIAN_POINT('Ctrl Pts',(2.76550131064522,-1.,3.07614198408488));
#42201=CARTESIAN_POINT('Ctrl Pts',(2.76550131064522,1.,3.07614198408488));
#42202=CARTESIAN_POINT('Ctrl Pts',(2.76317341453415,-1.,3.06871724843121));
#42203=CARTESIAN_POINT('Ctrl Pts',(2.76317341453415,1.,3.06871724843121));
#42204=CARTESIAN_POINT('Ctrl Pts',(2.76081448760011,-1.,3.06131152247599));
#42205=CARTESIAN_POINT('Ctrl Pts',(2.76081448760011,1.,3.06131152247599));
#42206=CARTESIAN_POINT('Ctrl Pts',(2.75842427253164,-1.,3.05392498750112));
#42207=CARTESIAN_POINT('Ctrl Pts',(2.75842427253164,1.,3.05392498750112));
#42208=CARTESIAN_POINT('Ctrl Pts',(2.7560024745616,-1.,3.04655777351333));
#42209=CARTESIAN_POINT('Ctrl Pts',(2.7560024745616,1.,3.04655777351333));
#42210=CARTESIAN_POINT('Ctrl Pts',(2.75354880060473,-1.,3.03921001108158));
#42211=CARTESIAN_POINT('Ctrl Pts',(2.75354880060473,1.,3.03921001108158));
#42212=CARTESIAN_POINT('Ctrl Pts',(2.75106299523032,-1.,3.03188187589168));
#42213=CARTESIAN_POINT('Ctrl Pts',(2.75106299523032,1.,3.03188187589168));
#42214=CARTESIAN_POINT('Ctrl Pts',(2.74854487184099,-1.,3.02457362909199));
#42215=CARTESIAN_POINT('Ctrl Pts',(2.74854487184099,1.,3.02457362909199));
#42216=CARTESIAN_POINT('Ctrl Pts',(2.74599436193528,-1.,3.01728567646502));
#42217=CARTESIAN_POINT('Ctrl Pts',(2.74599436193528,1.,3.01728567646502));
#42218=CARTESIAN_POINT('Ctrl Pts',(2.7434115023978,-1.,3.01001855960041));
#42219=CARTESIAN_POINT('Ctrl Pts',(2.7434115023978,1.,3.01001855960041));
#42220=CARTESIAN_POINT('Ctrl Pts',(2.74079632883852,-1.,3.00277284351431));
#42221=CARTESIAN_POINT('Ctrl Pts',(2.74079632883852,1.,3.00277284351431));
#42222=CARTESIAN_POINT('Ctrl Pts',(2.73814878711609,-1.,2.99554902409741));
#42223=CARTESIAN_POINT('Ctrl Pts',(2.73814878711609,1.,2.99554902409741));
#42224=CARTESIAN_POINT('Ctrl Pts',(2.73546864694548,-1.,2.98834743696455));
#42225=CARTESIAN_POINT('Ctrl Pts',(2.73546864694548,1.,2.98834743696455));
#42226=CARTESIAN_POINT('Ctrl Pts',(2.73275539286537,-1.,2.98116814232175));
#42227=CARTESIAN_POINT('Ctrl Pts',(2.73275539286537,1.,2.98116814232175));
#42228=CARTESIAN_POINT('Ctrl Pts',(2.7300081921846,-1.,2.97401089032729));
#42229=CARTESIAN_POINT('Ctrl Pts',(2.7300081921846,1.,2.97401089032729));
#42230=CARTESIAN_POINT('Ctrl Pts',(2.72722614084112,-1.,2.96687537842492));
#42231=CARTESIAN_POINT('Ctrl Pts',(2.72722614084112,1.,2.96687537842492));
#42232=CARTESIAN_POINT('Ctrl Pts',(2.72440846811745,-1.,2.95976146492595));
#42233=CARTESIAN_POINT('Ctrl Pts',(2.72440846811745,1.,2.95976146492595));
#42234=CARTESIAN_POINT('Ctrl Pts',(2.72155475123361,-1.,2.95266939280617));
#42235=CARTESIAN_POINT('Ctrl Pts',(2.72155475123361,1.,2.95266939280617));
#42236=CARTESIAN_POINT('Ctrl Pts',(2.71866514227951,-1.,2.94560002559789));
#42237=CARTESIAN_POINT('Ctrl Pts',(2.71866514227951,1.,2.94560002559789));
#42238=CARTESIAN_POINT('Ctrl Pts',(2.71574054592575,-1.,2.93855503247248));
#42239=CARTESIAN_POINT('Ctrl Pts',(2.71574054592575,1.,2.93855503247248));
#42240=CARTESIAN_POINT('Ctrl Pts',(2.71278207520807,-1.,2.93153633192583));
#42241=CARTESIAN_POINT('Ctrl Pts',(2.71278207520807,1.,2.93153633192583));
#42242=CARTESIAN_POINT('Ctrl Pts',(2.70979055994751,-1.,2.92454558914774));
#42243=CARTESIAN_POINT('Ctrl Pts',(2.70979055994751,1.,2.92454558914774));
#42244=CARTESIAN_POINT('Ctrl Pts',(2.70676602302518,-1.,2.91758367994738));
#42245=CARTESIAN_POINT('Ctrl Pts',(2.70676602302518,1.,2.91758367994738));
#42246=CARTESIAN_POINT('Ctrl Pts',(2.70370719782114,-1.,2.91065019668331));
#42247=CARTESIAN_POINT('Ctrl Pts',(2.70370719782114,1.,2.91065019668331));
#42248=CARTESIAN_POINT('Ctrl Pts',(2.70061095078692,-1.,2.90374285605839));
#42249=CARTESIAN_POINT('Ctrl Pts',(2.70061095078692,1.,2.90374285605839));
#42250=CARTESIAN_POINT('Ctrl Pts',(2.69747340630621,-1.,2.89685866123668));
#42251=CARTESIAN_POINT('Ctrl Pts',(2.69747340630621,1.,2.89685866123668));
#42252=CARTESIAN_POINT('Ctrl Pts',(2.69429113011369,-1.,2.88999512410304));
#42253=CARTESIAN_POINT('Ctrl Pts',(2.69429113011369,1.,2.88999512410304));
#42254=CARTESIAN_POINT('Ctrl Pts',(2.69106236420196,-1.,2.88315153980464));
#42255=CARTESIAN_POINT('Ctrl Pts',(2.69106236420196,1.,2.88315153980464));
#42256=CARTESIAN_POINT('Ctrl Pts',(2.68778807801691,-1.,2.87633007243885));
#42257=CARTESIAN_POINT('Ctrl Pts',(2.68778807801691,1.,2.87633007243885));
#42258=CARTESIAN_POINT('Ctrl Pts',(2.6844735313961,-1.,2.8695373654725));
#42259=CARTESIAN_POINT('Ctrl Pts',(2.6844735313961,1.,2.8695373654725));
#42260=CARTESIAN_POINT('Ctrl Pts',(2.68112602796323,-1.,2.86278224277705));
#42261=CARTESIAN_POINT('Ctrl Pts',(2.68112602796323,1.,2.86278224277705));
#42262=CARTESIAN_POINT('Ctrl Pts',(2.67775201955736,-1.,2.85607274378031));
#42263=CARTESIAN_POINT('Ctrl Pts',(2.67775201955736,1.,2.85607274378031));
#42264=CARTESIAN_POINT('Ctrl Pts',(2.67435421039682,-1.,2.84941315703096));
#42265=CARTESIAN_POINT('Ctrl Pts',(2.67435421039682,1.,2.84941315703096));
#42266=CARTESIAN_POINT('Ctrl Pts',(2.67092916452116,-1.,2.84280157191314));
#42267=CARTESIAN_POINT('Ctrl Pts',(2.67092916452116,1.,2.84280157191314));
#42268=CARTESIAN_POINT('Ctrl Pts',(2.66746339678085,-1.,2.8362258685396));
#42269=CARTESIAN_POINT('Ctrl Pts',(2.66746339678085,1.,2.8362258685396));
#42270=CARTESIAN_POINT('Ctrl Pts',(2.66393764726902,-1.,2.82966813308969));
#42271=CARTESIAN_POINT('Ctrl Pts',(2.66393764726902,1.,2.82966813308969));
#42272=CARTESIAN_POINT('Ctrl Pts',(2.66033388273437,-1.,2.82311188135053));
#42273=CARTESIAN_POINT('Ctrl Pts',(2.66033388273437,1.,2.82311188135053));
#42274=CARTESIAN_POINT('Ctrl Pts',(2.65664198781335,-1.,2.81654896073874));
#42275=CARTESIAN_POINT('Ctrl Pts',(2.65664198781335,1.,2.81654896073874));
#42276=CARTESIAN_POINT('Ctrl Pts',(2.65286529532221,-1.,2.80998526078179));
#42277=CARTESIAN_POINT('Ctrl Pts',(2.65286529532221,1.,2.80998526078179));
#42278=CARTESIAN_POINT('Ctrl Pts',(2.64902988983373,-1.,2.80345029781191));
#42279=CARTESIAN_POINT('Ctrl Pts',(2.64902988983373,1.,2.80345029781191));
#42280=CARTESIAN_POINT('Ctrl Pts',(2.6451766779937,-1.,2.7969891067079));
#42281=CARTESIAN_POINT('Ctrl Pts',(2.6451766779937,1.,2.7969891067079));
#42282=CARTESIAN_POINT('Ctrl Pts',(2.64134450532632,-1.,2.79064495573275));
#42283=CARTESIAN_POINT('Ctrl Pts',(2.64134450532632,1.,2.79064495573275));
#42284=CARTESIAN_POINT('Ctrl Pts',(2.63755471430322,-1.,2.78444351041594));
#42285=CARTESIAN_POINT('Ctrl Pts',(2.63755471430322,1.,2.78444351041594));
#42286=CARTESIAN_POINT('Ctrl Pts',(2.63379800904575,-1.,2.77837943466423));
#42287=CARTESIAN_POINT('Ctrl Pts',(2.63379800904575,1.,2.77837943466423));
#42288=CARTESIAN_POINT('Ctrl Pts',(2.63001305229548,-1.,2.77239433377839));
#42289=CARTESIAN_POINT('Ctrl Pts',(2.63001305229548,1.,2.77239433377839));
#42290=CARTESIAN_POINT('Ctrl Pts',(2.6260995650624,-1.,2.76639078478898));
#42291=CARTESIAN_POINT('Ctrl Pts',(2.6260995650624,1.,2.76639078478898));
#42292=CARTESIAN_POINT('Ctrl Pts',(2.62195665834491,-1.,2.76027271596564));
#42293=CARTESIAN_POINT('Ctrl Pts',(2.62195665834491,1.,2.76027271596564));
#42294=CARTESIAN_POINT('Ctrl Pts',(2.61751580407608,-1.,2.75398025025967));
#42295=CARTESIAN_POINT('Ctrl Pts',(2.61751580407608,1.,2.75398025025967));
#42296=CARTESIAN_POINT('Ctrl Pts',(2.61277170105864,-1.,2.74752219567307));
#42297=CARTESIAN_POINT('Ctrl Pts',(2.61277170105864,1.,2.74752219567307));
#42298=CARTESIAN_POINT('Ctrl Pts',(2.60782480638629,-1.,2.74102110999284));
#42299=CARTESIAN_POINT('Ctrl Pts',(2.60782480638629,1.,2.74102110999284));
#42300=CARTESIAN_POINT('Ctrl Pts',(2.60287635689,-1.,2.73470730109906));
#42301=CARTESIAN_POINT('Ctrl Pts',(2.60287635689,1.,2.73470730109906));
#42302=CARTESIAN_POINT('Ctrl Pts',(2.5981786903501,-1.,2.72886483481804));
#42303=CARTESIAN_POINT('Ctrl Pts',(2.5981786903501,1.,2.72886483481804));
#42304=CARTESIAN_POINT('Ctrl Pts',(2.59399625537407,-1.,2.72378896977273));
#42305=CARTESIAN_POINT('Ctrl Pts',(2.59399625537407,1.,2.72378896977273));
#42306=CARTESIAN_POINT('Ctrl Pts',(2.59056604771863,-1.,2.7197430895797));
#42307=CARTESIAN_POINT('Ctrl Pts',(2.59056604771863,1.,2.7197430895797));
#42308=CARTESIAN_POINT('Ctrl Pts',(2.58804906785077,-1.,2.71690570241274));
#42309=CARTESIAN_POINT('Ctrl Pts',(2.58804906785077,1.,2.71690570241274));
#42310=CARTESIAN_POINT('Ctrl Pts',(2.58682657352212,-1.,2.71566956750046));
#42311=CARTESIAN_POINT('Ctrl Pts',(2.58682657352212,1.,2.71566956750046));
#42312=CARTESIAN_POINT('Ctrl Pts',(2.58636629903847,-1.,2.71533674140979));
#42313=CARTESIAN_POINT('Ctrl Pts',(2.58636629903847,1.,2.71533674140979));
#42314=CARTESIAN_POINT('Ctrl Pts',(2.58626222935706,-1.,2.71537879705));
#42315=CARTESIAN_POINT('Ctrl Pts',(2.58626222935706,1.,2.71537879705));
#42316=CARTESIAN_POINT('Ctrl Pts',(2.58626089374824,-1.,2.71546581445404));
#42317=CARTESIAN_POINT('Ctrl Pts',(2.58626089374824,1.,2.71546581445404));
#42318=CARTESIAN_POINT('',(2.78507268004355,1.,3.14378277984898));
#42319=CARTESIAN_POINT('Ctrl Pts',(2.78507268004355,1.,3.14378277984898));
#42320=CARTESIAN_POINT('Ctrl Pts',(2.78466475036183,1.,3.14226401019149));
#42321=CARTESIAN_POINT('Ctrl Pts',(2.78384588958965,1.,3.13922819750185));
#42322=CARTESIAN_POINT('Ctrl Pts',(2.78260859420629,1.,3.1346796583452));
#42323=CARTESIAN_POINT('Ctrl Pts',(2.78094085162947,1.,3.12862530320194));
#42324=CARTESIAN_POINT('Ctrl Pts',(2.77882610147986,1.,3.12107467038623));
#42325=CARTESIAN_POINT('Ctrl Pts',(2.77668121003225,1.,3.11354142304692));
#42326=CARTESIAN_POINT('Ctrl Pts',(2.7745060912343,1.,3.10602568032641));
#42327=CARTESIAN_POINT('Ctrl Pts',(2.77230064795679,1.,3.09852761277432));
#42328=CARTESIAN_POINT('Ctrl Pts',(2.77006478033937,1.,3.09104745381882));
#42329=CARTESIAN_POINT('Ctrl Pts',(2.76779837828843,1.,3.08358548000904));
#42330=CARTESIAN_POINT('Ctrl Pts',(2.76550131064522,1.,3.07614198408488));
#42331=CARTESIAN_POINT('Ctrl Pts',(2.76317341453415,1.,3.06871724843121));
#42332=CARTESIAN_POINT('Ctrl Pts',(2.76081448760011,1.,3.06131152247599));
#42333=CARTESIAN_POINT('Ctrl Pts',(2.75842427253164,1.,3.05392498750112));
#42334=CARTESIAN_POINT('Ctrl Pts',(2.7560024745616,1.,3.04655777351333));
#42335=CARTESIAN_POINT('Ctrl Pts',(2.75354880060473,1.,3.03921001108158));
#42336=CARTESIAN_POINT('Ctrl Pts',(2.75106299523032,1.,3.03188187589168));
#42337=CARTESIAN_POINT('Ctrl Pts',(2.74854487184099,1.,3.02457362909199));
#42338=CARTESIAN_POINT('Ctrl Pts',(2.74599436193528,1.,3.01728567646502));
#42339=CARTESIAN_POINT('Ctrl Pts',(2.7434115023978,1.,3.01001855960041));
#42340=CARTESIAN_POINT('Ctrl Pts',(2.74079632883852,1.,3.00277284351431));
#42341=CARTESIAN_POINT('Ctrl Pts',(2.73814878711609,1.,2.99554902409741));
#42342=CARTESIAN_POINT('Ctrl Pts',(2.73546864694548,1.,2.98834743696455));
#42343=CARTESIAN_POINT('Ctrl Pts',(2.73275539286537,1.,2.98116814232175));
#42344=CARTESIAN_POINT('Ctrl Pts',(2.7300081921846,1.,2.97401089032729));
#42345=CARTESIAN_POINT('Ctrl Pts',(2.72722614084112,1.,2.96687537842492));
#42346=CARTESIAN_POINT('Ctrl Pts',(2.72440846811745,1.,2.95976146492595));
#42347=CARTESIAN_POINT('Ctrl Pts',(2.72155475123361,1.,2.95266939280617));
#42348=CARTESIAN_POINT('Ctrl Pts',(2.71866514227951,1.,2.94560002559789));
#42349=CARTESIAN_POINT('Ctrl Pts',(2.71574054592575,1.,2.93855503247248));
#42350=CARTESIAN_POINT('Ctrl Pts',(2.71278207520807,1.,2.93153633192583));
#42351=CARTESIAN_POINT('Ctrl Pts',(2.70979055994751,1.,2.92454558914774));
#42352=CARTESIAN_POINT('Ctrl Pts',(2.70676602302518,1.,2.91758367994738));
#42353=CARTESIAN_POINT('Ctrl Pts',(2.70370719782114,1.,2.91065019668331));
#42354=CARTESIAN_POINT('Ctrl Pts',(2.70061095078692,1.,2.90374285605839));
#42355=CARTESIAN_POINT('Ctrl Pts',(2.69747340630621,1.,2.89685866123668));
#42356=CARTESIAN_POINT('Ctrl Pts',(2.69429113011369,1.,2.88999512410304));
#42357=CARTESIAN_POINT('Ctrl Pts',(2.69106236420196,1.,2.88315153980464));
#42358=CARTESIAN_POINT('Ctrl Pts',(2.68778807801691,1.,2.87633007243885));
#42359=CARTESIAN_POINT('Ctrl Pts',(2.6844735313961,1.,2.8695373654725));
#42360=CARTESIAN_POINT('Ctrl Pts',(2.68112602796323,1.,2.86278224277705));
#42361=CARTESIAN_POINT('Ctrl Pts',(2.67775201955736,1.,2.85607274378031));
#42362=CARTESIAN_POINT('Ctrl Pts',(2.67435421039682,1.,2.84941315703096));
#42363=CARTESIAN_POINT('Ctrl Pts',(2.67092916452116,1.,2.84280157191314));
#42364=CARTESIAN_POINT('Ctrl Pts',(2.66746339678085,1.,2.8362258685396));
#42365=CARTESIAN_POINT('Ctrl Pts',(2.66393764726902,1.,2.82966813308969));
#42366=CARTESIAN_POINT('Ctrl Pts',(2.66033388273437,1.,2.82311188135053));
#42367=CARTESIAN_POINT('Ctrl Pts',(2.65664198781335,1.,2.81654896073874));
#42368=CARTESIAN_POINT('Ctrl Pts',(2.65286529532221,1.,2.80998526078179));
#42369=CARTESIAN_POINT('Ctrl Pts',(2.64902988983373,1.,2.80345029781191));
#42370=CARTESIAN_POINT('Ctrl Pts',(2.6451766779937,1.,2.7969891067079));
#42371=CARTESIAN_POINT('Ctrl Pts',(2.64134450532632,1.,2.79064495573275));
#42372=CARTESIAN_POINT('Ctrl Pts',(2.63755471430322,1.,2.78444351041594));
#42373=CARTESIAN_POINT('Ctrl Pts',(2.63379800904575,1.,2.77837943466423));
#42374=CARTESIAN_POINT('Ctrl Pts',(2.63001305229548,1.,2.77239433377839));
#42375=CARTESIAN_POINT('Ctrl Pts',(2.6260995650624,1.,2.76639078478898));
#42376=CARTESIAN_POINT('Ctrl Pts',(2.62195665834491,1.,2.76027271596564));
#42377=CARTESIAN_POINT('Ctrl Pts',(2.61751580407608,1.,2.75398025025967));
#42378=CARTESIAN_POINT('Ctrl Pts',(2.61277170105864,1.,2.74752219567307));
#42379=CARTESIAN_POINT('Ctrl Pts',(2.60782480638629,1.,2.74102110999284));
#42380=CARTESIAN_POINT('Ctrl Pts',(2.60287635689,1.,2.73470730109906));
#42381=CARTESIAN_POINT('Ctrl Pts',(2.5981786903501,1.,2.72886483481804));
#42382=CARTESIAN_POINT('Ctrl Pts',(2.59399625537407,1.,2.72378896977273));
#42383=CARTESIAN_POINT('Ctrl Pts',(2.59056604771863,1.,2.7197430895797));
#42384=CARTESIAN_POINT('Ctrl Pts',(2.58823792682724,1.,2.71711860281891));
#42385=CARTESIAN_POINT('Ctrl Pts',(2.58706285424469,1.,2.71591054189884));
#42386=CARTESIAN_POINT('Ctrl Pts',(2.58656037976884,1.,2.71548946460616));
#42387=CARTESIAN_POINT('Ctrl Pts',(2.58638312917291,1.,2.71540296615967));
#42388=CARTESIAN_POINT('Ctrl Pts',(2.58633475775051,1.,2.71539546306824));
#42389=CARTESIAN_POINT('',(2.78507268004355,0.,3.14378277984898));
#42390=CARTESIAN_POINT('Ctrl Pts',(2.27745358485296,-1.,2.97921217251145));
#42391=CARTESIAN_POINT('Ctrl Pts',(2.27745358485296,1.,2.97921217251145));
#42392=CARTESIAN_POINT('Ctrl Pts',(2.27736742984319,-1.,2.97919987915679));
#42393=CARTESIAN_POINT('Ctrl Pts',(2.27736742984319,1.,2.97919987915679));
#42394=CARTESIAN_POINT('Ctrl Pts',(2.2773096118942,-1.,2.97929608861798));
#42395=CARTESIAN_POINT('Ctrl Pts',(2.2773096118942,1.,2.97929608861798));
#42396=CARTESIAN_POINT('Ctrl Pts',(2.27756633755188,-1.,2.97980276183181));
#42397=CARTESIAN_POINT('Ctrl Pts',(2.27756633755188,1.,2.97980276183181));
#42398=CARTESIAN_POINT('Ctrl Pts',(2.27859601334547,-1.,2.98120357932994));
#42399=CARTESIAN_POINT('Ctrl Pts',(2.27859601334547,1.,2.98120357932994));
#42400=CARTESIAN_POINT('Ctrl Pts',(2.28100472516679,-1.,2.98413343613983));
#42401=CARTESIAN_POINT('Ctrl Pts',(2.28100472516679,1.,2.98413343613983));
#42402=CARTESIAN_POINT('Ctrl Pts',(2.28446419115919,-1.,2.9881543273478));
#42403=CARTESIAN_POINT('Ctrl Pts',(2.28446419115919,1.,2.9881543273478));
#42404=CARTESIAN_POINT('Ctrl Pts',(2.28882328690362,-1.,2.99307930984034));
#42405=CARTESIAN_POINT('Ctrl Pts',(2.28882328690362,1.,2.99307930984034));
#42406=CARTESIAN_POINT('Ctrl Pts',(2.29385894577754,-1.,2.99863310339691));
#42407=CARTESIAN_POINT('Ctrl Pts',(2.29385894577754,1.,2.99863310339691));
#42408=CARTESIAN_POINT('Ctrl Pts',(2.29932091315775,-1.,3.00450832658613));
#42409=CARTESIAN_POINT('Ctrl Pts',(2.29932091315775,1.,3.00450832658613));
#42410=CARTESIAN_POINT('Ctrl Pts',(2.30496809486482,-1.,3.01041131063823));
#42411=CARTESIAN_POINT('Ctrl Pts',(2.30496809486482,1.,3.01041131063823));
#42412=CARTESIAN_POINT('Ctrl Pts',(2.31060449886629,-1.,3.01610726819086));
#42413=CARTESIAN_POINT('Ctrl Pts',(2.31060449886629,1.,3.01610726819086));
#42414=CARTESIAN_POINT('Ctrl Pts',(2.31612479121631,-1.,3.02147780668161));
#42415=CARTESIAN_POINT('Ctrl Pts',(2.31612479121631,1.,3.02147780668161));
#42416=CARTESIAN_POINT('Ctrl Pts',(2.32151944306402,-1.,3.02652678416611));
#42417=CARTESIAN_POINT('Ctrl Pts',(2.32151944306402,1.,3.02652678416611));
#42418=CARTESIAN_POINT('Ctrl Pts',(2.32683687412096,-1.,3.03133125185136));
#42419=CARTESIAN_POINT('Ctrl Pts',(2.32683687412096,1.,3.03133125185136));
#42420=CARTESIAN_POINT('Ctrl Pts',(2.33215619079829,-1.,3.03600588555793));
#42421=CARTESIAN_POINT('Ctrl Pts',(2.33215619079829,1.,3.03600588555793));
#42422=CARTESIAN_POINT('Ctrl Pts',(2.33755792953706,-1.,3.04066496998544));
#42423=CARTESIAN_POINT('Ctrl Pts',(2.33755792953706,1.,3.04066496998544));
#42424=CARTESIAN_POINT('Ctrl Pts',(2.34309017083976,-1.,3.04537822217256));
#42425=CARTESIAN_POINT('Ctrl Pts',(2.34309017083976,1.,3.04537822217256));
#42426=CARTESIAN_POINT('Ctrl Pts',(2.3487567309077,-1.,3.05015565829918));
#42427=CARTESIAN_POINT('Ctrl Pts',(2.3487567309077,1.,3.05015565829918));
#42428=CARTESIAN_POINT('Ctrl Pts',(2.35453559889474,-1.,3.05497218368146));
#42429=CARTESIAN_POINT('Ctrl Pts',(2.35453559889474,1.,3.05497218368146));
#42430=CARTESIAN_POINT('Ctrl Pts',(2.36039011602072,-1.,3.0597826624004));
#42431=CARTESIAN_POINT('Ctrl Pts',(2.36039011602072,1.,3.0597826624004));
#42432=CARTESIAN_POINT('Ctrl Pts',(2.36628220107009,-1.,3.06453964643162));
#42433=CARTESIAN_POINT('Ctrl Pts',(2.36628220107009,1.,3.06453964643162));
#42434=CARTESIAN_POINT('Ctrl Pts',(2.37218678163178,-1.,3.069212754975));
#42435=CARTESIAN_POINT('Ctrl Pts',(2.37218678163178,1.,3.069212754975));
#42436=CARTESIAN_POINT('Ctrl Pts',(2.37809856205548,-1.,3.07379777492165));
#42437=CARTESIAN_POINT('Ctrl Pts',(2.37809856205548,1.,3.07379777492165));
#42438=CARTESIAN_POINT('Ctrl Pts',(2.38402401216126,-1.,3.07830597244326));
#42439=CARTESIAN_POINT('Ctrl Pts',(2.38402401216126,1.,3.07830597244326));
#42440=CARTESIAN_POINT('Ctrl Pts',(2.38997659219199,-1.,3.08275773747093));
#42441=CARTESIAN_POINT('Ctrl Pts',(2.38997659219199,1.,3.08275773747093));
#42442=CARTESIAN_POINT('Ctrl Pts',(2.39597098250631,-1.,3.08717489512914));
#42443=CARTESIAN_POINT('Ctrl Pts',(2.39597098250631,1.,3.08717489512914));
#42444=CARTESIAN_POINT('Ctrl Pts',(2.40201704423341,-1.,3.091572660511));
#42445=CARTESIAN_POINT('Ctrl Pts',(2.40201704423341,1.,3.091572660511));
#42446=CARTESIAN_POINT('Ctrl Pts',(2.40811612696369,-1.,3.09595472616076));
#42447=CARTESIAN_POINT('Ctrl Pts',(2.40811612696369,1.,3.09595472616076));
#42448=CARTESIAN_POINT('Ctrl Pts',(2.41426441798057,-1.,3.1003177502767));
#42449=CARTESIAN_POINT('Ctrl Pts',(2.41426441798057,1.,3.1003177502767));
#42450=CARTESIAN_POINT('Ctrl Pts',(2.42045498612489,-1.,3.10465410280896));
#42451=CARTESIAN_POINT('Ctrl Pts',(2.42045498612489,1.,3.10465410280896));
#42452=CARTESIAN_POINT('Ctrl Pts',(2.42668025870015,-1.,3.10895518969595));
#42453=CARTESIAN_POINT('Ctrl Pts',(2.42668025870015,1.,3.10895518969595));
#42454=CARTESIAN_POINT('Ctrl Pts',(2.43293449685144,-1.,3.11321477659018));
#42455=CARTESIAN_POINT('Ctrl Pts',(2.43293449685144,1.,3.11321477659018));
#42456=CARTESIAN_POINT('Ctrl Pts',(2.43921571477977,-1.,3.11743156744186));
#42457=CARTESIAN_POINT('Ctrl Pts',(2.43921571477977,1.,3.11743156744186));
#42458=CARTESIAN_POINT('Ctrl Pts',(2.44552433364715,-1.,3.12160740887768));
#42459=CARTESIAN_POINT('Ctrl Pts',(2.44552433364715,1.,3.12160740887768));
#42460=CARTESIAN_POINT('Ctrl Pts',(2.45186227369846,-1.,3.12574608210847));
#42461=CARTESIAN_POINT('Ctrl Pts',(2.45186227369846,1.,3.12574608210847));
#42462=CARTESIAN_POINT('Ctrl Pts',(2.45823188859366,-1.,3.12985188384371));
#42463=CARTESIAN_POINT('Ctrl Pts',(2.45823188859366,1.,3.12985188384371));
#42464=CARTESIAN_POINT('Ctrl Pts',(2.46463494332374,-1.,3.13392826623906));
#42465=CARTESIAN_POINT('Ctrl Pts',(2.46463494332374,1.,3.13392826623906));
#42466=CARTESIAN_POINT('Ctrl Pts',(2.47107164236838,-1.,3.13797654408943));
#42467=CARTESIAN_POINT('Ctrl Pts',(2.47107164236838,1.,3.13797654408943));
#42468=CARTESIAN_POINT('Ctrl Pts',(2.47754112428043,-1.,3.14199655778863));
#42469=CARTESIAN_POINT('Ctrl Pts',(2.47754112428043,1.,3.14199655778863));
#42470=CARTESIAN_POINT('Ctrl Pts',(2.4840418741839,-1.,3.14598722723896));
#42471=CARTESIAN_POINT('Ctrl Pts',(2.4840418741839,1.,3.14598722723896));
#42472=CARTESIAN_POINT('Ctrl Pts',(2.49057217131988,-1.,3.14994715298907));
#42473=CARTESIAN_POINT('Ctrl Pts',(2.49057217131988,1.,3.14994715298907));
#42474=CARTESIAN_POINT('Ctrl Pts',(2.49713050858896,-1.,3.15387518039046));
#42475=CARTESIAN_POINT('Ctrl Pts',(2.49713050858896,1.,3.15387518039046));
#42476=CARTESIAN_POINT('Ctrl Pts',(2.50371605688252,-1.,3.15777102413957));
#42477=CARTESIAN_POINT('Ctrl Pts',(2.50371605688252,1.,3.15777102413957));
#42478=CARTESIAN_POINT('Ctrl Pts',(2.51032851007894,-1.,3.16163506380157));
#42479=CARTESIAN_POINT('Ctrl Pts',(2.51032851007894,1.,3.16163506380157));
#42480=CARTESIAN_POINT('Ctrl Pts',(2.51696788755577,-1.,3.16546808277023));
#42481=CARTESIAN_POINT('Ctrl Pts',(2.51696788755577,1.,3.16546808277023));
#42482=CARTESIAN_POINT('Ctrl Pts',(2.52363434671788,-1.,3.16927102130736));
#42483=CARTESIAN_POINT('Ctrl Pts',(2.52363434671788,1.,3.16927102130736));
#42484=CARTESIAN_POINT('Ctrl Pts',(2.53032800406941,-1.,3.17304474093612));
#42485=CARTESIAN_POINT('Ctrl Pts',(2.53032800406941,1.,3.17304474093612));
#42486=CARTESIAN_POINT('Ctrl Pts',(2.53704871950948,-1.,3.17678974135318));
#42487=CARTESIAN_POINT('Ctrl Pts',(2.53704871950948,1.,3.17678974135318));
#42488=CARTESIAN_POINT('Ctrl Pts',(2.5437961255305,-1.,3.1805061975064));
#42489=CARTESIAN_POINT('Ctrl Pts',(2.5437961255305,1.,3.1805061975064));
#42490=CARTESIAN_POINT('Ctrl Pts',(2.5505697238773,-1.,3.18419408529594));
#42491=CARTESIAN_POINT('Ctrl Pts',(2.5505697238773,1.,3.18419408529594));
#42492=CARTESIAN_POINT('Ctrl Pts',(2.55736896206056,-1.,3.18785328116218));
#42493=CARTESIAN_POINT('Ctrl Pts',(2.55736896206056,1.,3.18785328116218));
#42494=CARTESIAN_POINT('Ctrl Pts',(2.56419331092858,-1.,3.19148366395139));
#42495=CARTESIAN_POINT('Ctrl Pts',(2.56419331092858,1.,3.19148366395139));
#42496=CARTESIAN_POINT('Ctrl Pts',(2.57104235897899,-1.,3.19508523784363));
#42497=CARTESIAN_POINT('Ctrl Pts',(2.57104235897899,1.,3.19508523784363));
#42498=CARTESIAN_POINT('Ctrl Pts',(2.57791581908874,-1.,3.19865814628682));
#42499=CARTESIAN_POINT('Ctrl Pts',(2.57791581908874,1.,3.19865814628682));
#42500=CARTESIAN_POINT('Ctrl Pts',(2.58481347777728,-1.,3.20220261408414));
#42501=CARTESIAN_POINT('Ctrl Pts',(2.58481347777728,1.,3.20220261408414));
#42502=CARTESIAN_POINT('Ctrl Pts',(2.59173516023481,-1.,3.2057189102873));
#42503=CARTESIAN_POINT('Ctrl Pts',(2.59173516023481,1.,3.2057189102873));
#42504=CARTESIAN_POINT('Ctrl Pts',(2.59868069194341,-1.,3.20920730569681));
#42505=CARTESIAN_POINT('Ctrl Pts',(2.59868069194341,1.,3.20920730569681));
#42506=CARTESIAN_POINT('Ctrl Pts',(2.60564985360017,-1.,3.21266802609682));
#42507=CARTESIAN_POINT('Ctrl Pts',(2.60564985360017,1.,3.21266802609682));
#42508=CARTESIAN_POINT('Ctrl Pts',(2.61264236719171,-1.,3.21610123233082));
#42509=CARTESIAN_POINT('Ctrl Pts',(2.61264236719171,1.,3.21610123233082));
#42510=CARTESIAN_POINT('Ctrl Pts',(2.61965792832947,-1.,3.21950704109321));
#42511=CARTESIAN_POINT('Ctrl Pts',(2.61965792832947,1.,3.21950704109321));
#42512=CARTESIAN_POINT('Ctrl Pts',(2.62669622735912,-1.,3.2228855361324));
#42513=CARTESIAN_POINT('Ctrl Pts',(2.62669622735912,1.,3.2228855361324));
#42514=CARTESIAN_POINT('Ctrl Pts',(2.63375697391372,-1.,3.2262367829246));
#42515=CARTESIAN_POINT('Ctrl Pts',(2.63375697391372,1.,3.2262367829246));
#42516=CARTESIAN_POINT('Ctrl Pts',(2.64083992181823,-1.,3.22956084358547));
#42517=CARTESIAN_POINT('Ctrl Pts',(2.64083992181823,1.,3.22956084358547));
#42518=CARTESIAN_POINT('Ctrl Pts',(2.64794488743038,-1.,3.23285778737096));
#42519=CARTESIAN_POINT('Ctrl Pts',(2.64794488743038,1.,3.23285778737096));
#42520=CARTESIAN_POINT('Ctrl Pts',(2.65507173961555,-1.,3.236127680639));
#42521=CARTESIAN_POINT('Ctrl Pts',(2.65507173961555,1.,3.236127680639));
#42522=CARTESIAN_POINT('Ctrl Pts',(2.6607906631847,-1.,3.23872200034785));
#42523=CARTESIAN_POINT('Ctrl Pts',(2.6607906631847,1.,3.23872200034785));
#42524=CARTESIAN_POINT('Ctrl Pts',(2.66508964663997,-1.,3.24065561086749));
#42525=CARTESIAN_POINT('Ctrl Pts',(2.66508964663997,1.,3.24065561086749));
#42526=CARTESIAN_POINT('Ctrl Pts',(2.66795998539579,-1.,3.24193929584471));
#42527=CARTESIAN_POINT('Ctrl Pts',(2.66795998539579,1.,3.24193929584471));
#42528=CARTESIAN_POINT('Ctrl Pts',(2.66939624221984,-1.,3.24257979115744));
#42529=CARTESIAN_POINT('Ctrl Pts',(2.66939624221984,1.,3.24257979115744));
#42530=CARTESIAN_POINT('',(2.27737254473521,1.,2.97927412174279));
#42531=CARTESIAN_POINT('Ctrl Pts',(2.27737254473521,-1.,2.97927412174279));
#42532=CARTESIAN_POINT('Ctrl Pts',(2.27737254473521,-0.666666666666667,
2.97927412174279));
#42533=CARTESIAN_POINT('Ctrl Pts',(2.27737254473521,-0.333333333333333,
2.97927412174279));
#42534=CARTESIAN_POINT('Ctrl Pts',(2.27737254473521,0.333333333333333,2.97927412174279));
#42535=CARTESIAN_POINT('Ctrl Pts',(2.27737254473521,0.666666666666667,2.97927412174279));
#42536=CARTESIAN_POINT('Ctrl Pts',(2.27737254473521,1.,2.97927412174279));
#42537=CARTESIAN_POINT('',(2.66939624221984,1.,3.24257979115744));
#42538=CARTESIAN_POINT('',(2.66939624221984,0.,3.24257979115744));
#42539=CARTESIAN_POINT('Ctrl Pts',(2.27737254473521,1.,2.97927412174279));
#42540=CARTESIAN_POINT('Ctrl Pts',(2.27737238849287,1.,2.97932307137477));
#42541=CARTESIAN_POINT('Ctrl Pts',(2.27743009389684,1.,2.9795116710597));
#42542=CARTESIAN_POINT('Ctrl Pts',(2.27776738270289,1.,2.98007383024208));
#42543=CARTESIAN_POINT('Ctrl Pts',(2.27877674853766,1.,2.9814234180956));
#42544=CARTESIAN_POINT('Ctrl Pts',(2.28100472516679,1.,2.98413343613983));
#42545=CARTESIAN_POINT('Ctrl Pts',(2.28446419115919,1.,2.9881543273478));
#42546=CARTESIAN_POINT('Ctrl Pts',(2.28882328690362,1.,2.99307930984034));
#42547=CARTESIAN_POINT('Ctrl Pts',(2.29385894577754,1.,2.99863310339691));
#42548=CARTESIAN_POINT('Ctrl Pts',(2.29932091315775,1.,3.00450832658613));
#42549=CARTESIAN_POINT('Ctrl Pts',(2.30496809486482,1.,3.01041131063823));
#42550=CARTESIAN_POINT('Ctrl Pts',(2.31060449886629,1.,3.01610726819086));
#42551=CARTESIAN_POINT('Ctrl Pts',(2.31612479121631,1.,3.02147780668161));
#42552=CARTESIAN_POINT('Ctrl Pts',(2.32151944306402,1.,3.02652678416611));
#42553=CARTESIAN_POINT('Ctrl Pts',(2.32683687412096,1.,3.03133125185136));
#42554=CARTESIAN_POINT('Ctrl Pts',(2.33215619079829,1.,3.03600588555793));
#42555=CARTESIAN_POINT('Ctrl Pts',(2.33755792953706,1.,3.04066496998544));
#42556=CARTESIAN_POINT('Ctrl Pts',(2.34309017083976,1.,3.04537822217256));
#42557=CARTESIAN_POINT('Ctrl Pts',(2.3487567309077,1.,3.05015565829918));
#42558=CARTESIAN_POINT('Ctrl Pts',(2.35453559889474,1.,3.05497218368146));
#42559=CARTESIAN_POINT('Ctrl Pts',(2.36039011602072,1.,3.0597826624004));
#42560=CARTESIAN_POINT('Ctrl Pts',(2.36628220107009,1.,3.06453964643162));
#42561=CARTESIAN_POINT('Ctrl Pts',(2.37218678163178,1.,3.069212754975));
#42562=CARTESIAN_POINT('Ctrl Pts',(2.37809856205548,1.,3.07379777492165));
#42563=CARTESIAN_POINT('Ctrl Pts',(2.38402401216126,1.,3.07830597244326));
#42564=CARTESIAN_POINT('Ctrl Pts',(2.38997659219199,1.,3.08275773747093));
#42565=CARTESIAN_POINT('Ctrl Pts',(2.39597098250631,1.,3.08717489512914));
#42566=CARTESIAN_POINT('Ctrl Pts',(2.40201704423341,1.,3.091572660511));
#42567=CARTESIAN_POINT('Ctrl Pts',(2.40811612696369,1.,3.09595472616076));
#42568=CARTESIAN_POINT('Ctrl Pts',(2.41426441798057,1.,3.1003177502767));
#42569=CARTESIAN_POINT('Ctrl Pts',(2.42045498612489,1.,3.10465410280896));
#42570=CARTESIAN_POINT('Ctrl Pts',(2.42668025870015,1.,3.10895518969595));
#42571=CARTESIAN_POINT('Ctrl Pts',(2.43293449685144,1.,3.11321477659018));
#42572=CARTESIAN_POINT('Ctrl Pts',(2.43921571477977,1.,3.11743156744186));
#42573=CARTESIAN_POINT('Ctrl Pts',(2.44552433364715,1.,3.12160740887768));
#42574=CARTESIAN_POINT('Ctrl Pts',(2.45186227369846,1.,3.12574608210847));
#42575=CARTESIAN_POINT('Ctrl Pts',(2.45823188859366,1.,3.12985188384371));
#42576=CARTESIAN_POINT('Ctrl Pts',(2.46463494332374,1.,3.13392826623906));
#42577=CARTESIAN_POINT('Ctrl Pts',(2.47107164236838,1.,3.13797654408943));
#42578=CARTESIAN_POINT('Ctrl Pts',(2.47754112428043,1.,3.14199655778863));
#42579=CARTESIAN_POINT('Ctrl Pts',(2.4840418741839,1.,3.14598722723896));
#42580=CARTESIAN_POINT('Ctrl Pts',(2.49057217131988,1.,3.14994715298907));
#42581=CARTESIAN_POINT('Ctrl Pts',(2.49713050858896,1.,3.15387518039046));
#42582=CARTESIAN_POINT('Ctrl Pts',(2.50371605688252,1.,3.15777102413957));
#42583=CARTESIAN_POINT('Ctrl Pts',(2.51032851007894,1.,3.16163506380157));
#42584=CARTESIAN_POINT('Ctrl Pts',(2.51696788755577,1.,3.16546808277023));
#42585=CARTESIAN_POINT('Ctrl Pts',(2.52363434671788,1.,3.16927102130736));
#42586=CARTESIAN_POINT('Ctrl Pts',(2.53032800406941,1.,3.17304474093612));
#42587=CARTESIAN_POINT('Ctrl Pts',(2.53704871950948,1.,3.17678974135318));
#42588=CARTESIAN_POINT('Ctrl Pts',(2.5437961255305,1.,3.1805061975064));
#42589=CARTESIAN_POINT('Ctrl Pts',(2.5505697238773,1.,3.18419408529594));
#42590=CARTESIAN_POINT('Ctrl Pts',(2.55736896206056,1.,3.18785328116218));
#42591=CARTESIAN_POINT('Ctrl Pts',(2.56419331092858,1.,3.19148366395139));
#42592=CARTESIAN_POINT('Ctrl Pts',(2.57104235897899,1.,3.19508523784363));
#42593=CARTESIAN_POINT('Ctrl Pts',(2.57791581908874,1.,3.19865814628682));
#42594=CARTESIAN_POINT('Ctrl Pts',(2.58481347777728,1.,3.20220261408414));
#42595=CARTESIAN_POINT('Ctrl Pts',(2.59173516023481,1.,3.2057189102873));
#42596=CARTESIAN_POINT('Ctrl Pts',(2.59868069194341,1.,3.20920730569681));
#42597=CARTESIAN_POINT('Ctrl Pts',(2.60564985360017,1.,3.21266802609682));
#42598=CARTESIAN_POINT('Ctrl Pts',(2.61264236719171,1.,3.21610123233082));
#42599=CARTESIAN_POINT('Ctrl Pts',(2.61965792832947,1.,3.21950704109321));
#42600=CARTESIAN_POINT('Ctrl Pts',(2.62669622735912,1.,3.2228855361324));
#42601=CARTESIAN_POINT('Ctrl Pts',(2.63375697391372,1.,3.2262367829246));
#42602=CARTESIAN_POINT('Ctrl Pts',(2.64083992181823,1.,3.22956084358547));
#42603=CARTESIAN_POINT('Ctrl Pts',(2.64794488743038,1.,3.23285778737096));
#42604=CARTESIAN_POINT('Ctrl Pts',(2.65507173961555,1.,3.236127680639));
#42605=CARTESIAN_POINT('Ctrl Pts',(2.6607906631847,1.,3.23872200034785));
#42606=CARTESIAN_POINT('Ctrl Pts',(2.66508964663997,1.,3.24065561086749));
#42607=CARTESIAN_POINT('Ctrl Pts',(2.66795998539579,1.,3.24193929584471));
#42608=CARTESIAN_POINT('Ctrl Pts',(2.66939624221984,1.,3.24257979115744));
#42609=CARTESIAN_POINT('Origin',(2.66939624221984,0.,3.24257979115744));
#42610=CARTESIAN_POINT('',(2.78507268004355,1.,3.14378277984898));
#42611=CARTESIAN_POINT('Origin',(0.,0.,0.));
#42612=CARTESIAN_POINT('',(2.12971124846838,1.,3.08655633322109));
#42613=CARTESIAN_POINT('Origin',(0.,1.,0.));
#42614=CARTESIAN_POINT('Ctrl Pts',(2.12971124846838,1.,3.08655633322109));
#42615=CARTESIAN_POINT('Ctrl Pts',(2.12971124846838,0.666666666666667,3.08655633322109));
#42616=CARTESIAN_POINT('Ctrl Pts',(2.12971124846838,0.333333333333333,3.08655633322109));
#42617=CARTESIAN_POINT('Ctrl Pts',(2.12971124846838,-0.333333333333333,
3.08655633322109));
#42618=CARTESIAN_POINT('Ctrl Pts',(2.12971124846838,-0.666666666666667,
3.08655633322109));
#42619=CARTESIAN_POINT('Ctrl Pts',(2.12971124846838,-1.,3.08655633322109));
#42620=CARTESIAN_POINT('Ctrl Pts',(2.25898783642071,-1.,3.54075895182139));
#42621=CARTESIAN_POINT('Ctrl Pts',(2.25898783642071,1.,3.54075895182139));
#42622=CARTESIAN_POINT('Ctrl Pts',(2.25882251694918,-1.,3.5391950664771));
#42623=CARTESIAN_POINT('Ctrl Pts',(2.25882251694918,1.,3.5391950664771));
#42624=CARTESIAN_POINT('Ctrl Pts',(2.25848864344599,-1.,3.53606853163247));
#42625=CARTESIAN_POINT('Ctrl Pts',(2.25848864344599,1.,3.53606853163247));
#42626=CARTESIAN_POINT('Ctrl Pts',(2.25797812951166,-1.,3.53138243689932));
#42627=CARTESIAN_POINT('Ctrl Pts',(2.25797812951166,1.,3.53138243689932));
#42628=CARTESIAN_POINT('Ctrl Pts',(2.25727802942141,-1.,3.52514172849666));
#42629=CARTESIAN_POINT('Ctrl Pts',(2.25727802942141,1.,3.52514172849666));
#42630=CARTESIAN_POINT('Ctrl Pts',(2.25637049456061,-1.,3.51735323669213));
#42631=CARTESIAN_POINT('Ctrl Pts',(2.25637049456061,1.,3.51735323669213));
#42632=CARTESIAN_POINT('Ctrl Pts',(2.25543046980351,-1.,3.50957720118209));
#42633=CARTESIAN_POINT('Ctrl Pts',(2.25543046980351,1.,3.50957720118209));
#42634=CARTESIAN_POINT('Ctrl Pts',(2.25445785151923,-1.,3.50181372618058));
#42635=CARTESIAN_POINT('Ctrl Pts',(2.25445785151923,1.,3.50181372618058));
#42636=CARTESIAN_POINT('Ctrl Pts',(2.25345251709453,-1.,3.49406296494309));
#42637=CARTESIAN_POINT('Ctrl Pts',(2.25345251709453,1.,3.49406296494309));
#42638=CARTESIAN_POINT('Ctrl Pts',(2.25241433138231,-1.,3.48632513240231));
#42639=CARTESIAN_POINT('Ctrl Pts',(2.25241433138231,1.,3.48632513240231));
#42640=CARTESIAN_POINT('Ctrl Pts',(2.25134314238258,-1.,3.47860048448015));
#42641=CARTESIAN_POINT('Ctrl Pts',(2.25134314238258,1.,3.47860048448015));
#42642=CARTESIAN_POINT('Ctrl Pts',(2.25023877475674,-1.,3.47088928979467));
#42643=CARTESIAN_POINT('Ctrl Pts',(2.25023877475674,1.,3.47088928979467));
#42644=CARTESIAN_POINT('Ctrl Pts',(2.24910102345977,-1.,3.46319180177474));
#42645=CARTESIAN_POINT('Ctrl Pts',(2.24910102345977,1.,3.46319180177474));
#42646=CARTESIAN_POINT('Ctrl Pts',(2.24792964960874,-1.,3.45550823512213));
#42647=CARTESIAN_POINT('Ctrl Pts',(2.24792964960874,1.,3.45550823512213));
#42648=CARTESIAN_POINT('Ctrl Pts',(2.24672437070139,-1.,3.44783872863448));
#42649=CARTESIAN_POINT('Ctrl Pts',(2.24672437070139,1.,3.44783872863448));
#42650=CARTESIAN_POINT('Ctrl Pts',(2.24548487526212,-1.,3.44018336460619));
#42651=CARTESIAN_POINT('Ctrl Pts',(2.24548487526212,1.,3.44018336460619));
#42652=CARTESIAN_POINT('Ctrl Pts',(2.24421085338856,-1.,3.43254222615007));
#42653=CARTESIAN_POINT('Ctrl Pts',(2.24421085338856,1.,3.43254222615007));
#42654=CARTESIAN_POINT('Ctrl Pts',(2.24290202531144,-1.,3.42491544683075));
#42655=CARTESIAN_POINT('Ctrl Pts',(2.24290202531144,1.,3.42491544683075));
#42656=CARTESIAN_POINT('Ctrl Pts',(2.24155816587811,-1.,3.41730325539119));
#42657=CARTESIAN_POINT('Ctrl Pts',(2.24155816587811,1.,3.41730325539119));
#42658=CARTESIAN_POINT('Ctrl Pts',(2.24017914395211,-1.,3.40970604190205));
#42659=CARTESIAN_POINT('Ctrl Pts',(2.24017914395211,1.,3.40970604190205));
#42660=CARTESIAN_POINT('Ctrl Pts',(2.23876491124064,-1.,3.40212434705511));
#42661=CARTESIAN_POINT('Ctrl Pts',(2.23876491124064,1.,3.40212434705511));
#42662=CARTESIAN_POINT('Ctrl Pts',(2.23731541452726,-1.,3.39455873448088));
#42663=CARTESIAN_POINT('Ctrl Pts',(2.23731541452726,1.,3.39455873448088));
#42664=CARTESIAN_POINT('Ctrl Pts',(2.23583052276281,-1.,3.38700968549522));
#42665=CARTESIAN_POINT('Ctrl Pts',(2.23583052276281,1.,3.38700968549522));
#42666=CARTESIAN_POINT('Ctrl Pts',(2.23430995599572,-1.,3.37947749555649));
#42667=CARTESIAN_POINT('Ctrl Pts',(2.23430995599572,1.,3.37947749555649));
#42668=CARTESIAN_POINT('Ctrl Pts',(2.23275319569253,-1.,3.37196214349356));
#42669=CARTESIAN_POINT('Ctrl Pts',(2.23275319569253,1.,3.37196214349356));
#42670=CARTESIAN_POINT('Ctrl Pts',(2.23115945849777,-1.,3.36446325227908));
#42671=CARTESIAN_POINT('Ctrl Pts',(2.23115945849777,1.,3.36446325227908));
#42672=CARTESIAN_POINT('Ctrl Pts',(2.22952789881011,-1.,3.35698038165529));
#42673=CARTESIAN_POINT('Ctrl Pts',(2.22952789881011,1.,3.35698038165529));
#42674=CARTESIAN_POINT('Ctrl Pts',(2.22785777756588,-1.,3.34951327111117));
#42675=CARTESIAN_POINT('Ctrl Pts',(2.22785777756588,1.,3.34951327111117));
#42676=CARTESIAN_POINT('Ctrl Pts',(2.22614863918044,-1.,3.34206209449371));
#42677=CARTESIAN_POINT('Ctrl Pts',(2.22614863918044,1.,3.34206209449371));
#42678=CARTESIAN_POINT('Ctrl Pts',(2.224400498785,-1.,3.3346277284958));
#42679=CARTESIAN_POINT('Ctrl Pts',(2.224400498785,1.,3.3346277284958));
#42680=CARTESIAN_POINT('Ctrl Pts',(2.22261398879623,-1.,3.32721196326019));
#42681=CARTESIAN_POINT('Ctrl Pts',(2.22261398879623,1.,3.32721196326019));
#42682=CARTESIAN_POINT('Ctrl Pts',(2.22078990842768,-1.,3.31981686778008));
#42683=CARTESIAN_POINT('Ctrl Pts',(2.22078990842768,1.,3.31981686778008));
#42684=CARTESIAN_POINT('Ctrl Pts',(2.21892881679083,-1.,3.31244421655662));
#42685=CARTESIAN_POINT('Ctrl Pts',(2.21892881679083,1.,3.31244421655662));
#42686=CARTESIAN_POINT('Ctrl Pts',(2.21703059947837,-1.,3.3050948781957));
#42687=CARTESIAN_POINT('Ctrl Pts',(2.21703059947837,1.,3.3050948781957));
#42688=CARTESIAN_POINT('Ctrl Pts',(2.21509406923369,-1.,3.29776825193162));
#42689=CARTESIAN_POINT('Ctrl Pts',(2.21509406923369,1.,3.29776825193162));
#42690=CARTESIAN_POINT('Ctrl Pts',(2.2131164882739,-1.,3.29046159238344));
#42691=CARTESIAN_POINT('Ctrl Pts',(2.2131164882739,1.,3.29046159238344));
#42692=CARTESIAN_POINT('Ctrl Pts',(2.21109449750638,-1.,3.28317133333127));
#42693=CARTESIAN_POINT('Ctrl Pts',(2.21109449750638,1.,3.28317133333127));
#42694=CARTESIAN_POINT('Ctrl Pts',(2.20902509417425,-1.,3.27589448005534));
#42695=CARTESIAN_POINT('Ctrl Pts',(2.20902509417425,1.,3.27589448005534));
#42696=CARTESIAN_POINT('Ctrl Pts',(2.20690665217741,-1.,3.2686300613678));
#42697=CARTESIAN_POINT('Ctrl Pts',(2.20690665217741,1.,3.2686300613678));
#42698=CARTESIAN_POINT('Ctrl Pts',(2.20473979048682,-1.,3.26138036637711));
#42699=CARTESIAN_POINT('Ctrl Pts',(2.20473979048682,1.,3.26138036637711));
#42700=CARTESIAN_POINT('Ctrl Pts',(2.20252866491554,-1.,3.25415277957789));
#42701=CARTESIAN_POINT('Ctrl Pts',(2.20252866491554,1.,3.25415277957789));
#42702=CARTESIAN_POINT('Ctrl Pts',(2.20027910880993,-1.,3.24695715874356));
#42703=CARTESIAN_POINT('Ctrl Pts',(2.20027910880993,1.,3.24695715874356));
#42704=CARTESIAN_POINT('Ctrl Pts',(2.19799623693263,-1.,3.23980245361323));
#42705=CARTESIAN_POINT('Ctrl Pts',(2.19799623693263,1.,3.23980245361323));
#42706=CARTESIAN_POINT('Ctrl Pts',(2.19568204933172,-1.,3.23269332296938));
#42707=CARTESIAN_POINT('Ctrl Pts',(2.19568204933172,1.,3.23269332296938));
#42708=CARTESIAN_POINT('Ctrl Pts',(2.19333345123531,-1.,3.22562734221636));
#42709=CARTESIAN_POINT('Ctrl Pts',(2.19333345123531,1.,3.22562734221636));
#42710=CARTESIAN_POINT('Ctrl Pts',(2.1909390194865,-1.,3.21859043114069));
#42711=CARTESIAN_POINT('Ctrl Pts',(2.1909390194865,1.,3.21859043114069));
#42712=CARTESIAN_POINT('Ctrl Pts',(2.18848253363878,-1.,3.21156188355736));
#42713=CARTESIAN_POINT('Ctrl Pts',(2.18848253363878,1.,3.21156188355736));
#42714=CARTESIAN_POINT('Ctrl Pts',(2.18594876115914,-1.,3.20452259717947));
#42715=CARTESIAN_POINT('Ctrl Pts',(2.18594876115914,1.,3.20452259717947));
#42716=CARTESIAN_POINT('Ctrl Pts',(2.18332898656595,-1.,3.197462937404));
#42717=CARTESIAN_POINT('Ctrl Pts',(2.18332898656595,1.,3.197462937404));
#42718=CARTESIAN_POINT('Ctrl Pts',(2.18062558031789,-1.,3.19038924261589));
#42719=CARTESIAN_POINT('Ctrl Pts',(2.18062558031789,1.,3.19038924261589));
#42720=CARTESIAN_POINT('Ctrl Pts',(2.17785968847172,-1.,3.18333474627851));
#42721=CARTESIAN_POINT('Ctrl Pts',(2.17785968847172,1.,3.18333474627851));
#42722=CARTESIAN_POINT('Ctrl Pts',(2.17506466903736,-1.,3.17635032802584));
#42723=CARTESIAN_POINT('Ctrl Pts',(2.17506466903736,1.,3.17635032802584));
#42724=CARTESIAN_POINT('Ctrl Pts',(2.17227212063857,-1.,3.16948480019555));
#42725=CARTESIAN_POINT('Ctrl Pts',(2.17227212063857,1.,3.16948480019555));
#42726=CARTESIAN_POINT('Ctrl Pts',(2.16949910801237,-1.,3.16276685102999));
#42727=CARTESIAN_POINT('Ctrl Pts',(2.16949910801237,1.,3.16276685102999));
#42728=CARTESIAN_POINT('Ctrl Pts',(2.1667372844767,-1.,3.15618975593627));
#42729=CARTESIAN_POINT('Ctrl Pts',(2.1667372844767,1.,3.15618975593627));
#42730=CARTESIAN_POINT('Ctrl Pts',(2.16393520288009,-1.,3.14968624388961));
#42731=CARTESIAN_POINT('Ctrl Pts',(2.16393520288009,1.,3.14968624388961));
#42732=CARTESIAN_POINT('Ctrl Pts',(2.16100905914341,-1.,3.14314440426882));
#42733=CARTESIAN_POINT('Ctrl Pts',(2.16100905914341,1.,3.14314440426882));
#42734=CARTESIAN_POINT('Ctrl Pts',(2.15787423530583,-1.,3.136453565629));
#42735=CARTESIAN_POINT('Ctrl Pts',(2.15787423530583,1.,3.136453565629));
#42736=CARTESIAN_POINT('Ctrl Pts',(2.15447241382872,-1.,3.12954386795575));
#42737=CARTESIAN_POINT('Ctrl Pts',(2.15447241382872,1.,3.12954386795575));
#42738=CARTESIAN_POINT('Ctrl Pts',(2.15079698090627,-1.,3.12242318152001));
#42739=CARTESIAN_POINT('Ctrl Pts',(2.15079698090627,1.,3.12242318152001));
#42740=CARTESIAN_POINT('Ctrl Pts',(2.1469279845768,-1.,3.11522827017075));
#42741=CARTESIAN_POINT('Ctrl Pts',(2.1469279845768,1.,3.11522827017075));
#42742=CARTESIAN_POINT('Ctrl Pts',(2.14302815602195,-1.,3.10821808669189));
#42743=CARTESIAN_POINT('Ctrl Pts',(2.14302815602195,1.,3.10821808669189));
#42744=CARTESIAN_POINT('Ctrl Pts',(2.13930228863968,-1.,3.1017126739137));
#42745=CARTESIAN_POINT('Ctrl Pts',(2.13930228863968,1.,3.1017126739137));
#42746=CARTESIAN_POINT('Ctrl Pts',(2.13596538661154,-1.,3.09604502421197));
#42747=CARTESIAN_POINT('Ctrl Pts',(2.13596538661154,1.,3.09604502421197));
#42748=CARTESIAN_POINT('Ctrl Pts',(2.13321032560805,-1.,3.09151235281832));
#42749=CARTESIAN_POINT('Ctrl Pts',(2.13321032560805,1.,3.09151235281832));
#42750=CARTESIAN_POINT('Ctrl Pts',(2.13116819908263,-1.,3.08831615619661));
#42751=CARTESIAN_POINT('Ctrl Pts',(2.13116819908263,1.,3.08831615619661));
#42752=CARTESIAN_POINT('Ctrl Pts',(2.1301541297915,-1.,3.08690399991003));
#42753=CARTESIAN_POINT('Ctrl Pts',(2.1301541297915,1.,3.08690399991003));
#42754=CARTESIAN_POINT('Ctrl Pts',(2.12975158752197,-1.,3.08650326866821));
#42755=CARTESIAN_POINT('Ctrl Pts',(2.12975158752197,1.,3.08650326866821));
#42756=CARTESIAN_POINT('Ctrl Pts',(2.12964222015945,-1.,3.08652852644876));
#42757=CARTESIAN_POINT('Ctrl Pts',(2.12964222015945,1.,3.08652852644876));
#42758=CARTESIAN_POINT('Ctrl Pts',(2.12962728847314,-1.,3.08661426358891));
#42759=CARTESIAN_POINT('Ctrl Pts',(2.12962728847314,1.,3.08661426358891));
#42760=CARTESIAN_POINT('',(2.25898783642071,1.,3.54075895182139));
#42761=CARTESIAN_POINT('Ctrl Pts',(2.25898783642071,1.,3.54075895182139));
#42762=CARTESIAN_POINT('Ctrl Pts',(2.25882251694918,1.,3.5391950664771));
#42763=CARTESIAN_POINT('Ctrl Pts',(2.25848864344599,1.,3.53606853163247));
#42764=CARTESIAN_POINT('Ctrl Pts',(2.25797812951166,1.,3.53138243689932));
#42765=CARTESIAN_POINT('Ctrl Pts',(2.25727802942141,1.,3.52514172849666));
#42766=CARTESIAN_POINT('Ctrl Pts',(2.25637049456061,1.,3.51735323669213));
#42767=CARTESIAN_POINT('Ctrl Pts',(2.25543046980351,1.,3.50957720118209));
#42768=CARTESIAN_POINT('Ctrl Pts',(2.25445785151923,1.,3.50181372618058));
#42769=CARTESIAN_POINT('Ctrl Pts',(2.25345251709453,1.,3.49406296494309));
#42770=CARTESIAN_POINT('Ctrl Pts',(2.25241433138231,1.,3.48632513240231));
#42771=CARTESIAN_POINT('Ctrl Pts',(2.25134314238258,1.,3.47860048448015));
#42772=CARTESIAN_POINT('Ctrl Pts',(2.25023877475674,1.,3.47088928979467));
#42773=CARTESIAN_POINT('Ctrl Pts',(2.24910102345977,1.,3.46319180177474));
#42774=CARTESIAN_POINT('Ctrl Pts',(2.24792964960874,1.,3.45550823512213));
#42775=CARTESIAN_POINT('Ctrl Pts',(2.24672437070139,1.,3.44783872863448));
#42776=CARTESIAN_POINT('Ctrl Pts',(2.24548487526212,1.,3.44018336460619));
#42777=CARTESIAN_POINT('Ctrl Pts',(2.24421085338856,1.,3.43254222615007));
#42778=CARTESIAN_POINT('Ctrl Pts',(2.24290202531144,1.,3.42491544683075));
#42779=CARTESIAN_POINT('Ctrl Pts',(2.24155816587811,1.,3.41730325539119));
#42780=CARTESIAN_POINT('Ctrl Pts',(2.24017914395211,1.,3.40970604190205));
#42781=CARTESIAN_POINT('Ctrl Pts',(2.23876491124064,1.,3.40212434705511));
#42782=CARTESIAN_POINT('Ctrl Pts',(2.23731541452726,1.,3.39455873448088));
#42783=CARTESIAN_POINT('Ctrl Pts',(2.23583052276281,1.,3.38700968549522));
#42784=CARTESIAN_POINT('Ctrl Pts',(2.23430995599572,1.,3.37947749555649));
#42785=CARTESIAN_POINT('Ctrl Pts',(2.23275319569253,1.,3.37196214349356));
#42786=CARTESIAN_POINT('Ctrl Pts',(2.23115945849777,1.,3.36446325227908));
#42787=CARTESIAN_POINT('Ctrl Pts',(2.22952789881011,1.,3.35698038165529));
#42788=CARTESIAN_POINT('Ctrl Pts',(2.22785777756588,1.,3.34951327111117));
#42789=CARTESIAN_POINT('Ctrl Pts',(2.22614863918044,1.,3.34206209449371));
#42790=CARTESIAN_POINT('Ctrl Pts',(2.224400498785,1.,3.3346277284958));
#42791=CARTESIAN_POINT('Ctrl Pts',(2.22261398879623,1.,3.32721196326019));
#42792=CARTESIAN_POINT('Ctrl Pts',(2.22078990842768,1.,3.31981686778008));
#42793=CARTESIAN_POINT('Ctrl Pts',(2.21892881679083,1.,3.31244421655662));
#42794=CARTESIAN_POINT('Ctrl Pts',(2.21703059947837,1.,3.3050948781957));
#42795=CARTESIAN_POINT('Ctrl Pts',(2.21509406923369,1.,3.29776825193162));
#42796=CARTESIAN_POINT('Ctrl Pts',(2.2131164882739,1.,3.29046159238344));
#42797=CARTESIAN_POINT('Ctrl Pts',(2.21109449750638,1.,3.28317133333127));
#42798=CARTESIAN_POINT('Ctrl Pts',(2.20902509417425,1.,3.27589448005534));
#42799=CARTESIAN_POINT('Ctrl Pts',(2.20690665217741,1.,3.2686300613678));
#42800=CARTESIAN_POINT('Ctrl Pts',(2.20473979048682,1.,3.26138036637711));
#42801=CARTESIAN_POINT('Ctrl Pts',(2.20252866491554,1.,3.25415277957789));
#42802=CARTESIAN_POINT('Ctrl Pts',(2.20027910880993,1.,3.24695715874356));
#42803=CARTESIAN_POINT('Ctrl Pts',(2.19799623693263,1.,3.23980245361323));
#42804=CARTESIAN_POINT('Ctrl Pts',(2.19568204933172,1.,3.23269332296938));
#42805=CARTESIAN_POINT('Ctrl Pts',(2.19333345123531,1.,3.22562734221636));
#42806=CARTESIAN_POINT('Ctrl Pts',(2.1909390194865,1.,3.21859043114069));
#42807=CARTESIAN_POINT('Ctrl Pts',(2.18848253363878,1.,3.21156188355736));
#42808=CARTESIAN_POINT('Ctrl Pts',(2.18594876115914,1.,3.20452259717947));
#42809=CARTESIAN_POINT('Ctrl Pts',(2.18332898656595,1.,3.197462937404));
#42810=CARTESIAN_POINT('Ctrl Pts',(2.18062558031789,1.,3.19038924261589));
#42811=CARTESIAN_POINT('Ctrl Pts',(2.17785968847172,1.,3.18333474627851));
#42812=CARTESIAN_POINT('Ctrl Pts',(2.17506466903736,1.,3.17635032802584));
#42813=CARTESIAN_POINT('Ctrl Pts',(2.17227212063857,1.,3.16948480019555));
#42814=CARTESIAN_POINT('Ctrl Pts',(2.16949910801237,1.,3.16276685102999));
#42815=CARTESIAN_POINT('Ctrl Pts',(2.1667372844767,1.,3.15618975593627));
#42816=CARTESIAN_POINT('Ctrl Pts',(2.16393520288009,1.,3.14968624388961));
#42817=CARTESIAN_POINT('Ctrl Pts',(2.16100905914341,1.,3.14314440426882));
#42818=CARTESIAN_POINT('Ctrl Pts',(2.15787423530583,1.,3.136453565629));
#42819=CARTESIAN_POINT('Ctrl Pts',(2.15447241382872,1.,3.12954386795575));
#42820=CARTESIAN_POINT('Ctrl Pts',(2.15079698090627,1.,3.12242318152001));
#42821=CARTESIAN_POINT('Ctrl Pts',(2.1469279845768,1.,3.11522827017075));
#42822=CARTESIAN_POINT('Ctrl Pts',(2.14302815602195,1.,3.10821808669189));
#42823=CARTESIAN_POINT('Ctrl Pts',(2.13930228863968,1.,3.1017126739137));
#42824=CARTESIAN_POINT('Ctrl Pts',(2.13596538661154,1.,3.09604502421197));
#42825=CARTESIAN_POINT('Ctrl Pts',(2.13321032560805,1.,3.09151235281832));
#42826=CARTESIAN_POINT('Ctrl Pts',(2.13132142793056,1.,3.08855597949844));
#42827=CARTESIAN_POINT('Ctrl Pts',(2.13034980480519,1.,3.08717896996213));
#42828=CARTESIAN_POINT('Ctrl Pts',(2.12991938762497,1.,3.08668447250383));
#42829=CARTESIAN_POINT('Ctrl Pts',(2.1297578506162,1.,3.0865713108946));
#42830=CARTESIAN_POINT('Ctrl Pts',(2.12971124846838,1.,3.0865563332211));
#42831=CARTESIAN_POINT('',(2.25898783642071,0.,3.54075895182139));
#42832=CARTESIAN_POINT('Ctrl Pts',(1.7833628895577,-1.,3.2988053601491));
#42833=CARTESIAN_POINT('Ctrl Pts',(1.7833628895577,1.,3.2988053601491));
#42834=CARTESIAN_POINT('Ctrl Pts',(1.78327971836342,-1.,3.29877974053316));
#42835=CARTESIAN_POINT('Ctrl Pts',(1.78327971836342,1.,3.29877974053316));
#42836=CARTESIAN_POINT('Ctrl Pts',(1.78320756177373,-1.,3.29886572077632));
#42837=CARTESIAN_POINT('Ctrl Pts',(1.78320756177373,1.,3.29886572077632));
#42838=CARTESIAN_POINT('Ctrl Pts',(1.7833818655594,-1.,3.29940631674303));
#42839=CARTESIAN_POINT('Ctrl Pts',(1.7833818655594,1.,3.29940631674303));
#42840=CARTESIAN_POINT('Ctrl Pts',(1.78417972819938,-1.,3.30095096463517));
#42841=CARTESIAN_POINT('Ctrl Pts',(1.78417972819938,1.,3.30095096463517));
#42842=CARTESIAN_POINT('Ctrl Pts',(1.78610045419846,-1.,3.30422155559112));
#42843=CARTESIAN_POINT('Ctrl Pts',(1.78610045419846,1.,3.30422155559112));
#42844=CARTESIAN_POINT('Ctrl Pts',(1.78888832245873,-1.,3.30873412266788));
#42845=CARTESIAN_POINT('Ctrl Pts',(1.78888832245873,1.,3.30873412266788));
#42846=CARTESIAN_POINT('Ctrl Pts',(1.79242331349949,-1.,3.31428038326424));
#42847=CARTESIAN_POINT('Ctrl Pts',(1.79242331349949,1.,3.31428038326424));
#42848=CARTESIAN_POINT('Ctrl Pts',(1.79652817033251,-1.,3.3205535510082));
#42849=CARTESIAN_POINT('Ctrl Pts',(1.79652817033251,1.,3.3205535510082));
#42850=CARTESIAN_POINT('Ctrl Pts',(1.80100380443406,-1.,3.32721088039578));
#42851=CARTESIAN_POINT('Ctrl Pts',(1.80100380443406,1.,3.32721088039578));
#42852=CARTESIAN_POINT('Ctrl Pts',(1.80565802981102,-1.,3.33392460276808));
#42853=CARTESIAN_POINT('Ctrl Pts',(1.80565802981102,1.,3.33392460276808));
#42854=CARTESIAN_POINT('Ctrl Pts',(1.81033399625352,-1.,3.34043216147606));
#42855=CARTESIAN_POINT('Ctrl Pts',(1.81033399625352,1.,3.34043216147606));
#42856=CARTESIAN_POINT('Ctrl Pts',(1.81494618732853,-1.,3.34660014370673));
#42857=CARTESIAN_POINT('Ctrl Pts',(1.81494618732853,1.,3.34660014370673));
#42858=CARTESIAN_POINT('Ctrl Pts',(1.81948458796829,-1.,3.35243086937598));
#42859=CARTESIAN_POINT('Ctrl Pts',(1.81948458796829,1.,3.35243086937598));
#42860=CARTESIAN_POINT('Ctrl Pts',(1.82398496829301,-1.,3.35800801557424));
#42861=CARTESIAN_POINT('Ctrl Pts',(1.82398496829301,1.,3.35800801557424));
#42862=CARTESIAN_POINT('Ctrl Pts',(1.82850752153199,-1.,3.36345722124158));
#42863=CARTESIAN_POINT('Ctrl Pts',(1.82850752153199,1.,3.36345722124158));
#42864=CARTESIAN_POINT('Ctrl Pts',(1.83311391452322,-1.,3.36890396271836));
#42865=CARTESIAN_POINT('Ctrl Pts',(1.83311391452322,1.,3.36890396271836));
#42866=CARTESIAN_POINT('Ctrl Pts',(1.83784072967077,-1.,3.37442462015853));
#42867=CARTESIAN_POINT('Ctrl Pts',(1.83784072967077,1.,3.37442462015853));
#42868=CARTESIAN_POINT('Ctrl Pts',(1.84269016931643,-1.,3.38002968341157));
#42869=CARTESIAN_POINT('Ctrl Pts',(1.84269016931643,1.,3.38002968341157));
#42870=CARTESIAN_POINT('Ctrl Pts',(1.84764441927753,-1.,3.38569092349592));
#42871=CARTESIAN_POINT('Ctrl Pts',(1.84764441927753,1.,3.38569092349592));
#42872=CARTESIAN_POINT('Ctrl Pts',(1.85267433291769,-1.,3.39135802549398));
#42873=CARTESIAN_POINT('Ctrl Pts',(1.85267433291769,1.,3.39135802549398));
#42874=CARTESIAN_POINT('Ctrl Pts',(1.85774972037062,-1.,3.39697816833067));
#42875=CARTESIAN_POINT('Ctrl Pts',(1.85774972037062,1.,3.39697816833067));
#42876=CARTESIAN_POINT('Ctrl Pts',(1.86285057051245,-1.,3.40251742305476));
#42877=CARTESIAN_POINT('Ctrl Pts',(1.86285057051245,1.,3.40251742305476));
#42878=CARTESIAN_POINT('Ctrl Pts',(1.86797231196654,-1.,3.40797080000549));
#42879=CARTESIAN_POINT('Ctrl Pts',(1.86797231196654,1.,3.40797080000549));
#42880=CARTESIAN_POINT('Ctrl Pts',(1.87311957248121,-1.,3.41335043875209));
#42881=CARTESIAN_POINT('Ctrl Pts',(1.87311957248121,1.,3.41335043875209));
#42882=CARTESIAN_POINT('Ctrl Pts',(1.87830245689344,-1.,3.41867858383771));
#42883=CARTESIAN_POINT('Ctrl Pts',(1.87830245689344,1.,3.41867858383771));
#42884=CARTESIAN_POINT('Ctrl Pts',(1.8835320506206,-1.,3.42397908819736));
#42885=CARTESIAN_POINT('Ctrl Pts',(1.8835320506206,1.,3.42397908819736));
#42886=CARTESIAN_POINT('Ctrl Pts',(1.88881571322009,-1.,3.42926852222158));
#42887=CARTESIAN_POINT('Ctrl Pts',(1.88881571322009,1.,3.42926852222158));
#42888=CARTESIAN_POINT('Ctrl Pts',(1.89415420002542,-1.,3.43455074411571));
#42889=CARTESIAN_POINT('Ctrl Pts',(1.89415420002542,1.,3.43455074411571));
#42890=CARTESIAN_POINT('Ctrl Pts',(1.89954426803384,-1.,3.4398218567809));
#42891=CARTESIAN_POINT('Ctrl Pts',(1.89954426803384,1.,3.4398218567809));
#42892=CARTESIAN_POINT('Ctrl Pts',(1.90498026502304,-1.,3.44507323983368));
#42893=CARTESIAN_POINT('Ctrl Pts',(1.90498026502304,1.,3.44507323983368));
#42894=CARTESIAN_POINT('Ctrl Pts',(1.91045605593639,-1.,3.45029522038888));
#42895=CARTESIAN_POINT('Ctrl Pts',(1.91045605593639,1.,3.45029522038888));
#42896=CARTESIAN_POINT('Ctrl Pts',(1.91596694784063,-1.,3.4554807430995));
#42897=CARTESIAN_POINT('Ctrl Pts',(1.91596694784063,1.,3.4554807430995));
#42898=CARTESIAN_POINT('Ctrl Pts',(1.92151118213212,-1.,3.46062821722485));
#42899=CARTESIAN_POINT('Ctrl Pts',(1.92151118213212,1.,3.46062821722485));
#42900=CARTESIAN_POINT('Ctrl Pts',(1.92708888591158,-1.,3.46573953254084));
#42901=CARTESIAN_POINT('Ctrl Pts',(1.92708888591158,1.,3.46573953254084));
#42902=CARTESIAN_POINT('Ctrl Pts',(1.93270136427081,-1.,3.47081872409781));
#42903=CARTESIAN_POINT('Ctrl Pts',(1.93270136427081,1.,3.47081872409781));
#42904=CARTESIAN_POINT('Ctrl Pts',(1.93835026973887,-1.,3.47587040389915));
#42905=CARTESIAN_POINT('Ctrl Pts',(1.93835026973887,1.,3.47587040389915));
#42906=CARTESIAN_POINT('Ctrl Pts',(1.94403680554065,-1.,3.48089825770416));
#42907=CARTESIAN_POINT('Ctrl Pts',(1.94403680554065,1.,3.48089825770416));
#42908=CARTESIAN_POINT('Ctrl Pts',(1.94976096795911,-1.,3.48590361610814));
#42909=CARTESIAN_POINT('Ctrl Pts',(1.94976096795911,1.,3.48590361610814));
#42910=CARTESIAN_POINT('Ctrl Pts',(1.95552193112084,-1.,3.49088618670987));
#42911=CARTESIAN_POINT('Ctrl Pts',(1.95552193112084,1.,3.49088618670987));
#42912=CARTESIAN_POINT('Ctrl Pts',(1.961318367765,-1.,3.49584466573064));
#42913=CARTESIAN_POINT('Ctrl Pts',(1.961318367765,1.,3.49584466573064));
#42914=CARTESIAN_POINT('Ctrl Pts',(1.96714879724052,-1.,3.50077740176267));
#42915=CARTESIAN_POINT('Ctrl Pts',(1.96714879724052,1.,3.50077740176267));
#42916=CARTESIAN_POINT('Ctrl Pts',(1.97301191162968,-1.,3.5056830186108));
#42917=CARTESIAN_POINT('Ctrl Pts',(1.97301191162968,1.,3.5056830186108));
#42918=CARTESIAN_POINT('Ctrl Pts',(1.97890693666288,-1.,3.51056110478287));
#42919=CARTESIAN_POINT('Ctrl Pts',(1.97890693666288,1.,3.51056110478287));
#42920=CARTESIAN_POINT('Ctrl Pts',(1.9848335106103,-1.,3.51541198728301));
#42921=CARTESIAN_POINT('Ctrl Pts',(1.9848335106103,1.,3.51541198728301));
#42922=CARTESIAN_POINT('Ctrl Pts',(1.99079153006112,-1.,3.52023644289142));
#42923=CARTESIAN_POINT('Ctrl Pts',(1.99079153006112,1.,3.52023644289142));
#42924=CARTESIAN_POINT('Ctrl Pts',(1.99678100339295,-1.,3.52503542491728));
#42925=CARTESIAN_POINT('Ctrl Pts',(1.99678100339295,1.,3.52503542491728));
#42926=CARTESIAN_POINT('Ctrl Pts',(2.00280191090366,-1.,3.52980980250224));
#42927=CARTESIAN_POINT('Ctrl Pts',(2.00280191090366,1.,3.52980980250224));
#42928=CARTESIAN_POINT('Ctrl Pts',(2.00885403604746,-1.,3.53456004727424));
#42929=CARTESIAN_POINT('Ctrl Pts',(2.00885403604746,1.,3.53456004727424));
#42930=CARTESIAN_POINT('Ctrl Pts',(2.01493698847351,-1.,3.53928627453642));
#42931=CARTESIAN_POINT('Ctrl Pts',(2.01493698847351,1.,3.53928627453642));
#42932=CARTESIAN_POINT('Ctrl Pts',(2.02105027983104,-1.,3.54398838254136));
#42933=CARTESIAN_POINT('Ctrl Pts',(2.02105027983104,1.,3.54398838254136));
#42934=CARTESIAN_POINT('Ctrl Pts',(2.02719338376175,-1.,3.54866616282227));
#42935=CARTESIAN_POINT('Ctrl Pts',(2.02719338376175,1.,3.54866616282227));
#42936=CARTESIAN_POINT('Ctrl Pts',(2.03336579658133,-1.,3.55331941293949));
#42937=CARTESIAN_POINT('Ctrl Pts',(2.03336579658133,1.,3.55331941293949));
#42938=CARTESIAN_POINT('Ctrl Pts',(2.03956711119976,-1.,3.55794807264844));
#42939=CARTESIAN_POINT('Ctrl Pts',(2.03956711119976,1.,3.55794807264844));
#42940=CARTESIAN_POINT('Ctrl Pts',(2.04579702158876,-1.,3.56255223871505));
#42941=CARTESIAN_POINT('Ctrl Pts',(2.04579702158876,1.,3.56255223871505));
#42942=CARTESIAN_POINT('Ctrl Pts',(2.05205528172911,-1.,3.56713209977904));
#42943=CARTESIAN_POINT('Ctrl Pts',(2.05205528172911,1.,3.56713209977904));
#42944=CARTESIAN_POINT('Ctrl Pts',(2.05834167687425,-1.,3.5716878942334));
#42945=CARTESIAN_POINT('Ctrl Pts',(2.05834167687425,1.,3.5716878942334));
#42946=CARTESIAN_POINT('Ctrl Pts',(2.06465599229234,-1.,3.57621986224402));
#42947=CARTESIAN_POINT('Ctrl Pts',(2.06465599229234,1.,3.57621986224402));
#42948=CARTESIAN_POINT('Ctrl Pts',(2.07099797606,-1.,3.58072819250872));
#42949=CARTESIAN_POINT('Ctrl Pts',(2.07099797606,1.,3.58072819250872));
#42950=CARTESIAN_POINT('Ctrl Pts',(2.07736732842524,-1.,3.58521300039988));
#42951=CARTESIAN_POINT('Ctrl Pts',(2.07736732842524,1.,3.58521300039988));
#42952=CARTESIAN_POINT('Ctrl Pts',(2.08376373049196,-1.,3.58967435355834));
#42953=CARTESIAN_POINT('Ctrl Pts',(2.08376373049196,1.,3.58967435355834));
#42954=CARTESIAN_POINT('Ctrl Pts',(2.09018686331706,-1.,3.5941122862608));
#42955=CARTESIAN_POINT('Ctrl Pts',(2.09018686331706,1.,3.5941122862608));
#42956=CARTESIAN_POINT('Ctrl Pts',(2.09663642986579,-1.,3.59852681775396));
#42957=CARTESIAN_POINT('Ctrl Pts',(2.09663642986579,1.,3.59852681775396));
#42958=CARTESIAN_POINT('Ctrl Pts',(2.10311217727687,-1.,3.60291797087849));
#42959=CARTESIAN_POINT('Ctrl Pts',(2.10311217727687,1.,3.60291797087849));
#42960=CARTESIAN_POINT('Ctrl Pts',(2.10961391333497,-1.,3.60728578530968));
#42961=CARTESIAN_POINT('Ctrl Pts',(2.10961391333497,1.,3.60728578530968));
#42962=CARTESIAN_POINT('Ctrl Pts',(2.11614149813928,-1.,3.61163030607452));
#42963=CARTESIAN_POINT('Ctrl Pts',(2.11614149813928,1.,3.61163030607452));
#42964=CARTESIAN_POINT('Ctrl Pts',(2.12138417125349,-1.,3.61508732215187));
#42965=CARTESIAN_POINT('Ctrl Pts',(2.12138417125349,1.,3.61508732215187));
#42966=CARTESIAN_POINT('Ctrl Pts',(2.12532774376144,-1.,3.61766963589442));
#42967=CARTESIAN_POINT('Ctrl Pts',(2.12532774376144,1.,3.61766963589442));
#42968=CARTESIAN_POINT('Ctrl Pts',(2.12796193131142,-1.,3.61938653648716));
#42969=CARTESIAN_POINT('Ctrl Pts',(2.12796193131142,1.,3.61938653648716));
#42970=CARTESIAN_POINT('Ctrl Pts',(2.12928030988903,-1.,3.62024382630768));
#42971=CARTESIAN_POINT('Ctrl Pts',(2.12928030988903,1.,3.62024382630768));
#42972=CARTESIAN_POINT('',(1.78327315618341,1.,3.29885386921513));
#42973=CARTESIAN_POINT('Ctrl Pts',(1.78327315618341,-1.,3.29885386921514));
#42974=CARTESIAN_POINT('Ctrl Pts',(1.78327315618341,-0.666666666666667,
3.29885386921514));
#42975=CARTESIAN_POINT('Ctrl Pts',(1.78327315618341,-0.333333333333333,
3.29885386921514));
#42976=CARTESIAN_POINT('Ctrl Pts',(1.78327315618341,0.333333333333333,3.29885386921514));
#42977=CARTESIAN_POINT('Ctrl Pts',(1.78327315618341,0.666666666666667,3.29885386921513));
#42978=CARTESIAN_POINT('Ctrl Pts',(1.78327315618341,1.,3.29885386921513));
#42979=CARTESIAN_POINT('',(2.12928030988903,1.,3.62024382630768));
#42980=CARTESIAN_POINT('',(2.12928030988903,0.,3.62024382630768));
#42981=CARTESIAN_POINT('Ctrl Pts',(1.78327315618341,1.,3.29885386921513));
#42982=CARTESIAN_POINT('Ctrl Pts',(1.78326534445518,1.,3.29890219175423));
#42983=CARTESIAN_POINT('Ctrl Pts',(1.78329283591905,1.,3.29909749657808));
#42984=CARTESIAN_POINT('Ctrl Pts',(1.78353803106924,1.,3.299705498242));
#42985=CARTESIAN_POINT('Ctrl Pts',(1.78432384788174,1.,3.30119637003393));
#42986=CARTESIAN_POINT('Ctrl Pts',(1.78610045419846,1.,3.30422155559112));
#42987=CARTESIAN_POINT('Ctrl Pts',(1.78888832245873,1.,3.30873412266788));
#42988=CARTESIAN_POINT('Ctrl Pts',(1.79242331349949,1.,3.31428038326424));
#42989=CARTESIAN_POINT('Ctrl Pts',(1.79652817033251,1.,3.3205535510082));
#42990=CARTESIAN_POINT('Ctrl Pts',(1.80100380443406,1.,3.32721088039578));
#42991=CARTESIAN_POINT('Ctrl Pts',(1.80565802981102,1.,3.33392460276808));
#42992=CARTESIAN_POINT('Ctrl Pts',(1.81033399625352,1.,3.34043216147606));
#42993=CARTESIAN_POINT('Ctrl Pts',(1.81494618732853,1.,3.34660014370673));
#42994=CARTESIAN_POINT('Ctrl Pts',(1.81948458796829,1.,3.35243086937598));
#42995=CARTESIAN_POINT('Ctrl Pts',(1.82398496829301,1.,3.35800801557424));
#42996=CARTESIAN_POINT('Ctrl Pts',(1.82850752153199,1.,3.36345722124158));
#42997=CARTESIAN_POINT('Ctrl Pts',(1.83311391452322,1.,3.36890396271836));
#42998=CARTESIAN_POINT('Ctrl Pts',(1.83784072967077,1.,3.37442462015853));
#42999=CARTESIAN_POINT('Ctrl Pts',(1.84269016931643,1.,3.38002968341157));
#43000=CARTESIAN_POINT('Ctrl Pts',(1.84764441927753,1.,3.38569092349592));
#43001=CARTESIAN_POINT('Ctrl Pts',(1.85267433291769,1.,3.39135802549398));
#43002=CARTESIAN_POINT('Ctrl Pts',(1.85774972037062,1.,3.39697816833067));
#43003=CARTESIAN_POINT('Ctrl Pts',(1.86285057051245,1.,3.40251742305476));
#43004=CARTESIAN_POINT('Ctrl Pts',(1.86797231196654,1.,3.40797080000549));
#43005=CARTESIAN_POINT('Ctrl Pts',(1.87311957248121,1.,3.41335043875209));
#43006=CARTESIAN_POINT('Ctrl Pts',(1.87830245689344,1.,3.41867858383771));
#43007=CARTESIAN_POINT('Ctrl Pts',(1.8835320506206,1.,3.42397908819736));
#43008=CARTESIAN_POINT('Ctrl Pts',(1.88881571322009,1.,3.42926852222158));
#43009=CARTESIAN_POINT('Ctrl Pts',(1.89415420002542,1.,3.43455074411571));
#43010=CARTESIAN_POINT('Ctrl Pts',(1.89954426803384,1.,3.4398218567809));
#43011=CARTESIAN_POINT('Ctrl Pts',(1.90498026502304,1.,3.44507323983368));
#43012=CARTESIAN_POINT('Ctrl Pts',(1.91045605593639,1.,3.45029522038888));
#43013=CARTESIAN_POINT('Ctrl Pts',(1.91596694784063,1.,3.4554807430995));
#43014=CARTESIAN_POINT('Ctrl Pts',(1.92151118213212,1.,3.46062821722485));
#43015=CARTESIAN_POINT('Ctrl Pts',(1.92708888591158,1.,3.46573953254084));
#43016=CARTESIAN_POINT('Ctrl Pts',(1.93270136427081,1.,3.47081872409781));
#43017=CARTESIAN_POINT('Ctrl Pts',(1.93835026973887,1.,3.47587040389915));
#43018=CARTESIAN_POINT('Ctrl Pts',(1.94403680554065,1.,3.48089825770416));
#43019=CARTESIAN_POINT('Ctrl Pts',(1.94976096795911,1.,3.48590361610814));
#43020=CARTESIAN_POINT('Ctrl Pts',(1.95552193112084,1.,3.49088618670987));
#43021=CARTESIAN_POINT('Ctrl Pts',(1.961318367765,1.,3.49584466573064));
#43022=CARTESIAN_POINT('Ctrl Pts',(1.96714879724052,1.,3.50077740176267));
#43023=CARTESIAN_POINT('Ctrl Pts',(1.97301191162968,1.,3.5056830186108));
#43024=CARTESIAN_POINT('Ctrl Pts',(1.97890693666288,1.,3.51056110478287));
#43025=CARTESIAN_POINT('Ctrl Pts',(1.9848335106103,1.,3.51541198728301));
#43026=CARTESIAN_POINT('Ctrl Pts',(1.99079153006112,1.,3.52023644289142));
#43027=CARTESIAN_POINT('Ctrl Pts',(1.99678100339295,1.,3.52503542491728));
#43028=CARTESIAN_POINT('Ctrl Pts',(2.00280191090366,1.,3.52980980250224));
#43029=CARTESIAN_POINT('Ctrl Pts',(2.00885403604746,1.,3.53456004727424));
#43030=CARTESIAN_POINT('Ctrl Pts',(2.01493698847351,1.,3.53928627453642));
#43031=CARTESIAN_POINT('Ctrl Pts',(2.02105027983104,1.,3.54398838254136));
#43032=CARTESIAN_POINT('Ctrl Pts',(2.02719338376175,1.,3.54866616282227));
#43033=CARTESIAN_POINT('Ctrl Pts',(2.03336579658133,1.,3.55331941293949));
#43034=CARTESIAN_POINT('Ctrl Pts',(2.03956711119976,1.,3.55794807264844));
#43035=CARTESIAN_POINT('Ctrl Pts',(2.04579702158876,1.,3.56255223871505));
#43036=CARTESIAN_POINT('Ctrl Pts',(2.05205528172911,1.,3.56713209977904));
#43037=CARTESIAN_POINT('Ctrl Pts',(2.05834167687425,1.,3.5716878942334));
#43038=CARTESIAN_POINT('Ctrl Pts',(2.06465599229234,1.,3.57621986224402));
#43039=CARTESIAN_POINT('Ctrl Pts',(2.07099797606,1.,3.58072819250872));
#43040=CARTESIAN_POINT('Ctrl Pts',(2.07736732842524,1.,3.58521300039988));
#43041=CARTESIAN_POINT('Ctrl Pts',(2.08376373049196,1.,3.58967435355834));
#43042=CARTESIAN_POINT('Ctrl Pts',(2.09018686331706,1.,3.5941122862608));
#43043=CARTESIAN_POINT('Ctrl Pts',(2.09663642986579,1.,3.59852681775396));
#43044=CARTESIAN_POINT('Ctrl Pts',(2.10311217727687,1.,3.60291797087849));
#43045=CARTESIAN_POINT('Ctrl Pts',(2.10961391333497,1.,3.60728578530968));
#43046=CARTESIAN_POINT('Ctrl Pts',(2.11614149813928,1.,3.61163030607452));
#43047=CARTESIAN_POINT('Ctrl Pts',(2.12138417125349,1.,3.61508732215187));
#43048=CARTESIAN_POINT('Ctrl Pts',(2.12532774376144,1.,3.61766963589442));
#43049=CARTESIAN_POINT('Ctrl Pts',(2.12796193131142,1.,3.61938653648716));
#43050=CARTESIAN_POINT('Ctrl Pts',(2.12928030988903,1.,3.62024382630768));
#43051=CARTESIAN_POINT('Origin',(2.12928030988903,0.,3.62024382630768));
#43052=CARTESIAN_POINT('',(2.25898783642071,1.,3.54075895182139));
#43053=CARTESIAN_POINT('Origin',(0.,0.,0.));
#43054=CARTESIAN_POINT('',(1.62064718014256,1.,3.38171594275687));
#43055=CARTESIAN_POINT('Origin',(0.,1.,0.));
#43056=CARTESIAN_POINT('Ctrl Pts',(1.62064718014256,1.,3.38171594275687));
#43057=CARTESIAN_POINT('Ctrl Pts',(1.62064718014256,0.666666666666667,3.38171594275687));
#43058=CARTESIAN_POINT('Ctrl Pts',(1.62064718014256,0.333333333333333,3.38171594275687));
#43059=CARTESIAN_POINT('Ctrl Pts',(1.62064718014256,-0.333333333333333,
3.38171594275687));
#43060=CARTESIAN_POINT('Ctrl Pts',(1.62064718014256,-0.666666666666667,
3.38171594275687));
#43061=CARTESIAN_POINT('Ctrl Pts',(1.62064718014256,-1.,3.38171594275687));
#43062=CARTESIAN_POINT('Ctrl Pts',(1.67727921511438,-1.,3.85054988729471));
#43063=CARTESIAN_POINT('Ctrl Pts',(1.67727921511438,1.,3.85054988729471));
#43064=CARTESIAN_POINT('Ctrl Pts',(1.6773605765671,-1.,3.84897939431104));
#43065=CARTESIAN_POINT('Ctrl Pts',(1.6773605765671,1.,3.84897939431104));
#43066=CARTESIAN_POINT('Ctrl Pts',(1.67751991140661,-1.,3.84583912297567));
#43067=CARTESIAN_POINT('Ctrl Pts',(1.67751991140661,1.,3.84583912297567));
#43068=CARTESIAN_POINT('Ctrl Pts',(1.67774874946867,-1.,3.8411308598706));
#43069=CARTESIAN_POINT('Ctrl Pts',(1.67774874946867,1.,3.8411308598706));
#43070=CARTESIAN_POINT('Ctrl Pts',(1.67803353065273,-1.,3.83485746516115));
#43071=CARTESIAN_POINT('Ctrl Pts',(1.67803353065273,1.,3.83485746516115));
#43072=CARTESIAN_POINT('Ctrl Pts',(1.67835555760094,-1.,3.82702289288453));
#43073=CARTESIAN_POINT('Ctrl Pts',(1.67835555760094,1.,3.82702289288453));
#43074=CARTESIAN_POINT('Ctrl Pts',(1.67864354606363,-1.,3.81919554100522));
#43075=CARTESIAN_POINT('Ctrl Pts',(1.67864354606363,1.,3.81919554100522));
#43076=CARTESIAN_POINT('Ctrl Pts',(1.67889737738311,-1.,3.81137549624273));
#43077=CARTESIAN_POINT('Ctrl Pts',(1.67889737738311,1.,3.81137549624273));
#43078=CARTESIAN_POINT('Ctrl Pts',(1.67911690648128,-1.,3.80356289078481));
#43079=CARTESIAN_POINT('Ctrl Pts',(1.67911690648128,1.,3.80356289078481));
#43080=CARTESIAN_POINT('Ctrl Pts',(1.67930196625203,-1.,3.7957579157763));
#43081=CARTESIAN_POINT('Ctrl Pts',(1.67930196625203,1.,3.7957579157763));
#43082=CARTESIAN_POINT('Ctrl Pts',(1.67945236653175,-1.,3.78796080021026));
#43083=CARTESIAN_POINT('Ctrl Pts',(1.67945236653175,1.,3.78796080021026));
#43084=CARTESIAN_POINT('Ctrl Pts',(1.67956789211943,-1.,3.78017178196859));
#43085=CARTESIAN_POINT('Ctrl Pts',(1.67956789211943,1.,3.78017178196859));
#43086=CARTESIAN_POINT('Ctrl Pts',(1.67964830084946,-1.,3.77239107928394));
#43087=CARTESIAN_POINT('Ctrl Pts',(1.67964830084946,1.,3.77239107928394));
#43088=CARTESIAN_POINT('Ctrl Pts',(1.67969332319322,-1.,3.76461886684523));
#43089=CARTESIAN_POINT('Ctrl Pts',(1.67969332319322,1.,3.76461886684523));
#43090=CARTESIAN_POINT('Ctrl Pts',(1.67970265841379,-1.,3.75685523754816));
#43091=CARTESIAN_POINT('Ctrl Pts',(1.67970265841379,1.,3.75685523754816));
#43092=CARTESIAN_POINT('Ctrl Pts',(1.67967598599665,-1.,3.74910022394845));
#43093=CARTESIAN_POINT('Ctrl Pts',(1.67967598599665,1.,3.74910022394845));
#43094=CARTESIAN_POINT('Ctrl Pts',(1.67961298685316,-1.,3.74135385965622));
#43095=CARTESIAN_POINT('Ctrl Pts',(1.67961298685316,1.,3.74135385965622));
#43096=CARTESIAN_POINT('Ctrl Pts',(1.67951336376434,-1.,3.73361623282617));
#43097=CARTESIAN_POINT('Ctrl Pts',(1.67951336376434,1.,3.73361623282617));
#43098=CARTESIAN_POINT('Ctrl Pts',(1.67937685856627,-1.,3.72588753416339));
#43099=CARTESIAN_POINT('Ctrl Pts',(1.67937685856627,1.,3.72588753416339));
#43100=CARTESIAN_POINT('Ctrl Pts',(1.6792032807165,-1.,3.71816812842188));
#43101=CARTESIAN_POINT('Ctrl Pts',(1.6792032807165,1.,3.71816812842188));
#43102=CARTESIAN_POINT('Ctrl Pts',(1.67899249793398,-1.,3.71045854208195));
#43103=CARTESIAN_POINT('Ctrl Pts',(1.67899249793398,1.,3.71045854208195));
#43104=CARTESIAN_POINT('Ctrl Pts',(1.6787443694862,-1.,3.70275932350998));
#43105=CARTESIAN_POINT('Ctrl Pts',(1.6787443694862,1.,3.70275932350998));
#43106=CARTESIAN_POINT('Ctrl Pts',(1.67845869064304,-1.,3.69507092759545));
#43107=CARTESIAN_POINT('Ctrl Pts',(1.67845869064304,1.,3.69507092759545));
#43108=CARTESIAN_POINT('Ctrl Pts',(1.67813513867973,-1.,3.68739360236505));
#43109=CARTESIAN_POINT('Ctrl Pts',(1.67813513867973,1.,3.68739360236505));
#43110=CARTESIAN_POINT('Ctrl Pts',(1.67777320475872,-1.,3.6797272457918));
#43111=CARTESIAN_POINT('Ctrl Pts',(1.67777320475872,1.,3.6797272457918));
#43112=CARTESIAN_POINT('Ctrl Pts',(1.67737217414901,-1.,3.67207136294639));
#43113=CARTESIAN_POINT('Ctrl Pts',(1.67737217414901,1.,3.67207136294639));
#43114=CARTESIAN_POINT('Ctrl Pts',(1.67693128053153,-1.,3.66442538671018));
#43115=CARTESIAN_POINT('Ctrl Pts',(1.67693128053153,1.,3.66442538671018));
#43116=CARTESIAN_POINT('Ctrl Pts',(1.67644983469459,-1.,3.65678894416442));
#43117=CARTESIAN_POINT('Ctrl Pts',(1.67644983469459,1.,3.65678894416442));
#43118=CARTESIAN_POINT('Ctrl Pts',(1.6759273594669,-1.,3.64916213574663));
#43119=CARTESIAN_POINT('Ctrl Pts',(1.6759273594669,1.,3.64916213574663));
#43120=CARTESIAN_POINT('Ctrl Pts',(1.67536373264839,-1.,3.6415458297232));
#43121=CARTESIAN_POINT('Ctrl Pts',(1.67536373264839,1.,3.6415458297232));
#43122=CARTESIAN_POINT('Ctrl Pts',(1.67475929882962,-1.,3.63394189312902));
#43123=CARTESIAN_POINT('Ctrl Pts',(1.67475929882962,1.,3.63394189312902));
#43124=CARTESIAN_POINT('Ctrl Pts',(1.67411452372265,-1.,3.62635249450908));
#43125=CARTESIAN_POINT('Ctrl Pts',(1.67411452372265,1.,3.62635249450908));
#43126=CARTESIAN_POINT('Ctrl Pts',(1.67342968196223,-1.,3.61877947398179));
#43127=CARTESIAN_POINT('Ctrl Pts',(1.67342968196223,1.,3.61877947398179));
#43128=CARTESIAN_POINT('Ctrl Pts',(1.67270452466968,-1.,3.61122367156182));
#43129=CARTESIAN_POINT('Ctrl Pts',(1.67270452466968,1.,3.61122367156182));
#43130=CARTESIAN_POINT('Ctrl Pts',(1.67193797318598,-1.,3.60368430815203));
#43131=CARTESIAN_POINT('Ctrl Pts',(1.67193797318598,1.,3.60368430815203));
#43132=CARTESIAN_POINT('Ctrl Pts',(1.67112775290706,-1.,3.59615824388808));
#43133=CARTESIAN_POINT('Ctrl Pts',(1.67112775290706,1.,3.59615824388808));
#43134=CARTESIAN_POINT('Ctrl Pts',(1.67027110397601,-1.,3.5886414309783));
#43135=CARTESIAN_POINT('Ctrl Pts',(1.67027110397601,1.,3.5886414309783));
#43136=CARTESIAN_POINT('Ctrl Pts',(1.66936552908228,-1.,3.58113044183823));
#43137=CARTESIAN_POINT('Ctrl Pts',(1.66936552908228,1.,3.58113044183823));
#43138=CARTESIAN_POINT('Ctrl Pts',(1.66840957407299,-1.,3.57362406285884));
#43139=CARTESIAN_POINT('Ctrl Pts',(1.66840957407299,1.,3.57362406285884));
#43140=CARTESIAN_POINT('Ctrl Pts',(1.66740349220308,-1.,3.56612465179429));
#43141=CARTESIAN_POINT('Ctrl Pts',(1.66740349220308,1.,3.56612465179429));
#43142=CARTESIAN_POINT('Ctrl Pts',(1.66635023293121,-1.,3.55864015233617));
#43143=CARTESIAN_POINT('Ctrl Pts',(1.66635023293121,1.,3.55864015233617));
#43144=CARTESIAN_POINT('Ctrl Pts',(1.66525401569004,-1.,3.5511812134288));
#43145=CARTESIAN_POINT('Ctrl Pts',(1.66525401569004,1.,3.5511812134288));
#43146=CARTESIAN_POINT('Ctrl Pts',(1.66411849222334,-1.,3.5437574747503));
#43147=CARTESIAN_POINT('Ctrl Pts',(1.66411849222334,1.,3.5437574747503));
#43148=CARTESIAN_POINT('Ctrl Pts',(1.66294490916113,-1.,3.53637385060225));
#43149=CARTESIAN_POINT('Ctrl Pts',(1.66294490916113,1.,3.53637385060225));
#43150=CARTESIAN_POINT('Ctrl Pts',(1.66173058912365,-1.,3.52902746211082));
#43151=CARTESIAN_POINT('Ctrl Pts',(1.66173058912365,1.,3.52902746211082));
#43152=CARTESIAN_POINT('Ctrl Pts',(1.66046645222266,-1.,3.52170261543787));
#43153=CARTESIAN_POINT('Ctrl Pts',(1.66046645222266,1.,3.52170261543787));
#43154=CARTESIAN_POINT('Ctrl Pts',(1.65913971687324,-1.,3.51437632188903));
#43155=CARTESIAN_POINT('Ctrl Pts',(1.65913971687324,1.,3.51437632188903));
#43156=CARTESIAN_POINT('Ctrl Pts',(1.65773832633617,-1.,3.5070273314651));
#43157=CARTESIAN_POINT('Ctrl Pts',(1.65773832633617,1.,3.5070273314651));
#43158=CARTESIAN_POINT('Ctrl Pts',(1.65625517961583,-1.,3.49964476477929));
#43159=CARTESIAN_POINT('Ctrl Pts',(1.65625517961583,1.,3.49964476477929));
#43160=CARTESIAN_POINT('Ctrl Pts',(1.65469162644476,-1.,3.49223525300194));
#43161=CARTESIAN_POINT('Ctrl Pts',(1.65469162644476,1.,3.49223525300194));
#43162=CARTESIAN_POINT('Ctrl Pts',(1.65306335367762,-1.,3.48483492840942));
#43163=CARTESIAN_POINT('Ctrl Pts',(1.65306335367762,1.,3.48483492840942));
#43164=CARTESIAN_POINT('Ctrl Pts',(1.65139534930353,-1.,3.47749926256543));
#43165=CARTESIAN_POINT('Ctrl Pts',(1.65139534930353,1.,3.47749926256543));
#43166=CARTESIAN_POINT('Ctrl Pts',(1.64971118698285,-1.,3.47028140996055));
#43167=CARTESIAN_POINT('Ctrl Pts',(1.64971118698285,1.,3.47028140996055));
#43168=CARTESIAN_POINT('Ctrl Pts',(1.64802323352752,-1.,3.46321237515029));
#43169=CARTESIAN_POINT('Ctrl Pts',(1.64802323352752,1.,3.46321237515029));
#43170=CARTESIAN_POINT('Ctrl Pts',(1.64632429697506,-1.,3.4562842106239));
#43171=CARTESIAN_POINT('Ctrl Pts',(1.64632429697506,1.,3.4562842106239));
#43172=CARTESIAN_POINT('Ctrl Pts',(1.64457408708059,-1.,3.44942242546693));
#43173=CARTESIAN_POINT('Ctrl Pts',(1.64457408708059,1.,3.44942242546693));
#43174=CARTESIAN_POINT('Ctrl Pts',(1.64270733821042,-1.,3.44250337701736));
#43175=CARTESIAN_POINT('Ctrl Pts',(1.64270733821042,1.,3.44250337701736));
#43176=CARTESIAN_POINT('Ctrl Pts',(1.64065778701952,-1.,3.43540451921397));
#43177=CARTESIAN_POINT('Ctrl Pts',(1.64065778701952,1.,3.43540451921397));
#43178=CARTESIAN_POINT('Ctrl Pts',(1.6383787624689,-1.,3.42804772926214));
#43179=CARTESIAN_POINT('Ctrl Pts',(1.6383787624689,1.,3.42804772926214));
#43180=CARTESIAN_POINT('Ctrl Pts',(1.63586250099804,-1.,3.4204397459095));
#43181=CARTESIAN_POINT('Ctrl Pts',(1.63586250099804,1.,3.4204397459095));
#43182=CARTESIAN_POINT('Ctrl Pts',(1.63316667054156,-1.,3.41272817148719));
#43183=CARTESIAN_POINT('Ctrl Pts',(1.63316667054156,1.,3.41272817148719));
#43184=CARTESIAN_POINT('Ctrl Pts',(1.63041148964996,-1.,3.40519422740596));
#43185=CARTESIAN_POINT('Ctrl Pts',(1.63041148964996,1.,3.40519422740596));
#43186=CARTESIAN_POINT('Ctrl Pts',(1.62774916464571,-1.,3.39818605298342));
#43187=CARTESIAN_POINT('Ctrl Pts',(1.62774916464571,1.,3.39818605298342));
#43188=CARTESIAN_POINT('Ctrl Pts',(1.62533996116793,-1.,3.39206617497078));
#43189=CARTESIAN_POINT('Ctrl Pts',(1.62533996116793,1.,3.39206617497078));
#43190=CARTESIAN_POINT('Ctrl Pts',(1.62332788556183,-1.,3.38715832178929));
#43191=CARTESIAN_POINT('Ctrl Pts',(1.62332788556183,1.,3.38715832178929));
#43192=CARTESIAN_POINT('Ctrl Pts',(1.62181089631134,-1.,3.38368201668123));
#43193=CARTESIAN_POINT('Ctrl Pts',(1.62181089631134,1.,3.38368201668123));
#43194=CARTESIAN_POINT('Ctrl Pts',(1.62103022180917,-1.,3.38212861099481));
#43195=CARTESIAN_POINT('Ctrl Pts',(1.62103022180917,1.,3.38212861099481));
#43196=CARTESIAN_POINT('Ctrl Pts',(1.6206953236804,-1.,3.38166984193496));
#43197=CARTESIAN_POINT('Ctrl Pts',(1.6206953236804,1.,3.38166984193496));
#43198=CARTESIAN_POINT('Ctrl Pts',(1.62058335162421,-1.,3.38167767992546));
#43199=CARTESIAN_POINT('Ctrl Pts',(1.62058335162421,1.,3.38167767992546));
#43200=CARTESIAN_POINT('Ctrl Pts',(1.62055519152808,-1.,3.38176002566879));
#43201=CARTESIAN_POINT('Ctrl Pts',(1.62055519152808,1.,3.38176002566879));
#43202=CARTESIAN_POINT('',(1.67727921511438,1.,3.85054988729471));
#43203=CARTESIAN_POINT('Ctrl Pts',(1.67727921511438,1.,3.85054988729471));
#43204=CARTESIAN_POINT('Ctrl Pts',(1.6773605765671,1.,3.84897939431104));
#43205=CARTESIAN_POINT('Ctrl Pts',(1.67751991140661,1.,3.84583912297567));
#43206=CARTESIAN_POINT('Ctrl Pts',(1.67774874946867,1.,3.8411308598706));
#43207=CARTESIAN_POINT('Ctrl Pts',(1.67803353065273,1.,3.83485746516115));
#43208=CARTESIAN_POINT('Ctrl Pts',(1.67835555760094,1.,3.82702289288453));
#43209=CARTESIAN_POINT('Ctrl Pts',(1.67864354606363,1.,3.81919554100522));
#43210=CARTESIAN_POINT('Ctrl Pts',(1.67889737738311,1.,3.81137549624273));
#43211=CARTESIAN_POINT('Ctrl Pts',(1.67911690648128,1.,3.80356289078481));
#43212=CARTESIAN_POINT('Ctrl Pts',(1.67930196625203,1.,3.7957579157763));
#43213=CARTESIAN_POINT('Ctrl Pts',(1.67945236653175,1.,3.78796080021026));
#43214=CARTESIAN_POINT('Ctrl Pts',(1.67956789211943,1.,3.78017178196859));
#43215=CARTESIAN_POINT('Ctrl Pts',(1.67964830084946,1.,3.77239107928394));
#43216=CARTESIAN_POINT('Ctrl Pts',(1.67969332319322,1.,3.76461886684523));
#43217=CARTESIAN_POINT('Ctrl Pts',(1.67970265841379,1.,3.75685523754816));
#43218=CARTESIAN_POINT('Ctrl Pts',(1.67967598599665,1.,3.74910022394845));
#43219=CARTESIAN_POINT('Ctrl Pts',(1.67961298685316,1.,3.74135385965622));
#43220=CARTESIAN_POINT('Ctrl Pts',(1.67951336376434,1.,3.73361623282617));
#43221=CARTESIAN_POINT('Ctrl Pts',(1.67937685856627,1.,3.72588753416339));
#43222=CARTESIAN_POINT('Ctrl Pts',(1.6792032807165,1.,3.71816812842188));
#43223=CARTESIAN_POINT('Ctrl Pts',(1.67899249793398,1.,3.71045854208195));
#43224=CARTESIAN_POINT('Ctrl Pts',(1.6787443694862,1.,3.70275932350998));
#43225=CARTESIAN_POINT('Ctrl Pts',(1.67845869064304,1.,3.69507092759545));
#43226=CARTESIAN_POINT('Ctrl Pts',(1.67813513867973,1.,3.68739360236505));
#43227=CARTESIAN_POINT('Ctrl Pts',(1.67777320475872,1.,3.6797272457918));
#43228=CARTESIAN_POINT('Ctrl Pts',(1.67737217414901,1.,3.67207136294639));
#43229=CARTESIAN_POINT('Ctrl Pts',(1.67693128053153,1.,3.66442538671018));
#43230=CARTESIAN_POINT('Ctrl Pts',(1.67644983469459,1.,3.65678894416442));
#43231=CARTESIAN_POINT('Ctrl Pts',(1.6759273594669,1.,3.64916213574663));
#43232=CARTESIAN_POINT('Ctrl Pts',(1.67536373264839,1.,3.6415458297232));
#43233=CARTESIAN_POINT('Ctrl Pts',(1.67475929882962,1.,3.63394189312902));
#43234=CARTESIAN_POINT('Ctrl Pts',(1.67411452372265,1.,3.62635249450908));
#43235=CARTESIAN_POINT('Ctrl Pts',(1.67342968196223,1.,3.61877947398179));
#43236=CARTESIAN_POINT('Ctrl Pts',(1.67270452466968,1.,3.61122367156182));
#43237=CARTESIAN_POINT('Ctrl Pts',(1.67193797318598,1.,3.60368430815203));
#43238=CARTESIAN_POINT('Ctrl Pts',(1.67112775290706,1.,3.59615824388808));
#43239=CARTESIAN_POINT('Ctrl Pts',(1.67027110397601,1.,3.5886414309783));
#43240=CARTESIAN_POINT('Ctrl Pts',(1.66936552908228,1.,3.58113044183823));
#43241=CARTESIAN_POINT('Ctrl Pts',(1.66840957407299,1.,3.57362406285884));
#43242=CARTESIAN_POINT('Ctrl Pts',(1.66740349220308,1.,3.56612465179429));
#43243=CARTESIAN_POINT('Ctrl Pts',(1.66635023293121,1.,3.55864015233617));
#43244=CARTESIAN_POINT('Ctrl Pts',(1.66525401569004,1.,3.5511812134288));
#43245=CARTESIAN_POINT('Ctrl Pts',(1.66411849222334,1.,3.5437574747503));
#43246=CARTESIAN_POINT('Ctrl Pts',(1.66294490916113,1.,3.53637385060225));
#43247=CARTESIAN_POINT('Ctrl Pts',(1.66173058912365,1.,3.52902746211082));
#43248=CARTESIAN_POINT('Ctrl Pts',(1.66046645222266,1.,3.52170261543787));
#43249=CARTESIAN_POINT('Ctrl Pts',(1.65913971687324,1.,3.51437632188903));
#43250=CARTESIAN_POINT('Ctrl Pts',(1.65773832633617,1.,3.5070273314651));
#43251=CARTESIAN_POINT('Ctrl Pts',(1.65625517961583,1.,3.49964476477929));
#43252=CARTESIAN_POINT('Ctrl Pts',(1.65469162644476,1.,3.49223525300194));
#43253=CARTESIAN_POINT('Ctrl Pts',(1.65306335367762,1.,3.48483492840942));
#43254=CARTESIAN_POINT('Ctrl Pts',(1.65139534930353,1.,3.47749926256543));
#43255=CARTESIAN_POINT('Ctrl Pts',(1.64971118698285,1.,3.47028140996055));
#43256=CARTESIAN_POINT('Ctrl Pts',(1.64802323352752,1.,3.46321237515029));
#43257=CARTESIAN_POINT('Ctrl Pts',(1.64632429697506,1.,3.4562842106239));
#43258=CARTESIAN_POINT('Ctrl Pts',(1.64457408708059,1.,3.44942242546693));
#43259=CARTESIAN_POINT('Ctrl Pts',(1.64270733821042,1.,3.44250337701736));
#43260=CARTESIAN_POINT('Ctrl Pts',(1.64065778701952,1.,3.43540451921397));
#43261=CARTESIAN_POINT('Ctrl Pts',(1.6383787624689,1.,3.42804772926214));
#43262=CARTESIAN_POINT('Ctrl Pts',(1.63586250099804,1.,3.4204397459095));
#43263=CARTESIAN_POINT('Ctrl Pts',(1.63316667054156,1.,3.41272817148719));
#43264=CARTESIAN_POINT('Ctrl Pts',(1.63041148964996,1.,3.40519422740596));
#43265=CARTESIAN_POINT('Ctrl Pts',(1.62774916464571,1.,3.39818605298342));
#43266=CARTESIAN_POINT('Ctrl Pts',(1.62533996116793,1.,3.39206617497078));
#43267=CARTESIAN_POINT('Ctrl Pts',(1.62332788556183,1.,3.38715832178929));
#43268=CARTESIAN_POINT('Ctrl Pts',(1.62192472202795,1.,3.3839428576331));
#43269=CARTESIAN_POINT('Ctrl Pts',(1.62118047294574,1.,3.38243080602536));
#43270=CARTESIAN_POINT('Ctrl Pts',(1.62083271136059,1.,3.38187506457001));
#43271=CARTESIAN_POINT('Ctrl Pts',(1.62069086551626,1.,3.38173802621243));
#43272=CARTESIAN_POINT('Ctrl Pts',(1.62064718014256,1.,3.38171594275687));
#43273=CARTESIAN_POINT('',(1.67727921511438,0.,3.85054988729471));
#43274=CARTESIAN_POINT('Ctrl Pts',(1.24535988127942,-1.,3.53717101171257));
#43275=CARTESIAN_POINT('Ctrl Pts',(1.24535988127942,1.,3.53717101171257));
#43276=CARTESIAN_POINT('Ctrl Pts',(1.24528174185147,-1.,3.53713269667534));
#43277=CARTESIAN_POINT('Ctrl Pts',(1.24528174185147,1.,3.53713269667534));
#43278=CARTESIAN_POINT('Ctrl Pts',(1.2451970233558,-1.,3.53720633058152));
#43279=CARTESIAN_POINT('Ctrl Pts',(1.2451970233558,1.,3.53720633058152));
#43280=CARTESIAN_POINT('Ctrl Pts',(1.24528461333177,-1.,3.53776753803428));
#43281=CARTESIAN_POINT('Ctrl Pts',(1.24528461333177,1.,3.53776753803428));
#43282=CARTESIAN_POINT('Ctrl Pts',(1.24583101679199,-1.,3.53941798196293));
#43283=CARTESIAN_POINT('Ctrl Pts',(1.24583101679199,1.,3.53941798196293));
#43284=CARTESIAN_POINT('Ctrl Pts',(1.2472164623202,-1.,3.54294877426113));
#43285=CARTESIAN_POINT('Ctrl Pts',(1.2472164623202,1.,3.54294877426113));
#43286=CARTESIAN_POINT('Ctrl Pts',(1.24926408627938,-1.,3.54784190282889));
#43287=CARTESIAN_POINT('Ctrl Pts',(1.24926408627938,1.,3.54784190282889));
#43288=CARTESIAN_POINT('Ctrl Pts',(1.25188792940508,-1.,3.5538728741862));
#43289=CARTESIAN_POINT('Ctrl Pts',(1.25188792940508,1.,3.5538728741862));
#43290=CARTESIAN_POINT('Ctrl Pts',(1.25496090899873,-1.,3.56071094990825));
#43291=CARTESIAN_POINT('Ctrl Pts',(1.25496090899873,1.,3.56071094990825));
#43292=CARTESIAN_POINT('Ctrl Pts',(1.25834000485626,-1.,3.56798645995025));
#43293=CARTESIAN_POINT('Ctrl Pts',(1.25834000485626,1.,3.56798645995025));
#43294=CARTESIAN_POINT('Ctrl Pts',(1.26188667142784,-1.,3.5753456065164));
#43295=CARTESIAN_POINT('Ctrl Pts',(1.26188667142784,1.,3.5753456065164));
#43296=CARTESIAN_POINT('Ctrl Pts',(1.26548706249891,-1.,3.58250452868699));
#43297=CARTESIAN_POINT('Ctrl Pts',(1.26548706249891,1.,3.58250452868699));
#43298=CARTESIAN_POINT('Ctrl Pts',(1.26907758484766,-1.,3.5893180784647));
#43299=CARTESIAN_POINT('Ctrl Pts',(1.26907758484766,1.,3.5893180784647));
#43300=CARTESIAN_POINT('Ctrl Pts',(1.27264798379365,-1.,3.59578698050164));
#43301=CARTESIAN_POINT('Ctrl Pts',(1.27264798379365,1.,3.59578698050164));
#43302=CARTESIAN_POINT('Ctrl Pts',(1.27622049908664,-1.,3.60199947736404));
#43303=CARTESIAN_POINT('Ctrl Pts',(1.27622049908664,1.,3.60199947736404));
#43304=CARTESIAN_POINT('Ctrl Pts',(1.27983492861703,-1.,3.60808907746372));
#43305=CARTESIAN_POINT('Ctrl Pts',(1.27983492861703,1.,3.60808907746372));
#43306=CARTESIAN_POINT('Ctrl Pts',(1.28353255117754,-1.,3.61418935913793));
#43307=CARTESIAN_POINT('Ctrl Pts',(1.28353255117754,1.,3.61418935913793));
#43308=CARTESIAN_POINT('Ctrl Pts',(1.2873375502936,-1.,3.62038148492295));
#43309=CARTESIAN_POINT('Ctrl Pts',(1.2873375502936,1.,3.62038148492295));
#43310=CARTESIAN_POINT('Ctrl Pts',(1.29125046021853,-1.,3.62667616004299));
#43311=CARTESIAN_POINT('Ctrl Pts',(1.29125046021853,1.,3.62667616004299));
#43312=CARTESIAN_POINT('Ctrl Pts',(1.29525810207744,-1.,3.63304271630995));
#43313=CARTESIAN_POINT('Ctrl Pts',(1.29525810207744,1.,3.63304271630995));
#43314=CARTESIAN_POINT('Ctrl Pts',(1.29933955906463,-1.,3.6394268987279));
#43315=CARTESIAN_POINT('Ctrl Pts',(1.29933955906463,1.,3.6394268987279));
#43316=CARTESIAN_POINT('Ctrl Pts',(1.30347327603778,-1.,3.64577181380125));
#43317=CARTESIAN_POINT('Ctrl Pts',(1.30347327603778,1.,3.64577181380125));
#43318=CARTESIAN_POINT('Ctrl Pts',(1.30764479590051,-1.,3.65204081987101));
#43319=CARTESIAN_POINT('Ctrl Pts',(1.30764479590051,1.,3.65204081987101));
#43320=CARTESIAN_POINT('Ctrl Pts',(1.31185038411231,-1.,3.65822827358655));
#43321=CARTESIAN_POINT('Ctrl Pts',(1.31185038411231,1.,3.65822827358655));
#43322=CARTESIAN_POINT('Ctrl Pts',(1.31609271239922,-1.,3.66434688899822));
#43323=CARTESIAN_POINT('Ctrl Pts',(1.31609271239922,1.,3.66434688899822));
#43324=CARTESIAN_POINT('Ctrl Pts',(1.3203782813777,-1.,3.67042021752668));
#43325=CARTESIAN_POINT('Ctrl Pts',(1.3203782813777,1.,3.67042021752668));
#43326=CARTESIAN_POINT('Ctrl Pts',(1.32471430856413,-1.,3.67647355257906));
#43327=CARTESIAN_POINT('Ctrl Pts',(1.32471430856413,1.,3.67647355257906));
#43328=CARTESIAN_POINT('Ctrl Pts',(1.32910547072734,-1.,3.68252441182534));
#43329=CARTESIAN_POINT('Ctrl Pts',(1.32910547072734,1.,3.68252441182534));
#43330=CARTESIAN_POINT('Ctrl Pts',(1.33355191034515,-1.,3.68857672413013));
#43331=CARTESIAN_POINT('Ctrl Pts',(1.33355191034515,1.,3.68857672413013));
#43332=CARTESIAN_POINT('Ctrl Pts',(1.33805103398214,-1.,3.69462613305692));
#43333=CARTESIAN_POINT('Ctrl Pts',(1.33805103398214,1.,3.69462613305692));
#43334=CARTESIAN_POINT('Ctrl Pts',(1.3425986075293,-1.,3.70066324015112));
#43335=CARTESIAN_POINT('Ctrl Pts',(1.3425986075293,1.,3.70066324015112));
#43336=CARTESIAN_POINT('Ctrl Pts',(1.34719008463535,-1.,3.7066775318825));
#43337=CARTESIAN_POINT('Ctrl Pts',(1.34719008463535,1.,3.7066775318825));
#43338=CARTESIAN_POINT('Ctrl Pts',(1.35182193384426,-1.,3.71266130563061));
#43339=CARTESIAN_POINT('Ctrl Pts',(1.35182193384426,1.,3.71266130563061));
#43340=CARTESIAN_POINT('Ctrl Pts',(1.35649266705038,-1.,3.71861271513318));
#43341=CARTESIAN_POINT('Ctrl Pts',(1.35649266705038,1.,3.71861271513318));
#43342=CARTESIAN_POINT('Ctrl Pts',(1.36120211416353,-1.,3.72453364678279));
#43343=CARTESIAN_POINT('Ctrl Pts',(1.36120211416353,1.,3.72453364678279));
#43344=CARTESIAN_POINT('Ctrl Pts',(1.36595093298674,-1.,3.73042829011293));
#43345=CARTESIAN_POINT('Ctrl Pts',(1.36595093298674,1.,3.73042829011293));
#43346=CARTESIAN_POINT('Ctrl Pts',(1.37074003422739,-1.,3.73630145885809));
#43347=CARTESIAN_POINT('Ctrl Pts',(1.37074003422739,1.,3.73630145885809));
#43348=CARTESIAN_POINT('Ctrl Pts',(1.3755700297169,-1.,3.7421569816256));
#43349=CARTESIAN_POINT('Ctrl Pts',(1.3755700297169,1.,3.7421569816256));
#43350=CARTESIAN_POINT('Ctrl Pts',(1.38044070763302,-1.,3.74799617204744));
#43351=CARTESIAN_POINT('Ctrl Pts',(1.38044070763302,1.,3.74799617204744));
#43352=CARTESIAN_POINT('Ctrl Pts',(1.38535129801185,-1.,3.75381861212728));
#43353=CARTESIAN_POINT('Ctrl Pts',(1.38535129801185,1.,3.75381861212728));
#43354=CARTESIAN_POINT('Ctrl Pts',(1.39030069388926,-1.,3.75962280650875));
#43355=CARTESIAN_POINT('Ctrl Pts',(1.39030069388926,1.,3.75962280650875));
#43356=CARTESIAN_POINT('Ctrl Pts',(1.39528769118054,-1.,3.76540689249078));
#43357=CARTESIAN_POINT('Ctrl Pts',(1.39528769118054,1.,3.76540689249078));
#43358=CARTESIAN_POINT('Ctrl Pts',(1.40031121335495,-1.,3.77116930621804));
#43359=CARTESIAN_POINT('Ctrl Pts',(1.40031121335495,1.,3.77116930621804));
#43360=CARTESIAN_POINT('Ctrl Pts',(1.40537056004702,-1.,3.77690952014209));
#43361=CARTESIAN_POINT('Ctrl Pts',(1.40537056004702,1.,3.77690952014209));
#43362=CARTESIAN_POINT('Ctrl Pts',(1.41046532282567,-1.,3.78262780065406));
#43363=CARTESIAN_POINT('Ctrl Pts',(1.41046532282567,1.,3.78262780065406));
#43364=CARTESIAN_POINT('Ctrl Pts',(1.41559527803808,-1.,3.78832489879369));
#43365=CARTESIAN_POINT('Ctrl Pts',(1.41559527803808,1.,3.78832489879369));
#43366=CARTESIAN_POINT('Ctrl Pts',(1.42076028482828,-1.,3.7940017574439));
#43367=CARTESIAN_POINT('Ctrl Pts',(1.42076028482828,1.,3.7940017574439));
#43368=CARTESIAN_POINT('Ctrl Pts',(1.42596018777301,-1.,3.79965923196365));
#43369=CARTESIAN_POINT('Ctrl Pts',(1.42596018777301,1.,3.79965923196365));
#43370=CARTESIAN_POINT('Ctrl Pts',(1.43119469921364,-1.,3.80529775429916));
#43371=CARTESIAN_POINT('Ctrl Pts',(1.43119469921364,1.,3.80529775429916));
#43372=CARTESIAN_POINT('Ctrl Pts',(1.43646341556783,-1.,3.81091737726965));
#43373=CARTESIAN_POINT('Ctrl Pts',(1.43646341556783,1.,3.81091737726965));
#43374=CARTESIAN_POINT('Ctrl Pts',(1.441765870414,-1.,3.8165179239855));
#43375=CARTESIAN_POINT('Ctrl Pts',(1.441765870414,1.,3.8165179239855));
#43376=CARTESIAN_POINT('Ctrl Pts',(1.44710157648562,-1.,3.82209910620591));
#43377=CARTESIAN_POINT('Ctrl Pts',(1.44710157648562,1.,3.82209910620591));
#43378=CARTESIAN_POINT('Ctrl Pts',(1.45247006796807,-1.,3.82766064519));
#43379=CARTESIAN_POINT('Ctrl Pts',(1.45247006796807,1.,3.82766064519));
#43380=CARTESIAN_POINT('Ctrl Pts',(1.45787095220763,-1.,3.83320241775199));
#43381=CARTESIAN_POINT('Ctrl Pts',(1.45787095220763,1.,3.83320241775199));
#43382=CARTESIAN_POINT('Ctrl Pts',(1.46330391180621,-1.,3.83872447159309));
#43383=CARTESIAN_POINT('Ctrl Pts',(1.46330391180621,1.,3.83872447159309));
#43384=CARTESIAN_POINT('Ctrl Pts',(1.46876867426374,-1.,3.84422695454469));
#43385=CARTESIAN_POINT('Ctrl Pts',(1.46876867426374,1.,3.84422695454469));
#43386=CARTESIAN_POINT('Ctrl Pts',(1.47426499018467,-1.,3.84971006847096));
#43387=CARTESIAN_POINT('Ctrl Pts',(1.47426499018467,1.,3.84971006847096));
#43388=CARTESIAN_POINT('Ctrl Pts',(1.47979260991063,-1.,3.85517401698952));
#43389=CARTESIAN_POINT('Ctrl Pts',(1.47979260991063,1.,3.85517401698952));
#43390=CARTESIAN_POINT('Ctrl Pts',(1.48535125510102,-1.,3.86061894706551));
#43391=CARTESIAN_POINT('Ctrl Pts',(1.48535125510102,1.,3.86061894706551));
#43392=CARTESIAN_POINT('Ctrl Pts',(1.49094061164604,-1.,3.86604492575933));
#43393=CARTESIAN_POINT('Ctrl Pts',(1.49094061164604,1.,3.86604492575933));
#43394=CARTESIAN_POINT('Ctrl Pts',(1.4965603539944,-1.,3.8714519699927));
#43395=CARTESIAN_POINT('Ctrl Pts',(1.4965603539944,1.,3.8714519699927));
#43396=CARTESIAN_POINT('Ctrl Pts',(1.50221016176766,-1.,3.87684006372665));
#43397=CARTESIAN_POINT('Ctrl Pts',(1.50221016176766,1.,3.87684006372665));
#43398=CARTESIAN_POINT('Ctrl Pts',(1.50788973857719,-1.,3.88220917950443));
#43399=CARTESIAN_POINT('Ctrl Pts',(1.50788973857719,1.,3.88220917950443));
#43400=CARTESIAN_POINT('Ctrl Pts',(1.51359883110181,-1.,3.88755930032927));
#43401=CARTESIAN_POINT('Ctrl Pts',(1.51359883110181,1.,3.88755930032927));
#43402=CARTESIAN_POINT('Ctrl Pts',(1.51933724328609,-1.,3.89289043531893));
#43403=CARTESIAN_POINT('Ctrl Pts',(1.51933724328609,1.,3.89289043531893));
#43404=CARTESIAN_POINT('Ctrl Pts',(1.52510482990784,-1.,3.8982026070607));
#43405=CARTESIAN_POINT('Ctrl Pts',(1.52510482990784,1.,3.8982026070607));
#43406=CARTESIAN_POINT('Ctrl Pts',(1.5297421605556,-1.,3.90243719629755));
#43407=CARTESIAN_POINT('Ctrl Pts',(1.5297421605556,1.,3.90243719629755));
#43408=CARTESIAN_POINT('Ctrl Pts',(1.53323321827311,-1.,3.90560462812846));
#43409=CARTESIAN_POINT('Ctrl Pts',(1.53323321827311,1.,3.90560462812846));
#43410=CARTESIAN_POINT('Ctrl Pts',(1.53556639217742,-1.,3.90771246854607));
#43411=CARTESIAN_POINT('Ctrl Pts',(1.53556639217742,1.,3.90771246854607));
#43412=CARTESIAN_POINT('Ctrl Pts',(1.53673442965255,-1.,3.90876544355381));
#43413=CARTESIAN_POINT('Ctrl Pts',(1.53673442965255,1.,3.90876544355381));
#43414=CARTESIAN_POINT('',(1.24526366418208,1.,3.5372048861591));
#43415=CARTESIAN_POINT('Ctrl Pts',(1.24526366418208,-1.,3.5372048861591));
#43416=CARTESIAN_POINT('Ctrl Pts',(1.24526366418208,-0.666666666666667,
3.5372048861591));
#43417=CARTESIAN_POINT('Ctrl Pts',(1.24526366418208,-0.333333333333333,
3.5372048861591));
#43418=CARTESIAN_POINT('Ctrl Pts',(1.24526366418208,0.333333333333333,3.5372048861591));
#43419=CARTESIAN_POINT('Ctrl Pts',(1.24526366418208,0.666666666666667,3.5372048861591));
#43420=CARTESIAN_POINT('Ctrl Pts',(1.24526366418208,1.,3.5372048861591));
#43421=CARTESIAN_POINT('',(1.53673442965255,1.,3.90876544355381));
#43422=CARTESIAN_POINT('',(1.53673442965255,0.,3.90876544355381));
#43423=CARTESIAN_POINT('Ctrl Pts',(1.24526366418208,1.,3.5372048861591));
#43424=CARTESIAN_POINT('Ctrl Pts',(1.24524838931864,1.,3.53725139174402));
#43425=CARTESIAN_POINT('Ctrl Pts',(1.24524498991133,1.,3.53744859265385));
#43426=CARTESIAN_POINT('Ctrl Pts',(1.2453920538873,1.,3.53808746578052));
#43427=CARTESIAN_POINT('Ctrl Pts',(1.24593497225964,1.,3.53968291129942));
#43428=CARTESIAN_POINT('Ctrl Pts',(1.2472164623202,1.,3.54294877426113));
#43429=CARTESIAN_POINT('Ctrl Pts',(1.24926408627938,1.,3.54784190282889));
#43430=CARTESIAN_POINT('Ctrl Pts',(1.25188792940508,1.,3.5538728741862));
#43431=CARTESIAN_POINT('Ctrl Pts',(1.25496090899873,1.,3.56071094990825));
#43432=CARTESIAN_POINT('Ctrl Pts',(1.25834000485626,1.,3.56798645995025));
#43433=CARTESIAN_POINT('Ctrl Pts',(1.26188667142784,1.,3.5753456065164));
#43434=CARTESIAN_POINT('Ctrl Pts',(1.26548706249891,1.,3.58250452868699));
#43435=CARTESIAN_POINT('Ctrl Pts',(1.26907758484766,1.,3.5893180784647));
#43436=CARTESIAN_POINT('Ctrl Pts',(1.27264798379365,1.,3.59578698050164));
#43437=CARTESIAN_POINT('Ctrl Pts',(1.27622049908664,1.,3.60199947736404));
#43438=CARTESIAN_POINT('Ctrl Pts',(1.27983492861703,1.,3.60808907746372));
#43439=CARTESIAN_POINT('Ctrl Pts',(1.28353255117754,1.,3.61418935913793));
#43440=CARTESIAN_POINT('Ctrl Pts',(1.2873375502936,1.,3.62038148492295));
#43441=CARTESIAN_POINT('Ctrl Pts',(1.29125046021853,1.,3.62667616004299));
#43442=CARTESIAN_POINT('Ctrl Pts',(1.29525810207744,1.,3.63304271630995));
#43443=CARTESIAN_POINT('Ctrl Pts',(1.29933955906463,1.,3.6394268987279));
#43444=CARTESIAN_POINT('Ctrl Pts',(1.30347327603778,1.,3.64577181380125));
#43445=CARTESIAN_POINT('Ctrl Pts',(1.30764479590051,1.,3.65204081987101));
#43446=CARTESIAN_POINT('Ctrl Pts',(1.31185038411231,1.,3.65822827358655));
#43447=CARTESIAN_POINT('Ctrl Pts',(1.31609271239922,1.,3.66434688899822));
#43448=CARTESIAN_POINT('Ctrl Pts',(1.3203782813777,1.,3.67042021752668));
#43449=CARTESIAN_POINT('Ctrl Pts',(1.32471430856413,1.,3.67647355257906));
#43450=CARTESIAN_POINT('Ctrl Pts',(1.32910547072734,1.,3.68252441182534));
#43451=CARTESIAN_POINT('Ctrl Pts',(1.33355191034515,1.,3.68857672413013));
#43452=CARTESIAN_POINT('Ctrl Pts',(1.33805103398214,1.,3.69462613305692));
#43453=CARTESIAN_POINT('Ctrl Pts',(1.3425986075293,1.,3.70066324015112));
#43454=CARTESIAN_POINT('Ctrl Pts',(1.34719008463535,1.,3.7066775318825));
#43455=CARTESIAN_POINT('Ctrl Pts',(1.35182193384426,1.,3.71266130563061));
#43456=CARTESIAN_POINT('Ctrl Pts',(1.35649266705038,1.,3.71861271513318));
#43457=CARTESIAN_POINT('Ctrl Pts',(1.36120211416353,1.,3.72453364678279));
#43458=CARTESIAN_POINT('Ctrl Pts',(1.36595093298674,1.,3.73042829011293));
#43459=CARTESIAN_POINT('Ctrl Pts',(1.37074003422739,1.,3.73630145885809));
#43460=CARTESIAN_POINT('Ctrl Pts',(1.3755700297169,1.,3.7421569816256));
#43461=CARTESIAN_POINT('Ctrl Pts',(1.38044070763302,1.,3.74799617204744));
#43462=CARTESIAN_POINT('Ctrl Pts',(1.38535129801185,1.,3.75381861212728));
#43463=CARTESIAN_POINT('Ctrl Pts',(1.39030069388926,1.,3.75962280650875));
#43464=CARTESIAN_POINT('Ctrl Pts',(1.39528769118054,1.,3.76540689249078));
#43465=CARTESIAN_POINT('Ctrl Pts',(1.40031121335495,1.,3.77116930621804));
#43466=CARTESIAN_POINT('Ctrl Pts',(1.40537056004702,1.,3.77690952014209));
#43467=CARTESIAN_POINT('Ctrl Pts',(1.41046532282567,1.,3.78262780065406));
#43468=CARTESIAN_POINT('Ctrl Pts',(1.41559527803808,1.,3.78832489879369));
#43469=CARTESIAN_POINT('Ctrl Pts',(1.42076028482828,1.,3.7940017574439));
#43470=CARTESIAN_POINT('Ctrl Pts',(1.42596018777301,1.,3.79965923196365));
#43471=CARTESIAN_POINT('Ctrl Pts',(1.43119469921364,1.,3.80529775429916));
#43472=CARTESIAN_POINT('Ctrl Pts',(1.43646341556783,1.,3.81091737726965));
#43473=CARTESIAN_POINT('Ctrl Pts',(1.441765870414,1.,3.8165179239855));
#43474=CARTESIAN_POINT('Ctrl Pts',(1.44710157648562,1.,3.82209910620591));
#43475=CARTESIAN_POINT('Ctrl Pts',(1.45247006796807,1.,3.82766064519));
#43476=CARTESIAN_POINT('Ctrl Pts',(1.45787095220763,1.,3.83320241775199));
#43477=CARTESIAN_POINT('Ctrl Pts',(1.46330391180621,1.,3.83872447159309));
#43478=CARTESIAN_POINT('Ctrl Pts',(1.46876867426374,1.,3.84422695454469));
#43479=CARTESIAN_POINT('Ctrl Pts',(1.47426499018467,1.,3.84971006847096));
#43480=CARTESIAN_POINT('Ctrl Pts',(1.47979260991063,1.,3.85517401698952));
#43481=CARTESIAN_POINT('Ctrl Pts',(1.48535125510102,1.,3.86061894706551));
#43482=CARTESIAN_POINT('Ctrl Pts',(1.49094061164604,1.,3.86604492575933));
#43483=CARTESIAN_POINT('Ctrl Pts',(1.4965603539944,1.,3.8714519699927));
#43484=CARTESIAN_POINT('Ctrl Pts',(1.50221016176766,1.,3.87684006372665));
#43485=CARTESIAN_POINT('Ctrl Pts',(1.50788973857719,1.,3.88220917950443));
#43486=CARTESIAN_POINT('Ctrl Pts',(1.51359883110181,1.,3.88755930032927));
#43487=CARTESIAN_POINT('Ctrl Pts',(1.51933724328609,1.,3.89289043531893));
#43488=CARTESIAN_POINT('Ctrl Pts',(1.52510482990784,1.,3.8982026070607));
#43489=CARTESIAN_POINT('Ctrl Pts',(1.5297421605556,1.,3.90243719629755));
#43490=CARTESIAN_POINT('Ctrl Pts',(1.53323321827311,1.,3.90560462812846));
#43491=CARTESIAN_POINT('Ctrl Pts',(1.53556639217742,1.,3.90771246854607));
#43492=CARTESIAN_POINT('Ctrl Pts',(1.53673442965255,1.,3.90876544355381));
#43493=CARTESIAN_POINT('Origin',(1.53673442965255,0.,3.90876544355381));
#43494=CARTESIAN_POINT('',(1.67727921511438,1.,3.85054988729471));
#43495=CARTESIAN_POINT('Origin',(0.,0.,0.));
#43496=CARTESIAN_POINT('',(1.071677399622,1.,3.59360648251021));
#43497=CARTESIAN_POINT('Origin',(0.,1.,0.));
#43498=CARTESIAN_POINT('Ctrl Pts',(1.071677399622,1.,3.59360648251021));
#43499=CARTESIAN_POINT('Ctrl Pts',(1.071677399622,0.666666666666667,3.59360648251021));
#43500=CARTESIAN_POINT('Ctrl Pts',(1.071677399622,0.333333333333333,3.59360648251021));
#43501=CARTESIAN_POINT('Ctrl Pts',(1.071677399622,-0.333333333333333,3.59360648251021));
#43502=CARTESIAN_POINT('Ctrl Pts',(1.071677399622,-0.666666666666667,3.59360648251021));
#43503=CARTESIAN_POINT('Ctrl Pts',(1.071677399622,-1.,3.59360648251021));
#43504=CARTESIAN_POINT('Ctrl Pts',(1.05427041296137,-1.,4.06552750530042));
#43505=CARTESIAN_POINT('Ctrl Pts',(1.05427041296137,1.,4.06552750530042));
#43506=CARTESIAN_POINT('Ctrl Pts',(1.05459645194934,-1.,4.06398907542679));
#43507=CARTESIAN_POINT('Ctrl Pts',(1.05459645194934,1.,4.06398907542679));
#43508=CARTESIAN_POINT('Ctrl Pts',(1.05524507177901,-1.,4.06091239150293));
#43509=CARTESIAN_POINT('Ctrl Pts',(1.05524507177901,1.,4.06091239150293));
#43510=CARTESIAN_POINT('Ctrl Pts',(1.0562076270849,-1.,4.05629789308941));
#43511=CARTESIAN_POINT('Ctrl Pts',(1.0562076270849,1.,4.05629789308941));
#43512=CARTESIAN_POINT('Ctrl Pts',(1.05747027728537,-1.,4.05014628387112));
#43513=CARTESIAN_POINT('Ctrl Pts',(1.05747027728537,1.,4.05014628387112));
#43514=CARTESIAN_POINT('Ctrl Pts',(1.05901393667039,-1.,4.04245854429333));
#43515=CARTESIAN_POINT('Ctrl Pts',(1.05901393667039,1.,4.04245854429333));
#43516=CARTESIAN_POINT('Ctrl Pts',(1.06052284712114,-1.,4.03477261142549));
#43517=CARTESIAN_POINT('Ctrl Pts',(1.06052284712114,1.,4.03477261142549));
#43518=CARTESIAN_POINT('Ctrl Pts',(1.06199687787488,-1.,4.02708855235732));
#43519=CARTESIAN_POINT('Ctrl Pts',(1.06199687787488,1.,4.02708855235732));
#43520=CARTESIAN_POINT('Ctrl Pts',(1.06343586496094,-1.,4.0194064749539));
#43521=CARTESIAN_POINT('Ctrl Pts',(1.06343586496094,1.,4.0194064749539));
#43522=CARTESIAN_POINT('Ctrl Pts',(1.06483961342894,-1.,4.0117265418656));
#43523=CARTESIAN_POINT('Ctrl Pts',(1.06483961342894,1.,4.0117265418656));
#43524=CARTESIAN_POINT('Ctrl Pts',(1.06620789963406,-1.,4.00404894951804));
#43525=CARTESIAN_POINT('Ctrl Pts',(1.06620789963406,1.,4.00404894951804));
#43526=CARTESIAN_POINT('Ctrl Pts',(1.06754047381188,-1.,3.99637389919958));
#43527=CARTESIAN_POINT('Ctrl Pts',(1.06754047381188,1.,3.99637389919958));
#43528=CARTESIAN_POINT('Ctrl Pts',(1.06883706263912,-1.,3.98870156857298));
#43529=CARTESIAN_POINT('Ctrl Pts',(1.06883706263912,1.,3.98870156857298));
#43530=CARTESIAN_POINT('Ctrl Pts',(1.07009737257815,-1.,3.98103208801289));
#43531=CARTESIAN_POINT('Ctrl Pts',(1.07009737257815,1.,3.98103208801289));
#43532=CARTESIAN_POINT('Ctrl Pts',(1.07132109206252,-1.,3.97336550222571));
#43533=CARTESIAN_POINT('Ctrl Pts',(1.07132109206252,1.,3.97336550222571));
#43534=CARTESIAN_POINT('Ctrl Pts',(1.07250789943095,-1.,3.96570179322681));
#43535=CARTESIAN_POINT('Ctrl Pts',(1.07250789943095,1.,3.96570179322681));
#43536=CARTESIAN_POINT('Ctrl Pts',(1.07365747426551,-1.,3.95804094429606));
#43537=CARTESIAN_POINT('Ctrl Pts',(1.07365747426551,1.,3.95804094429606));
#43538=CARTESIAN_POINT('Ctrl Pts',(1.07476950921607,-1.,3.95038299600754));
#43539=CARTESIAN_POINT('Ctrl Pts',(1.07476950921607,1.,3.95038299600754));
#43540=CARTESIAN_POINT('Ctrl Pts',(1.07584371946428,-1.,3.94272809633271));
#43541=CARTESIAN_POINT('Ctrl Pts',(1.07584371946428,1.,3.94272809633271));
#43542=CARTESIAN_POINT('Ctrl Pts',(1.07687985975348,-1.,3.93507657572743));
#43543=CARTESIAN_POINT('Ctrl Pts',(1.07687985975348,1.,3.93507657572743));
#43544=CARTESIAN_POINT('Ctrl Pts',(1.07787771707155,-1.,3.92742893349684));
#43545=CARTESIAN_POINT('Ctrl Pts',(1.07787771707155,1.,3.92742893349684));
#43546=CARTESIAN_POINT('Ctrl Pts',(1.07883706663524,-1.,3.91978568924062));
#43547=CARTESIAN_POINT('Ctrl Pts',(1.07883706663524,1.,3.91978568924062));
#43548=CARTESIAN_POINT('Ctrl Pts',(1.0797576350746,-1.,3.91214726022096));
#43549=CARTESIAN_POINT('Ctrl Pts',(1.0797576350746,1.,3.91214726022096));
#43550=CARTESIAN_POINT('Ctrl Pts',(1.08063906483822,-1.,3.90451384092564));
#43551=CARTESIAN_POINT('Ctrl Pts',(1.08063906483822,1.,3.90451384092564));
#43552=CARTESIAN_POINT('Ctrl Pts',(1.08148086931373,-1.,3.89688525098408));
#43553=CARTESIAN_POINT('Ctrl Pts',(1.08148086931373,1.,3.89688525098408));
#43554=CARTESIAN_POINT('Ctrl Pts',(1.08228241999363,-1.,3.88926088975182));
#43555=CARTESIAN_POINT('Ctrl Pts',(1.08228241999363,1.,3.88926088975182));
#43556=CARTESIAN_POINT('Ctrl Pts',(1.08304304871042,-1.,3.88164007721365));
#43557=CARTESIAN_POINT('Ctrl Pts',(1.08304304871042,1.,3.88164007721365));
#43558=CARTESIAN_POINT('Ctrl Pts',(1.0837621330751,-1.,3.87402233722563));
#43559=CARTESIAN_POINT('Ctrl Pts',(1.0837621330751,1.,3.87402233722563));
#43560=CARTESIAN_POINT('Ctrl Pts',(1.08443918607926,-1.,3.86640769434269));
#43561=CARTESIAN_POINT('Ctrl Pts',(1.08443918607926,1.,3.86640769434269));
#43562=CARTESIAN_POINT('Ctrl Pts',(1.08507395120054,-1.,3.85879698702511));
#43563=CARTESIAN_POINT('Ctrl Pts',(1.08507395120054,1.,3.85879698702511));
#43564=CARTESIAN_POINT('Ctrl Pts',(1.08566647671838,-1.,3.85119211322732));
#43565=CARTESIAN_POINT('Ctrl Pts',(1.08566647671838,1.,3.85119211322732));
#43566=CARTESIAN_POINT('Ctrl Pts',(1.08621688337601,-1.,3.84359528764934));
#43567=CARTESIAN_POINT('Ctrl Pts',(1.08621688337601,1.,3.84359528764934));
#43568=CARTESIAN_POINT('Ctrl Pts',(1.08672515456901,-1.,3.83600837071702));
#43569=CARTESIAN_POINT('Ctrl Pts',(1.08672515456901,1.,3.83600837071702));
#43570=CARTESIAN_POINT('Ctrl Pts',(1.08719091307558,-1.,3.82843215316985));
#43571=CARTESIAN_POINT('Ctrl Pts',(1.08719091307558,1.,3.82843215316985));
#43572=CARTESIAN_POINT('Ctrl Pts',(1.08761321539442,-1.,3.82086569676321));
#43573=CARTESIAN_POINT('Ctrl Pts',(1.08761321539442,1.,3.82086569676321));
#43574=CARTESIAN_POINT('Ctrl Pts',(1.08799030610861,-1.,3.81330554446324));
#43575=CARTESIAN_POINT('Ctrl Pts',(1.08799030610861,1.,3.81330554446324));
#43576=CARTESIAN_POINT('Ctrl Pts',(1.08832009255378,-1.,3.80574726657656));
#43577=CARTESIAN_POINT('Ctrl Pts',(1.08832009255378,1.,3.80574726657656));
#43578=CARTESIAN_POINT('Ctrl Pts',(1.08860064435775,-1.,3.79818708705252));
#43579=CARTESIAN_POINT('Ctrl Pts',(1.08860064435775,1.,3.79818708705252));
#43580=CARTESIAN_POINT('Ctrl Pts',(1.08883071512097,-1.,3.79062357974401));
#43581=CARTESIAN_POINT('Ctrl Pts',(1.08883071512097,1.,3.79062357974401));
#43582=CARTESIAN_POINT('Ctrl Pts',(1.08901018614638,-1.,3.78305911299511));
#43583=CARTESIAN_POINT('Ctrl Pts',(1.08901018614638,1.,3.78305911299511));
#43584=CARTESIAN_POINT('Ctrl Pts',(1.08914072791275,-1.,3.7755019940944));
#43585=CARTESIAN_POINT('Ctrl Pts',(1.08914072791275,1.,3.7755019940944));
#43586=CARTESIAN_POINT('Ctrl Pts',(1.08922484204263,-1.,3.76796340094469));
#43587=CARTESIAN_POINT('Ctrl Pts',(1.08922484204263,1.,3.76796340094469));
#43588=CARTESIAN_POINT('Ctrl Pts',(1.08926462734287,-1.,3.76045342580226));
#43589=CARTESIAN_POINT('Ctrl Pts',(1.08926462734287,1.,3.76045342580226));
#43590=CARTESIAN_POINT('Ctrl Pts',(1.08926054632927,-1.,3.75297711748138));
#43591=CARTESIAN_POINT('Ctrl Pts',(1.08926054632927,1.,3.75297711748138));
#43592=CARTESIAN_POINT('Ctrl Pts',(1.08921040494013,-1.,3.74553121371745));
#43593=CARTESIAN_POINT('Ctrl Pts',(1.08921040494013,1.,3.74553121371745));
#43594=CARTESIAN_POINT('Ctrl Pts',(1.08910769013288,-1.,3.73809879348209));
#43595=CARTESIAN_POINT('Ctrl Pts',(1.08910769013288,1.,3.73809879348209));
#43596=CARTESIAN_POINT('Ctrl Pts',(1.08894337390925,-1.,3.73065515162949));
#43597=CARTESIAN_POINT('Ctrl Pts',(1.08894337390925,1.,3.73065515162949));
#43598=CARTESIAN_POINT('Ctrl Pts',(1.08870887220072,-1.,3.72317741369364));
#43599=CARTESIAN_POINT('Ctrl Pts',(1.08870887220072,1.,3.72317741369364));
#43600=CARTESIAN_POINT('Ctrl Pts',(1.08839887334776,-1.,3.71565372339063));
#43601=CARTESIAN_POINT('Ctrl Pts',(1.08839887334776,1.,3.71565372339063));
#43602=CARTESIAN_POINT('Ctrl Pts',(1.0880136731219,-1.,3.70809084139476));
#43603=CARTESIAN_POINT('Ctrl Pts',(1.0880136731219,1.,3.70809084139476));
#43604=CARTESIAN_POINT('Ctrl Pts',(1.08756311291324,-1.,3.70052690909884));
#43605=CARTESIAN_POINT('Ctrl Pts',(1.08756311291324,1.,3.70052690909884));
#43606=CARTESIAN_POINT('Ctrl Pts',(1.08706319540291,-1.,3.69302062410229));
#43607=CARTESIAN_POINT('Ctrl Pts',(1.08706319540291,1.,3.69302062410229));
#43608=CARTESIAN_POINT('Ctrl Pts',(1.08652888882609,-1.,3.68562817420864));
#43609=CARTESIAN_POINT('Ctrl Pts',(1.08652888882609,1.,3.68562817420864));
#43610=CARTESIAN_POINT('Ctrl Pts',(1.08596755755768,-1.,3.67838211685148));
#43611=CARTESIAN_POINT('Ctrl Pts',(1.08596755755768,1.,3.67838211685148));
#43612=CARTESIAN_POINT('Ctrl Pts',(1.0853733414448,-1.,3.67127347729632));
#43613=CARTESIAN_POINT('Ctrl Pts',(1.0853733414448,1.,3.67127347729632));
#43614=CARTESIAN_POINT('Ctrl Pts',(1.0847180992287,-1.,3.66422237895256));
#43615=CARTESIAN_POINT('Ctrl Pts',(1.0847180992287,1.,3.66422237895256));
#43616=CARTESIAN_POINT('Ctrl Pts',(1.08395671077761,-1.,3.65709649161004));
#43617=CARTESIAN_POINT('Ctrl Pts',(1.08395671077761,1.,3.65709649161004));
#43618=CARTESIAN_POINT('Ctrl Pts',(1.08304289898577,-1.,3.64976441208197));
#43619=CARTESIAN_POINT('Ctrl Pts',(1.08304289898577,1.,3.64976441208197));
#43620=CARTESIAN_POINT('Ctrl Pts',(1.08194278850972,-1.,3.64214167843595));
#43621=CARTESIAN_POINT('Ctrl Pts',(1.08194278850972,1.,3.64214167843595));
#43622=CARTESIAN_POINT('Ctrl Pts',(1.08064765719887,-1.,3.63423373196602));
#43623=CARTESIAN_POINT('Ctrl Pts',(1.08064765719887,1.,3.63423373196602));
#43624=CARTESIAN_POINT('Ctrl Pts',(1.07919137290815,-1.,3.62619537902616));
#43625=CARTESIAN_POINT('Ctrl Pts',(1.07919137290815,1.,3.62619537902616));
#43626=CARTESIAN_POINT('Ctrl Pts',(1.07764868137729,-1.,3.61832318504957));
#43627=CARTESIAN_POINT('Ctrl Pts',(1.07764868137729,1.,3.61832318504957));
#43628=CARTESIAN_POINT('Ctrl Pts',(1.07611545402841,-1.,3.61098481349577));
#43629=CARTESIAN_POINT('Ctrl Pts',(1.07611545402841,1.,3.61098481349577));
#43630=CARTESIAN_POINT('Ctrl Pts',(1.0746932716863,-1.,3.6045633988796));
#43631=CARTESIAN_POINT('Ctrl Pts',(1.0746932716863,1.,3.6045633988796));
#43632=CARTESIAN_POINT('Ctrl Pts',(1.0734737254567,-1.,3.59940121154383));
#43633=CARTESIAN_POINT('Ctrl Pts',(1.0734737254567,1.,3.59940121154383));
#43634=CARTESIAN_POINT('Ctrl Pts',(1.07251922679108,-1.,3.59573039611837));
#43635=CARTESIAN_POINT('Ctrl Pts',(1.07251922679108,1.,3.59573039611837));
#43636=CARTESIAN_POINT('Ctrl Pts',(1.07199116987503,-1.,3.59407399103556));
#43637=CARTESIAN_POINT('Ctrl Pts',(1.07199116987503,1.,3.59407399103556));
#43638=CARTESIAN_POINT('Ctrl Pts',(1.07173216219041,-1.,3.59356848057451));
#43639=CARTESIAN_POINT('Ctrl Pts',(1.07173216219041,1.,3.59356848057451));
#43640=CARTESIAN_POINT('Ctrl Pts',(1.07162034256419,-1.,3.59355870577763));
#43641=CARTESIAN_POINT('Ctrl Pts',(1.07162034256419,1.,3.59355870577763));
#43642=CARTESIAN_POINT('Ctrl Pts',(1.07157964745328,-1.,3.59363563249864));
#43643=CARTESIAN_POINT('Ctrl Pts',(1.07157964745328,1.,3.59363563249864));
#43644=CARTESIAN_POINT('',(1.05427041296137,1.,4.06552750530042));
#43645=CARTESIAN_POINT('Ctrl Pts',(1.05427041296137,1.,4.06552750530042));
#43646=CARTESIAN_POINT('Ctrl Pts',(1.05459645194934,1.,4.06398907542679));
#43647=CARTESIAN_POINT('Ctrl Pts',(1.05524507177901,1.,4.06091239150293));
#43648=CARTESIAN_POINT('Ctrl Pts',(1.0562076270849,1.,4.05629789308941));
#43649=CARTESIAN_POINT('Ctrl Pts',(1.05747027728537,1.,4.05014628387112));
#43650=CARTESIAN_POINT('Ctrl Pts',(1.05901393667039,1.,4.04245854429333));
#43651=CARTESIAN_POINT('Ctrl Pts',(1.06052284712114,1.,4.03477261142549));
#43652=CARTESIAN_POINT('Ctrl Pts',(1.06199687787488,1.,4.02708855235732));
#43653=CARTESIAN_POINT('Ctrl Pts',(1.06343586496094,1.,4.0194064749539));
#43654=CARTESIAN_POINT('Ctrl Pts',(1.06483961342894,1.,4.0117265418656));
#43655=CARTESIAN_POINT('Ctrl Pts',(1.06620789963406,1.,4.00404894951804));
#43656=CARTESIAN_POINT('Ctrl Pts',(1.06754047381188,1.,3.99637389919958));
#43657=CARTESIAN_POINT('Ctrl Pts',(1.06883706263912,1.,3.98870156857298));
#43658=CARTESIAN_POINT('Ctrl Pts',(1.07009737257815,1.,3.98103208801289));
#43659=CARTESIAN_POINT('Ctrl Pts',(1.07132109206252,1.,3.97336550222571));
#43660=CARTESIAN_POINT('Ctrl Pts',(1.07250789943095,1.,3.96570179322681));
#43661=CARTESIAN_POINT('Ctrl Pts',(1.07365747426551,1.,3.95804094429606));
#43662=CARTESIAN_POINT('Ctrl Pts',(1.07476950921607,1.,3.95038299600754));
#43663=CARTESIAN_POINT('Ctrl Pts',(1.07584371946428,1.,3.94272809633271));
#43664=CARTESIAN_POINT('Ctrl Pts',(1.07687985975348,1.,3.93507657572743));
#43665=CARTESIAN_POINT('Ctrl Pts',(1.07787771707155,1.,3.92742893349684));
#43666=CARTESIAN_POINT('Ctrl Pts',(1.07883706663524,1.,3.91978568924062));
#43667=CARTESIAN_POINT('Ctrl Pts',(1.0797576350746,1.,3.91214726022096));
#43668=CARTESIAN_POINT('Ctrl Pts',(1.08063906483822,1.,3.90451384092564));
#43669=CARTESIAN_POINT('Ctrl Pts',(1.08148086931373,1.,3.89688525098408));
#43670=CARTESIAN_POINT('Ctrl Pts',(1.08228241999363,1.,3.88926088975182));
#43671=CARTESIAN_POINT('Ctrl Pts',(1.08304304871042,1.,3.88164007721365));
#43672=CARTESIAN_POINT('Ctrl Pts',(1.0837621330751,1.,3.87402233722563));
#43673=CARTESIAN_POINT('Ctrl Pts',(1.08443918607926,1.,3.86640769434269));
#43674=CARTESIAN_POINT('Ctrl Pts',(1.08507395120054,1.,3.85879698702511));
#43675=CARTESIAN_POINT('Ctrl Pts',(1.08566647671838,1.,3.85119211322732));
#43676=CARTESIAN_POINT('Ctrl Pts',(1.08621688337601,1.,3.84359528764934));
#43677=CARTESIAN_POINT('Ctrl Pts',(1.08672515456901,1.,3.83600837071702));
#43678=CARTESIAN_POINT('Ctrl Pts',(1.08719091307558,1.,3.82843215316985));
#43679=CARTESIAN_POINT('Ctrl Pts',(1.08761321539442,1.,3.82086569676321));
#43680=CARTESIAN_POINT('Ctrl Pts',(1.08799030610861,1.,3.81330554446324));
#43681=CARTESIAN_POINT('Ctrl Pts',(1.08832009255378,1.,3.80574726657656));
#43682=CARTESIAN_POINT('Ctrl Pts',(1.08860064435775,1.,3.79818708705252));
#43683=CARTESIAN_POINT('Ctrl Pts',(1.08883071512097,1.,3.79062357974401));
#43684=CARTESIAN_POINT('Ctrl Pts',(1.08901018614638,1.,3.78305911299511));
#43685=CARTESIAN_POINT('Ctrl Pts',(1.08914072791275,1.,3.7755019940944));
#43686=CARTESIAN_POINT('Ctrl Pts',(1.08922484204263,1.,3.76796340094469));
#43687=CARTESIAN_POINT('Ctrl Pts',(1.08926462734287,1.,3.76045342580226));
#43688=CARTESIAN_POINT('Ctrl Pts',(1.08926054632927,1.,3.75297711748138));
#43689=CARTESIAN_POINT('Ctrl Pts',(1.08921040494013,1.,3.74553121371745));
#43690=CARTESIAN_POINT('Ctrl Pts',(1.08910769013288,1.,3.73809879348209));
#43691=CARTESIAN_POINT('Ctrl Pts',(1.08894337390925,1.,3.73065515162949));
#43692=CARTESIAN_POINT('Ctrl Pts',(1.08870887220072,1.,3.72317741369364));
#43693=CARTESIAN_POINT('Ctrl Pts',(1.08839887334776,1.,3.71565372339063));
#43694=CARTESIAN_POINT('Ctrl Pts',(1.0880136731219,1.,3.70809084139476));
#43695=CARTESIAN_POINT('Ctrl Pts',(1.08756311291324,1.,3.70052690909884));
#43696=CARTESIAN_POINT('Ctrl Pts',(1.08706319540291,1.,3.69302062410229));
#43697=CARTESIAN_POINT('Ctrl Pts',(1.08652888882609,1.,3.68562817420864));
#43698=CARTESIAN_POINT('Ctrl Pts',(1.08596755755768,1.,3.67838211685148));
#43699=CARTESIAN_POINT('Ctrl Pts',(1.0853733414448,1.,3.67127347729632));
#43700=CARTESIAN_POINT('Ctrl Pts',(1.0847180992287,1.,3.66422237895256));
#43701=CARTESIAN_POINT('Ctrl Pts',(1.08395671077761,1.,3.65709649161004));
#43702=CARTESIAN_POINT('Ctrl Pts',(1.08304289898577,1.,3.64976441208197));
#43703=CARTESIAN_POINT('Ctrl Pts',(1.08194278850972,1.,3.64214167843595));
#43704=CARTESIAN_POINT('Ctrl Pts',(1.08064765719887,1.,3.63423373196602));
#43705=CARTESIAN_POINT('Ctrl Pts',(1.07919137290815,1.,3.62619537902616));
#43706=CARTESIAN_POINT('Ctrl Pts',(1.07764868137729,1.,3.61832318504957));
#43707=CARTESIAN_POINT('Ctrl Pts',(1.07611545402841,1.,3.61098481349577));
#43708=CARTESIAN_POINT('Ctrl Pts',(1.0746932716863,1.,3.6045633988796));
#43709=CARTESIAN_POINT('Ctrl Pts',(1.0734737254567,1.,3.59940121154383));
#43710=CARTESIAN_POINT('Ctrl Pts',(1.07259084660947,1.,3.59600583195037));
#43711=CARTESIAN_POINT('Ctrl Pts',(1.07209229745284,1.,3.59439597));
#43712=CARTESIAN_POINT('Ctrl Pts',(1.07183575450716,1.,3.59379266874663));
#43713=CARTESIAN_POINT('Ctrl Pts',(1.07171709254271,1.,3.59363512797985));
#43714=CARTESIAN_POINT('Ctrl Pts',(1.071677399622,1.,3.59360648251021));
#43715=CARTESIAN_POINT('',(1.05427041296137,0.,4.06552750530042));
#43716=CARTESIAN_POINT('Ctrl Pts',(0.67669197961156,-1.,3.68843977377012));
#43717=CARTESIAN_POINT('Ctrl Pts',(0.67669197961156,1.,3.68843977377012));
#43718=CARTESIAN_POINT('Ctrl Pts',(0.676620796001989,-1.,3.68838970675497));
#43719=CARTESIAN_POINT('Ctrl Pts',(0.676620796001989,1.,3.68838970675497));
#43720=CARTESIAN_POINT('Ctrl Pts',(0.676525601650855,-1.,3.68844918121303));
#43721=CARTESIAN_POINT('Ctrl Pts',(0.676525601650855,1.,3.68844918121303));
#43722=CARTESIAN_POINT('Ctrl Pts',(0.676524321061226,-1.,3.68901718136181));
#43723=CARTESIAN_POINT('Ctrl Pts',(0.676524321061226,1.,3.68901718136181));
#43724=CARTESIAN_POINT('Ctrl Pts',(0.67680581107509,-1.,3.69073278191994));
#43725=CARTESIAN_POINT('Ctrl Pts',(0.67680581107509,1.,3.69073278191994));
#43726=CARTESIAN_POINT('Ctrl Pts',(0.677621861865497,-1.,3.69443683573598));
#43727=CARTESIAN_POINT('Ctrl Pts',(0.677621861865497,1.,3.69443683573598));
#43728=CARTESIAN_POINT('Ctrl Pts',(0.678878822226026,-1.,3.69959004073005));
#43729=CARTESIAN_POINT('Ctrl Pts',(0.678878822226026,1.,3.69959004073005));
#43730=CARTESIAN_POINT('Ctrl Pts',(0.680526909710876,-1.,3.70595722031785));
#43731=CARTESIAN_POINT('Ctrl Pts',(0.680526909710876,1.,3.70595722031785));
#43732=CARTESIAN_POINT('Ctrl Pts',(0.682492345108929,-1.,3.71319182789943));
#43733=CARTESIAN_POINT('Ctrl Pts',(0.682492345108929,1.,3.71319182789943));
#43734=CARTESIAN_POINT('Ctrl Pts',(0.684691698167848,-1.,3.7209063713926));
#43735=CARTESIAN_POINT('Ctrl Pts',(0.684691698167848,1.,3.7209063713926));
#43736=CARTESIAN_POINT('Ctrl Pts',(0.687043475232354,-1.,3.72872973554051));
#43737=CARTESIAN_POINT('Ctrl Pts',(0.687043475232354,1.,3.72872973554051));
#43738=CARTESIAN_POINT('Ctrl Pts',(0.689479637354813,-1.,3.73636374475077));
#43739=CARTESIAN_POINT('Ctrl Pts',(0.689479637354813,1.,3.73636374475077));
#43740=CARTESIAN_POINT('Ctrl Pts',(0.69196008040082,-1.,3.74365508986712));
#43741=CARTESIAN_POINT('Ctrl Pts',(0.69196008040082,1.,3.74365508986712));
#43742=CARTESIAN_POINT('Ctrl Pts',(0.694474562581492,-1.,3.75060288243455));
#43743=CARTESIAN_POINT('Ctrl Pts',(0.694474562581492,1.,3.75060288243455));
#43744=CARTESIAN_POINT('Ctrl Pts',(0.697031245659743,-1.,3.75729775767023));
#43745=CARTESIAN_POINT('Ctrl Pts',(0.697031245659743,1.,3.75729775767023));
#43746=CARTESIAN_POINT('Ctrl Pts',(0.699648552230917,-1.,3.76387780603759));
#43747=CARTESIAN_POINT('Ctrl Pts',(0.699648552230917,1.,3.76387780603759));
#43748=CARTESIAN_POINT('Ctrl Pts',(0.702346356621551,-1.,3.77048141872872));
#43749=CARTESIAN_POINT('Ctrl Pts',(0.702346356621551,1.,3.77048141872872));
#43750=CARTESIAN_POINT('Ctrl Pts',(0.705135847999816,-1.,3.77719254217129));
#43751=CARTESIAN_POINT('Ctrl Pts',(0.705135847999816,1.,3.77719254217129));
#43752=CARTESIAN_POINT('Ctrl Pts',(0.708015879375459,-1.,3.78402183336605));
#43753=CARTESIAN_POINT('Ctrl Pts',(0.708015879375459,1.,3.78402183336605));
#43754=CARTESIAN_POINT('Ctrl Pts',(0.710978231689016,-1.,3.79093694007094));
#43755=CARTESIAN_POINT('Ctrl Pts',(0.710978231689016,1.,3.79093694007094));
#43756=CARTESIAN_POINT('Ctrl Pts',(0.71401073300664,-1.,3.79788100314975));
#43757=CARTESIAN_POINT('Ctrl Pts',(0.71401073300664,1.,3.79788100314975));
#43758=CARTESIAN_POINT('Ctrl Pts',(0.717100993669114,-1.,3.80479445759309));
#43759=CARTESIAN_POINT('Ctrl Pts',(0.717100993669114,1.,3.80479445759309));
#43760=CARTESIAN_POINT('Ctrl Pts',(0.720240466589236,-1.,3.81163885127344));
#43761=CARTESIAN_POINT('Ctrl Pts',(0.720240466589236,1.,3.81163885127344));
#43762=CARTESIAN_POINT('Ctrl Pts',(0.723426346019422,-1.,3.81840802610835));
#43763=CARTESIAN_POINT('Ctrl Pts',(0.723426346019422,1.,3.81840802610835));
#43764=CARTESIAN_POINT('Ctrl Pts',(0.726659281876663,-1.,3.82511495756713));
#43765=CARTESIAN_POINT('Ctrl Pts',(0.726659281876663,1.,3.82511495756713));
#43766=CARTESIAN_POINT('Ctrl Pts',(0.729942010490167,-1.,3.83178392403383));
#43767=CARTESIAN_POINT('Ctrl Pts',(0.729942010490167,1.,3.83178392403383));
#43768=CARTESIAN_POINT('Ctrl Pts',(0.733277703756078,-1.,3.83844103658009));
#43769=CARTESIAN_POINT('Ctrl Pts',(0.733277703756078,1.,3.83844103658009));
#43770=CARTESIAN_POINT('Ctrl Pts',(0.736668240497117,-1.,3.84510432881213));
#43771=CARTESIAN_POINT('Ctrl Pts',(0.736668240497117,1.,3.84510432881213));
#43772=CARTESIAN_POINT('Ctrl Pts',(0.740113146827137,-1.,3.85177770351216));
#43773=CARTESIAN_POINT('Ctrl Pts',(0.740113146827137,1.,3.85177770351216));
#43774=CARTESIAN_POINT('Ctrl Pts',(0.743610542737012,-1.,3.85845645217594));
#43775=CARTESIAN_POINT('Ctrl Pts',(0.743610542737012,1.,3.85845645217594));
#43776=CARTESIAN_POINT('Ctrl Pts',(0.747157716488871,-1.,3.86513062969889));
#43777=CARTESIAN_POINT('Ctrl Pts',(0.747157716488871,1.,3.86513062969889));
#43778=CARTESIAN_POINT('Ctrl Pts',(0.750751822383027,-1.,3.87178914078374));
#43779=CARTESIAN_POINT('Ctrl Pts',(0.750751822383027,1.,3.87178914078374));
#43780=CARTESIAN_POINT('Ctrl Pts',(0.754390577396856,-1.,3.87842382520065));
#43781=CARTESIAN_POINT('Ctrl Pts',(0.754390577396856,1.,3.87842382520065));
#43782=CARTESIAN_POINT('Ctrl Pts',(0.758072800564801,-1.,3.88503262662689));
#43783=CARTESIAN_POINT('Ctrl Pts',(0.758072800564801,1.,3.88503262662689));
#43784=CARTESIAN_POINT('Ctrl Pts',(0.761798028793969,-1.,3.89161738162245));
#43785=CARTESIAN_POINT('Ctrl Pts',(0.761798028793969,1.,3.89161738162245));
#43786=CARTESIAN_POINT('Ctrl Pts',(0.765566256401295,-1.,3.89818233104378));
#43787=CARTESIAN_POINT('Ctrl Pts',(0.765566256401295,1.,3.89818233104378));
#43788=CARTESIAN_POINT('Ctrl Pts',(0.769377629847873,-1.,3.90473237182633));
#43789=CARTESIAN_POINT('Ctrl Pts',(0.769377629847873,1.,3.90473237182633));
#43790=CARTESIAN_POINT('Ctrl Pts',(0.77323215450632,-1.,3.91127138115243));
#43791=CARTESIAN_POINT('Ctrl Pts',(0.77323215450632,1.,3.91127138115243));
#43792=CARTESIAN_POINT('Ctrl Pts',(0.777129415664956,-1.,3.9178006233448));
#43793=CARTESIAN_POINT('Ctrl Pts',(0.777129415664956,1.,3.9178006233448));
#43794=CARTESIAN_POINT('Ctrl Pts',(0.781068718228451,-1.,3.92431956510441));
#43795=CARTESIAN_POINT('Ctrl Pts',(0.781068718228451,1.,3.92431956510441));
#43796=CARTESIAN_POINT('Ctrl Pts',(0.785049202786507,-1.,3.93082655631789));
#43797=CARTESIAN_POINT('Ctrl Pts',(0.785049202786507,1.,3.93082655631789));
#43798=CARTESIAN_POINT('Ctrl Pts',(0.789069971469332,-1.,3.93731956885676));
#43799=CARTESIAN_POINT('Ctrl Pts',(0.789069971469332,1.,3.93731956885676));
#43800=CARTESIAN_POINT('Ctrl Pts',(0.79313020564096,-1.,3.94379688971283));
#43801=CARTESIAN_POINT('Ctrl Pts',(0.79313020564096,1.,3.94379688971283));
#43802=CARTESIAN_POINT('Ctrl Pts',(0.797229296085315,-1.,3.95025788827136));
#43803=CARTESIAN_POINT('Ctrl Pts',(0.797229296085315,1.,3.95025788827136));
#43804=CARTESIAN_POINT('Ctrl Pts',(0.801366797727049,-1.,3.95670276375108));
#43805=CARTESIAN_POINT('Ctrl Pts',(0.801366797727049,1.,3.95670276375108));
#43806=CARTESIAN_POINT('Ctrl Pts',(0.805542372178361,-1.,3.96313222295815));
#43807=CARTESIAN_POINT('Ctrl Pts',(0.805542372178361,1.,3.96313222295815));
#43808=CARTESIAN_POINT('Ctrl Pts',(0.80975573281809,-1.,3.96954717513232));
#43809=CARTESIAN_POINT('Ctrl Pts',(0.80975573281809,1.,3.96954717513232));
#43810=CARTESIAN_POINT('Ctrl Pts',(0.814006592328843,-1.,3.97594844078811));
#43811=CARTESIAN_POINT('Ctrl Pts',(0.814006592328843,1.,3.97594844078811));
#43812=CARTESIAN_POINT('Ctrl Pts',(0.818294599022293,-1.,3.98233640155404));
#43813=CARTESIAN_POINT('Ctrl Pts',(0.818294599022293,1.,3.98233640155404));
#43814=CARTESIAN_POINT('Ctrl Pts',(0.822619346022118,-1.,3.98871104646485));
#43815=CARTESIAN_POINT('Ctrl Pts',(0.822619346022118,1.,3.98871104646485));
#43816=CARTESIAN_POINT('Ctrl Pts',(0.826980400320789,-1.,3.99507212784431));
#43817=CARTESIAN_POINT('Ctrl Pts',(0.826980400320789,1.,3.99507212784431));
#43818=CARTESIAN_POINT('Ctrl Pts',(0.831377325741622,-1.,4.00141928477507));
#43819=CARTESIAN_POINT('Ctrl Pts',(0.831377325741622,1.,4.00141928477507));
#43820=CARTESIAN_POINT('Ctrl Pts',(0.835809705809645,-1.,4.00775216907856));
#43821=CARTESIAN_POINT('Ctrl Pts',(0.835809705809645,1.,4.00775216907856));
#43822=CARTESIAN_POINT('Ctrl Pts',(0.840277171975854,-1.,4.01407059766103));
#43823=CARTESIAN_POINT('Ctrl Pts',(0.840277171975854,1.,4.01407059766103));
#43824=CARTESIAN_POINT('Ctrl Pts',(0.844779403287745,-1.,4.02037456798441));
#43825=CARTESIAN_POINT('Ctrl Pts',(0.844779403287745,1.,4.02037456798441));
#43826=CARTESIAN_POINT('Ctrl Pts',(0.849316107474244,-1.,4.02666418343164));
#43827=CARTESIAN_POINT('Ctrl Pts',(0.849316107474244,1.,4.02666418343164));
#43828=CARTESIAN_POINT('Ctrl Pts',(0.853887006631755,-1.,4.03293960436756));
#43829=CARTESIAN_POINT('Ctrl Pts',(0.853887006631755,1.,4.03293960436756));
#43830=CARTESIAN_POINT('Ctrl Pts',(0.858491822322827,-1.,4.03920099284773));
#43831=CARTESIAN_POINT('Ctrl Pts',(0.858491822322827,1.,4.03920099284773));
#43832=CARTESIAN_POINT('Ctrl Pts',(0.863130256643258,-1.,4.04544845048584));
#43833=CARTESIAN_POINT('Ctrl Pts',(0.863130256643258,1.,4.04544845048584));
#43834=CARTESIAN_POINT('Ctrl Pts',(0.867801988859917,-1.,4.05168199437909));
#43835=CARTESIAN_POINT('Ctrl Pts',(0.867801988859917,1.,4.05168199437909));
#43836=CARTESIAN_POINT('Ctrl Pts',(0.872506694782446,-1.,4.0579015903134));
#43837=CARTESIAN_POINT('Ctrl Pts',(0.872506694782446,1.,4.0579015903134));
#43838=CARTESIAN_POINT('Ctrl Pts',(0.877244060485837,-1.,4.06410717232905));
#43839=CARTESIAN_POINT('Ctrl Pts',(0.877244060485837,1.,4.06410717232905));
#43840=CARTESIAN_POINT('Ctrl Pts',(0.882013797525691,-1.,4.07029866694192));
#43841=CARTESIAN_POINT('Ctrl Pts',(0.882013797525691,1.,4.07029866694192));
#43842=CARTESIAN_POINT('Ctrl Pts',(0.886815658358501,-1.,4.07647601773635));
#43843=CARTESIAN_POINT('Ctrl Pts',(0.886815658358501,1.,4.07647601773635));
#43844=CARTESIAN_POINT('Ctrl Pts',(0.891649447916277,-1.,4.08263920304799));
#43845=CARTESIAN_POINT('Ctrl Pts',(0.891649447916277,1.,4.08263920304799));
#43846=CARTESIAN_POINT('Ctrl Pts',(0.896515019231333,-1.,4.08878822246833));
#43847=CARTESIAN_POINT('Ctrl Pts',(0.896515019231333,1.,4.08878822246833));
#43848=CARTESIAN_POINT('Ctrl Pts',(0.900432820941674,-1.,4.09369611522387));
#43849=CARTESIAN_POINT('Ctrl Pts',(0.900432820941674,1.,4.09369611522387));
#43850=CARTESIAN_POINT('Ctrl Pts',(0.903385402441587,-1.,4.09737067245935));
#43851=CARTESIAN_POINT('Ctrl Pts',(0.903385402441587,1.,4.09737067245935));
#43852=CARTESIAN_POINT('Ctrl Pts',(0.905360112215337,-1.,4.09981755067523));
#43853=CARTESIAN_POINT('Ctrl Pts',(0.905360112215337,1.,4.09981755067523));
#43854=CARTESIAN_POINT('Ctrl Pts',(0.906349047628865,-1.,4.10104028313088));
#43855=CARTESIAN_POINT('Ctrl Pts',(0.906349047628865,1.,4.10104028313088));
#43856=CARTESIAN_POINT('',(0.676591647975428,1.,3.68845817949586));
#43857=CARTESIAN_POINT('Ctrl Pts',(0.676591647975428,-1.,3.68845817949586));
#43858=CARTESIAN_POINT('Ctrl Pts',(0.676591647975428,-0.666666666666667,
3.68845817949586));
#43859=CARTESIAN_POINT('Ctrl Pts',(0.676591647975428,-0.333333333333333,
3.68845817949586));
#43860=CARTESIAN_POINT('Ctrl Pts',(0.676591647975428,0.333333333333333,
3.68845817949586));
#43861=CARTESIAN_POINT('Ctrl Pts',(0.676591647975428,0.666666666666667,
3.68845817949586));
#43862=CARTESIAN_POINT('Ctrl Pts',(0.676591647975428,1.,3.68845817949586));
#43863=CARTESIAN_POINT('',(0.906349047628865,1.,4.10104028313088));
#43864=CARTESIAN_POINT('',(0.906349047628865,0.,4.10104028313088));
#43865=CARTESIAN_POINT('Ctrl Pts',(0.676591647975428,1.,3.68845817949586));
#43866=CARTESIAN_POINT('Ctrl Pts',(0.676569286094606,1.,3.68850172300477));
#43867=CARTESIAN_POINT('Ctrl Pts',(0.676535079520806,1.,3.68869596425969));
#43868=CARTESIAN_POINT('Ctrl Pts',(0.676580391119396,1.,3.68934997767243));
#43869=CARTESIAN_POINT('Ctrl Pts',(0.676867042599401,1.,3.69101071175464));
#43870=CARTESIAN_POINT('Ctrl Pts',(0.677621861865497,1.,3.69443683573598));
#43871=CARTESIAN_POINT('Ctrl Pts',(0.678878822226026,1.,3.69959004073005));
#43872=CARTESIAN_POINT('Ctrl Pts',(0.680526909710876,1.,3.70595722031785));
#43873=CARTESIAN_POINT('Ctrl Pts',(0.682492345108929,1.,3.71319182789943));
#43874=CARTESIAN_POINT('Ctrl Pts',(0.684691698167848,1.,3.7209063713926));
#43875=CARTESIAN_POINT('Ctrl Pts',(0.687043475232354,1.,3.72872973554051));
#43876=CARTESIAN_POINT('Ctrl Pts',(0.689479637354813,1.,3.73636374475077));
#43877=CARTESIAN_POINT('Ctrl Pts',(0.69196008040082,1.,3.74365508986712));
#43878=CARTESIAN_POINT('Ctrl Pts',(0.694474562581492,1.,3.75060288243455));
#43879=CARTESIAN_POINT('Ctrl Pts',(0.697031245659743,1.,3.75729775767023));
#43880=CARTESIAN_POINT('Ctrl Pts',(0.699648552230917,1.,3.76387780603759));
#43881=CARTESIAN_POINT('Ctrl Pts',(0.702346356621551,1.,3.77048141872872));
#43882=CARTESIAN_POINT('Ctrl Pts',(0.705135847999816,1.,3.77719254217129));
#43883=CARTESIAN_POINT('Ctrl Pts',(0.708015879375459,1.,3.78402183336605));
#43884=CARTESIAN_POINT('Ctrl Pts',(0.710978231689016,1.,3.79093694007094));
#43885=CARTESIAN_POINT('Ctrl Pts',(0.71401073300664,1.,3.79788100314975));
#43886=CARTESIAN_POINT('Ctrl Pts',(0.717100993669114,1.,3.80479445759309));
#43887=CARTESIAN_POINT('Ctrl Pts',(0.720240466589236,1.,3.81163885127344));
#43888=CARTESIAN_POINT('Ctrl Pts',(0.723426346019422,1.,3.81840802610835));
#43889=CARTESIAN_POINT('Ctrl Pts',(0.726659281876663,1.,3.82511495756713));
#43890=CARTESIAN_POINT('Ctrl Pts',(0.729942010490167,1.,3.83178392403383));
#43891=CARTESIAN_POINT('Ctrl Pts',(0.733277703756078,1.,3.83844103658009));
#43892=CARTESIAN_POINT('Ctrl Pts',(0.736668240497117,1.,3.84510432881213));
#43893=CARTESIAN_POINT('Ctrl Pts',(0.740113146827137,1.,3.85177770351216));
#43894=CARTESIAN_POINT('Ctrl Pts',(0.743610542737012,1.,3.85845645217594));
#43895=CARTESIAN_POINT('Ctrl Pts',(0.747157716488871,1.,3.86513062969889));
#43896=CARTESIAN_POINT('Ctrl Pts',(0.750751822383027,1.,3.87178914078374));
#43897=CARTESIAN_POINT('Ctrl Pts',(0.754390577396856,1.,3.87842382520065));
#43898=CARTESIAN_POINT('Ctrl Pts',(0.758072800564801,1.,3.88503262662689));
#43899=CARTESIAN_POINT('Ctrl Pts',(0.761798028793969,1.,3.89161738162245));
#43900=CARTESIAN_POINT('Ctrl Pts',(0.765566256401295,1.,3.89818233104378));
#43901=CARTESIAN_POINT('Ctrl Pts',(0.769377629847873,1.,3.90473237182633));
#43902=CARTESIAN_POINT('Ctrl Pts',(0.77323215450632,1.,3.91127138115243));
#43903=CARTESIAN_POINT('Ctrl Pts',(0.777129415664956,1.,3.9178006233448));
#43904=CARTESIAN_POINT('Ctrl Pts',(0.781068718228451,1.,3.92431956510441));
#43905=CARTESIAN_POINT('Ctrl Pts',(0.785049202786507,1.,3.93082655631789));
#43906=CARTESIAN_POINT('Ctrl Pts',(0.789069971469332,1.,3.93731956885676));
#43907=CARTESIAN_POINT('Ctrl Pts',(0.79313020564096,1.,3.94379688971283));
#43908=CARTESIAN_POINT('Ctrl Pts',(0.797229296085315,1.,3.95025788827136));
#43909=CARTESIAN_POINT('Ctrl Pts',(0.801366797727049,1.,3.95670276375108));
#43910=CARTESIAN_POINT('Ctrl Pts',(0.805542372178361,1.,3.96313222295815));
#43911=CARTESIAN_POINT('Ctrl Pts',(0.80975573281809,1.,3.96954717513232));
#43912=CARTESIAN_POINT('Ctrl Pts',(0.814006592328843,1.,3.97594844078811));
#43913=CARTESIAN_POINT('Ctrl Pts',(0.818294599022293,1.,3.98233640155404));
#43914=CARTESIAN_POINT('Ctrl Pts',(0.822619346022118,1.,3.98871104646485));
#43915=CARTESIAN_POINT('Ctrl Pts',(0.826980400320789,1.,3.99507212784431));
#43916=CARTESIAN_POINT('Ctrl Pts',(0.831377325741622,1.,4.00141928477507));
#43917=CARTESIAN_POINT('Ctrl Pts',(0.835809705809645,1.,4.00775216907856));
#43918=CARTESIAN_POINT('Ctrl Pts',(0.840277171975854,1.,4.01407059766103));
#43919=CARTESIAN_POINT('Ctrl Pts',(0.844779403287745,1.,4.02037456798441));
#43920=CARTESIAN_POINT('Ctrl Pts',(0.849316107474244,1.,4.02666418343164));
#43921=CARTESIAN_POINT('Ctrl Pts',(0.853887006631755,1.,4.03293960436756));
#43922=CARTESIAN_POINT('Ctrl Pts',(0.858491822322827,1.,4.03920099284773));
#43923=CARTESIAN_POINT('Ctrl Pts',(0.863130256643258,1.,4.04544845048584));
#43924=CARTESIAN_POINT('Ctrl Pts',(0.867801988859917,1.,4.05168199437909));
#43925=CARTESIAN_POINT('Ctrl Pts',(0.872506694782446,1.,4.0579015903134));
#43926=CARTESIAN_POINT('Ctrl Pts',(0.877244060485837,1.,4.06410717232905));
#43927=CARTESIAN_POINT('Ctrl Pts',(0.882013797525691,1.,4.07029866694192));
#43928=CARTESIAN_POINT('Ctrl Pts',(0.886815658358501,1.,4.07647601773635));
#43929=CARTESIAN_POINT('Ctrl Pts',(0.891649447916277,1.,4.08263920304799));
#43930=CARTESIAN_POINT('Ctrl Pts',(0.896515019231333,1.,4.08878822246833));
#43931=CARTESIAN_POINT('Ctrl Pts',(0.900432820941674,1.,4.09369611522387));
#43932=CARTESIAN_POINT('Ctrl Pts',(0.903385402441587,1.,4.09737067245935));
#43933=CARTESIAN_POINT('Ctrl Pts',(0.905360112215337,1.,4.09981755067523));
#43934=CARTESIAN_POINT('Ctrl Pts',(0.906349047628865,1.,4.10104028313088));
#43935=CARTESIAN_POINT('Origin',(0.906349047628865,0.,4.10104028313088));
#43936=CARTESIAN_POINT('',(1.05427041296137,1.,4.06552750530042));
#43937=CARTESIAN_POINT('Origin',(0.,0.,0.));
#43938=CARTESIAN_POINT('',(0.496319364829374,1.,3.71701050416802));
#43939=CARTESIAN_POINT('Origin',(0.,1.,0.));
#43940=CARTESIAN_POINT('Ctrl Pts',(0.496319364829373,1.,3.71701050416802));
#43941=CARTESIAN_POINT('Ctrl Pts',(0.496319364829373,0.666666666666667,
3.71701050416802));
#43942=CARTESIAN_POINT('Ctrl Pts',(0.496319364829373,0.333333333333333,
3.71701050416802));
#43943=CARTESIAN_POINT('Ctrl Pts',(0.496319364829373,-0.333333333333333,
3.71701050416802));
#43944=CARTESIAN_POINT('Ctrl Pts',(0.496319364829373,-0.666666666666667,
3.71701050416802));
#43945=CARTESIAN_POINT('Ctrl Pts',(0.496319364829373,-1.,3.71701050416802));
#43946=CARTESIAN_POINT('Ctrl Pts',(0.405301974318349,-1.,4.18039834341342));
#43947=CARTESIAN_POINT('Ctrl Pts',(0.405301974318349,1.,4.18039834341342));
#43948=CARTESIAN_POINT('Ctrl Pts',(0.40586466267963,-1.,4.17892985789908));
#43949=CARTESIAN_POINT('Ctrl Pts',(0.40586466267963,1.,4.17892985789908));
#43950=CARTESIAN_POINT('Ctrl Pts',(0.406986596326602,-1.,4.17599251955585));
#43951=CARTESIAN_POINT('Ctrl Pts',(0.406986596326602,1.,4.17599251955585));
#43952=CARTESIAN_POINT('Ctrl Pts',(0.408659167570152,-1.,4.17158541009947));
#43953=CARTESIAN_POINT('Ctrl Pts',(0.408659167570152,1.,4.17158541009947));
#43954=CARTESIAN_POINT('Ctrl Pts',(0.410868596148613,-1.,4.16570705940731));
#43955=CARTESIAN_POINT('Ctrl Pts',(0.410868596148613,1.,4.16570705940731));
#43956=CARTESIAN_POINT('Ctrl Pts',(0.413595877953268,-1.,4.1583554501909));
#43957=CARTESIAN_POINT('Ctrl Pts',(0.413595877953268,1.,4.1583554501909));
#43958=CARTESIAN_POINT('Ctrl Pts',(0.416288556008986,-1.,4.15100018950989));
#43959=CARTESIAN_POINT('Ctrl Pts',(0.416288556008986,1.,4.15100018950989));
#43960=CARTESIAN_POINT('Ctrl Pts',(0.418946490667799,-1.,4.14364132317223));
#43961=CARTESIAN_POINT('Ctrl Pts',(0.418946490667799,1.,4.14364132317223));
#43962=CARTESIAN_POINT('Ctrl Pts',(0.421569503103971,-1.,4.13627893206433));
#43963=CARTESIAN_POINT('Ctrl Pts',(0.421569503103971,1.,4.13627893206433));
#43964=CARTESIAN_POINT('Ctrl Pts',(0.424157375323155,-1.,4.1289131463371));
#43965=CARTESIAN_POINT('Ctrl Pts',(0.424157375323155,1.,4.1289131463371));
#43966=CARTESIAN_POINT('Ctrl Pts',(0.426709855706242,-1.,4.1215441250121));
#43967=CARTESIAN_POINT('Ctrl Pts',(0.426709855706242,1.,4.1215441250121));
#43968=CARTESIAN_POINT('Ctrl Pts',(0.429226666075372,-1.,4.1141720278277));
#43969=CARTESIAN_POINT('Ctrl Pts',(0.429226666075372,1.,4.1141720278277));
#43970=CARTESIAN_POINT('Ctrl Pts',(0.431707508679771,-1.,4.10679698750219));
#43971=CARTESIAN_POINT('Ctrl Pts',(0.431707508679771,1.,4.10679698750219));
#43972=CARTESIAN_POINT('Ctrl Pts',(0.434152073200642,-1.,4.09941908688567));
#43973=CARTESIAN_POINT('Ctrl Pts',(0.434152073200642,1.,4.09941908688567));
#43974=CARTESIAN_POINT('Ctrl Pts',(0.436560044913814,-1.,4.09203832139439));
#43975=CARTESIAN_POINT('Ctrl Pts',(0.436560044913814,1.,4.09203832139439));
#43976=CARTESIAN_POINT('Ctrl Pts',(0.438931108931613,-1.,4.08465462294625));
#43977=CARTESIAN_POINT('Ctrl Pts',(0.438931108931613,1.,4.08465462294625));
#43978=CARTESIAN_POINT('Ctrl Pts',(0.441264951396587,-1.,4.07726792490256));
#43979=CARTESIAN_POINT('Ctrl Pts',(0.441264951396587,1.,4.07726792490256));
#43980=CARTESIAN_POINT('Ctrl Pts',(0.443561262395407,-1.,4.0698782192577));
#43981=CARTESIAN_POINT('Ctrl Pts',(0.443561262395407,1.,4.0698782192577));
#43982=CARTESIAN_POINT('Ctrl Pts',(0.445819737468477,-1.,4.06248560760596));
#43983=CARTESIAN_POINT('Ctrl Pts',(0.445819737468477,1.,4.06248560760596));
#43984=CARTESIAN_POINT('Ctrl Pts',(0.448040082683976,-1.,4.05509037796815));
#43985=CARTESIAN_POINT('Ctrl Pts',(0.448040082683976,1.,4.05509037796815));
#43986=CARTESIAN_POINT('Ctrl Pts',(0.450222009543773,-1.,4.0476929901797));
#43987=CARTESIAN_POINT('Ctrl Pts',(0.450222009543773,1.,4.0476929901797));
#43988=CARTESIAN_POINT('Ctrl Pts',(0.452365214748778,-1.,4.0402939222793));
#43989=CARTESIAN_POINT('Ctrl Pts',(0.452365214748778,1.,4.0402939222793));
#43990=CARTESIAN_POINT('Ctrl Pts',(0.454469363020495,-1.,4.03289354362745));
#43991=CARTESIAN_POINT('Ctrl Pts',(0.454469363020495,1.,4.03289354362745));
#43992=CARTESIAN_POINT('Ctrl Pts',(0.456534070784968,-1.,4.02549199038414));
#43993=CARTESIAN_POINT('Ctrl Pts',(0.456534070784968,1.,4.02549199038414));
#43994=CARTESIAN_POINT('Ctrl Pts',(0.458558885637,-1.,4.01808900827647));
#43995=CARTESIAN_POINT('Ctrl Pts',(0.458558885637,1.,4.01808900827647));
#43996=CARTESIAN_POINT('Ctrl Pts',(0.460543280768577,-1.,4.01068390573469));
#43997=CARTESIAN_POINT('Ctrl Pts',(0.460543280768577,1.,4.01068390573469));
#43998=CARTESIAN_POINT('Ctrl Pts',(0.462486702616251,-1.,4.00327590659129));
#43999=CARTESIAN_POINT('Ctrl Pts',(0.462486702616251,1.,4.00327590659129));
#44000=CARTESIAN_POINT('Ctrl Pts',(0.464388610938994,-1.,3.99586444320135));
#44001=CARTESIAN_POINT('Ctrl Pts',(0.464388610938994,1.,3.99586444320135));
#44002=CARTESIAN_POINT('Ctrl Pts',(0.466248520883034,-1.,3.98844946363258));
#44003=CARTESIAN_POINT('Ctrl Pts',(0.466248520883034,1.,3.98844946363258));
#44004=CARTESIAN_POINT('Ctrl Pts',(0.468066047920139,-1.,3.98103175589349));
#44005=CARTESIAN_POINT('Ctrl Pts',(0.468066047920139,1.,3.98103175589349));
#44006=CARTESIAN_POINT('Ctrl Pts',(0.469840942829878,-1.,3.97361320212413));
#44007=CARTESIAN_POINT('Ctrl Pts',(0.469840942829878,1.,3.97361320212413));
#44008=CARTESIAN_POINT('Ctrl Pts',(0.471572978413493,-1.,3.96619600864626));
#44009=CARTESIAN_POINT('Ctrl Pts',(0.471572978413493,1.,3.96619600864626));
#44010=CARTESIAN_POINT('Ctrl Pts',(0.473261847236295,-1.,3.95878201038332));
#44011=CARTESIAN_POINT('Ctrl Pts',(0.473261847236295,1.,3.95878201038332));
#44012=CARTESIAN_POINT('Ctrl Pts',(0.47490705302179,-1.,3.95137192932898));
#44013=CARTESIAN_POINT('Ctrl Pts',(0.47490705302179,1.,3.95137192932898));
#44014=CARTESIAN_POINT('Ctrl Pts',(0.476507810658534,-1.,3.94396469119385));
#44015=CARTESIAN_POINT('Ctrl Pts',(0.476507810658534,1.,3.94396469119385));
#44016=CARTESIAN_POINT('Ctrl Pts',(0.478062927140957,-1.,3.93655660689819));
#44017=CARTESIAN_POINT('Ctrl Pts',(0.478062927140957,1.,3.93655660689819));
#44018=CARTESIAN_POINT('Ctrl Pts',(0.479571028525565,-1.,3.92914297392067));
#44019=CARTESIAN_POINT('Ctrl Pts',(0.479571028525565,1.,3.92914297392067));
#44020=CARTESIAN_POINT('Ctrl Pts',(0.481030798910735,-1.,3.92171976072334));
#44021=CARTESIAN_POINT('Ctrl Pts',(0.481030798910735,1.,3.92171976072334));
#44022=CARTESIAN_POINT('Ctrl Pts',(0.482441230340708,-1.,3.91428536373749));
#44023=CARTESIAN_POINT('Ctrl Pts',(0.482441230340708,1.,3.91428536373749));
#44024=CARTESIAN_POINT('Ctrl Pts',(0.48380183508916,-1.,3.90684210358063));
#44025=CARTESIAN_POINT('Ctrl Pts',(0.48380183508916,1.,3.90684210358063));
#44026=CARTESIAN_POINT('Ctrl Pts',(0.485112963522245,-1.,3.89939844658529));
#44027=CARTESIAN_POINT('Ctrl Pts',(0.485112963522245,1.,3.89939844658529));
#44028=CARTESIAN_POINT('Ctrl Pts',(0.486375337854133,-1.,3.89196582437574));
#44029=CARTESIAN_POINT('Ctrl Pts',(0.486375337854133,1.,3.89196582437574));
#44030=CARTESIAN_POINT('Ctrl Pts',(0.487589452275179,-1.,3.88455453328156));
#44031=CARTESIAN_POINT('Ctrl Pts',(0.487589452275179,1.,3.88455453328156));
#44032=CARTESIAN_POINT('Ctrl Pts',(0.488754973798281,-1.,3.87716963231115));
#44033=CARTESIAN_POINT('Ctrl Pts',(0.488754973798281,1.,3.87716963231115));
#44034=CARTESIAN_POINT('Ctrl Pts',(0.489870245704899,-1.,3.86980755613694));
#44035=CARTESIAN_POINT('Ctrl Pts',(0.489870245704899,1.,3.86980755613694));
#44036=CARTESIAN_POINT('Ctrl Pts',(0.490931482170849,-1.,3.86245057319215));
#44037=CARTESIAN_POINT('Ctrl Pts',(0.490931482170849,1.,3.86245057319215));
#44038=CARTESIAN_POINT('Ctrl Pts',(0.49193363108376,-1.,3.85507287020223));
#44039=CARTESIAN_POINT('Ctrl Pts',(0.49193363108376,1.,3.85507287020223));
#44040=CARTESIAN_POINT('Ctrl Pts',(0.492871792414095,-1.,3.84765051147965));
#44041=CARTESIAN_POINT('Ctrl Pts',(0.492871792414095,1.,3.84765051147965));
#44042=CARTESIAN_POINT('Ctrl Pts',(0.493742574629117,-1.,3.84017095578438));
#44043=CARTESIAN_POINT('Ctrl Pts',(0.493742574629117,1.,3.84017095578438));
#44044=CARTESIAN_POINT('Ctrl Pts',(0.494545212256425,-1.,3.8326409268245));
#44045=CARTESIAN_POINT('Ctrl Pts',(0.494545212256425,1.,3.8326409268245));
#44046=CARTESIAN_POINT('Ctrl Pts',(0.495283458893903,-1.,3.82509963594156));
#44047=CARTESIAN_POINT('Ctrl Pts',(0.495283458893903,1.,3.82509963594156));
#44048=CARTESIAN_POINT('Ctrl Pts',(0.495963937875571,-1.,3.81760756144099));
#44049=CARTESIAN_POINT('Ctrl Pts',(0.495963937875571,1.,3.81760756144099));
#44050=CARTESIAN_POINT('Ctrl Pts',(0.496592643443789,-1.,3.81022254090909));
#44051=CARTESIAN_POINT('Ctrl Pts',(0.496592643443789,1.,3.81022254090909));
#44052=CARTESIAN_POINT('Ctrl Pts',(0.49717175620109,-1.,3.80297788298545));
#44053=CARTESIAN_POINT('Ctrl Pts',(0.49717175620109,1.,3.80297788298545));
#44054=CARTESIAN_POINT('Ctrl Pts',(0.49769689210058,-1.,3.79586380669959));
#44055=CARTESIAN_POINT('Ctrl Pts',(0.49769689210058,1.,3.79586380669959));
#44056=CARTESIAN_POINT('Ctrl Pts',(0.498152751800819,-1.,3.78879701661152));
#44057=CARTESIAN_POINT('Ctrl Pts',(0.498152751800819,1.,3.78879701661152));
#44058=CARTESIAN_POINT('Ctrl Pts',(0.498515471679378,-1.,3.78163975337189));
#44059=CARTESIAN_POINT('Ctrl Pts',(0.498515471679378,1.,3.78163975337189));
#44060=CARTESIAN_POINT('Ctrl Pts',(0.498759900365686,-1.,3.77425499225089));
#44061=CARTESIAN_POINT('Ctrl Pts',(0.498759900365686,1.,3.77425499225089));
#44062=CARTESIAN_POINT('Ctrl Pts',(0.498865792335185,-1.,3.76655401191144));
#44063=CARTESIAN_POINT('Ctrl Pts',(0.498865792335185,1.,3.76655401191144));
#44064=CARTESIAN_POINT('Ctrl Pts',(0.498823681615513,-1.,3.75854082221127));
#44065=CARTESIAN_POINT('Ctrl Pts',(0.498823681615513,1.,3.75854082221127));
#44066=CARTESIAN_POINT('Ctrl Pts',(0.498642802042929,-1.,3.75037362168103));
#44067=CARTESIAN_POINT('Ctrl Pts',(0.498642802042929,1.,3.75037362168103));
#44068=CARTESIAN_POINT('Ctrl Pts',(0.498350586058176,-1.,3.74235701735109));
#44069=CARTESIAN_POINT('Ctrl Pts',(0.498350586058176,1.,3.74235701735109));
#44070=CARTESIAN_POINT('Ctrl Pts',(0.497984209510495,-1.,3.73486914372834));
#44071=CARTESIAN_POINT('Ctrl Pts',(0.497984209510495,1.,3.73486914372834));
#44072=CARTESIAN_POINT('Ctrl Pts',(0.497584067153279,-1.,3.72830430904794));
#44073=CARTESIAN_POINT('Ctrl Pts',(0.497584067153279,1.,3.72830430904794));
#44074=CARTESIAN_POINT('Ctrl Pts',(0.497187079575794,-1.,3.72301489774241));
#44075=CARTESIAN_POINT('Ctrl Pts',(0.497187079575794,1.,3.72301489774241));
#44076=CARTESIAN_POINT('Ctrl Pts',(0.496818574419988,-1.,3.71923995965807));
#44077=CARTESIAN_POINT('Ctrl Pts',(0.496818574419988,1.,3.71923995965807));
#44078=CARTESIAN_POINT('Ctrl Pts',(0.496556137603856,-1.,3.71752134136931));
#44079=CARTESIAN_POINT('Ctrl Pts',(0.496556137603856,1.,3.71752134136931));
#44080=CARTESIAN_POINT('Ctrl Pts',(0.496379397992181,-1.,3.71698153685229));
#44081=CARTESIAN_POINT('Ctrl Pts',(0.496379397992181,1.,3.71698153685229));
#44082=CARTESIAN_POINT('Ctrl Pts',(0.496270484166233,-1.,3.71695438995598));
#44083=CARTESIAN_POINT('Ctrl Pts',(0.496270484166233,1.,3.71695438995598));
#44084=CARTESIAN_POINT('Ctrl Pts',(0.496218256089211,-1.,3.71702400346349));
#44085=CARTESIAN_POINT('Ctrl Pts',(0.496218256089211,1.,3.71702400346349));
#44086=CARTESIAN_POINT('',(0.405301974318349,1.,4.18039834341342));
#44087=CARTESIAN_POINT('Ctrl Pts',(0.405301974318349,1.,4.18039834341342));
#44088=CARTESIAN_POINT('Ctrl Pts',(0.40586466267963,1.,4.17892985789908));
#44089=CARTESIAN_POINT('Ctrl Pts',(0.406986596326602,1.,4.17599251955585));
#44090=CARTESIAN_POINT('Ctrl Pts',(0.408659167570152,1.,4.17158541009947));
#44091=CARTESIAN_POINT('Ctrl Pts',(0.410868596148613,1.,4.16570705940731));
#44092=CARTESIAN_POINT('Ctrl Pts',(0.413595877953268,1.,4.1583554501909));
#44093=CARTESIAN_POINT('Ctrl Pts',(0.416288556008986,1.,4.15100018950989));
#44094=CARTESIAN_POINT('Ctrl Pts',(0.418946490667799,1.,4.14364132317223));
#44095=CARTESIAN_POINT('Ctrl Pts',(0.421569503103971,1.,4.13627893206433));
#44096=CARTESIAN_POINT('Ctrl Pts',(0.424157375323155,1.,4.1289131463371));
#44097=CARTESIAN_POINT('Ctrl Pts',(0.426709855706242,1.,4.1215441250121));
#44098=CARTESIAN_POINT('Ctrl Pts',(0.429226666075372,1.,4.1141720278277));
#44099=CARTESIAN_POINT('Ctrl Pts',(0.431707508679771,1.,4.10679698750219));
#44100=CARTESIAN_POINT('Ctrl Pts',(0.434152073200642,1.,4.09941908688567));
#44101=CARTESIAN_POINT('Ctrl Pts',(0.436560044913814,1.,4.09203832139439));
#44102=CARTESIAN_POINT('Ctrl Pts',(0.438931108931613,1.,4.08465462294625));
#44103=CARTESIAN_POINT('Ctrl Pts',(0.441264951396587,1.,4.07726792490256));
#44104=CARTESIAN_POINT('Ctrl Pts',(0.443561262395407,1.,4.0698782192577));
#44105=CARTESIAN_POINT('Ctrl Pts',(0.445819737468477,1.,4.06248560760596));
#44106=CARTESIAN_POINT('Ctrl Pts',(0.448040082683976,1.,4.05509037796815));
#44107=CARTESIAN_POINT('Ctrl Pts',(0.450222009543773,1.,4.0476929901797));
#44108=CARTESIAN_POINT('Ctrl Pts',(0.452365214748778,1.,4.0402939222793));
#44109=CARTESIAN_POINT('Ctrl Pts',(0.454469363020495,1.,4.03289354362745));
#44110=CARTESIAN_POINT('Ctrl Pts',(0.456534070784968,1.,4.02549199038414));
#44111=CARTESIAN_POINT('Ctrl Pts',(0.458558885637,1.,4.01808900827647));
#44112=CARTESIAN_POINT('Ctrl Pts',(0.460543280768577,1.,4.01068390573469));
#44113=CARTESIAN_POINT('Ctrl Pts',(0.462486702616251,1.,4.00327590659129));
#44114=CARTESIAN_POINT('Ctrl Pts',(0.464388610938994,1.,3.99586444320135));
#44115=CARTESIAN_POINT('Ctrl Pts',(0.466248520883034,1.,3.98844946363258));
#44116=CARTESIAN_POINT('Ctrl Pts',(0.468066047920139,1.,3.98103175589349));
#44117=CARTESIAN_POINT('Ctrl Pts',(0.469840942829878,1.,3.97361320212413));
#44118=CARTESIAN_POINT('Ctrl Pts',(0.471572978413493,1.,3.96619600864626));
#44119=CARTESIAN_POINT('Ctrl Pts',(0.473261847236295,1.,3.95878201038332));
#44120=CARTESIAN_POINT('Ctrl Pts',(0.47490705302179,1.,3.95137192932898));
#44121=CARTESIAN_POINT('Ctrl Pts',(0.476507810658534,1.,3.94396469119385));
#44122=CARTESIAN_POINT('Ctrl Pts',(0.478062927140957,1.,3.93655660689819));
#44123=CARTESIAN_POINT('Ctrl Pts',(0.479571028525565,1.,3.92914297392067));
#44124=CARTESIAN_POINT('Ctrl Pts',(0.481030798910735,1.,3.92171976072334));
#44125=CARTESIAN_POINT('Ctrl Pts',(0.482441230340708,1.,3.91428536373749));
#44126=CARTESIAN_POINT('Ctrl Pts',(0.48380183508916,1.,3.90684210358063));
#44127=CARTESIAN_POINT('Ctrl Pts',(0.485112963522245,1.,3.89939844658529));
#44128=CARTESIAN_POINT('Ctrl Pts',(0.486375337854133,1.,3.89196582437574));
#44129=CARTESIAN_POINT('Ctrl Pts',(0.487589452275179,1.,3.88455453328156));
#44130=CARTESIAN_POINT('Ctrl Pts',(0.488754973798281,1.,3.87716963231115));
#44131=CARTESIAN_POINT('Ctrl Pts',(0.489870245704899,1.,3.86980755613694));
#44132=CARTESIAN_POINT('Ctrl Pts',(0.490931482170849,1.,3.86245057319215));
#44133=CARTESIAN_POINT('Ctrl Pts',(0.49193363108376,1.,3.85507287020223));
#44134=CARTESIAN_POINT('Ctrl Pts',(0.492871792414095,1.,3.84765051147965));
#44135=CARTESIAN_POINT('Ctrl Pts',(0.493742574629117,1.,3.84017095578438));
#44136=CARTESIAN_POINT('Ctrl Pts',(0.494545212256425,1.,3.8326409268245));
#44137=CARTESIAN_POINT('Ctrl Pts',(0.495283458893903,1.,3.82509963594156));
#44138=CARTESIAN_POINT('Ctrl Pts',(0.495963937875571,1.,3.81760756144099));
#44139=CARTESIAN_POINT('Ctrl Pts',(0.496592643443789,1.,3.81022254090909));
#44140=CARTESIAN_POINT('Ctrl Pts',(0.49717175620109,1.,3.80297788298545));
#44141=CARTESIAN_POINT('Ctrl Pts',(0.49769689210058,1.,3.79586380669959));
#44142=CARTESIAN_POINT('Ctrl Pts',(0.498152751800819,1.,3.78879701661152));
#44143=CARTESIAN_POINT('Ctrl Pts',(0.498515471679378,1.,3.78163975337189));
#44144=CARTESIAN_POINT('Ctrl Pts',(0.498759900365686,1.,3.77425499225089));
#44145=CARTESIAN_POINT('Ctrl Pts',(0.498865792335185,1.,3.76655401191144));
#44146=CARTESIAN_POINT('Ctrl Pts',(0.498823681615513,1.,3.75854082221127));
#44147=CARTESIAN_POINT('Ctrl Pts',(0.498642802042929,1.,3.75037362168103));
#44148=CARTESIAN_POINT('Ctrl Pts',(0.498350586058176,1.,3.74235701735109));
#44149=CARTESIAN_POINT('Ctrl Pts',(0.497984209510495,1.,3.73486914372834));
#44150=CARTESIAN_POINT('Ctrl Pts',(0.497584067153279,1.,3.72830430904794));
#44151=CARTESIAN_POINT('Ctrl Pts',(0.497187079575794,1.,3.72301489774241));
#44152=CARTESIAN_POINT('Ctrl Pts',(0.496846224822534,1.,3.7195232082259));
#44153=CARTESIAN_POINT('Ctrl Pts',(0.496605651526313,1.,3.71785517607694));
#44154=CARTESIAN_POINT('Ctrl Pts',(0.496446644158827,1.,3.71721917030465));
#44155=CARTESIAN_POINT('Ctrl Pts',(0.496354087925645,1.,3.71704500630521));
#44156=CARTESIAN_POINT('Ctrl Pts',(0.496319364829374,1.,3.71701050416802));
#44157=CARTESIAN_POINT('',(0.405301974318349,0.,4.18039834341342));
#44158=CARTESIAN_POINT('Ctrl Pts',(0.0913616755937418,-1.,3.74888690736767));
#44159=CARTESIAN_POINT('Ctrl Pts',(0.0913616755937418,1.,3.74888690736767));
#44160=CARTESIAN_POINT('Ctrl Pts',(0.0912992005792582,-1.,3.74882632119067));
#44161=CARTESIAN_POINT('Ctrl Pts',(0.0912992005792582,1.,3.74882632119067));
#44162=CARTESIAN_POINT('Ctrl Pts',(0.0911958743735231,-1.,3.74887017174206));
#44163=CARTESIAN_POINT('Ctrl Pts',(0.0911958743735231,1.,3.74887017174206));
#44164=CARTESIAN_POINT('Ctrl Pts',(0.0911057547506597,-1.,3.74943097853811));
#44165=CARTESIAN_POINT('Ctrl Pts',(0.0911057547506597,1.,3.74943097853811));
#44166=CARTESIAN_POINT('Ctrl Pts',(0.0911154000998139,-1.,3.75116949194623));
#44167=CARTESIAN_POINT('Ctrl Pts',(0.0911154000998139,1.,3.75116949194623));
#44168=CARTESIAN_POINT('Ctrl Pts',(0.0913419622736395,-1.,3.75495560118212));
#44169=CARTESIAN_POINT('Ctrl Pts',(0.0913419622736395,1.,3.75495560118212));
#44170=CARTESIAN_POINT('Ctrl Pts',(0.0917773084998332,-1.,3.76024199359303));
#44171=CARTESIAN_POINT('Ctrl Pts',(0.0917773084998332,1.,3.76024199359303));
#44172=CARTESIAN_POINT('Ctrl Pts',(0.0924090589602688,-1.,3.76678860031841));
#44173=CARTESIAN_POINT('Ctrl Pts',(0.0924090589602688,1.,3.76678860031841));
#44174=CARTESIAN_POINT('Ctrl Pts',(0.0932185546203175,-1.,3.77424159971059));
#44175=CARTESIAN_POINT('Ctrl Pts',(0.0932185546203175,1.,3.77424159971059));
#44176=CARTESIAN_POINT('Ctrl Pts',(0.0941840095090811,-1.,3.782205218991));
#44177=CARTESIAN_POINT('Ctrl Pts',(0.0941840095090811,1.,3.782205218991));
#44178=CARTESIAN_POINT('Ctrl Pts',(0.0952829885100798,-1.,3.79030016353111));
#44179=CARTESIAN_POINT('Ctrl Pts',(0.0952829885100798,1.,3.79030016353111));
#44180=CARTESIAN_POINT('Ctrl Pts',(0.0964949352873128,-1.,3.79822128513845));
#44181=CARTESIAN_POINT('Ctrl Pts',(0.0964949352873128,1.,3.79822128513845));
#44182=CARTESIAN_POINT('Ctrl Pts',(0.097804222290664,-1.,3.80581088847809));
#44183=CARTESIAN_POINT('Ctrl Pts',(0.097804222290664,1.,3.80581088847809));
#44184=CARTESIAN_POINT('Ctrl Pts',(0.0992008728096511,-1.,3.81306649386461));
#44185=CARTESIAN_POINT('Ctrl Pts',(0.0992008728096511,1.,3.81306649386461));
#44186=CARTESIAN_POINT('Ctrl Pts',(0.100678769650632,-1.,3.82007889742625));
#44187=CARTESIAN_POINT('Ctrl Pts',(0.100678769650632,1.,3.82007889742625));
#44188=CARTESIAN_POINT('Ctrl Pts',(0.102234506488456,-1.,3.82698737143255));
#44189=CARTESIAN_POINT('Ctrl Pts',(0.102234506488456,1.,3.82698737143255));
#44190=CARTESIAN_POINT('Ctrl Pts',(0.103866063811622,-1.,3.83393171228002));
#44191=CARTESIAN_POINT('Ctrl Pts',(0.103866063811622,1.,3.83393171228002));
#44192=CARTESIAN_POINT('Ctrl Pts',(0.105571360916569,-1.,3.84099658324803));
#44193=CARTESIAN_POINT('Ctrl Pts',(0.105571360916569,1.,3.84099658324803));
#44194=CARTESIAN_POINT('Ctrl Pts',(0.107347597812183,-1.,3.84819233070317));
#44195=CARTESIAN_POINT('Ctrl Pts',(0.107347597812183,1.,3.84819233070317));
#44196=CARTESIAN_POINT('Ctrl Pts',(0.109191717634943,-1.,3.855485714969));
#44197=CARTESIAN_POINT('Ctrl Pts',(0.109191717634943,1.,3.855485714969));
#44198=CARTESIAN_POINT('Ctrl Pts',(0.11110059303626,-1.,3.86281867282965));
#44199=CARTESIAN_POINT('Ctrl Pts',(0.11110059303626,1.,3.86281867282965));
#44200=CARTESIAN_POINT('Ctrl Pts',(0.113071304914561,-1.,3.87013043445014));
#44201=CARTESIAN_POINT('Ctrl Pts',(0.113071304914561,1.,3.87013043445014));
#44202=CARTESIAN_POINT('Ctrl Pts',(0.115101426649469,-1.,3.87738168405343));
#44203=CARTESIAN_POINT('Ctrl Pts',(0.115101426649469,1.,3.87738168405343));
#44204=CARTESIAN_POINT('Ctrl Pts',(0.117189150373144,-1.,3.88456590045767));
#44205=CARTESIAN_POINT('Ctrl Pts',(0.117189150373144,1.,3.88456590045767));
#44206=CARTESIAN_POINT('Ctrl Pts',(0.119333088190417,-1.,3.89169600105201));
#44207=CARTESIAN_POINT('Ctrl Pts',(0.119333088190417,1.,3.89169600105201));
#44208=CARTESIAN_POINT('Ctrl Pts',(0.121532144765723,-1.,3.89879639336952));
#44209=CARTESIAN_POINT('Ctrl Pts',(0.121532144765723,1.,3.89879639336952));
#44210=CARTESIAN_POINT('Ctrl Pts',(0.123785368272377,-1.,3.90589336320508));
#44211=CARTESIAN_POINT('Ctrl Pts',(0.123785368272377,1.,3.90589336320508));
#44212=CARTESIAN_POINT('Ctrl Pts',(0.126091793324136,-1.,3.91300501605392));
#44213=CARTESIAN_POINT('Ctrl Pts',(0.126091793324136,1.,3.91300501605392));
#44214=CARTESIAN_POINT('Ctrl Pts',(0.128450341339527,-1.,3.92013513251642));
#44215=CARTESIAN_POINT('Ctrl Pts',(0.128450341339527,1.,3.92013513251642));
#44216=CARTESIAN_POINT('Ctrl Pts',(0.130859892027798,-1.,3.9272787679596));
#44217=CARTESIAN_POINT('Ctrl Pts',(0.130859892027798,1.,3.9272787679596));
#44218=CARTESIAN_POINT('Ctrl Pts',(0.133319322794189,-1.,3.93442567551035));
#44219=CARTESIAN_POINT('Ctrl Pts',(0.133319322794189,1.,3.93442567551035));
#44220=CARTESIAN_POINT('Ctrl Pts',(0.135827558661187,-1.,3.94156445130744));
#44221=CARTESIAN_POINT('Ctrl Pts',(0.135827558661187,1.,3.94156445130744));
#44222=CARTESIAN_POINT('Ctrl Pts',(0.138383621255159,-1.,3.94868667844355));
#44223=CARTESIAN_POINT('Ctrl Pts',(0.138383621255159,1.,3.94868667844355));
#44224=CARTESIAN_POINT('Ctrl Pts',(0.140986665829936,-1.,3.95579014116899));
#44225=CARTESIAN_POINT('Ctrl Pts',(0.140986665829936,1.,3.95579014116899));
#44226=CARTESIAN_POINT('Ctrl Pts',(0.143635947692791,-1.,3.96287658098896));
#44227=CARTESIAN_POINT('Ctrl Pts',(0.143635947692791,1.,3.96287658098896));
#44228=CARTESIAN_POINT('Ctrl Pts',(0.146330797814513,-1.,3.96995018565891));
#44229=CARTESIAN_POINT('Ctrl Pts',(0.146330797814513,1.,3.96995018565891));
#44230=CARTESIAN_POINT('Ctrl Pts',(0.149070594803543,-1.,3.97701581473643));
#44231=CARTESIAN_POINT('Ctrl Pts',(0.149070594803543,1.,3.97701581473643));
#44232=CARTESIAN_POINT('Ctrl Pts',(0.151854737441405,-1.,3.9840772985098));
#44233=CARTESIAN_POINT('Ctrl Pts',(0.151854737441405,1.,3.9840772985098));
#44234=CARTESIAN_POINT('Ctrl Pts',(0.154682618338563,-1.,3.99113582086059));
#44235=CARTESIAN_POINT('Ctrl Pts',(0.154682618338563,1.,3.99113582086059));
#44236=CARTESIAN_POINT('Ctrl Pts',(0.157553634383809,-1.,3.99819074631874));
#44237=CARTESIAN_POINT('Ctrl Pts',(0.157553634383809,1.,3.99819074631874));
#44238=CARTESIAN_POINT('Ctrl Pts',(0.160467194882218,-1.,4.00524031064509));
#44239=CARTESIAN_POINT('Ctrl Pts',(0.160467194882218,1.,4.00524031064509));
#44240=CARTESIAN_POINT('Ctrl Pts',(0.163422730287458,-1.,4.01228237022301));
#44241=CARTESIAN_POINT('Ctrl Pts',(0.163422730287458,1.,4.01228237022301));
#44242=CARTESIAN_POINT('Ctrl Pts',(0.166419700015847,-1.,4.01931510507143));
#44243=CARTESIAN_POINT('Ctrl Pts',(0.166419700015847,1.,4.01931510507143));
#44244=CARTESIAN_POINT('Ctrl Pts',(0.169457601001653,-1.,4.0263377970371));
#44245=CARTESIAN_POINT('Ctrl Pts',(0.169457601001653,1.,4.0263377970371));
#44246=CARTESIAN_POINT('Ctrl Pts',(0.172535962484466,-1.,4.03335057326093));
#44247=CARTESIAN_POINT('Ctrl Pts',(0.172535962484466,1.,4.03335057326093));
#44248=CARTESIAN_POINT('Ctrl Pts',(0.175654339673757,-1.,4.04035407891161));
#44249=CARTESIAN_POINT('Ctrl Pts',(0.175654339673757,1.,4.04035407891161));
#44250=CARTESIAN_POINT('Ctrl Pts',(0.178812307240715,-1.,4.04734916719722));
#44251=CARTESIAN_POINT('Ctrl Pts',(0.178812307240715,1.,4.04734916719722));
#44252=CARTESIAN_POINT('Ctrl Pts',(0.18200945304855,-1.,4.05433660358402));
#44253=CARTESIAN_POINT('Ctrl Pts',(0.18200945304855,1.,4.05433660358402));
#44254=CARTESIAN_POINT('Ctrl Pts',(0.185245370038947,-1.,4.06131670998589));
#44255=CARTESIAN_POINT('Ctrl Pts',(0.185245370038947,1.,4.06131670998589));
#44256=CARTESIAN_POINT('Ctrl Pts',(0.188519658060255,-1.,4.06828941192308));
#44257=CARTESIAN_POINT('Ctrl Pts',(0.188519658060255,1.,4.06828941192308));
#44258=CARTESIAN_POINT('Ctrl Pts',(0.191831928181081,-1.,4.07525439703137));
#44259=CARTESIAN_POINT('Ctrl Pts',(0.191831928181081,1.,4.07525439703137));
#44260=CARTESIAN_POINT('Ctrl Pts',(0.195181806054714,-1.,4.08221124060385));
#44261=CARTESIAN_POINT('Ctrl Pts',(0.195181806054714,1.,4.08221124060385));
#44262=CARTESIAN_POINT('Ctrl Pts',(0.19856893480081,-1.,4.08915953359753));
#44263=CARTESIAN_POINT('Ctrl Pts',(0.19856893480081,1.,4.08915953359753));
#44264=CARTESIAN_POINT('Ctrl Pts',(0.201992979049984,-1.,4.09609903751912));
#44265=CARTESIAN_POINT('Ctrl Pts',(0.201992979049984,1.,4.09609903751912));
#44266=CARTESIAN_POINT('Ctrl Pts',(0.205453622198233,-1.,4.10302969965374));
#44267=CARTESIAN_POINT('Ctrl Pts',(0.205453622198233,1.,4.10302969965374));
#44268=CARTESIAN_POINT('Ctrl Pts',(0.208950559400171,-1.,4.10995157639026));
#44269=CARTESIAN_POINT('Ctrl Pts',(0.208950559400171,1.,4.10995157639026));
#44270=CARTESIAN_POINT('Ctrl Pts',(0.212483491087067,-1.,4.11686478264545));
#44271=CARTESIAN_POINT('Ctrl Pts',(0.212483491087067,1.,4.11686478264545));
#44272=CARTESIAN_POINT('Ctrl Pts',(0.216052116898424,-1.,4.12376943492249));
#44273=CARTESIAN_POINT('Ctrl Pts',(0.216052116898424,1.,4.12376943492249));
#44274=CARTESIAN_POINT('Ctrl Pts',(0.219656126701851,-1.,4.13066558698156));
#44275=CARTESIAN_POINT('Ctrl Pts',(0.219656126701851,1.,4.13066558698156));
#44276=CARTESIAN_POINT('Ctrl Pts',(0.223295201038383,-1.,4.13755320553563));
#44277=CARTESIAN_POINT('Ctrl Pts',(0.223295201038383,1.,4.13755320553563));
#44278=CARTESIAN_POINT('Ctrl Pts',(0.226969025061243,-1.,4.14443220607733));
#44279=CARTESIAN_POINT('Ctrl Pts',(0.226969025061243,1.,4.14443220607733));
#44280=CARTESIAN_POINT('Ctrl Pts',(0.230677299028737,-1.,4.15130247435029));
#44281=CARTESIAN_POINT('Ctrl Pts',(0.230677299028737,1.,4.15130247435029));
#44282=CARTESIAN_POINT('Ctrl Pts',(0.234419749543142,-1.,4.1581638926525));
#44283=CARTESIAN_POINT('Ctrl Pts',(0.234419749543142,1.,4.1581638926525));
#44284=CARTESIAN_POINT('Ctrl Pts',(0.238196140933976,-1.,4.1650163665385));
#44285=CARTESIAN_POINT('Ctrl Pts',(0.238196140933976,1.,4.1650163665385));
#44286=CARTESIAN_POINT('Ctrl Pts',(0.242006283923911,-1.,4.17185984409533));
#44287=CARTESIAN_POINT('Ctrl Pts',(0.242006283923911,1.,4.17185984409533));
#44288=CARTESIAN_POINT('Ctrl Pts',(0.245850033418583,-1.,4.17869430192868));
#44289=CARTESIAN_POINT('Ctrl Pts',(0.245850033418583,1.,4.17869430192868));
#44290=CARTESIAN_POINT('Ctrl Pts',(0.248951836910963,-1.,4.18415464959491));
#44291=CARTESIAN_POINT('Ctrl Pts',(0.248951836910963,1.,4.18415464959491));
#44292=CARTESIAN_POINT('Ctrl Pts',(0.251293239837692,-1.,4.18824585244066));
#44293=CARTESIAN_POINT('Ctrl Pts',(0.251293239837692,1.,4.18824585244066));
#44294=CARTESIAN_POINT('Ctrl Pts',(0.252860861572565,-1.,4.19097151819241));
#44295=CARTESIAN_POINT('Ctrl Pts',(0.252860861572565,1.,4.19097151819241));
#44296=CARTESIAN_POINT('Ctrl Pts',(0.253646344052521,-1.,4.1923339003649));
#44297=CARTESIAN_POINT('Ctrl Pts',(0.253646344052521,1.,4.1923339003649));
#44298=CARTESIAN_POINT('',(0.0912596999166814,1.,3.74888939116255));
#44299=CARTESIAN_POINT('Ctrl Pts',(0.0912596999166821,-1.,3.74888939116255));
#44300=CARTESIAN_POINT('Ctrl Pts',(0.0912596999166821,-0.666666666666667,
3.74888939116255));
#44301=CARTESIAN_POINT('Ctrl Pts',(0.0912596999166821,-0.333333333333333,
3.74888939116255));
#44302=CARTESIAN_POINT('Ctrl Pts',(0.0912596999166821,0.333333333333333,
3.74888939116255));
#44303=CARTESIAN_POINT('Ctrl Pts',(0.0912596999166819,0.666666666666667,
3.74888939116255));
#44304=CARTESIAN_POINT('Ctrl Pts',(0.0912596999166819,1.,3.74888939116255));
#44305=CARTESIAN_POINT('',(0.253646344052521,1.,4.1923339003649));
#44306=CARTESIAN_POINT('',(0.253646344052521,0.,4.1923339003649));
#44307=CARTESIAN_POINT('Ctrl Pts',(0.0912596999166818,1.,3.74888939116255));
#44308=CARTESIAN_POINT('Ctrl Pts',(0.0912308016421978,1.,3.74892890040975));
#44309=CARTESIAN_POINT('Ctrl Pts',(0.0911666301812813,1.,3.74911539914542));
#44310=CARTESIAN_POINT('Ctrl Pts',(0.0911090736805507,1.,3.74976844886347));
#44311=CARTESIAN_POINT('Ctrl Pts',(0.0911323999574424,1.,3.75145357872422));
#44312=CARTESIAN_POINT('Ctrl Pts',(0.0913419622736395,1.,3.75495560118212));
#44313=CARTESIAN_POINT('Ctrl Pts',(0.0917773084998332,1.,3.76024199359303));
#44314=CARTESIAN_POINT('Ctrl Pts',(0.0924090589602688,1.,3.76678860031841));
#44315=CARTESIAN_POINT('Ctrl Pts',(0.0932185546203175,1.,3.77424159971059));
#44316=CARTESIAN_POINT('Ctrl Pts',(0.0941840095090811,1.,3.782205218991));
#44317=CARTESIAN_POINT('Ctrl Pts',(0.0952829885100798,1.,3.79030016353111));
#44318=CARTESIAN_POINT('Ctrl Pts',(0.0964949352873128,1.,3.79822128513845));
#44319=CARTESIAN_POINT('Ctrl Pts',(0.097804222290664,1.,3.80581088847809));
#44320=CARTESIAN_POINT('Ctrl Pts',(0.0992008728096511,1.,3.81306649386461));
#44321=CARTESIAN_POINT('Ctrl Pts',(0.100678769650632,1.,3.82007889742625));
#44322=CARTESIAN_POINT('Ctrl Pts',(0.102234506488456,1.,3.82698737143255));
#44323=CARTESIAN_POINT('Ctrl Pts',(0.103866063811622,1.,3.83393171228002));
#44324=CARTESIAN_POINT('Ctrl Pts',(0.105571360916569,1.,3.84099658324803));
#44325=CARTESIAN_POINT('Ctrl Pts',(0.107347597812183,1.,3.84819233070317));
#44326=CARTESIAN_POINT('Ctrl Pts',(0.109191717634943,1.,3.855485714969));
#44327=CARTESIAN_POINT('Ctrl Pts',(0.11110059303626,1.,3.86281867282965));
#44328=CARTESIAN_POINT('Ctrl Pts',(0.113071304914561,1.,3.87013043445014));
#44329=CARTESIAN_POINT('Ctrl Pts',(0.115101426649469,1.,3.87738168405343));
#44330=CARTESIAN_POINT('Ctrl Pts',(0.117189150373144,1.,3.88456590045767));
#44331=CARTESIAN_POINT('Ctrl Pts',(0.119333088190417,1.,3.89169600105201));
#44332=CARTESIAN_POINT('Ctrl Pts',(0.121532144765723,1.,3.89879639336952));
#44333=CARTESIAN_POINT('Ctrl Pts',(0.123785368272377,1.,3.90589336320508));
#44334=CARTESIAN_POINT('Ctrl Pts',(0.126091793324136,1.,3.91300501605392));
#44335=CARTESIAN_POINT('Ctrl Pts',(0.128450341339527,1.,3.92013513251642));
#44336=CARTESIAN_POINT('Ctrl Pts',(0.130859892027798,1.,3.9272787679596));
#44337=CARTESIAN_POINT('Ctrl Pts',(0.133319322794189,1.,3.93442567551035));
#44338=CARTESIAN_POINT('Ctrl Pts',(0.135827558661187,1.,3.94156445130744));
#44339=CARTESIAN_POINT('Ctrl Pts',(0.138383621255159,1.,3.94868667844355));
#44340=CARTESIAN_POINT('Ctrl Pts',(0.140986665829936,1.,3.95579014116899));
#44341=CARTESIAN_POINT('Ctrl Pts',(0.143635947692791,1.,3.96287658098896));
#44342=CARTESIAN_POINT('Ctrl Pts',(0.146330797814513,1.,3.96995018565891));
#44343=CARTESIAN_POINT('Ctrl Pts',(0.149070594803543,1.,3.97701581473643));
#44344=CARTESIAN_POINT('Ctrl Pts',(0.151854737441405,1.,3.9840772985098));
#44345=CARTESIAN_POINT('Ctrl Pts',(0.154682618338563,1.,3.99113582086059));
#44346=CARTESIAN_POINT('Ctrl Pts',(0.157553634383809,1.,3.99819074631874));
#44347=CARTESIAN_POINT('Ctrl Pts',(0.160467194882218,1.,4.00524031064509));
#44348=CARTESIAN_POINT('Ctrl Pts',(0.163422730287458,1.,4.01228237022301));
#44349=CARTESIAN_POINT('Ctrl Pts',(0.166419700015847,1.,4.01931510507143));
#44350=CARTESIAN_POINT('Ctrl Pts',(0.169457601001653,1.,4.0263377970371));
#44351=CARTESIAN_POINT('Ctrl Pts',(0.172535962484466,1.,4.03335057326093));
#44352=CARTESIAN_POINT('Ctrl Pts',(0.175654339673757,1.,4.04035407891161));
#44353=CARTESIAN_POINT('Ctrl Pts',(0.178812307240715,1.,4.04734916719722));
#44354=CARTESIAN_POINT('Ctrl Pts',(0.18200945304855,1.,4.05433660358402));
#44355=CARTESIAN_POINT('Ctrl Pts',(0.185245370038947,1.,4.06131670998589));
#44356=CARTESIAN_POINT('Ctrl Pts',(0.188519658060255,1.,4.06828941192308));
#44357=CARTESIAN_POINT('Ctrl Pts',(0.191831928181081,1.,4.07525439703137));
#44358=CARTESIAN_POINT('Ctrl Pts',(0.195181806054714,1.,4.08221124060385));
#44359=CARTESIAN_POINT('Ctrl Pts',(0.19856893480081,1.,4.08915953359753));
#44360=CARTESIAN_POINT('Ctrl Pts',(0.201992979049984,1.,4.09609903751912));
#44361=CARTESIAN_POINT('Ctrl Pts',(0.205453622198233,1.,4.10302969965374));
#44362=CARTESIAN_POINT('Ctrl Pts',(0.208950559400171,1.,4.10995157639026));
#44363=CARTESIAN_POINT('Ctrl Pts',(0.212483491087067,1.,4.11686478264545));
#44364=CARTESIAN_POINT('Ctrl Pts',(0.216052116898424,1.,4.12376943492249));
#44365=CARTESIAN_POINT('Ctrl Pts',(0.219656126701851,1.,4.13066558698156));
#44366=CARTESIAN_POINT('Ctrl Pts',(0.223295201038383,1.,4.13755320553563));
#44367=CARTESIAN_POINT('Ctrl Pts',(0.226969025061243,1.,4.14443220607733));
#44368=CARTESIAN_POINT('Ctrl Pts',(0.230677299028737,1.,4.15130247435029));
#44369=CARTESIAN_POINT('Ctrl Pts',(0.234419749543142,1.,4.1581638926525));
#44370=CARTESIAN_POINT('Ctrl Pts',(0.238196140933976,1.,4.1650163665385));
#44371=CARTESIAN_POINT('Ctrl Pts',(0.242006283923911,1.,4.17185984409533));
#44372=CARTESIAN_POINT('Ctrl Pts',(0.245850033418583,1.,4.17869430192868));
#44373=CARTESIAN_POINT('Ctrl Pts',(0.248951836910963,1.,4.18415464959491));
#44374=CARTESIAN_POINT('Ctrl Pts',(0.251293239837692,1.,4.18824585244066));
#44375=CARTESIAN_POINT('Ctrl Pts',(0.252860861572565,1.,4.19097151819241));
#44376=CARTESIAN_POINT('Ctrl Pts',(0.253646344052521,1.,4.1923339003649));
#44377=CARTESIAN_POINT('Origin',(0.253646344052521,0.,4.1923339003649));
#44378=CARTESIAN_POINT('',(0.405301974318349,1.,4.18039834341342));
#44379=CARTESIAN_POINT('Origin',(0.,0.,0.));
#44380=CARTESIAN_POINT('',(-0.0912596999148862,1.,3.74888939116259));
#44381=CARTESIAN_POINT('Origin',(0.,1.,0.));
#44382=CARTESIAN_POINT('Ctrl Pts',(-0.0912596999148859,1.,3.74888939116259));
#44383=CARTESIAN_POINT('Ctrl Pts',(-0.0912596999148859,0.666666666666667,
3.74888939116259));
#44384=CARTESIAN_POINT('Ctrl Pts',(-0.0912596999148859,0.333333333333333,
3.74888939116259));
#44385=CARTESIAN_POINT('Ctrl Pts',(-0.0912596999148859,-0.333333333333333,
3.74888939116259));
#44386=CARTESIAN_POINT('Ctrl Pts',(-0.0912596999148859,-0.666666666666667,
3.74888939116259));
#44387=CARTESIAN_POINT('Ctrl Pts',(-0.0912596999148859,-1.,3.74888939116259));
#44388=CARTESIAN_POINT('Ctrl Pts',(-0.253646344052522,-1.,4.1923339003649));
#44389=CARTESIAN_POINT('Ctrl Pts',(-0.253646344052522,1.,4.1923339003649));
#44390=CARTESIAN_POINT('Ctrl Pts',(-0.252860861572841,-1.,4.19097151819684));
#44391=CARTESIAN_POINT('Ctrl Pts',(-0.252860861572841,1.,4.19097151819684));
#44392=CARTESIAN_POINT('Ctrl Pts',(-0.251293239838441,-1.,4.18824585245272));
#44393=CARTESIAN_POINT('Ctrl Pts',(-0.251293239838441,1.,4.18824585245272));
#44394=CARTESIAN_POINT('Ctrl Pts',(-0.248951836912189,-1.,4.18415464961466));
#44395=CARTESIAN_POINT('Ctrl Pts',(-0.248951836912189,1.,4.18415464961466));
#44396=CARTESIAN_POINT('Ctrl Pts',(-0.245850033420019,-1.,4.1786943019518));
#44397=CARTESIAN_POINT('Ctrl Pts',(-0.245850033420019,1.,4.1786943019518));
#44398=CARTESIAN_POINT('Ctrl Pts',(-0.242006283925089,-1.,4.17185984411426));
#44399=CARTESIAN_POINT('Ctrl Pts',(-0.242006283925089,1.,4.17185984411426));
#44400=CARTESIAN_POINT('Ctrl Pts',(-0.238196140934616,-1.,4.16501636654877));
#44401=CARTESIAN_POINT('Ctrl Pts',(-0.238196140934616,1.,4.16501636654877));
#44402=CARTESIAN_POINT('Ctrl Pts',(-0.234419749543208,-1.,4.15816389265352));
#44403=CARTESIAN_POINT('Ctrl Pts',(-0.234419749543208,1.,4.15816389265352));
#44404=CARTESIAN_POINT('Ctrl Pts',(-0.230677299028383,-1.,4.15130247434459));
#44405=CARTESIAN_POINT('Ctrl Pts',(-0.230677299028383,1.,4.15130247434459));
#44406=CARTESIAN_POINT('Ctrl Pts',(-0.226969025060705,-1.,4.14443220606869));
#44407=CARTESIAN_POINT('Ctrl Pts',(-0.226969025060705,1.,4.14443220606869));
#44408=CARTESIAN_POINT('Ctrl Pts',(-0.223295201037886,-1.,4.13755320552764));
#44409=CARTESIAN_POINT('Ctrl Pts',(-0.223295201037886,1.,4.13755320552764));
#44410=CARTESIAN_POINT('Ctrl Pts',(-0.219656126701542,-1.,4.13066558697658));
#44411=CARTESIAN_POINT('Ctrl Pts',(-0.219656126701542,1.,4.13066558697658));
#44412=CARTESIAN_POINT('Ctrl Pts',(-0.216052116898352,-1.,4.12376943492132));
#44413=CARTESIAN_POINT('Ctrl Pts',(-0.216052116898352,1.,4.12376943492132));
#44414=CARTESIAN_POINT('Ctrl Pts',(-0.21248349108719,-1.,4.11686478264739));
#44415=CARTESIAN_POINT('Ctrl Pts',(-0.21248349108719,1.,4.11686478264739));
#44416=CARTESIAN_POINT('Ctrl Pts',(-0.208950559400393,-1.,4.10995157639377));
#44417=CARTESIAN_POINT('Ctrl Pts',(-0.208950559400393,1.,4.10995157639377));
#44418=CARTESIAN_POINT('Ctrl Pts',(-0.205453622198455,-1.,4.10302969965728));
#44419=CARTESIAN_POINT('Ctrl Pts',(-0.205453622198455,1.,4.10302969965728));
#44420=CARTESIAN_POINT('Ctrl Pts',(-0.201992979050136,-1.,4.09609903752152));
#44421=CARTESIAN_POINT('Ctrl Pts',(-0.201992979050136,1.,4.09609903752152));
#44422=CARTESIAN_POINT('Ctrl Pts',(-0.198568934800862,-1.,4.08915953359833));
#44423=CARTESIAN_POINT('Ctrl Pts',(-0.198568934800862,1.,4.08915953359833));
#44424=CARTESIAN_POINT('Ctrl Pts',(-0.195181806054676,-1.,4.08221124060322));
#44425=CARTESIAN_POINT('Ctrl Pts',(-0.195181806054676,1.,4.08221124060322));
#44426=CARTESIAN_POINT('Ctrl Pts',(-0.191831928180991,-1.,4.07525439702992));
#44427=CARTESIAN_POINT('Ctrl Pts',(-0.191831928180991,1.,4.07525439702992));
#44428=CARTESIAN_POINT('Ctrl Pts',(-0.188519658060156,-1.,4.06828941192148));
#44429=CARTESIAN_POINT('Ctrl Pts',(-0.188519658060156,1.,4.06828941192148));
#44430=CARTESIAN_POINT('Ctrl Pts',(-0.185245370038874,-1.,4.06131670998469));
#44431=CARTESIAN_POINT('Ctrl Pts',(-0.185245370038874,1.,4.06131670998469));
#44432=CARTESIAN_POINT('Ctrl Pts',(-0.18200945304852,-1.,4.05433660358353));
#44433=CARTESIAN_POINT('Ctrl Pts',(-0.18200945304852,1.,4.05433660358353));
#44434=CARTESIAN_POINT('Ctrl Pts',(-0.178812307240729,-1.,4.04734916719741));
#44435=CARTESIAN_POINT('Ctrl Pts',(-0.178812307240729,1.,4.04734916719741));
#44436=CARTESIAN_POINT('Ctrl Pts',(-0.175654339673798,-1.,4.04035407891222));
#44437=CARTESIAN_POINT('Ctrl Pts',(-0.175654339673798,1.,4.04035407891222));
#44438=CARTESIAN_POINT('Ctrl Pts',(-0.172535962484514,-1.,4.03335057326163));
#44439=CARTESIAN_POINT('Ctrl Pts',(-0.172535962484514,1.,4.03335057326163));
#44440=CARTESIAN_POINT('Ctrl Pts',(-0.169457601001691,-1.,4.02633779703764));
#44441=CARTESIAN_POINT('Ctrl Pts',(-0.169457601001691,1.,4.02633779703764));
#44442=CARTESIAN_POINT('Ctrl Pts',(-0.166419700015866,-1.,4.01931510507167));
#44443=CARTESIAN_POINT('Ctrl Pts',(-0.166419700015866,1.,4.01931510507167));
#44444=CARTESIAN_POINT('Ctrl Pts',(-0.163422730287457,-1.,4.01228237022296));
#44445=CARTESIAN_POINT('Ctrl Pts',(-0.163422730287457,1.,4.01228237022296));
#44446=CARTESIAN_POINT('Ctrl Pts',(-0.160467194882203,-1.,4.00524031064487));
#44447=CARTESIAN_POINT('Ctrl Pts',(-0.160467194882203,1.,4.00524031064487));
#44448=CARTESIAN_POINT('Ctrl Pts',(-0.15755363438379,-1.,3.9981907463185));
#44449=CARTESIAN_POINT('Ctrl Pts',(-0.15755363438379,1.,3.9981907463185));
#44450=CARTESIAN_POINT('Ctrl Pts',(-0.154682618338548,-1.,3.99113582086043));
#44451=CARTESIAN_POINT('Ctrl Pts',(-0.154682618338548,1.,3.99113582086043));
#44452=CARTESIAN_POINT('Ctrl Pts',(-0.151854737441398,-1.,3.98407729850975));
#44453=CARTESIAN_POINT('Ctrl Pts',(-0.151854737441398,1.,3.98407729850975));
#44454=CARTESIAN_POINT('Ctrl Pts',(-0.149070594803545,-1.,3.97701581473644));
#44455=CARTESIAN_POINT('Ctrl Pts',(-0.149070594803545,1.,3.97701581473644));
#44456=CARTESIAN_POINT('Ctrl Pts',(-0.14633079781452,-1.,3.96995018565893));
#44457=CARTESIAN_POINT('Ctrl Pts',(-0.14633079781452,1.,3.96995018565893));
#44458=CARTESIAN_POINT('Ctrl Pts',(-0.143635947692799,-1.,3.96287658098896));
#44459=CARTESIAN_POINT('Ctrl Pts',(-0.143635947692799,1.,3.96287658098896));
#44460=CARTESIAN_POINT('Ctrl Pts',(-0.140986665829942,-1.,3.95579014116894));
#44461=CARTESIAN_POINT('Ctrl Pts',(-0.140986665829942,1.,3.95579014116894));
#44462=CARTESIAN_POINT('Ctrl Pts',(-0.138383621255161,-1.,3.94868667844347));
#44463=CARTESIAN_POINT('Ctrl Pts',(-0.138383621255161,1.,3.94868667844347));
#44464=CARTESIAN_POINT('Ctrl Pts',(-0.135827558661188,-1.,3.94156445130741));
#44465=CARTESIAN_POINT('Ctrl Pts',(-0.135827558661188,1.,3.94156445130741));
#44466=CARTESIAN_POINT('Ctrl Pts',(-0.133319322794191,-1.,3.93442567551042));
#44467=CARTESIAN_POINT('Ctrl Pts',(-0.133319322794191,1.,3.93442567551042));
#44468=CARTESIAN_POINT('Ctrl Pts',(-0.130859892027802,-1.,3.92727876795977));
#44469=CARTESIAN_POINT('Ctrl Pts',(-0.130859892027802,1.,3.92727876795977));
#44470=CARTESIAN_POINT('Ctrl Pts',(-0.128450341339532,-1.,3.92013513251664));
#44471=CARTESIAN_POINT('Ctrl Pts',(-0.128450341339532,1.,3.92013513251664));
#44472=CARTESIAN_POINT('Ctrl Pts',(-0.126091793324141,-1.,3.91300501605411));
#44473=CARTESIAN_POINT('Ctrl Pts',(-0.126091793324141,1.,3.91300501605411));
#44474=CARTESIAN_POINT('Ctrl Pts',(-0.12378536827238,-1.,3.90589336320515));
#44475=CARTESIAN_POINT('Ctrl Pts',(-0.12378536827238,1.,3.90589336320515));
#44476=CARTESIAN_POINT('Ctrl Pts',(-0.121532144765721,-1.,3.89879639336939));
#44477=CARTESIAN_POINT('Ctrl Pts',(-0.121532144765721,1.,3.89879639336939));
#44478=CARTESIAN_POINT('Ctrl Pts',(-0.11933308819041,-1.,3.8916960010517));
#44479=CARTESIAN_POINT('Ctrl Pts',(-0.11933308819041,1.,3.8916960010517));
#44480=CARTESIAN_POINT('Ctrl Pts',(-0.117189150373134,-1.,3.88456590045726));
#44481=CARTESIAN_POINT('Ctrl Pts',(-0.117189150373134,1.,3.88456590045726));
#44482=CARTESIAN_POINT('Ctrl Pts',(-0.115101426649461,-1.,3.87738168405308));
#44483=CARTESIAN_POINT('Ctrl Pts',(-0.115101426649461,1.,3.87738168405308));
#44484=CARTESIAN_POINT('Ctrl Pts',(-0.113071304914559,-1.,3.87013043445001));
#44485=CARTESIAN_POINT('Ctrl Pts',(-0.113071304914559,1.,3.87013043445001));
#44486=CARTESIAN_POINT('Ctrl Pts',(-0.111100593036267,-1.,3.86281867282984));
#44487=CARTESIAN_POINT('Ctrl Pts',(-0.111100593036267,1.,3.86281867282984));
#44488=CARTESIAN_POINT('Ctrl Pts',(-0.109191717634961,-1.,3.85548571496953));
#44489=CARTESIAN_POINT('Ctrl Pts',(-0.109191717634961,1.,3.85548571496953));
#44490=CARTESIAN_POINT('Ctrl Pts',(-0.107347597812208,-1.,3.84819233070391));
#44491=CARTESIAN_POINT('Ctrl Pts',(-0.107347597812208,1.,3.84819233070391));
#44492=CARTESIAN_POINT('Ctrl Pts',(-0.105571360916593,-1.,3.84099658324873));
#44493=CARTESIAN_POINT('Ctrl Pts',(-0.105571360916593,1.,3.84099658324873));
#44494=CARTESIAN_POINT('Ctrl Pts',(-0.103866063811634,-1.,3.83393171228034));
#44495=CARTESIAN_POINT('Ctrl Pts',(-0.103866063811634,1.,3.83393171228034));
#44496=CARTESIAN_POINT('Ctrl Pts',(-0.102234506488445,-1.,3.8269873714322));
#44497=CARTESIAN_POINT('Ctrl Pts',(-0.102234506488445,1.,3.8269873714322));
#44498=CARTESIAN_POINT('Ctrl Pts',(-0.100678769650594,-1.,3.82007889742512));
#44499=CARTESIAN_POINT('Ctrl Pts',(-0.100678769650594,1.,3.82007889742512));
#44500=CARTESIAN_POINT('Ctrl Pts',(-0.0992008728095946,-1.,3.81306649386293));
#44501=CARTESIAN_POINT('Ctrl Pts',(-0.0992008728095946,1.,3.81306649386293));
#44502=CARTESIAN_POINT('Ctrl Pts',(-0.0978042222906077,-1.,3.80581088847642));
#44503=CARTESIAN_POINT('Ctrl Pts',(-0.0978042222906077,1.,3.80581088847642));
#44504=CARTESIAN_POINT('Ctrl Pts',(-0.0964949352872846,-1.,3.7982212851376));
#44505=CARTESIAN_POINT('Ctrl Pts',(-0.0964949352872846,1.,3.7982212851376));
#44506=CARTESIAN_POINT('Ctrl Pts',(-0.095282988510107,-1.,3.79030016353186));
#44507=CARTESIAN_POINT('Ctrl Pts',(-0.095282988510107,1.,3.79030016353186));
#44508=CARTESIAN_POINT('Ctrl Pts',(-0.0941840095091746,-1.,3.78220521899366));
#44509=CARTESIAN_POINT('Ctrl Pts',(-0.0941840095091746,1.,3.78220521899366));
#44510=CARTESIAN_POINT('Ctrl Pts',(-0.0932185546204576,-1.,3.77424159971456));
#44511=CARTESIAN_POINT('Ctrl Pts',(-0.0932185546204576,1.,3.77424159971456));
#44512=CARTESIAN_POINT('Ctrl Pts',(-0.0924090589604057,-1.,3.76678860032228));
#44513=CARTESIAN_POINT('Ctrl Pts',(-0.0924090589604057,1.,3.76678860032228));
#44514=CARTESIAN_POINT('Ctrl Pts',(-0.091777308499901,-1.,3.76024199359493));
#44515=CARTESIAN_POINT('Ctrl Pts',(-0.091777308499901,1.,3.76024199359493));
#44516=CARTESIAN_POINT('Ctrl Pts',(-0.0913419622735854,-1.,3.75495560118053));
#44517=CARTESIAN_POINT('Ctrl Pts',(-0.0913419622735854,1.,3.75495560118053));
#44518=CARTESIAN_POINT('Ctrl Pts',(-0.0911154000996408,-1.,3.75116949194125));
#44519=CARTESIAN_POINT('Ctrl Pts',(-0.0911154000996408,1.,3.75116949194125));
#44520=CARTESIAN_POINT('Ctrl Pts',(-0.0911057547504662,-1.,3.74943097853257));
#44521=CARTESIAN_POINT('Ctrl Pts',(-0.0911057547504662,1.,3.74943097853257));
#44522=CARTESIAN_POINT('Ctrl Pts',(-0.0911958743733928,-1.,3.7488701717383));
#44523=CARTESIAN_POINT('Ctrl Pts',(-0.0911958743733928,1.,3.7488701717383));
#44524=CARTESIAN_POINT('Ctrl Pts',(-0.0912992005792093,-1.,3.74882632118923));
#44525=CARTESIAN_POINT('Ctrl Pts',(-0.0912992005792093,1.,3.74882632118923));
#44526=CARTESIAN_POINT('Ctrl Pts',(-0.0913616755937431,-1.,3.74888690736767));
#44527=CARTESIAN_POINT('Ctrl Pts',(-0.0913616755937431,1.,3.74888690736767));
#44528=CARTESIAN_POINT('',(-0.253646344052522,1.,4.1923339003649));
#44529=CARTESIAN_POINT('Ctrl Pts',(-0.253646344052522,1.,4.1923339003649));
#44530=CARTESIAN_POINT('Ctrl Pts',(-0.252860861572841,1.,4.19097151819684));
#44531=CARTESIAN_POINT('Ctrl Pts',(-0.251293239838441,1.,4.18824585245272));
#44532=CARTESIAN_POINT('Ctrl Pts',(-0.248951836912189,1.,4.18415464961466));
#44533=CARTESIAN_POINT('Ctrl Pts',(-0.245850033420019,1.,4.1786943019518));
#44534=CARTESIAN_POINT('Ctrl Pts',(-0.242006283925089,1.,4.17185984411426));
#44535=CARTESIAN_POINT('Ctrl Pts',(-0.238196140934616,1.,4.16501636654877));
#44536=CARTESIAN_POINT('Ctrl Pts',(-0.234419749543208,1.,4.15816389265352));
#44537=CARTESIAN_POINT('Ctrl Pts',(-0.230677299028383,1.,4.15130247434459));
#44538=CARTESIAN_POINT('Ctrl Pts',(-0.226969025060705,1.,4.14443220606869));
#44539=CARTESIAN_POINT('Ctrl Pts',(-0.223295201037886,1.,4.13755320552764));
#44540=CARTESIAN_POINT('Ctrl Pts',(-0.219656126701542,1.,4.13066558697658));
#44541=CARTESIAN_POINT('Ctrl Pts',(-0.216052116898352,1.,4.12376943492132));
#44542=CARTESIAN_POINT('Ctrl Pts',(-0.21248349108719,1.,4.11686478264739));
#44543=CARTESIAN_POINT('Ctrl Pts',(-0.208950559400393,1.,4.10995157639377));
#44544=CARTESIAN_POINT('Ctrl Pts',(-0.205453622198455,1.,4.10302969965728));
#44545=CARTESIAN_POINT('Ctrl Pts',(-0.201992979050136,1.,4.09609903752152));
#44546=CARTESIAN_POINT('Ctrl Pts',(-0.198568934800862,1.,4.08915953359833));
#44547=CARTESIAN_POINT('Ctrl Pts',(-0.195181806054676,1.,4.08221124060322));
#44548=CARTESIAN_POINT('Ctrl Pts',(-0.191831928180991,1.,4.07525439702992));
#44549=CARTESIAN_POINT('Ctrl Pts',(-0.188519658060156,1.,4.06828941192148));
#44550=CARTESIAN_POINT('Ctrl Pts',(-0.185245370038874,1.,4.06131670998469));
#44551=CARTESIAN_POINT('Ctrl Pts',(-0.18200945304852,1.,4.05433660358353));
#44552=CARTESIAN_POINT('Ctrl Pts',(-0.178812307240729,1.,4.04734916719741));
#44553=CARTESIAN_POINT('Ctrl Pts',(-0.175654339673798,1.,4.04035407891222));
#44554=CARTESIAN_POINT('Ctrl Pts',(-0.172535962484514,1.,4.03335057326163));
#44555=CARTESIAN_POINT('Ctrl Pts',(-0.169457601001691,1.,4.02633779703764));
#44556=CARTESIAN_POINT('Ctrl Pts',(-0.166419700015866,1.,4.01931510507167));
#44557=CARTESIAN_POINT('Ctrl Pts',(-0.163422730287457,1.,4.01228237022296));
#44558=CARTESIAN_POINT('Ctrl Pts',(-0.160467194882203,1.,4.00524031064487));
#44559=CARTESIAN_POINT('Ctrl Pts',(-0.15755363438379,1.,3.9981907463185));
#44560=CARTESIAN_POINT('Ctrl Pts',(-0.154682618338548,1.,3.99113582086043));
#44561=CARTESIAN_POINT('Ctrl Pts',(-0.151854737441398,1.,3.98407729850975));
#44562=CARTESIAN_POINT('Ctrl Pts',(-0.149070594803545,1.,3.97701581473644));
#44563=CARTESIAN_POINT('Ctrl Pts',(-0.14633079781452,1.,3.96995018565893));
#44564=CARTESIAN_POINT('Ctrl Pts',(-0.143635947692799,1.,3.96287658098896));
#44565=CARTESIAN_POINT('Ctrl Pts',(-0.140986665829942,1.,3.95579014116894));
#44566=CARTESIAN_POINT('Ctrl Pts',(-0.138383621255161,1.,3.94868667844347));
#44567=CARTESIAN_POINT('Ctrl Pts',(-0.135827558661188,1.,3.94156445130741));
#44568=CARTESIAN_POINT('Ctrl Pts',(-0.133319322794191,1.,3.93442567551042));
#44569=CARTESIAN_POINT('Ctrl Pts',(-0.130859892027802,1.,3.92727876795977));
#44570=CARTESIAN_POINT('Ctrl Pts',(-0.128450341339532,1.,3.92013513251664));
#44571=CARTESIAN_POINT('Ctrl Pts',(-0.126091793324141,1.,3.91300501605411));
#44572=CARTESIAN_POINT('Ctrl Pts',(-0.12378536827238,1.,3.90589336320515));
#44573=CARTESIAN_POINT('Ctrl Pts',(-0.121532144765721,1.,3.89879639336939));
#44574=CARTESIAN_POINT('Ctrl Pts',(-0.11933308819041,1.,3.8916960010517));
#44575=CARTESIAN_POINT('Ctrl Pts',(-0.117189150373134,1.,3.88456590045726));
#44576=CARTESIAN_POINT('Ctrl Pts',(-0.115101426649461,1.,3.87738168405308));
#44577=CARTESIAN_POINT('Ctrl Pts',(-0.113071304914559,1.,3.87013043445001));
#44578=CARTESIAN_POINT('Ctrl Pts',(-0.111100593036267,1.,3.86281867282984));
#44579=CARTESIAN_POINT('Ctrl Pts',(-0.109191717634961,1.,3.85548571496953));
#44580=CARTESIAN_POINT('Ctrl Pts',(-0.107347597812208,1.,3.84819233070391));
#44581=CARTESIAN_POINT('Ctrl Pts',(-0.105571360916593,1.,3.84099658324873));
#44582=CARTESIAN_POINT('Ctrl Pts',(-0.103866063811634,1.,3.83393171228034));
#44583=CARTESIAN_POINT('Ctrl Pts',(-0.102234506488445,1.,3.8269873714322));
#44584=CARTESIAN_POINT('Ctrl Pts',(-0.100678769650594,1.,3.82007889742512));
#44585=CARTESIAN_POINT('Ctrl Pts',(-0.0992008728095946,1.,3.81306649386293));
#44586=CARTESIAN_POINT('Ctrl Pts',(-0.0978042222906077,1.,3.80581088847642));
#44587=CARTESIAN_POINT('Ctrl Pts',(-0.0964949352872846,1.,3.7982212851376));
#44588=CARTESIAN_POINT('Ctrl Pts',(-0.095282988510107,1.,3.79030016353186));
#44589=CARTESIAN_POINT('Ctrl Pts',(-0.0941840095091746,1.,3.78220521899366));
#44590=CARTESIAN_POINT('Ctrl Pts',(-0.0932185546204576,1.,3.77424159971456));
#44591=CARTESIAN_POINT('Ctrl Pts',(-0.0924090589604057,1.,3.76678860032228));
#44592=CARTESIAN_POINT('Ctrl Pts',(-0.091777308499901,1.,3.76024199359493));
#44593=CARTESIAN_POINT('Ctrl Pts',(-0.0913419622735854,1.,3.75495560118053));
#44594=CARTESIAN_POINT('Ctrl Pts',(-0.0911323999576145,1.,3.75145357872511));
#44595=CARTESIAN_POINT('Ctrl Pts',(-0.0911090736804573,1.,3.74976844886494));
#44596=CARTESIAN_POINT('Ctrl Pts',(-0.0911666301806427,1.,3.74911539914664));
#44597=CARTESIAN_POINT('Ctrl Pts',(-0.0912308016409236,1.,3.74892890041021));
#44598=CARTESIAN_POINT('Ctrl Pts',(-0.0912596999148861,1.,3.74888939116259));
#44599=CARTESIAN_POINT('',(-0.253646344052522,0.,4.1923339003649));
#44600=CARTESIAN_POINT('Ctrl Pts',(-0.496218256089212,-1.,3.71702400346349));
#44601=CARTESIAN_POINT('Ctrl Pts',(-0.496218256089212,1.,3.71702400346349));
#44602=CARTESIAN_POINT('Ctrl Pts',(-0.496270484166409,-1.,3.7169543899574));
#44603=CARTESIAN_POINT('Ctrl Pts',(-0.496270484166409,1.,3.7169543899574));
#44604=CARTESIAN_POINT('Ctrl Pts',(-0.49637939799264,-1.,3.71698153685602));
#44605=CARTESIAN_POINT('Ctrl Pts',(-0.49637939799264,1.,3.71698153685602));
#44606=CARTESIAN_POINT('Ctrl Pts',(-0.496556137604532,-1.,3.71752134137482));
#44607=CARTESIAN_POINT('Ctrl Pts',(-0.496556137604532,1.,3.71752134137482));
#44608=CARTESIAN_POINT('Ctrl Pts',(-0.496818574420596,-1.,3.71923995966302));
#44609=CARTESIAN_POINT('Ctrl Pts',(-0.496818574420596,1.,3.71923995966302));
#44610=CARTESIAN_POINT('Ctrl Pts',(-0.497187079575988,-1.,3.72301489774398));
#44611=CARTESIAN_POINT('Ctrl Pts',(-0.497187079575988,1.,3.72301489774398));
#44612=CARTESIAN_POINT('Ctrl Pts',(-0.497584067153049,-1.,3.72830430904606));
#44613=CARTESIAN_POINT('Ctrl Pts',(-0.497584067153049,1.,3.72830430904606));
#44614=CARTESIAN_POINT('Ctrl Pts',(-0.497984209510024,-1.,3.73486914372449));
#44615=CARTESIAN_POINT('Ctrl Pts',(-0.497984209510024,1.,3.73486914372449));
#44616=CARTESIAN_POINT('Ctrl Pts',(-0.498350586057692,-1.,3.74235701734714));
#44617=CARTESIAN_POINT('Ctrl Pts',(-0.498350586057692,1.,3.74235701734714));
#44618=CARTESIAN_POINT('Ctrl Pts',(-0.498642802042606,-1.,3.75037362167839));
#44619=CARTESIAN_POINT('Ctrl Pts',(-0.498642802042606,1.,3.75037362167839));
#44620=CARTESIAN_POINT('Ctrl Pts',(-0.498823681615422,-1.,3.75854082221053));
#44621=CARTESIAN_POINT('Ctrl Pts',(-0.498823681615422,1.,3.75854082221053));
#44622=CARTESIAN_POINT('Ctrl Pts',(-0.498865792335291,-1.,3.76655401191229));
#44623=CARTESIAN_POINT('Ctrl Pts',(-0.498865792335291,1.,3.76655401191229));
#44624=CARTESIAN_POINT('Ctrl Pts',(-0.498759900365892,-1.,3.77425499225255));
#44625=CARTESIAN_POINT('Ctrl Pts',(-0.498759900365892,1.,3.77425499225255));
#44626=CARTESIAN_POINT('Ctrl Pts',(-0.498515471679585,-1.,3.78163975337356));
#44627=CARTESIAN_POINT('Ctrl Pts',(-0.498515471679585,1.,3.78163975337356));
#44628=CARTESIAN_POINT('Ctrl Pts',(-0.498152751800958,-1.,3.78879701661264));
#44629=CARTESIAN_POINT('Ctrl Pts',(-0.498152751800958,1.,3.78879701661264));
#44630=CARTESIAN_POINT('Ctrl Pts',(-0.497696892100625,-1.,3.79586380669994));
#44631=CARTESIAN_POINT('Ctrl Pts',(-0.497696892100625,1.,3.79586380669994));
#44632=CARTESIAN_POINT('Ctrl Pts',(-0.497171756201052,-1.,3.80297788298514));
#44633=CARTESIAN_POINT('Ctrl Pts',(-0.497171756201052,1.,3.80297788298514));
#44634=CARTESIAN_POINT('Ctrl Pts',(-0.496592643443704,-1.,3.81022254090839));
#44635=CARTESIAN_POINT('Ctrl Pts',(-0.496592643443704,1.,3.81022254090839));
#44636=CARTESIAN_POINT('Ctrl Pts',(-0.49596393787548,-1.,3.81760756144025));
#44637=CARTESIAN_POINT('Ctrl Pts',(-0.49596393787548,1.,3.81760756144025));
#44638=CARTESIAN_POINT('Ctrl Pts',(-0.495283458893837,-1.,3.82509963594103));
#44639=CARTESIAN_POINT('Ctrl Pts',(-0.495283458893837,1.,3.82509963594103));
#44640=CARTESIAN_POINT('Ctrl Pts',(-0.494545212256401,-1.,3.83264092682431));
#44641=CARTESIAN_POINT('Ctrl Pts',(-0.494545212256401,1.,3.83264092682431));
#44642=CARTESIAN_POINT('Ctrl Pts',(-0.493742574629135,-1.,3.84017095578451));
#44643=CARTESIAN_POINT('Ctrl Pts',(-0.493742574629135,1.,3.84017095578451));
#44644=CARTESIAN_POINT('Ctrl Pts',(-0.492871792414141,-1.,3.84765051147999));
#44645=CARTESIAN_POINT('Ctrl Pts',(-0.492871792414141,1.,3.84765051147999));
#44646=CARTESIAN_POINT('Ctrl Pts',(-0.491933631083813,-1.,3.85507287020263));
#44647=CARTESIAN_POINT('Ctrl Pts',(-0.491933631083813,1.,3.85507287020263));
#44648=CARTESIAN_POINT('Ctrl Pts',(-0.490931482170891,-1.,3.86245057319246));
#44649=CARTESIAN_POINT('Ctrl Pts',(-0.490931482170891,1.,3.86245057319246));
#44650=CARTESIAN_POINT('Ctrl Pts',(-0.489870245704918,-1.,3.86980755613707));
#44651=CARTESIAN_POINT('Ctrl Pts',(-0.489870245704918,1.,3.86980755613707));
#44652=CARTESIAN_POINT('Ctrl Pts',(-0.488754973798274,-1.,3.87716963231109));
#44653=CARTESIAN_POINT('Ctrl Pts',(-0.488754973798274,1.,3.87716963231109));
#44654=CARTESIAN_POINT('Ctrl Pts',(-0.487589452275155,-1.,3.88455453328138));
#44655=CARTESIAN_POINT('Ctrl Pts',(-0.487589452275155,1.,3.88455453328138));
#44656=CARTESIAN_POINT('Ctrl Pts',(-0.486375337854103,-1.,3.89196582437552));
#44657=CARTESIAN_POINT('Ctrl Pts',(-0.486375337854103,1.,3.89196582437552));
#44658=CARTESIAN_POINT('Ctrl Pts',(-0.485112963522222,-1.,3.89939844658513));
#44659=CARTESIAN_POINT('Ctrl Pts',(-0.485112963522222,1.,3.89939844658513));
#44660=CARTESIAN_POINT('Ctrl Pts',(-0.48380183508915,-1.,3.90684210358056));
#44661=CARTESIAN_POINT('Ctrl Pts',(-0.48380183508915,1.,3.90684210358056));
#44662=CARTESIAN_POINT('Ctrl Pts',(-0.482441230340713,-1.,3.91428536373751));
#44663=CARTESIAN_POINT('Ctrl Pts',(-0.482441230340713,1.,3.91428536373751));
#44664=CARTESIAN_POINT('Ctrl Pts',(-0.481030798910748,-1.,3.92171976072341));
#44665=CARTESIAN_POINT('Ctrl Pts',(-0.481030798910748,1.,3.92171976072341));
#44666=CARTESIAN_POINT('Ctrl Pts',(-0.479571028525579,-1.,3.92914297392071));
#44667=CARTESIAN_POINT('Ctrl Pts',(-0.479571028525579,1.,3.92914297392071));
#44668=CARTESIAN_POINT('Ctrl Pts',(-0.478062927140965,-1.,3.93655660689819));
#44669=CARTESIAN_POINT('Ctrl Pts',(-0.478062927140965,1.,3.93655660689819));
#44670=CARTESIAN_POINT('Ctrl Pts',(-0.476507810658537,-1.,3.94396469119383));
#44671=CARTESIAN_POINT('Ctrl Pts',(-0.476507810658537,1.,3.94396469119383));
#44672=CARTESIAN_POINT('Ctrl Pts',(-0.47490705302179,-1.,3.95137192932897));
#44673=CARTESIAN_POINT('Ctrl Pts',(-0.47490705302179,1.,3.95137192932897));
#44674=CARTESIAN_POINT('Ctrl Pts',(-0.473261847236297,-1.,3.95878201038338));
#44675=CARTESIAN_POINT('Ctrl Pts',(-0.473261847236297,1.,3.95878201038338));
#44676=CARTESIAN_POINT('Ctrl Pts',(-0.471572978413504,-1.,3.96619600864643));
#44677=CARTESIAN_POINT('Ctrl Pts',(-0.471572978413504,1.,3.96619600864643));
#44678=CARTESIAN_POINT('Ctrl Pts',(-0.469840942829896,-1.,3.97361320212436));
#44679=CARTESIAN_POINT('Ctrl Pts',(-0.469840942829896,1.,3.97361320212436));
#44680=CARTESIAN_POINT('Ctrl Pts',(-0.468066047920157,-1.,3.98103175589371));
#44681=CARTESIAN_POINT('Ctrl Pts',(-0.468066047920157,1.,3.98103175589371));
#44682=CARTESIAN_POINT('Ctrl Pts',(-0.46624852088304,-1.,3.98844946363262));
#44683=CARTESIAN_POINT('Ctrl Pts',(-0.46624852088304,1.,3.98844946363262));
#44684=CARTESIAN_POINT('Ctrl Pts',(-0.464388610938975,-1.,3.9958644432011));
#44685=CARTESIAN_POINT('Ctrl Pts',(-0.464388610938975,1.,3.9958644432011));
#44686=CARTESIAN_POINT('Ctrl Pts',(-0.462486702616205,-1.,4.00327590659075));
#44687=CARTESIAN_POINT('Ctrl Pts',(-0.462486702616205,1.,4.00327590659075));
#44688=CARTESIAN_POINT('Ctrl Pts',(-0.460543280768515,-1.,4.01068390573399));
#44689=CARTESIAN_POINT('Ctrl Pts',(-0.460543280768515,1.,4.01068390573399));
#44690=CARTESIAN_POINT('Ctrl Pts',(-0.458558885636946,-1.,4.01808900827587));
#44691=CARTESIAN_POINT('Ctrl Pts',(-0.458558885636946,1.,4.01808900827587));
#44692=CARTESIAN_POINT('Ctrl Pts',(-0.456534070784951,-1.,4.02549199038394));
#44693=CARTESIAN_POINT('Ctrl Pts',(-0.456534070784951,1.,4.02549199038394));
#44694=CARTESIAN_POINT('Ctrl Pts',(-0.454469363020542,-1.,4.03289354362794));
#44695=CARTESIAN_POINT('Ctrl Pts',(-0.454469363020542,1.,4.03289354362794));
#44696=CARTESIAN_POINT('Ctrl Pts',(-0.452365214748893,-1.,4.04029392228049));
#44697=CARTESIAN_POINT('Ctrl Pts',(-0.452365214748893,1.,4.04029392228049));
#44698=CARTESIAN_POINT('Ctrl Pts',(-0.450222009543927,-1.,4.0476929901813));
#44699=CARTESIAN_POINT('Ctrl Pts',(-0.450222009543927,1.,4.0476929901813));
#44700=CARTESIAN_POINT('Ctrl Pts',(-0.448040082684115,-1.,4.0550903779696));
#44701=CARTESIAN_POINT('Ctrl Pts',(-0.448040082684115,1.,4.0550903779696));
#44702=CARTESIAN_POINT('Ctrl Pts',(-0.445819737468538,-1.,4.06248560760659));
#44703=CARTESIAN_POINT('Ctrl Pts',(-0.445819737468538,1.,4.06248560760659));
#44704=CARTESIAN_POINT('Ctrl Pts',(-0.443561262395333,-1.,4.0698782192569));
#44705=CARTESIAN_POINT('Ctrl Pts',(-0.443561262395333,1.,4.0698782192569));
#44706=CARTESIAN_POINT('Ctrl Pts',(-0.441264951396361,-1.,4.07726792490016));
#44707=CARTESIAN_POINT('Ctrl Pts',(-0.441264951396361,1.,4.07726792490016));
#44708=CARTESIAN_POINT('Ctrl Pts',(-0.43893110893128,-1.,4.08465462294273));
#44709=CARTESIAN_POINT('Ctrl Pts',(-0.43893110893128,1.,4.08465462294273));
#44710=CARTESIAN_POINT('Ctrl Pts',(-0.436560044913482,-1.,4.09203832139089));
#44711=CARTESIAN_POINT('Ctrl Pts',(-0.436560044913482,1.,4.09203832139089));
#44712=CARTESIAN_POINT('Ctrl Pts',(-0.43415207320046,-1.,4.09941908688373));
#44713=CARTESIAN_POINT('Ctrl Pts',(-0.43415207320046,1.,4.09941908688373));
#44714=CARTESIAN_POINT('Ctrl Pts',(-0.431707508679884,-1.,4.10679698750336));
#44715=CARTESIAN_POINT('Ctrl Pts',(-0.431707508679884,1.,4.10679698750336));
#44716=CARTESIAN_POINT('Ctrl Pts',(-0.429226666075845,-1.,4.11417202783267));
#44717=CARTESIAN_POINT('Ctrl Pts',(-0.429226666075845,1.,4.11417202783267));
#44718=CARTESIAN_POINT('Ctrl Pts',(-0.426709855707001,-1.,4.12154412502007));
#44719=CARTESIAN_POINT('Ctrl Pts',(-0.426709855707001,1.,4.12154412502007));
#44720=CARTESIAN_POINT('Ctrl Pts',(-0.424157375323975,-1.,4.12891314634572));
#44721=CARTESIAN_POINT('Ctrl Pts',(-0.424157375323975,1.,4.12891314634572));
#44722=CARTESIAN_POINT('Ctrl Pts',(-0.421569503104513,-1.,4.13627893207002));
#44723=CARTESIAN_POINT('Ctrl Pts',(-0.421569503104513,1.,4.13627893207002));
#44724=CARTESIAN_POINT('Ctrl Pts',(-0.418946490667703,-1.,4.14364132317121));
#44725=CARTESIAN_POINT('Ctrl Pts',(-0.418946490667703,1.,4.14364132317121));
#44726=CARTESIAN_POINT('Ctrl Pts',(-0.416288556008012,-1.,4.15100018949965));
#44727=CARTESIAN_POINT('Ctrl Pts',(-0.416288556008012,1.,4.15100018949965));
#44728=CARTESIAN_POINT('Ctrl Pts',(-0.41359587795147,-1.,4.15835545017202));
#44729=CARTESIAN_POINT('Ctrl Pts',(-0.41359587795147,1.,4.15835545017202));
#44730=CARTESIAN_POINT('Ctrl Pts',(-0.410868596146414,-1.,4.16570705938425));
#44731=CARTESIAN_POINT('Ctrl Pts',(-0.410868596146414,1.,4.16570705938425));
#44732=CARTESIAN_POINT('Ctrl Pts',(-0.408659167568273,-1.,4.17158541007977));
#44733=CARTESIAN_POINT('Ctrl Pts',(-0.408659167568273,1.,4.17158541007977));
#44734=CARTESIAN_POINT('Ctrl Pts',(-0.406986596325455,-1.,4.17599251954382));
#44735=CARTESIAN_POINT('Ctrl Pts',(-0.406986596325455,1.,4.17599251954382));
#44736=CARTESIAN_POINT('Ctrl Pts',(-0.40586466267921,-1.,4.17892985789466));
#44737=CARTESIAN_POINT('Ctrl Pts',(-0.40586466267921,1.,4.17892985789466));
#44738=CARTESIAN_POINT('Ctrl Pts',(-0.40530197431835,-1.,4.18039834341342));
#44739=CARTESIAN_POINT('Ctrl Pts',(-0.40530197431835,1.,4.18039834341342));
#44740=CARTESIAN_POINT('',(-0.496319364827592,1.,3.71701050416825));
#44741=CARTESIAN_POINT('Ctrl Pts',(-0.496319364827592,-1.,3.71701050416825));
#44742=CARTESIAN_POINT('Ctrl Pts',(-0.496319364827592,-0.666666666666667,
3.71701050416825));
#44743=CARTESIAN_POINT('Ctrl Pts',(-0.496319364827592,-0.333333333333333,
3.71701050416825));
#44744=CARTESIAN_POINT('Ctrl Pts',(-0.496319364827592,0.333333333333333,
3.71701050416825));
#44745=CARTESIAN_POINT('Ctrl Pts',(-0.496319364827592,0.666666666666667,
3.71701050416825));
#44746=CARTESIAN_POINT('Ctrl Pts',(-0.496319364827592,1.,3.71701050416825));
#44747=CARTESIAN_POINT('',(-0.40530197431835,1.,4.18039834341342));
#44748=CARTESIAN_POINT('',(-0.40530197431835,0.,4.18039834341342));
#44749=CARTESIAN_POINT('Ctrl Pts',(-0.496319364827592,1.,3.71701050416825));
#44750=CARTESIAN_POINT('Ctrl Pts',(-0.496354087924313,1.,3.71704500630495));
#44751=CARTESIAN_POINT('Ctrl Pts',(-0.496446644158005,1.,3.71721917030355));
#44752=CARTESIAN_POINT('Ctrl Pts',(-0.496605651525989,1.,3.71785517607549));
#44753=CARTESIAN_POINT('Ctrl Pts',(-0.496846224822564,1.,3.71952320822499));
#44754=CARTESIAN_POINT('Ctrl Pts',(-0.497187079575988,1.,3.72301489774398));
#44755=CARTESIAN_POINT('Ctrl Pts',(-0.497584067153049,1.,3.72830430904606));
#44756=CARTESIAN_POINT('Ctrl Pts',(-0.497984209510024,1.,3.73486914372449));
#44757=CARTESIAN_POINT('Ctrl Pts',(-0.498350586057692,1.,3.74235701734714));
#44758=CARTESIAN_POINT('Ctrl Pts',(-0.498642802042606,1.,3.75037362167839));
#44759=CARTESIAN_POINT('Ctrl Pts',(-0.498823681615422,1.,3.75854082221053));
#44760=CARTESIAN_POINT('Ctrl Pts',(-0.498865792335291,1.,3.76655401191229));
#44761=CARTESIAN_POINT('Ctrl Pts',(-0.498759900365892,1.,3.77425499225255));
#44762=CARTESIAN_POINT('Ctrl Pts',(-0.498515471679585,1.,3.78163975337356));
#44763=CARTESIAN_POINT('Ctrl Pts',(-0.498152751800958,1.,3.78879701661264));
#44764=CARTESIAN_POINT('Ctrl Pts',(-0.497696892100625,1.,3.79586380669994));
#44765=CARTESIAN_POINT('Ctrl Pts',(-0.497171756201052,1.,3.80297788298514));
#44766=CARTESIAN_POINT('Ctrl Pts',(-0.496592643443704,1.,3.81022254090839));
#44767=CARTESIAN_POINT('Ctrl Pts',(-0.49596393787548,1.,3.81760756144025));
#44768=CARTESIAN_POINT('Ctrl Pts',(-0.495283458893837,1.,3.82509963594103));
#44769=CARTESIAN_POINT('Ctrl Pts',(-0.494545212256401,1.,3.83264092682431));
#44770=CARTESIAN_POINT('Ctrl Pts',(-0.493742574629135,1.,3.84017095578451));
#44771=CARTESIAN_POINT('Ctrl Pts',(-0.492871792414141,1.,3.84765051147999));
#44772=CARTESIAN_POINT('Ctrl Pts',(-0.491933631083813,1.,3.85507287020263));
#44773=CARTESIAN_POINT('Ctrl Pts',(-0.490931482170891,1.,3.86245057319246));
#44774=CARTESIAN_POINT('Ctrl Pts',(-0.489870245704918,1.,3.86980755613707));
#44775=CARTESIAN_POINT('Ctrl Pts',(-0.488754973798274,1.,3.87716963231109));
#44776=CARTESIAN_POINT('Ctrl Pts',(-0.487589452275155,1.,3.88455453328138));
#44777=CARTESIAN_POINT('Ctrl Pts',(-0.486375337854103,1.,3.89196582437552));
#44778=CARTESIAN_POINT('Ctrl Pts',(-0.485112963522222,1.,3.89939844658513));
#44779=CARTESIAN_POINT('Ctrl Pts',(-0.48380183508915,1.,3.90684210358056));
#44780=CARTESIAN_POINT('Ctrl Pts',(-0.482441230340713,1.,3.91428536373751));
#44781=CARTESIAN_POINT('Ctrl Pts',(-0.481030798910748,1.,3.92171976072341));
#44782=CARTESIAN_POINT('Ctrl Pts',(-0.479571028525579,1.,3.92914297392071));
#44783=CARTESIAN_POINT('Ctrl Pts',(-0.478062927140965,1.,3.93655660689819));
#44784=CARTESIAN_POINT('Ctrl Pts',(-0.476507810658537,1.,3.94396469119383));
#44785=CARTESIAN_POINT('Ctrl Pts',(-0.47490705302179,1.,3.95137192932897));
#44786=CARTESIAN_POINT('Ctrl Pts',(-0.473261847236297,1.,3.95878201038338));
#44787=CARTESIAN_POINT('Ctrl Pts',(-0.471572978413504,1.,3.96619600864643));
#44788=CARTESIAN_POINT('Ctrl Pts',(-0.469840942829896,1.,3.97361320212436));
#44789=CARTESIAN_POINT('Ctrl Pts',(-0.468066047920157,1.,3.98103175589371));
#44790=CARTESIAN_POINT('Ctrl Pts',(-0.46624852088304,1.,3.98844946363262));
#44791=CARTESIAN_POINT('Ctrl Pts',(-0.464388610938975,1.,3.9958644432011));
#44792=CARTESIAN_POINT('Ctrl Pts',(-0.462486702616205,1.,4.00327590659075));
#44793=CARTESIAN_POINT('Ctrl Pts',(-0.460543280768515,1.,4.01068390573399));
#44794=CARTESIAN_POINT('Ctrl Pts',(-0.458558885636946,1.,4.01808900827587));
#44795=CARTESIAN_POINT('Ctrl Pts',(-0.456534070784951,1.,4.02549199038394));
#44796=CARTESIAN_POINT('Ctrl Pts',(-0.454469363020542,1.,4.03289354362794));
#44797=CARTESIAN_POINT('Ctrl Pts',(-0.452365214748893,1.,4.04029392228049));
#44798=CARTESIAN_POINT('Ctrl Pts',(-0.450222009543927,1.,4.0476929901813));
#44799=CARTESIAN_POINT('Ctrl Pts',(-0.448040082684115,1.,4.0550903779696));
#44800=CARTESIAN_POINT('Ctrl Pts',(-0.445819737468538,1.,4.06248560760659));
#44801=CARTESIAN_POINT('Ctrl Pts',(-0.443561262395333,1.,4.0698782192569));
#44802=CARTESIAN_POINT('Ctrl Pts',(-0.441264951396361,1.,4.07726792490016));
#44803=CARTESIAN_POINT('Ctrl Pts',(-0.43893110893128,1.,4.08465462294273));
#44804=CARTESIAN_POINT('Ctrl Pts',(-0.436560044913482,1.,4.09203832139089));
#44805=CARTESIAN_POINT('Ctrl Pts',(-0.43415207320046,1.,4.09941908688373));
#44806=CARTESIAN_POINT('Ctrl Pts',(-0.431707508679884,1.,4.10679698750336));
#44807=CARTESIAN_POINT('Ctrl Pts',(-0.429226666075845,1.,4.11417202783267));
#44808=CARTESIAN_POINT('Ctrl Pts',(-0.426709855707001,1.,4.12154412502007));
#44809=CARTESIAN_POINT('Ctrl Pts',(-0.424157375323975,1.,4.12891314634572));
#44810=CARTESIAN_POINT('Ctrl Pts',(-0.421569503104513,1.,4.13627893207002));
#44811=CARTESIAN_POINT('Ctrl Pts',(-0.418946490667703,1.,4.14364132317121));
#44812=CARTESIAN_POINT('Ctrl Pts',(-0.416288556008012,1.,4.15100018949965));
#44813=CARTESIAN_POINT('Ctrl Pts',(-0.41359587795147,1.,4.15835545017202));
#44814=CARTESIAN_POINT('Ctrl Pts',(-0.410868596146414,1.,4.16570705938425));
#44815=CARTESIAN_POINT('Ctrl Pts',(-0.408659167568273,1.,4.17158541007977));
#44816=CARTESIAN_POINT('Ctrl Pts',(-0.406986596325455,1.,4.17599251954382));
#44817=CARTESIAN_POINT('Ctrl Pts',(-0.40586466267921,1.,4.17892985789466));
#44818=CARTESIAN_POINT('Ctrl Pts',(-0.40530197431835,1.,4.18039834341342));
#44819=CARTESIAN_POINT('Origin',(-0.40530197431835,0.,4.18039834341342));
#44820=CARTESIAN_POINT('',(-0.253646344052522,1.,4.1923339003649));
#44821=CARTESIAN_POINT('Origin',(0.,0.,0.));
#44822=CARTESIAN_POINT('',(-0.676591647973661,1.,3.68845817949618));
#44823=CARTESIAN_POINT('Origin',(0.,1.,0.));
#44824=CARTESIAN_POINT('Ctrl Pts',(-0.676591647973661,1.,3.68845817949618));
#44825=CARTESIAN_POINT('Ctrl Pts',(-0.676591647973661,0.666666666666667,
3.68845817949618));
#44826=CARTESIAN_POINT('Ctrl Pts',(-0.676591647973661,0.333333333333333,
3.68845817949618));
#44827=CARTESIAN_POINT('Ctrl Pts',(-0.676591647973661,-0.333333333333333,
3.68845817949618));
#44828=CARTESIAN_POINT('Ctrl Pts',(-0.676591647973661,-0.666666666666667,
3.68845817949618));
#44829=CARTESIAN_POINT('Ctrl Pts',(-0.676591647973661,-1.,3.68845817949618));
#44830=CARTESIAN_POINT('Ctrl Pts',(-0.906349047628866,-1.,4.10104028313088));
#44831=CARTESIAN_POINT('Ctrl Pts',(-0.906349047628866,1.,4.10104028313088));
#44832=CARTESIAN_POINT('Ctrl Pts',(-0.905360112216302,-1.,4.09981755067956));
#44833=CARTESIAN_POINT('Ctrl Pts',(-0.905360112216302,1.,4.09981755067956));
#44834=CARTESIAN_POINT('Ctrl Pts',(-0.903385402444213,-1.,4.09737067247114));
#44835=CARTESIAN_POINT('Ctrl Pts',(-0.903385402444213,1.,4.09737067247114));
#44836=CARTESIAN_POINT('Ctrl Pts',(-0.900432820945975,-1.,4.09369611524319));
#44837=CARTESIAN_POINT('Ctrl Pts',(-0.900432820945975,1.,4.09369611524319));
#44838=CARTESIAN_POINT('Ctrl Pts',(-0.896515019236368,-1.,4.08878822249095));
#44839=CARTESIAN_POINT('Ctrl Pts',(-0.896515019236368,1.,4.08878822249095));
#44840=CARTESIAN_POINT('Ctrl Pts',(-0.891649447920401,-1.,4.08263920306651));
#44841=CARTESIAN_POINT('Ctrl Pts',(-0.891649447920401,1.,4.08263920306651));
#44842=CARTESIAN_POINT('Ctrl Pts',(-0.886815658360739,-1.,4.07647601774639));
#44843=CARTESIAN_POINT('Ctrl Pts',(-0.886815658360739,1.,4.07647601774639));
#44844=CARTESIAN_POINT('Ctrl Pts',(-0.882013797525916,-1.,4.07029866694292));
#44845=CARTESIAN_POINT('Ctrl Pts',(-0.882013797525916,1.,4.07029866694292));
#44846=CARTESIAN_POINT('Ctrl Pts',(-0.877244060484595,-1.,4.06410717232347));
#44847=CARTESIAN_POINT('Ctrl Pts',(-0.877244060484595,1.,4.06410717232347));
#44848=CARTESIAN_POINT('Ctrl Pts',(-0.872506694780563,-1.,4.05790159030495));
#44849=CARTESIAN_POINT('Ctrl Pts',(-0.872506694780563,1.,4.05790159030495));
#44850=CARTESIAN_POINT('Ctrl Pts',(-0.867801988858176,-1.,4.05168199437128));
#44851=CARTESIAN_POINT('Ctrl Pts',(-0.867801988858176,1.,4.05168199437128));
#44852=CARTESIAN_POINT('Ctrl Pts',(-0.863130256642173,-1.,4.04544845048097));
#44853=CARTESIAN_POINT('Ctrl Pts',(-0.863130256642173,1.,4.04544845048097));
#44854=CARTESIAN_POINT('Ctrl Pts',(-0.858491822322571,-1.,4.03920099284658));
#44855=CARTESIAN_POINT('Ctrl Pts',(-0.858491822322571,1.,4.03920099284658));
#44856=CARTESIAN_POINT('Ctrl Pts',(-0.853887006632178,-1.,4.03293960436945));
#44857=CARTESIAN_POINT('Ctrl Pts',(-0.853887006632178,1.,4.03293960436945));
#44858=CARTESIAN_POINT('Ctrl Pts',(-0.849316107475012,-1.,4.02666418343508));
#44859=CARTESIAN_POINT('Ctrl Pts',(-0.849316107475012,1.,4.02666418343508));
#44860=CARTESIAN_POINT('Ctrl Pts',(-0.844779403288517,-1.,4.02037456798787));
#44861=CARTESIAN_POINT('Ctrl Pts',(-0.844779403288517,1.,4.02037456798787));
#44862=CARTESIAN_POINT('Ctrl Pts',(-0.84027717197638,-1.,4.01407059766338));
#44863=CARTESIAN_POINT('Ctrl Pts',(-0.84027717197638,1.,4.01407059766338));
#44864=CARTESIAN_POINT('Ctrl Pts',(-0.835809705809822,-1.,4.00775216907934));
#44865=CARTESIAN_POINT('Ctrl Pts',(-0.835809705809822,1.,4.00775216907934));
#44866=CARTESIAN_POINT('Ctrl Pts',(-0.831377325741487,-1.,4.00141928477447));
#44867=CARTESIAN_POINT('Ctrl Pts',(-0.831377325741487,1.,4.00141928477447));
#44868=CARTESIAN_POINT('Ctrl Pts',(-0.826980400320473,-1.,3.99507212784289));
#44869=CARTESIAN_POINT('Ctrl Pts',(-0.826980400320473,1.,3.99507212784289));
#44870=CARTESIAN_POINT('Ctrl Pts',(-0.822619346021769,-1.,3.98871104646328));
#44871=CARTESIAN_POINT('Ctrl Pts',(-0.822619346021769,1.,3.98871104646328));
#44872=CARTESIAN_POINT('Ctrl Pts',(-0.818294599022033,-1.,3.98233640155287));
#44873=CARTESIAN_POINT('Ctrl Pts',(-0.818294599022033,1.,3.98233640155287));
#44874=CARTESIAN_POINT('Ctrl Pts',(-0.814006592328737,-1.,3.97594844078763));
#44875=CARTESIAN_POINT('Ctrl Pts',(-0.814006592328737,1.,3.97594844078763));
#44876=CARTESIAN_POINT('Ctrl Pts',(-0.809755732818134,-1.,3.96954717513251));
#44877=CARTESIAN_POINT('Ctrl Pts',(-0.809755732818134,1.,3.96954717513251));
#44878=CARTESIAN_POINT('Ctrl Pts',(-0.805542372178496,-1.,3.96313222295874));
#44879=CARTESIAN_POINT('Ctrl Pts',(-0.805542372178496,1.,3.96313222295874));
#44880=CARTESIAN_POINT('Ctrl Pts',(-0.801366797727206,-1.,3.95670276375176));
#44881=CARTESIAN_POINT('Ctrl Pts',(-0.801366797727206,1.,3.95670276375176));
#44882=CARTESIAN_POINT('Ctrl Pts',(-0.797229296085438,-1.,3.95025788827189));
#44883=CARTESIAN_POINT('Ctrl Pts',(-0.797229296085438,1.,3.95025788827189));
#44884=CARTESIAN_POINT('Ctrl Pts',(-0.793130205641017,-1.,3.94379688971307));
#44885=CARTESIAN_POINT('Ctrl Pts',(-0.793130205641017,1.,3.94379688971307));
#44886=CARTESIAN_POINT('Ctrl Pts',(-0.789069971469323,-1.,3.93731956885671));
#44887=CARTESIAN_POINT('Ctrl Pts',(-0.789069971469323,1.,3.93731956885671));
#44888=CARTESIAN_POINT('Ctrl Pts',(-0.785049202786458,-1.,3.93082655631768));
#44889=CARTESIAN_POINT('Ctrl Pts',(-0.785049202786458,1.,3.93082655631768));
#44890=CARTESIAN_POINT('Ctrl Pts',(-0.781068718228395,-1.,3.92431956510418));
#44891=CARTESIAN_POINT('Ctrl Pts',(-0.781068718228395,1.,3.92431956510418));
#44892=CARTESIAN_POINT('Ctrl Pts',(-0.777129415664915,-1.,3.91780062334464));
#44893=CARTESIAN_POINT('Ctrl Pts',(-0.777129415664915,1.,3.91780062334464));
#44894=CARTESIAN_POINT('Ctrl Pts',(-0.773232154506305,-1.,3.91127138115238));
#44895=CARTESIAN_POINT('Ctrl Pts',(-0.773232154506305,1.,3.91127138115238));
#44896=CARTESIAN_POINT('Ctrl Pts',(-0.769377629847877,-1.,3.90473237182634));
#44897=CARTESIAN_POINT('Ctrl Pts',(-0.769377629847877,1.,3.90473237182634));
#44898=CARTESIAN_POINT('Ctrl Pts',(-0.765566256401306,-1.,3.89818233104381));
#44899=CARTESIAN_POINT('Ctrl Pts',(-0.765566256401306,1.,3.89818233104381));
#44900=CARTESIAN_POINT('Ctrl Pts',(-0.761798028793978,-1.,3.89161738162245));
#44901=CARTESIAN_POINT('Ctrl Pts',(-0.761798028793978,1.,3.89161738162245));
#44902=CARTESIAN_POINT('Ctrl Pts',(-0.758072800564799,-1.,3.88503262662684));
#44903=CARTESIAN_POINT('Ctrl Pts',(-0.758072800564799,1.,3.88503262662684));
#44904=CARTESIAN_POINT('Ctrl Pts',(-0.754390577396847,-1.,3.87842382520058));
#44905=CARTESIAN_POINT('Ctrl Pts',(-0.754390577396847,1.,3.87842382520058));
#44906=CARTESIAN_POINT('Ctrl Pts',(-0.750751822383024,-1.,3.87178914078372));
#44907=CARTESIAN_POINT('Ctrl Pts',(-0.750751822383024,1.,3.87178914078372));
#44908=CARTESIAN_POINT('Ctrl Pts',(-0.747157716488884,-1.,3.86513062969896));
#44909=CARTESIAN_POINT('Ctrl Pts',(-0.747157716488884,1.,3.86513062969896));
#44910=CARTESIAN_POINT('Ctrl Pts',(-0.743610542737042,-1.,3.85845645217611));
#44911=CARTESIAN_POINT('Ctrl Pts',(-0.743610542737042,1.,3.85845645217611));
#44912=CARTESIAN_POINT('Ctrl Pts',(-0.740113146827176,-1.,3.85177770351237));
#44913=CARTESIAN_POINT('Ctrl Pts',(-0.740113146827176,1.,3.85177770351237));
#44914=CARTESIAN_POINT('Ctrl Pts',(-0.736668240497151,-1.,3.84510432881231));
#44915=CARTESIAN_POINT('Ctrl Pts',(-0.736668240497151,1.,3.84510432881231));
#44916=CARTESIAN_POINT('Ctrl Pts',(-0.73327770375609,-1.,3.83844103658016));
#44917=CARTESIAN_POINT('Ctrl Pts',(-0.73327770375609,1.,3.83844103658016));
#44918=CARTESIAN_POINT('Ctrl Pts',(-0.729942010490146,-1.,3.8317839240337));
#44919=CARTESIAN_POINT('Ctrl Pts',(-0.729942010490146,1.,3.8317839240337));
#44920=CARTESIAN_POINT('Ctrl Pts',(-0.726659281876608,-1.,3.82511495756682));
#44921=CARTESIAN_POINT('Ctrl Pts',(-0.726659281876608,1.,3.82511495756682));
#44922=CARTESIAN_POINT('Ctrl Pts',(-0.723426346019349,-1.,3.81840802610795));
#44923=CARTESIAN_POINT('Ctrl Pts',(-0.723426346019349,1.,3.81840802610795));
#44924=CARTESIAN_POINT('Ctrl Pts',(-0.720240466589172,-1.,3.81163885127309));
#44925=CARTESIAN_POINT('Ctrl Pts',(-0.720240466589172,1.,3.81163885127309));
#44926=CARTESIAN_POINT('Ctrl Pts',(-0.717100993669091,-1.,3.80479445759296));
#44927=CARTESIAN_POINT('Ctrl Pts',(-0.717100993669091,1.,3.80479445759296));
#44928=CARTESIAN_POINT('Ctrl Pts',(-0.714010733006677,-1.,3.79788100314994));
#44929=CARTESIAN_POINT('Ctrl Pts',(-0.714010733006677,1.,3.79788100314994));
#44930=CARTESIAN_POINT('Ctrl Pts',(-0.710978231689117,-1.,3.79093694007146));
#44931=CARTESIAN_POINT('Ctrl Pts',(-0.710978231689117,1.,3.79093694007146));
#44932=CARTESIAN_POINT('Ctrl Pts',(-0.7080158793756,-1.,3.78402183336678));
#44933=CARTESIAN_POINT('Ctrl Pts',(-0.7080158793756,1.,3.78402183336678));
#44934=CARTESIAN_POINT('Ctrl Pts',(-0.70513584799995,-1.,3.77719254217197));
#44935=CARTESIAN_POINT('Ctrl Pts',(-0.70513584799995,1.,3.77719254217197));
#44936=CARTESIAN_POINT('Ctrl Pts',(-0.702346356621613,-1.,3.77048141872904));
#44937=CARTESIAN_POINT('Ctrl Pts',(-0.702346356621613,1.,3.77048141872904));
#44938=CARTESIAN_POINT('Ctrl Pts',(-0.699648552230851,-1.,3.76387780603725));
#44939=CARTESIAN_POINT('Ctrl Pts',(-0.699648552230851,1.,3.76387780603725));
#44940=CARTESIAN_POINT('Ctrl Pts',(-0.69703124565953,-1.,3.75729775766913));
#44941=CARTESIAN_POINT('Ctrl Pts',(-0.69703124565953,1.,3.75729775766913));
#44942=CARTESIAN_POINT('Ctrl Pts',(-0.694474562581173,-1.,3.7506028824329));
#44943=CARTESIAN_POINT('Ctrl Pts',(-0.694474562581173,1.,3.7506028824329));
#44944=CARTESIAN_POINT('Ctrl Pts',(-0.691960080400503,-1.,3.74365508986548));
#44945=CARTESIAN_POINT('Ctrl Pts',(-0.691960080400503,1.,3.74365508986548));
#44946=CARTESIAN_POINT('Ctrl Pts',(-0.689479637354651,-1.,3.73636374474993));
#44947=CARTESIAN_POINT('Ctrl Pts',(-0.689479637354651,1.,3.73636374474993));
#44948=CARTESIAN_POINT('Ctrl Pts',(-0.687043475232499,-1.,3.72872973554125));
#44949=CARTESIAN_POINT('Ctrl Pts',(-0.687043475232499,1.,3.72872973554125));
#44950=CARTESIAN_POINT('Ctrl Pts',(-0.684691698168355,-1.,3.7209063713952));
#44951=CARTESIAN_POINT('Ctrl Pts',(-0.684691698168355,1.,3.7209063713952));
#44952=CARTESIAN_POINT('Ctrl Pts',(-0.682492345109689,-1.,3.71319182790334));
#44953=CARTESIAN_POINT('Ctrl Pts',(-0.682492345109689,1.,3.71319182790334));
#44954=CARTESIAN_POINT('Ctrl Pts',(-0.680526909711618,-1.,3.70595722032165));
#44955=CARTESIAN_POINT('Ctrl Pts',(-0.680526909711618,1.,3.70595722032165));
#44956=CARTESIAN_POINT('Ctrl Pts',(-0.67887882222639,-1.,3.69959004073192));
#44957=CARTESIAN_POINT('Ctrl Pts',(-0.67887882222639,1.,3.69959004073192));
#44958=CARTESIAN_POINT('Ctrl Pts',(-0.677621861865196,-1.,3.69443683573443));
#44959=CARTESIAN_POINT('Ctrl Pts',(-0.677621861865196,1.,3.69443683573443));
#44960=CARTESIAN_POINT('Ctrl Pts',(-0.676805811074141,-1.,3.69073278191505));
#44961=CARTESIAN_POINT('Ctrl Pts',(-0.676805811074141,1.,3.69073278191505));
#44962=CARTESIAN_POINT('Ctrl Pts',(-0.676524321060167,-1.,3.68901718135636));
#44963=CARTESIAN_POINT('Ctrl Pts',(-0.676524321060167,1.,3.68901718135636));
#44964=CARTESIAN_POINT('Ctrl Pts',(-0.676525601650139,-1.,3.68844918120934));
#44965=CARTESIAN_POINT('Ctrl Pts',(-0.676525601650139,1.,3.68844918120934));
#44966=CARTESIAN_POINT('Ctrl Pts',(-0.676620796001716,-1.,3.68838970675356));
#44967=CARTESIAN_POINT('Ctrl Pts',(-0.676620796001716,1.,3.68838970675356));
#44968=CARTESIAN_POINT('Ctrl Pts',(-0.676691979611562,-1.,3.68843977377012));
#44969=CARTESIAN_POINT('Ctrl Pts',(-0.676691979611562,1.,3.68843977377012));
#44970=CARTESIAN_POINT('',(-0.906349047628866,1.,4.10104028313088));
#44971=CARTESIAN_POINT('Ctrl Pts',(-0.906349047628866,1.,4.10104028313088));
#44972=CARTESIAN_POINT('Ctrl Pts',(-0.905360112216302,1.,4.09981755067956));
#44973=CARTESIAN_POINT('Ctrl Pts',(-0.903385402444213,1.,4.09737067247114));
#44974=CARTESIAN_POINT('Ctrl Pts',(-0.900432820945975,1.,4.09369611524319));
#44975=CARTESIAN_POINT('Ctrl Pts',(-0.896515019236368,1.,4.08878822249095));
#44976=CARTESIAN_POINT('Ctrl Pts',(-0.891649447920401,1.,4.08263920306651));
#44977=CARTESIAN_POINT('Ctrl Pts',(-0.886815658360739,1.,4.07647601774639));
#44978=CARTESIAN_POINT('Ctrl Pts',(-0.882013797525916,1.,4.07029866694292));
#44979=CARTESIAN_POINT('Ctrl Pts',(-0.877244060484595,1.,4.06410717232347));
#44980=CARTESIAN_POINT('Ctrl Pts',(-0.872506694780563,1.,4.05790159030495));
#44981=CARTESIAN_POINT('Ctrl Pts',(-0.867801988858176,1.,4.05168199437128));
#44982=CARTESIAN_POINT('Ctrl Pts',(-0.863130256642173,1.,4.04544845048097));
#44983=CARTESIAN_POINT('Ctrl Pts',(-0.858491822322571,1.,4.03920099284658));
#44984=CARTESIAN_POINT('Ctrl Pts',(-0.853887006632178,1.,4.03293960436945));
#44985=CARTESIAN_POINT('Ctrl Pts',(-0.849316107475012,1.,4.02666418343508));
#44986=CARTESIAN_POINT('Ctrl Pts',(-0.844779403288517,1.,4.02037456798787));
#44987=CARTESIAN_POINT('Ctrl Pts',(-0.84027717197638,1.,4.01407059766338));
#44988=CARTESIAN_POINT('Ctrl Pts',(-0.835809705809822,1.,4.00775216907934));
#44989=CARTESIAN_POINT('Ctrl Pts',(-0.831377325741487,1.,4.00141928477447));
#44990=CARTESIAN_POINT('Ctrl Pts',(-0.826980400320473,1.,3.99507212784289));
#44991=CARTESIAN_POINT('Ctrl Pts',(-0.822619346021769,1.,3.98871104646328));
#44992=CARTESIAN_POINT('Ctrl Pts',(-0.818294599022033,1.,3.98233640155287));
#44993=CARTESIAN_POINT('Ctrl Pts',(-0.814006592328737,1.,3.97594844078763));
#44994=CARTESIAN_POINT('Ctrl Pts',(-0.809755732818134,1.,3.96954717513251));
#44995=CARTESIAN_POINT('Ctrl Pts',(-0.805542372178496,1.,3.96313222295874));
#44996=CARTESIAN_POINT('Ctrl Pts',(-0.801366797727206,1.,3.95670276375176));
#44997=CARTESIAN_POINT('Ctrl Pts',(-0.797229296085438,1.,3.95025788827189));
#44998=CARTESIAN_POINT('Ctrl Pts',(-0.793130205641017,1.,3.94379688971307));
#44999=CARTESIAN_POINT('Ctrl Pts',(-0.789069971469323,1.,3.93731956885671));
#45000=CARTESIAN_POINT('Ctrl Pts',(-0.785049202786458,1.,3.93082655631768));
#45001=CARTESIAN_POINT('Ctrl Pts',(-0.781068718228395,1.,3.92431956510418));
#45002=CARTESIAN_POINT('Ctrl Pts',(-0.777129415664915,1.,3.91780062334464));
#45003=CARTESIAN_POINT('Ctrl Pts',(-0.773232154506305,1.,3.91127138115238));
#45004=CARTESIAN_POINT('Ctrl Pts',(-0.769377629847877,1.,3.90473237182634));
#45005=CARTESIAN_POINT('Ctrl Pts',(-0.765566256401306,1.,3.89818233104381));
#45006=CARTESIAN_POINT('Ctrl Pts',(-0.761798028793978,1.,3.89161738162245));
#45007=CARTESIAN_POINT('Ctrl Pts',(-0.758072800564799,1.,3.88503262662684));
#45008=CARTESIAN_POINT('Ctrl Pts',(-0.754390577396847,1.,3.87842382520058));
#45009=CARTESIAN_POINT('Ctrl Pts',(-0.750751822383024,1.,3.87178914078372));
#45010=CARTESIAN_POINT('Ctrl Pts',(-0.747157716488884,1.,3.86513062969896));
#45011=CARTESIAN_POINT('Ctrl Pts',(-0.743610542737042,1.,3.85845645217611));
#45012=CARTESIAN_POINT('Ctrl Pts',(-0.740113146827176,1.,3.85177770351237));
#45013=CARTESIAN_POINT('Ctrl Pts',(-0.736668240497151,1.,3.84510432881231));
#45014=CARTESIAN_POINT('Ctrl Pts',(-0.73327770375609,1.,3.83844103658016));
#45015=CARTESIAN_POINT('Ctrl Pts',(-0.729942010490146,1.,3.8317839240337));
#45016=CARTESIAN_POINT('Ctrl Pts',(-0.726659281876608,1.,3.82511495756682));
#45017=CARTESIAN_POINT('Ctrl Pts',(-0.723426346019349,1.,3.81840802610795));
#45018=CARTESIAN_POINT('Ctrl Pts',(-0.720240466589172,1.,3.81163885127309));
#45019=CARTESIAN_POINT('Ctrl Pts',(-0.717100993669091,1.,3.80479445759296));
#45020=CARTESIAN_POINT('Ctrl Pts',(-0.714010733006677,1.,3.79788100314994));
#45021=CARTESIAN_POINT('Ctrl Pts',(-0.710978231689117,1.,3.79093694007146));
#45022=CARTESIAN_POINT('Ctrl Pts',(-0.7080158793756,1.,3.78402183336678));
#45023=CARTESIAN_POINT('Ctrl Pts',(-0.70513584799995,1.,3.77719254217197));
#45024=CARTESIAN_POINT('Ctrl Pts',(-0.702346356621613,1.,3.77048141872904));
#45025=CARTESIAN_POINT('Ctrl Pts',(-0.699648552230851,1.,3.76387780603725));
#45026=CARTESIAN_POINT('Ctrl Pts',(-0.69703124565953,1.,3.75729775766913));
#45027=CARTESIAN_POINT('Ctrl Pts',(-0.694474562581173,1.,3.7506028824329));
#45028=CARTESIAN_POINT('Ctrl Pts',(-0.691960080400503,1.,3.74365508986548));
#45029=CARTESIAN_POINT('Ctrl Pts',(-0.689479637354651,1.,3.73636374474993));
#45030=CARTESIAN_POINT('Ctrl Pts',(-0.687043475232499,1.,3.72872973554125));
#45031=CARTESIAN_POINT('Ctrl Pts',(-0.684691698168355,1.,3.7209063713952));
#45032=CARTESIAN_POINT('Ctrl Pts',(-0.682492345109689,1.,3.71319182790334));
#45033=CARTESIAN_POINT('Ctrl Pts',(-0.680526909711618,1.,3.70595722032165));
#45034=CARTESIAN_POINT('Ctrl Pts',(-0.67887882222639,1.,3.69959004073192));
#45035=CARTESIAN_POINT('Ctrl Pts',(-0.677621861865196,1.,3.69443683573443));
#45036=CARTESIAN_POINT('Ctrl Pts',(-0.676867042599711,1.,3.6910107117555));
#45037=CARTESIAN_POINT('Ctrl Pts',(-0.676580391119535,1.,3.68934997767391));
#45038=CARTESIAN_POINT('Ctrl Pts',(-0.676535079520366,1.,3.68869596426099));
#45039=CARTESIAN_POINT('Ctrl Pts',(-0.67656928609342,1.,3.68850172300543));
#45040=CARTESIAN_POINT('Ctrl Pts',(-0.676591647973661,1.,3.68845817949618));
#45041=CARTESIAN_POINT('',(-0.906349047628866,0.,4.10104028313088));
#45042=CARTESIAN_POINT('Ctrl Pts',(-1.07157964745328,-1.,3.59363563249864));
#45043=CARTESIAN_POINT('Ctrl Pts',(-1.07157964745328,1.,3.59363563249864));
#45044=CARTESIAN_POINT('Ctrl Pts',(-1.07162034256459,-1.,3.59355870577901));
#45045=CARTESIAN_POINT('Ctrl Pts',(-1.07162034256459,1.,3.59355870577901));
#45046=CARTESIAN_POINT('Ctrl Pts',(-1.07173216219145,-1.,3.59356848057812));
#45047=CARTESIAN_POINT('Ctrl Pts',(-1.07173216219145,1.,3.59356848057812));
#45048=CARTESIAN_POINT('Ctrl Pts',(-1.07199116987656,-1.,3.5940739910409));
#45049=CARTESIAN_POINT('Ctrl Pts',(-1.07199116987656,1.,3.5940739910409));
#45050=CARTESIAN_POINT('Ctrl Pts',(-1.07251922679245,-1.,3.59573039612316));
#45051=CARTESIAN_POINT('Ctrl Pts',(-1.07251922679245,1.,3.59573039612316));
#45052=CARTESIAN_POINT('Ctrl Pts',(-1.07347372545714,-1.,3.59940121154535));
#45053=CARTESIAN_POINT('Ctrl Pts',(-1.07347372545714,1.,3.59940121154535));
#45054=CARTESIAN_POINT('Ctrl Pts',(-1.07469327168578,-1.,3.60456339887778));
#45055=CARTESIAN_POINT('Ctrl Pts',(-1.07469327168578,1.,3.60456339887778));
#45056=CARTESIAN_POINT('Ctrl Pts',(-1.07611545402734,-1.,3.61098481349204));
#45057=CARTESIAN_POINT('Ctrl Pts',(-1.07611545402734,1.,3.61098481349204));
#45058=CARTESIAN_POINT('Ctrl Pts',(-1.07764868137619,-1.,3.61832318504574));
#45059=CARTESIAN_POINT('Ctrl Pts',(-1.07764868137619,1.,3.61832318504574));
#45060=CARTESIAN_POINT('Ctrl Pts',(-1.07919137290742,-1.,3.62619537902361));
#45061=CARTESIAN_POINT('Ctrl Pts',(-1.07919137290742,1.,3.62619537902361));
#45062=CARTESIAN_POINT('Ctrl Pts',(-1.08064765719867,-1.,3.63423373196529));
#45063=CARTESIAN_POINT('Ctrl Pts',(-1.08064765719867,1.,3.63423373196529));
#45064=CARTESIAN_POINT('Ctrl Pts',(-1.08194278850996,-1.,3.64214167843677));
#45065=CARTESIAN_POINT('Ctrl Pts',(-1.08194278850996,1.,3.64214167843677));
#45066=CARTESIAN_POINT('Ctrl Pts',(-1.08304289898623,-1.,3.64976441208358));
#45067=CARTESIAN_POINT('Ctrl Pts',(-1.08304289898623,1.,3.64976441208358));
#45068=CARTESIAN_POINT('Ctrl Pts',(-1.08395671077807,-1.,3.65709649161166));
#45069=CARTESIAN_POINT('Ctrl Pts',(-1.08395671077807,1.,3.65709649161166));
#45070=CARTESIAN_POINT('Ctrl Pts',(-1.08471809922901,-1.,3.66422237895365));
#45071=CARTESIAN_POINT('Ctrl Pts',(-1.08471809922901,1.,3.66422237895365));
#45072=CARTESIAN_POINT('Ctrl Pts',(-1.0853733414449,-1.,3.67127347729666));
#45073=CARTESIAN_POINT('Ctrl Pts',(-1.0853733414449,1.,3.67127347729666));
#45074=CARTESIAN_POINT('Ctrl Pts',(-1.0859675575576,-1.,3.67838211685117));
#45075=CARTESIAN_POINT('Ctrl Pts',(-1.0859675575576,1.,3.67838211685117));
#45076=CARTESIAN_POINT('Ctrl Pts',(-1.0865288888259,-1.,3.68562817420797));
#45077=CARTESIAN_POINT('Ctrl Pts',(-1.0865288888259,1.,3.68562817420797));
#45078=CARTESIAN_POINT('Ctrl Pts',(-1.08706319540271,-1.,3.69302062410157));
#45079=CARTESIAN_POINT('Ctrl Pts',(-1.08706319540271,1.,3.69302062410157));
#45080=CARTESIAN_POINT('Ctrl Pts',(-1.08756311291309,-1.,3.70052690909833));
#45081=CARTESIAN_POINT('Ctrl Pts',(-1.08756311291309,1.,3.70052690909833));
#45082=CARTESIAN_POINT('Ctrl Pts',(-1.08801367312185,-1.,3.70809084139457));
#45083=CARTESIAN_POINT('Ctrl Pts',(-1.08801367312185,1.,3.70809084139457));
#45084=CARTESIAN_POINT('Ctrl Pts',(-1.0883988733478,-1.,3.71565372339075));
#45085=CARTESIAN_POINT('Ctrl Pts',(-1.0883988733478,1.,3.71565372339075));
#45086=CARTESIAN_POINT('Ctrl Pts',(-1.08870887220082,-1.,3.72317741369398));
#45087=CARTESIAN_POINT('Ctrl Pts',(-1.08870887220082,1.,3.72317741369398));
#45088=CARTESIAN_POINT('Ctrl Pts',(-1.08894337390937,-1.,3.73065515162988));
#45089=CARTESIAN_POINT('Ctrl Pts',(-1.08894337390937,1.,3.73065515162988));
#45090=CARTESIAN_POINT('Ctrl Pts',(-1.08910769013297,-1.,3.73809879348239));
#45091=CARTESIAN_POINT('Ctrl Pts',(-1.08910769013297,1.,3.73809879348239));
#45092=CARTESIAN_POINT('Ctrl Pts',(-1.08921040494017,-1.,3.74553121371757));
#45093=CARTESIAN_POINT('Ctrl Pts',(-1.08921040494017,1.,3.74553121371757));
#45094=CARTESIAN_POINT('Ctrl Pts',(-1.08926054632925,-1.,3.75297711748132));
#45095=CARTESIAN_POINT('Ctrl Pts',(-1.08926054632925,1.,3.75297711748132));
#45096=CARTESIAN_POINT('Ctrl Pts',(-1.08926462734282,-1.,3.76045342580208));
#45097=CARTESIAN_POINT('Ctrl Pts',(-1.08926462734282,1.,3.76045342580208));
#45098=CARTESIAN_POINT('Ctrl Pts',(-1.08922484204256,-1.,3.76796340094448));
#45099=CARTESIAN_POINT('Ctrl Pts',(-1.08922484204256,1.,3.76796340094448));
#45100=CARTESIAN_POINT('Ctrl Pts',(-1.0891407279127,-1.,3.77550199409424));
#45101=CARTESIAN_POINT('Ctrl Pts',(-1.0891407279127,1.,3.77550199409424));
#45102=CARTESIAN_POINT('Ctrl Pts',(-1.08901018614636,-1.,3.78305911299504));
#45103=CARTESIAN_POINT('Ctrl Pts',(-1.08901018614636,1.,3.78305911299504));
#45104=CARTESIAN_POINT('Ctrl Pts',(-1.08883071512098,-1.,3.79062357974404));
#45105=CARTESIAN_POINT('Ctrl Pts',(-1.08883071512098,1.,3.79062357974404));
#45106=CARTESIAN_POINT('Ctrl Pts',(-1.08860064435778,-1.,3.79818708705259));
#45107=CARTESIAN_POINT('Ctrl Pts',(-1.08860064435778,1.,3.79818708705259));
#45108=CARTESIAN_POINT('Ctrl Pts',(-1.0883200925538,-1.,3.8057472665766));
#45109=CARTESIAN_POINT('Ctrl Pts',(-1.0883200925538,1.,3.8057472665766));
#45110=CARTESIAN_POINT('Ctrl Pts',(-1.08799030610862,-1.,3.81330554446323));
#45111=CARTESIAN_POINT('Ctrl Pts',(-1.08799030610862,1.,3.81330554446323));
#45112=CARTESIAN_POINT('Ctrl Pts',(-1.08761321539442,-1.,3.82086569676319));
#45113=CARTESIAN_POINT('Ctrl Pts',(-1.08761321539442,1.,3.82086569676319));
#45114=CARTESIAN_POINT('Ctrl Pts',(-1.08719091307558,-1.,3.82843215316984));
#45115=CARTESIAN_POINT('Ctrl Pts',(-1.08719091307558,1.,3.82843215316984));
#45116=CARTESIAN_POINT('Ctrl Pts',(-1.08672515456902,-1.,3.83600837071708));
#45117=CARTESIAN_POINT('Ctrl Pts',(-1.08672515456902,1.,3.83600837071708));
#45118=CARTESIAN_POINT('Ctrl Pts',(-1.08621688337604,-1.,3.8435952876495));
#45119=CARTESIAN_POINT('Ctrl Pts',(-1.08621688337604,1.,3.8435952876495));
#45120=CARTESIAN_POINT('Ctrl Pts',(-1.08566647671844,-1.,3.85119211322755));
#45121=CARTESIAN_POINT('Ctrl Pts',(-1.08566647671844,1.,3.85119211322755));
#45122=CARTESIAN_POINT('Ctrl Pts',(-1.08507395120059,-1.,3.85879698702532));
#45123=CARTESIAN_POINT('Ctrl Pts',(-1.08507395120059,1.,3.85879698702532));
#45124=CARTESIAN_POINT('Ctrl Pts',(-1.08443918607927,-1.,3.86640769434274));
#45125=CARTESIAN_POINT('Ctrl Pts',(-1.08443918607927,1.,3.86640769434274));
#45126=CARTESIAN_POINT('Ctrl Pts',(-1.08376213307504,-1.,3.8740223372254));
#45127=CARTESIAN_POINT('Ctrl Pts',(-1.08376213307504,1.,3.8740223372254));
#45128=CARTESIAN_POINT('Ctrl Pts',(-1.08304304871028,-1.,3.88164007721312));
#45129=CARTESIAN_POINT('Ctrl Pts',(-1.08304304871028,1.,3.88164007721312));
#45130=CARTESIAN_POINT('Ctrl Pts',(-1.08228241999346,-1.,3.88926088975114));
#45131=CARTESIAN_POINT('Ctrl Pts',(-1.08228241999346,1.,3.88926088975114));
#45132=CARTESIAN_POINT('Ctrl Pts',(-1.08148086931358,-1.,3.8968852509835));
#45133=CARTESIAN_POINT('Ctrl Pts',(-1.08148086931358,1.,3.8968852509835));
#45134=CARTESIAN_POINT('Ctrl Pts',(-1.08063906483818,-1.,3.90451384092545));
#45135=CARTESIAN_POINT('Ctrl Pts',(-1.08063906483818,1.,3.90451384092545));
#45136=CARTESIAN_POINT('Ctrl Pts',(-1.07975763507473,-1.,3.91214726022143));
#45137=CARTESIAN_POINT('Ctrl Pts',(-1.07975763507473,1.,3.91214726022143));
#45138=CARTESIAN_POINT('Ctrl Pts',(-1.07883706663554,-1.,3.91978568924178));
#45139=CARTESIAN_POINT('Ctrl Pts',(-1.07883706663554,1.,3.91978568924178));
#45140=CARTESIAN_POINT('Ctrl Pts',(-1.07787771707195,-1.,3.9274289334984));
#45141=CARTESIAN_POINT('Ctrl Pts',(-1.07787771707195,1.,3.9274289334984));
#45142=CARTESIAN_POINT('Ctrl Pts',(-1.07687985975384,-1.,3.93507657572883));
#45143=CARTESIAN_POINT('Ctrl Pts',(-1.07687985975384,1.,3.93507657572883));
#45144=CARTESIAN_POINT('Ctrl Pts',(-1.07584371946443,-1.,3.94272809633331));
#45145=CARTESIAN_POINT('Ctrl Pts',(-1.07584371946443,1.,3.94272809633331));
#45146=CARTESIAN_POINT('Ctrl Pts',(-1.07476950921587,-1.,3.95038299600676));
#45147=CARTESIAN_POINT('Ctrl Pts',(-1.07476950921587,1.,3.95038299600676));
#45148=CARTESIAN_POINT('Ctrl Pts',(-1.07365747426491,-1.,3.95804094429373));
#45149=CARTESIAN_POINT('Ctrl Pts',(-1.07365747426491,1.,3.95804094429373));
#45150=CARTESIAN_POINT('Ctrl Pts',(-1.07250789943007,-1.,3.96570179322338));
#45151=CARTESIAN_POINT('Ctrl Pts',(-1.07250789943007,1.,3.96570179322338));
#45152=CARTESIAN_POINT('Ctrl Pts',(-1.07132109206164,-1.,3.9733655022223));
#45153=CARTESIAN_POINT('Ctrl Pts',(-1.07132109206164,1.,3.9733655022223));
#45154=CARTESIAN_POINT('Ctrl Pts',(-1.07009737257767,-1.,3.98103208801101));
#45155=CARTESIAN_POINT('Ctrl Pts',(-1.07009737257767,1.,3.98103208801101));
#45156=CARTESIAN_POINT('Ctrl Pts',(-1.06883706263942,-1.,3.98870156857412));
#45157=CARTESIAN_POINT('Ctrl Pts',(-1.06883706263942,1.,3.98870156857412));
#45158=CARTESIAN_POINT('Ctrl Pts',(-1.06754047381312,-1.,3.99637389920441));
#45159=CARTESIAN_POINT('Ctrl Pts',(-1.06754047381312,1.,3.99637389920441));
#45160=CARTESIAN_POINT('Ctrl Pts',(-1.06620789963606,-1.,4.00404894952579));
#45161=CARTESIAN_POINT('Ctrl Pts',(-1.06620789963606,1.,4.00404894952579));
#45162=CARTESIAN_POINT('Ctrl Pts',(-1.06483961343109,-1.,4.01172654187398));
#45163=CARTESIAN_POINT('Ctrl Pts',(-1.06483961343109,1.,4.01172654187398));
#45164=CARTESIAN_POINT('Ctrl Pts',(-1.06343586496236,-1.,4.01940647495943));
#45165=CARTESIAN_POINT('Ctrl Pts',(-1.06343586496236,1.,4.01940647495943));
#45166=CARTESIAN_POINT('Ctrl Pts',(-1.06199687787462,-1.,4.02708855235633));
#45167=CARTESIAN_POINT('Ctrl Pts',(-1.06199687787462,1.,4.02708855235633));
#45168=CARTESIAN_POINT('Ctrl Pts',(-1.06052284711857,-1.,4.03477261141553));
#45169=CARTESIAN_POINT('Ctrl Pts',(-1.06052284711857,1.,4.03477261141553));
#45170=CARTESIAN_POINT('Ctrl Pts',(-1.05901393666566,-1.,4.04245854427496));
#45171=CARTESIAN_POINT('Ctrl Pts',(-1.05901393666566,1.,4.04245854427496));
#45172=CARTESIAN_POINT('Ctrl Pts',(-1.05747027727959,-1.,4.05014628384869));
#45173=CARTESIAN_POINT('Ctrl Pts',(-1.05747027727959,1.,4.05014628384869));
#45174=CARTESIAN_POINT('Ctrl Pts',(-1.05620762707996,-1.,4.05629789307025));
#45175=CARTESIAN_POINT('Ctrl Pts',(-1.05620762707996,1.,4.05629789307025));
#45176=CARTESIAN_POINT('Ctrl Pts',(-1.055245071776,-1.,4.06091239149123));
#45177=CARTESIAN_POINT('Ctrl Pts',(-1.055245071776,1.,4.06091239149123));
#45178=CARTESIAN_POINT('Ctrl Pts',(-1.05459645194823,-1.,4.06398907542249));
#45179=CARTESIAN_POINT('Ctrl Pts',(-1.05459645194823,1.,4.06398907542249));
#45180=CARTESIAN_POINT('Ctrl Pts',(-1.05427041296137,-1.,4.06552750530042));
#45181=CARTESIAN_POINT('Ctrl Pts',(-1.05427041296137,1.,4.06552750530042));
#45182=CARTESIAN_POINT('',(-1.07167739962028,1.,3.59360648251073));
#45183=CARTESIAN_POINT('Ctrl Pts',(-1.07167739962028,-1.,3.59360648251073));
#45184=CARTESIAN_POINT('Ctrl Pts',(-1.07167739962028,-0.666666666666667,
3.59360648251073));
#45185=CARTESIAN_POINT('Ctrl Pts',(-1.07167739962028,-0.333333333333333,
3.59360648251073));
#45186=CARTESIAN_POINT('Ctrl Pts',(-1.07167739962028,0.333333333333333,
3.59360648251073));
#45187=CARTESIAN_POINT('Ctrl Pts',(-1.07167739962028,0.666666666666667,
3.59360648251073));
#45188=CARTESIAN_POINT('Ctrl Pts',(-1.07167739962028,1.,3.59360648251073));
#45189=CARTESIAN_POINT('',(-1.05427041296137,1.,4.06552750530042));
#45190=CARTESIAN_POINT('',(-1.05427041296137,0.,4.06552750530042));
#45191=CARTESIAN_POINT('Ctrl Pts',(-1.07167739962028,1.,3.59360648251073));
#45192=CARTESIAN_POINT('Ctrl Pts',(-1.07171709254135,1.,3.5936351279798));
#45193=CARTESIAN_POINT('Ctrl Pts',(-1.07183575450617,1.,3.59379266874567));
#45194=CARTESIAN_POINT('Ctrl Pts',(-1.07209229745229,1.,3.59439596999862));
#45195=CARTESIAN_POINT('Ctrl Pts',(-1.07259084660936,1.,3.59600583194946));
#45196=CARTESIAN_POINT('Ctrl Pts',(-1.07347372545714,1.,3.59940121154535));
#45197=CARTESIAN_POINT('Ctrl Pts',(-1.07469327168578,1.,3.60456339887778));
#45198=CARTESIAN_POINT('Ctrl Pts',(-1.07611545402734,1.,3.61098481349204));
#45199=CARTESIAN_POINT('Ctrl Pts',(-1.07764868137619,1.,3.61832318504574));
#45200=CARTESIAN_POINT('Ctrl Pts',(-1.07919137290742,1.,3.62619537902361));
#45201=CARTESIAN_POINT('Ctrl Pts',(-1.08064765719867,1.,3.63423373196529));
#45202=CARTESIAN_POINT('Ctrl Pts',(-1.08194278850996,1.,3.64214167843677));
#45203=CARTESIAN_POINT('Ctrl Pts',(-1.08304289898623,1.,3.64976441208358));
#45204=CARTESIAN_POINT('Ctrl Pts',(-1.08395671077807,1.,3.65709649161166));
#45205=CARTESIAN_POINT('Ctrl Pts',(-1.08471809922901,1.,3.66422237895365));
#45206=CARTESIAN_POINT('Ctrl Pts',(-1.0853733414449,1.,3.67127347729666));
#45207=CARTESIAN_POINT('Ctrl Pts',(-1.0859675575576,1.,3.67838211685117));
#45208=CARTESIAN_POINT('Ctrl Pts',(-1.0865288888259,1.,3.68562817420797));
#45209=CARTESIAN_POINT('Ctrl Pts',(-1.08706319540271,1.,3.69302062410157));
#45210=CARTESIAN_POINT('Ctrl Pts',(-1.08756311291309,1.,3.70052690909833));
#45211=CARTESIAN_POINT('Ctrl Pts',(-1.08801367312185,1.,3.70809084139457));
#45212=CARTESIAN_POINT('Ctrl Pts',(-1.0883988733478,1.,3.71565372339075));
#45213=CARTESIAN_POINT('Ctrl Pts',(-1.08870887220082,1.,3.72317741369398));
#45214=CARTESIAN_POINT('Ctrl Pts',(-1.08894337390937,1.,3.73065515162988));
#45215=CARTESIAN_POINT('Ctrl Pts',(-1.08910769013297,1.,3.73809879348239));
#45216=CARTESIAN_POINT('Ctrl Pts',(-1.08921040494017,1.,3.74553121371757));
#45217=CARTESIAN_POINT('Ctrl Pts',(-1.08926054632925,1.,3.75297711748132));
#45218=CARTESIAN_POINT('Ctrl Pts',(-1.08926462734282,1.,3.76045342580208));
#45219=CARTESIAN_POINT('Ctrl Pts',(-1.08922484204256,1.,3.76796340094448));
#45220=CARTESIAN_POINT('Ctrl Pts',(-1.0891407279127,1.,3.77550199409424));
#45221=CARTESIAN_POINT('Ctrl Pts',(-1.08901018614636,1.,3.78305911299504));
#45222=CARTESIAN_POINT('Ctrl Pts',(-1.08883071512098,1.,3.79062357974404));
#45223=CARTESIAN_POINT('Ctrl Pts',(-1.08860064435778,1.,3.79818708705259));
#45224=CARTESIAN_POINT('Ctrl Pts',(-1.0883200925538,1.,3.8057472665766));
#45225=CARTESIAN_POINT('Ctrl Pts',(-1.08799030610862,1.,3.81330554446323));
#45226=CARTESIAN_POINT('Ctrl Pts',(-1.08761321539442,1.,3.82086569676319));
#45227=CARTESIAN_POINT('Ctrl Pts',(-1.08719091307558,1.,3.82843215316984));
#45228=CARTESIAN_POINT('Ctrl Pts',(-1.08672515456902,1.,3.83600837071708));
#45229=CARTESIAN_POINT('Ctrl Pts',(-1.08621688337604,1.,3.8435952876495));
#45230=CARTESIAN_POINT('Ctrl Pts',(-1.08566647671844,1.,3.85119211322755));
#45231=CARTESIAN_POINT('Ctrl Pts',(-1.08507395120059,1.,3.85879698702532));
#45232=CARTESIAN_POINT('Ctrl Pts',(-1.08443918607927,1.,3.86640769434274));
#45233=CARTESIAN_POINT('Ctrl Pts',(-1.08376213307504,1.,3.8740223372254));
#45234=CARTESIAN_POINT('Ctrl Pts',(-1.08304304871028,1.,3.88164007721312));
#45235=CARTESIAN_POINT('Ctrl Pts',(-1.08228241999346,1.,3.88926088975114));
#45236=CARTESIAN_POINT('Ctrl Pts',(-1.08148086931358,1.,3.8968852509835));
#45237=CARTESIAN_POINT('Ctrl Pts',(-1.08063906483818,1.,3.90451384092545));
#45238=CARTESIAN_POINT('Ctrl Pts',(-1.07975763507473,1.,3.91214726022143));
#45239=CARTESIAN_POINT('Ctrl Pts',(-1.07883706663554,1.,3.91978568924178));
#45240=CARTESIAN_POINT('Ctrl Pts',(-1.07787771707195,1.,3.9274289334984));
#45241=CARTESIAN_POINT('Ctrl Pts',(-1.07687985975384,1.,3.93507657572883));
#45242=CARTESIAN_POINT('Ctrl Pts',(-1.07584371946443,1.,3.94272809633331));
#45243=CARTESIAN_POINT('Ctrl Pts',(-1.07476950921587,1.,3.95038299600676));
#45244=CARTESIAN_POINT('Ctrl Pts',(-1.07365747426491,1.,3.95804094429373));
#45245=CARTESIAN_POINT('Ctrl Pts',(-1.07250789943007,1.,3.96570179322338));
#45246=CARTESIAN_POINT('Ctrl Pts',(-1.07132109206164,1.,3.9733655022223));
#45247=CARTESIAN_POINT('Ctrl Pts',(-1.07009737257767,1.,3.98103208801101));
#45248=CARTESIAN_POINT('Ctrl Pts',(-1.06883706263942,1.,3.98870156857412));
#45249=CARTESIAN_POINT('Ctrl Pts',(-1.06754047381312,1.,3.99637389920441));
#45250=CARTESIAN_POINT('Ctrl Pts',(-1.06620789963606,1.,4.00404894952579));
#45251=CARTESIAN_POINT('Ctrl Pts',(-1.06483961343109,1.,4.01172654187398));
#45252=CARTESIAN_POINT('Ctrl Pts',(-1.06343586496236,1.,4.01940647495943));
#45253=CARTESIAN_POINT('Ctrl Pts',(-1.06199687787462,1.,4.02708855235633));
#45254=CARTESIAN_POINT('Ctrl Pts',(-1.06052284711857,1.,4.03477261141553));
#45255=CARTESIAN_POINT('Ctrl Pts',(-1.05901393666566,1.,4.04245854427496));
#45256=CARTESIAN_POINT('Ctrl Pts',(-1.05747027727959,1.,4.05014628384869));
#45257=CARTESIAN_POINT('Ctrl Pts',(-1.05620762707996,1.,4.05629789307025));
#45258=CARTESIAN_POINT('Ctrl Pts',(-1.055245071776,1.,4.06091239149123));
#45259=CARTESIAN_POINT('Ctrl Pts',(-1.05459645194823,1.,4.06398907542249));
#45260=CARTESIAN_POINT('Ctrl Pts',(-1.05427041296137,1.,4.06552750530042));
#45261=CARTESIAN_POINT('Origin',(-1.05427041296137,0.,4.06552750530042));
#45262=CARTESIAN_POINT('',(-0.906349047628866,1.,4.10104028313088));
#45263=CARTESIAN_POINT('Origin',(0.,0.,0.));
#45264=CARTESIAN_POINT('',(-1.24526366418038,1.,3.5372048861597));
#45265=CARTESIAN_POINT('Origin',(0.,1.,0.));
#45266=CARTESIAN_POINT('Ctrl Pts',(-1.24526366418038,1.,3.5372048861597));
#45267=CARTESIAN_POINT('Ctrl Pts',(-1.24526366418038,0.666666666666667,
3.5372048861597));
#45268=CARTESIAN_POINT('Ctrl Pts',(-1.24526366418038,0.333333333333333,
3.5372048861597));
#45269=CARTESIAN_POINT('Ctrl Pts',(-1.24526366418038,-0.333333333333333,
3.5372048861597));
#45270=CARTESIAN_POINT('Ctrl Pts',(-1.24526366418038,-0.666666666666667,
3.5372048861597));
#45271=CARTESIAN_POINT('Ctrl Pts',(-1.24526366418038,-1.,3.5372048861597));
#45272=CARTESIAN_POINT('Ctrl Pts',(-1.53673442965256,-1.,3.90876544355381));
#45273=CARTESIAN_POINT('Ctrl Pts',(-1.53673442965256,1.,3.90876544355381));
#45274=CARTESIAN_POINT('Ctrl Pts',(-1.53556639217905,-1.,3.90771246855019));
#45275=CARTESIAN_POINT('Ctrl Pts',(-1.53556639217905,1.,3.90771246855019));
#45276=CARTESIAN_POINT('Ctrl Pts',(-1.53323321827755,-1.,3.90560462813969));
#45277=CARTESIAN_POINT('Ctrl Pts',(-1.53323321827755,1.,3.90560462813969));
#45278=CARTESIAN_POINT('Ctrl Pts',(-1.52974216056287,-1.,3.90243719631596));
#45279=CARTESIAN_POINT('Ctrl Pts',(-1.52974216056287,1.,3.90243719631596));
#45280=CARTESIAN_POINT('Ctrl Pts',(-1.52510482991635,-1.,3.89820260708225));
#45281=CARTESIAN_POINT('Ctrl Pts',(-1.52510482991635,1.,3.89820260708225));
#45282=CARTESIAN_POINT('Ctrl Pts',(-1.51933724329306,-1.,3.89289043533657));
#45283=CARTESIAN_POINT('Ctrl Pts',(-1.51933724329306,1.,3.89289043533657));
#45284=CARTESIAN_POINT('Ctrl Pts',(-1.51359883110559,-1.,3.88755930033884));
#45285=CARTESIAN_POINT('Ctrl Pts',(-1.51359883110559,1.,3.88755930033884));
#45286=CARTESIAN_POINT('Ctrl Pts',(-1.50788973857757,-1.,3.88220917950538));
#45287=CARTESIAN_POINT('Ctrl Pts',(-1.50788973857757,1.,3.88220917950538));
#45288=CARTESIAN_POINT('Ctrl Pts',(-1.50221016176556,-1.,3.87684006372134));
#45289=CARTESIAN_POINT('Ctrl Pts',(-1.50221016176556,1.,3.87684006372134));
#45290=CARTESIAN_POINT('Ctrl Pts',(-1.49656035399122,-1.,3.87145196998465));
#45291=CARTESIAN_POINT('Ctrl Pts',(-1.49656035399122,1.,3.87145196998465));
#45292=CARTESIAN_POINT('Ctrl Pts',(-1.4909406116431,-1.,3.86604492575189));
#45293=CARTESIAN_POINT('Ctrl Pts',(-1.4909406116431,1.,3.86604492575189));
#45294=CARTESIAN_POINT('Ctrl Pts',(-1.48535125509919,-1.,3.86061894706087));
#45295=CARTESIAN_POINT('Ctrl Pts',(-1.48535125509919,1.,3.86061894706087));
#45296=CARTESIAN_POINT('Ctrl Pts',(-1.4797926099102,-1.,3.85517401698843));
#45297=CARTESIAN_POINT('Ctrl Pts',(-1.4797926099102,1.,3.85517401698843));
#45298=CARTESIAN_POINT('Ctrl Pts',(-1.47426499018538,-1.,3.84971006847277));
#45299=CARTESIAN_POINT('Ctrl Pts',(-1.47426499018538,1.,3.84971006847277));
#45300=CARTESIAN_POINT('Ctrl Pts',(-1.46876867426504,-1.,3.84422695454796));
#45301=CARTESIAN_POINT('Ctrl Pts',(-1.46876867426504,1.,3.84422695454796));
#45302=CARTESIAN_POINT('Ctrl Pts',(-1.46330391180752,-1.,3.83872447159639));
#45303=CARTESIAN_POINT('Ctrl Pts',(-1.46330391180752,1.,3.83872447159639));
#45304=CARTESIAN_POINT('Ctrl Pts',(-1.45787095220852,-1.,3.83320241775423));
#45305=CARTESIAN_POINT('Ctrl Pts',(-1.45787095220852,1.,3.83320241775423));
#45306=CARTESIAN_POINT('Ctrl Pts',(-1.45247006796836,-1.,3.82766064519074));
#45307=CARTESIAN_POINT('Ctrl Pts',(-1.45247006796836,1.,3.82766064519074));
#45308=CARTESIAN_POINT('Ctrl Pts',(-1.44710157648539,-1.,3.82209910620533));
#45309=CARTESIAN_POINT('Ctrl Pts',(-1.44710157648539,1.,3.82209910620533));
#45310=CARTESIAN_POINT('Ctrl Pts',(-1.44176587041347,-1.,3.81651792398414));
#45311=CARTESIAN_POINT('Ctrl Pts',(-1.44176587041347,1.,3.81651792398414));
#45312=CARTESIAN_POINT('Ctrl Pts',(-1.43646341556724,-1.,3.81091737726815));
#45313=CARTESIAN_POINT('Ctrl Pts',(-1.43646341556724,1.,3.81091737726815));
#45314=CARTESIAN_POINT('Ctrl Pts',(-1.4311946992132,-1.,3.80529775429805));
#45315=CARTESIAN_POINT('Ctrl Pts',(-1.4311946992132,1.,3.80529775429805));
#45316=CARTESIAN_POINT('Ctrl Pts',(-1.42596018777283,-1.,3.7996592319632));
#45317=CARTESIAN_POINT('Ctrl Pts',(-1.42596018777283,1.,3.7996592319632));
#45318=CARTESIAN_POINT('Ctrl Pts',(-1.42076028482836,-1.,3.79400175744408));
#45319=CARTESIAN_POINT('Ctrl Pts',(-1.42076028482836,1.,3.79400175744408));
#45320=CARTESIAN_POINT('Ctrl Pts',(-1.4155952780383,-1.,3.78832489879426));
#45321=CARTESIAN_POINT('Ctrl Pts',(-1.4155952780383,1.,3.78832489879426));
#45322=CARTESIAN_POINT('Ctrl Pts',(-1.41046532282593,-1.,3.78262780065471));
#45323=CARTESIAN_POINT('Ctrl Pts',(-1.41046532282593,1.,3.78262780065471));
#45324=CARTESIAN_POINT('Ctrl Pts',(-1.40537056004722,-1.,3.77690952014259));
#45325=CARTESIAN_POINT('Ctrl Pts',(-1.40537056004722,1.,3.77690952014259));
#45326=CARTESIAN_POINT('Ctrl Pts',(-1.40031121335505,-1.,3.77116930621827));
#45327=CARTESIAN_POINT('Ctrl Pts',(-1.40031121335505,1.,3.77116930621827));
#45328=CARTESIAN_POINT('Ctrl Pts',(-1.39528769118052,-1.,3.76540689249074));
#45329=CARTESIAN_POINT('Ctrl Pts',(-1.39528769118052,1.,3.76540689249074));
#45330=CARTESIAN_POINT('Ctrl Pts',(-1.39030069388918,-1.,3.75962280650855));
#45331=CARTESIAN_POINT('Ctrl Pts',(-1.39030069388918,1.,3.75962280650855));
#45332=CARTESIAN_POINT('Ctrl Pts',(-1.38535129801176,-1.,3.75381861212707));
#45333=CARTESIAN_POINT('Ctrl Pts',(-1.38535129801176,1.,3.75381861212707));
#45334=CARTESIAN_POINT('Ctrl Pts',(-1.38044070763295,-1.,3.74799617204729));
#45335=CARTESIAN_POINT('Ctrl Pts',(-1.38044070763295,1.,3.74799617204729));
#45336=CARTESIAN_POINT('Ctrl Pts',(-1.37557002971687,-1.,3.74215698162555));
#45337=CARTESIAN_POINT('Ctrl Pts',(-1.37557002971687,1.,3.74215698162555));
#45338=CARTESIAN_POINT('Ctrl Pts',(-1.37074003422739,-1.,3.7363014588581));
#45339=CARTESIAN_POINT('Ctrl Pts',(-1.37074003422739,1.,3.7363014588581));
#45340=CARTESIAN_POINT('Ctrl Pts',(-1.36595093298676,-1.,3.73042829011295));
#45341=CARTESIAN_POINT('Ctrl Pts',(-1.36595093298676,1.,3.73042829011295));
#45342=CARTESIAN_POINT('Ctrl Pts',(-1.36120211416354,-1.,3.72453364678279));
#45343=CARTESIAN_POINT('Ctrl Pts',(-1.36120211416354,1.,3.72453364678279));
#45344=CARTESIAN_POINT('Ctrl Pts',(-1.35649266705037,-1.,3.71861271513313));
#45345=CARTESIAN_POINT('Ctrl Pts',(-1.35649266705037,1.,3.71861271513313));
#45346=CARTESIAN_POINT('Ctrl Pts',(-1.35182193384424,-1.,3.71266130563054));
#45347=CARTESIAN_POINT('Ctrl Pts',(-1.35182193384424,1.,3.71266130563054));
#45348=CARTESIAN_POINT('Ctrl Pts',(-1.34719008463534,-1.,3.70667753188248));
#45349=CARTESIAN_POINT('Ctrl Pts',(-1.34719008463534,1.,3.70667753188248));
#45350=CARTESIAN_POINT('Ctrl Pts',(-1.34259860752933,-1.,3.70066324015119));
#45351=CARTESIAN_POINT('Ctrl Pts',(-1.34259860752933,1.,3.70066324015119));
#45352=CARTESIAN_POINT('Ctrl Pts',(-1.3380510339822,-1.,3.69462613305708));
#45353=CARTESIAN_POINT('Ctrl Pts',(-1.3380510339822,1.,3.69462613305708));
#45354=CARTESIAN_POINT('Ctrl Pts',(-1.33355191034523,-1.,3.68857672413033));
#45355=CARTESIAN_POINT('Ctrl Pts',(-1.33355191034523,1.,3.68857672413033));
#45356=CARTESIAN_POINT('Ctrl Pts',(-1.3291054707274,-1.,3.68252441182551));
#45357=CARTESIAN_POINT('Ctrl Pts',(-1.3291054707274,1.,3.68252441182551));
#45358=CARTESIAN_POINT('Ctrl Pts',(-1.32471430856415,-1.,3.67647355257912));
#45359=CARTESIAN_POINT('Ctrl Pts',(-1.32471430856415,1.,3.67647355257912));
#45360=CARTESIAN_POINT('Ctrl Pts',(-1.32037828137766,-1.,3.67042021752656));
#45361=CARTESIAN_POINT('Ctrl Pts',(-1.32037828137766,1.,3.67042021752656));
#45362=CARTESIAN_POINT('Ctrl Pts',(-1.31609271239911,-1.,3.66434688899793));
#45363=CARTESIAN_POINT('Ctrl Pts',(-1.31609271239911,1.,3.66434688899793));
#45364=CARTESIAN_POINT('Ctrl Pts',(-1.31185038411218,-1.,3.65822827358617));
#45365=CARTESIAN_POINT('Ctrl Pts',(-1.31185038411218,1.,3.65822827358617));
#45366=CARTESIAN_POINT('Ctrl Pts',(-1.30764479590039,-1.,3.65204081987068));
#45367=CARTESIAN_POINT('Ctrl Pts',(-1.30764479590039,1.,3.65204081987068));
#45368=CARTESIAN_POINT('Ctrl Pts',(-1.30347327603774,-1.,3.64577181380113));
#45369=CARTESIAN_POINT('Ctrl Pts',(-1.30347327603774,1.,3.64577181380113));
#45370=CARTESIAN_POINT('Ctrl Pts',(-1.2993395590647,-1.,3.63942689872808));
#45371=CARTESIAN_POINT('Ctrl Pts',(-1.2993395590647,1.,3.63942689872808));
#45372=CARTESIAN_POINT('Ctrl Pts',(-1.29525810207762,-1.,3.63304271631046));
#45373=CARTESIAN_POINT('Ctrl Pts',(-1.29525810207762,1.,3.63304271631046));
#45374=CARTESIAN_POINT('Ctrl Pts',(-1.29125046021878,-1.,3.62667616004369));
#45375=CARTESIAN_POINT('Ctrl Pts',(-1.29125046021878,1.,3.62667616004369));
#45376=CARTESIAN_POINT('Ctrl Pts',(-1.28733755029384,-1.,3.6203814849236));
#45377=CARTESIAN_POINT('Ctrl Pts',(-1.28733755029384,1.,3.6203814849236));
#45378=CARTESIAN_POINT('Ctrl Pts',(-1.28353255117765,-1.,3.61418935913823));
#45379=CARTESIAN_POINT('Ctrl Pts',(-1.28353255117765,1.,3.61418935913823));
#45380=CARTESIAN_POINT('Ctrl Pts',(-1.27983492861691,-1.,3.60808907746339));
#45381=CARTESIAN_POINT('Ctrl Pts',(-1.27983492861691,1.,3.60808907746339));
#45382=CARTESIAN_POINT('Ctrl Pts',(-1.27622049908625,-1.,3.60199947736298));
#45383=CARTESIAN_POINT('Ctrl Pts',(-1.27622049908625,1.,3.60199947736298));
#45384=CARTESIAN_POINT('Ctrl Pts',(-1.27264798379307,-1.,3.59578698050006));
#45385=CARTESIAN_POINT('Ctrl Pts',(-1.27264798379307,1.,3.59578698050006));
#45386=CARTESIAN_POINT('Ctrl Pts',(-1.26907758484709,-1.,3.58931807846313));
#45387=CARTESIAN_POINT('Ctrl Pts',(-1.26907758484709,1.,3.58931807846313));
#45388=CARTESIAN_POINT('Ctrl Pts',(-1.26548706249862,-1.,3.58250452868618));
#45389=CARTESIAN_POINT('Ctrl Pts',(-1.26548706249862,1.,3.58250452868618));
#45390=CARTESIAN_POINT('Ctrl Pts',(-1.2618866714281,-1.,3.5753456065171));
#45391=CARTESIAN_POINT('Ctrl Pts',(-1.2618866714281,1.,3.5753456065171));
#45392=CARTESIAN_POINT('Ctrl Pts',(-1.25834000485716,-1.,3.56798645995275));
#45393=CARTESIAN_POINT('Ctrl Pts',(-1.25834000485716,1.,3.56798645995275));
#45394=CARTESIAN_POINT('Ctrl Pts',(-1.25496090900009,-1.,3.56071094991199));
#45395=CARTESIAN_POINT('Ctrl Pts',(-1.25496090900009,1.,3.56071094991199));
#45396=CARTESIAN_POINT('Ctrl Pts',(-1.2518879294064,-1.,3.55387287418985));
#45397=CARTESIAN_POINT('Ctrl Pts',(-1.2518879294064,1.,3.55387287418985));
#45398=CARTESIAN_POINT('Ctrl Pts',(-1.24926408628003,-1.,3.54784190283068));
#45399=CARTESIAN_POINT('Ctrl Pts',(-1.24926408628003,1.,3.54784190283068));
#45400=CARTESIAN_POINT('Ctrl Pts',(-1.24721646231966,-1.,3.54294877425964));
#45401=CARTESIAN_POINT('Ctrl Pts',(-1.24721646231966,1.,3.54294877425964));
#45402=CARTESIAN_POINT('Ctrl Pts',(-1.24583101679029,-1.,3.53941798195825));
#45403=CARTESIAN_POINT('Ctrl Pts',(-1.24583101679029,1.,3.53941798195825));
#45404=CARTESIAN_POINT('Ctrl Pts',(-1.24528461332987,-1.,3.53776753802906));
#45405=CARTESIAN_POINT('Ctrl Pts',(-1.24528461332987,1.,3.53776753802906));
#45406=CARTESIAN_POINT('Ctrl Pts',(-1.24519702335451,-1.,3.53720633057798));
#45407=CARTESIAN_POINT('Ctrl Pts',(-1.24519702335451,1.,3.53720633057798));
#45408=CARTESIAN_POINT('Ctrl Pts',(-1.24528174185098,-1.,3.53713269667399));
#45409=CARTESIAN_POINT('Ctrl Pts',(-1.24528174185098,1.,3.53713269667399));
#45410=CARTESIAN_POINT('Ctrl Pts',(-1.24535988127942,-1.,3.53717101171257));
#45411=CARTESIAN_POINT('Ctrl Pts',(-1.24535988127942,1.,3.53717101171257));
#45412=CARTESIAN_POINT('',(-1.53673442965256,1.,3.90876544355381));
#45413=CARTESIAN_POINT('Ctrl Pts',(-1.53673442965256,1.,3.90876544355381));
#45414=CARTESIAN_POINT('Ctrl Pts',(-1.53556639217905,1.,3.90771246855019));
#45415=CARTESIAN_POINT('Ctrl Pts',(-1.53323321827755,1.,3.90560462813969));
#45416=CARTESIAN_POINT('Ctrl Pts',(-1.52974216056287,1.,3.90243719631596));
#45417=CARTESIAN_POINT('Ctrl Pts',(-1.52510482991635,1.,3.89820260708225));
#45418=CARTESIAN_POINT('Ctrl Pts',(-1.51933724329306,1.,3.89289043533657));
#45419=CARTESIAN_POINT('Ctrl Pts',(-1.51359883110559,1.,3.88755930033884));
#45420=CARTESIAN_POINT('Ctrl Pts',(-1.50788973857757,1.,3.88220917950538));
#45421=CARTESIAN_POINT('Ctrl Pts',(-1.50221016176556,1.,3.87684006372134));
#45422=CARTESIAN_POINT('Ctrl Pts',(-1.49656035399122,1.,3.87145196998465));
#45423=CARTESIAN_POINT('Ctrl Pts',(-1.4909406116431,1.,3.86604492575189));
#45424=CARTESIAN_POINT('Ctrl Pts',(-1.48535125509919,1.,3.86061894706087));
#45425=CARTESIAN_POINT('Ctrl Pts',(-1.4797926099102,1.,3.85517401698843));
#45426=CARTESIAN_POINT('Ctrl Pts',(-1.47426499018538,1.,3.84971006847277));
#45427=CARTESIAN_POINT('Ctrl Pts',(-1.46876867426504,1.,3.84422695454796));
#45428=CARTESIAN_POINT('Ctrl Pts',(-1.46330391180752,1.,3.83872447159639));
#45429=CARTESIAN_POINT('Ctrl Pts',(-1.45787095220852,1.,3.83320241775423));
#45430=CARTESIAN_POINT('Ctrl Pts',(-1.45247006796836,1.,3.82766064519074));
#45431=CARTESIAN_POINT('Ctrl Pts',(-1.44710157648539,1.,3.82209910620533));
#45432=CARTESIAN_POINT('Ctrl Pts',(-1.44176587041347,1.,3.81651792398414));
#45433=CARTESIAN_POINT('Ctrl Pts',(-1.43646341556724,1.,3.81091737726815));
#45434=CARTESIAN_POINT('Ctrl Pts',(-1.4311946992132,1.,3.80529775429805));
#45435=CARTESIAN_POINT('Ctrl Pts',(-1.42596018777283,1.,3.7996592319632));
#45436=CARTESIAN_POINT('Ctrl Pts',(-1.42076028482836,1.,3.79400175744408));
#45437=CARTESIAN_POINT('Ctrl Pts',(-1.4155952780383,1.,3.78832489879426));
#45438=CARTESIAN_POINT('Ctrl Pts',(-1.41046532282593,1.,3.78262780065471));
#45439=CARTESIAN_POINT('Ctrl Pts',(-1.40537056004722,1.,3.77690952014259));
#45440=CARTESIAN_POINT('Ctrl Pts',(-1.40031121335505,1.,3.77116930621827));
#45441=CARTESIAN_POINT('Ctrl Pts',(-1.39528769118052,1.,3.76540689249074));
#45442=CARTESIAN_POINT('Ctrl Pts',(-1.39030069388918,1.,3.75962280650855));
#45443=CARTESIAN_POINT('Ctrl Pts',(-1.38535129801176,1.,3.75381861212707));
#45444=CARTESIAN_POINT('Ctrl Pts',(-1.38044070763295,1.,3.74799617204729));
#45445=CARTESIAN_POINT('Ctrl Pts',(-1.37557002971687,1.,3.74215698162555));
#45446=CARTESIAN_POINT('Ctrl Pts',(-1.37074003422739,1.,3.7363014588581));
#45447=CARTESIAN_POINT('Ctrl Pts',(-1.36595093298676,1.,3.73042829011295));
#45448=CARTESIAN_POINT('Ctrl Pts',(-1.36120211416354,1.,3.72453364678279));
#45449=CARTESIAN_POINT('Ctrl Pts',(-1.35649266705037,1.,3.71861271513313));
#45450=CARTESIAN_POINT('Ctrl Pts',(-1.35182193384424,1.,3.71266130563054));
#45451=CARTESIAN_POINT('Ctrl Pts',(-1.34719008463534,1.,3.70667753188248));
#45452=CARTESIAN_POINT('Ctrl Pts',(-1.34259860752933,1.,3.70066324015119));
#45453=CARTESIAN_POINT('Ctrl Pts',(-1.3380510339822,1.,3.69462613305708));
#45454=CARTESIAN_POINT('Ctrl Pts',(-1.33355191034523,1.,3.68857672413033));
#45455=CARTESIAN_POINT('Ctrl Pts',(-1.3291054707274,1.,3.68252441182551));
#45456=CARTESIAN_POINT('Ctrl Pts',(-1.32471430856415,1.,3.67647355257912));
#45457=CARTESIAN_POINT('Ctrl Pts',(-1.32037828137766,1.,3.67042021752656));
#45458=CARTESIAN_POINT('Ctrl Pts',(-1.31609271239911,1.,3.66434688899793));
#45459=CARTESIAN_POINT('Ctrl Pts',(-1.31185038411218,1.,3.65822827358617));
#45460=CARTESIAN_POINT('Ctrl Pts',(-1.30764479590039,1.,3.65204081987068));
#45461=CARTESIAN_POINT('Ctrl Pts',(-1.30347327603774,1.,3.64577181380113));
#45462=CARTESIAN_POINT('Ctrl Pts',(-1.2993395590647,1.,3.63942689872808));
#45463=CARTESIAN_POINT('Ctrl Pts',(-1.29525810207762,1.,3.63304271631046));
#45464=CARTESIAN_POINT('Ctrl Pts',(-1.29125046021878,1.,3.62667616004369));
#45465=CARTESIAN_POINT('Ctrl Pts',(-1.28733755029384,1.,3.6203814849236));
#45466=CARTESIAN_POINT('Ctrl Pts',(-1.28353255117765,1.,3.61418935913823));
#45467=CARTESIAN_POINT('Ctrl Pts',(-1.27983492861691,1.,3.60808907746339));
#45468=CARTESIAN_POINT('Ctrl Pts',(-1.27622049908625,1.,3.60199947736298));
#45469=CARTESIAN_POINT('Ctrl Pts',(-1.27264798379307,1.,3.59578698050006));
#45470=CARTESIAN_POINT('Ctrl Pts',(-1.26907758484709,1.,3.58931807846313));
#45471=CARTESIAN_POINT('Ctrl Pts',(-1.26548706249862,1.,3.58250452868618));
#45472=CARTESIAN_POINT('Ctrl Pts',(-1.2618866714281,1.,3.5753456065171));
#45473=CARTESIAN_POINT('Ctrl Pts',(-1.25834000485716,1.,3.56798645995275));
#45474=CARTESIAN_POINT('Ctrl Pts',(-1.25496090900009,1.,3.56071094991199));
#45475=CARTESIAN_POINT('Ctrl Pts',(-1.2518879294064,1.,3.55387287418985));
#45476=CARTESIAN_POINT('Ctrl Pts',(-1.24926408628003,1.,3.54784190283068));
#45477=CARTESIAN_POINT('Ctrl Pts',(-1.24721646231966,1.,3.54294877425964));
#45478=CARTESIAN_POINT('Ctrl Pts',(-1.24593497226008,1.,3.53968291130022));
#45479=CARTESIAN_POINT('Ctrl Pts',(-1.24539205388767,1.,3.53808746578196));
#45480=CARTESIAN_POINT('Ctrl Pts',(-1.2452449899111,1.,3.5374485926552));
#45481=CARTESIAN_POINT('Ctrl Pts',(-1.24524838931757,1.,3.53725139174486));
#45482=CARTESIAN_POINT('Ctrl Pts',(-1.24526366418038,1.,3.5372048861597));
#45483=CARTESIAN_POINT('',(-1.53673442965256,0.,3.90876544355381));
#45484=CARTESIAN_POINT('Ctrl Pts',(-1.62055519152809,-1.,3.38176002566879));
#45485=CARTESIAN_POINT('Ctrl Pts',(-1.62055519152809,1.,3.38176002566879));
#45486=CARTESIAN_POINT('Ctrl Pts',(-1.62058335162482,-1.,3.38167767992676));
#45487=CARTESIAN_POINT('Ctrl Pts',(-1.62058335162482,1.,3.38167767992676));
#45488=CARTESIAN_POINT('Ctrl Pts',(-1.62069532368199,-1.,3.38166984193836));
#45489=CARTESIAN_POINT('Ctrl Pts',(-1.62069532368199,1.,3.38166984193836));
#45490=CARTESIAN_POINT('Ctrl Pts',(-1.62103022181151,-1.,3.38212861099983));
#45491=CARTESIAN_POINT('Ctrl Pts',(-1.62103022181151,1.,3.38212861099983));
#45492=CARTESIAN_POINT('Ctrl Pts',(-1.62181089631344,-1.,3.38368201668574));
#45493=CARTESIAN_POINT('Ctrl Pts',(-1.62181089631344,1.,3.38368201668574));
#45494=CARTESIAN_POINT('Ctrl Pts',(-1.6233278855625,-1.,3.38715832179072));
#45495=CARTESIAN_POINT('Ctrl Pts',(-1.6233278855625,1.,3.38715832179072));
#45496=CARTESIAN_POINT('Ctrl Pts',(-1.62533996116713,-1.,3.39206617496906));
#45497=CARTESIAN_POINT('Ctrl Pts',(-1.62533996116713,1.,3.39206617496906));
#45498=CARTESIAN_POINT('Ctrl Pts',(-1.62774916464408,-1.,3.39818605297991));
#45499=CARTESIAN_POINT('Ctrl Pts',(-1.62774916464408,1.,3.39818605297991));
#45500=CARTESIAN_POINT('Ctrl Pts',(-1.63041148964828,-1.,3.40519422740235));
#45501=CARTESIAN_POINT('Ctrl Pts',(-1.63041148964828,1.,3.40519422740235));
#45502=CARTESIAN_POINT('Ctrl Pts',(-1.63316667054044,-1.,3.41272817148478));
#45503=CARTESIAN_POINT('Ctrl Pts',(-1.63316667054044,1.,3.41272817148478));
#45504=CARTESIAN_POINT('Ctrl Pts',(-1.63586250099773,-1.,3.42043974590882));
#45505=CARTESIAN_POINT('Ctrl Pts',(-1.63586250099773,1.,3.42043974590882));
#45506=CARTESIAN_POINT('Ctrl Pts',(-1.63837876246926,-1.,3.42804772926291));
#45507=CARTESIAN_POINT('Ctrl Pts',(-1.63837876246926,1.,3.42804772926291));
#45508=CARTESIAN_POINT('Ctrl Pts',(-1.64065778702023,-1.,3.43540451921548));
#45509=CARTESIAN_POINT('Ctrl Pts',(-1.64065778702023,1.,3.43540451921548));
#45510=CARTESIAN_POINT('Ctrl Pts',(-1.64270733821113,-1.,3.44250337701888));
#45511=CARTESIAN_POINT('Ctrl Pts',(-1.64270733821113,1.,3.44250337701888));
#45512=CARTESIAN_POINT('Ctrl Pts',(-1.64457408708107,-1.,3.44942242546795));
#45513=CARTESIAN_POINT('Ctrl Pts',(-1.64457408708107,1.,3.44942242546795));
#45514=CARTESIAN_POINT('Ctrl Pts',(-1.64632429697521,-1.,3.45628421062422));
#45515=CARTESIAN_POINT('Ctrl Pts',(-1.64632429697521,1.,3.45628421062422));
#45516=CARTESIAN_POINT('Ctrl Pts',(-1.64802323352738,-1.,3.46321237515));
#45517=CARTESIAN_POINT('Ctrl Pts',(-1.64802323352738,1.,3.46321237515));
#45518=CARTESIAN_POINT('Ctrl Pts',(-1.64971118698256,-1.,3.47028140995992));
#45519=CARTESIAN_POINT('Ctrl Pts',(-1.64971118698256,1.,3.47028140995992));
#45520=CARTESIAN_POINT('Ctrl Pts',(-1.65139534930322,-1.,3.47749926256476));
#45521=CARTESIAN_POINT('Ctrl Pts',(-1.65139534930322,1.,3.47749926256476));
#45522=CARTESIAN_POINT('Ctrl Pts',(-1.65306335367739,-1.,3.48483492840894));
#45523=CARTESIAN_POINT('Ctrl Pts',(-1.65306335367739,1.,3.48483492840894));
#45524=CARTESIAN_POINT('Ctrl Pts',(-1.65469162644468,-1.,3.49223525300176));
#45525=CARTESIAN_POINT('Ctrl Pts',(-1.65469162644468,1.,3.49223525300176));
#45526=CARTESIAN_POINT('Ctrl Pts',(-1.65625517961588,-1.,3.4996447647794));
#45527=CARTESIAN_POINT('Ctrl Pts',(-1.65625517961588,1.,3.4996447647794));
#45528=CARTESIAN_POINT('Ctrl Pts',(-1.65773832633632,-1.,3.50702733146542));
#45529=CARTESIAN_POINT('Ctrl Pts',(-1.65773832633632,1.,3.50702733146542));
#45530=CARTESIAN_POINT('Ctrl Pts',(-1.65913971687342,-1.,3.5143763218894));
#45531=CARTESIAN_POINT('Ctrl Pts',(-1.65913971687342,1.,3.5143763218894));
#45532=CARTESIAN_POINT('Ctrl Pts',(-1.66046645222279,-1.,3.52170261543815));
#45533=CARTESIAN_POINT('Ctrl Pts',(-1.66046645222279,1.,3.52170261543815));
#45534=CARTESIAN_POINT('Ctrl Pts',(-1.66173058912371,-1.,3.52902746211093));
#45535=CARTESIAN_POINT('Ctrl Pts',(-1.66173058912371,1.,3.52902746211093));
#45536=CARTESIAN_POINT('Ctrl Pts',(-1.66294490916111,-1.,3.5363738506022));
#45537=CARTESIAN_POINT('Ctrl Pts',(-1.66294490916111,1.,3.5363738506022));
#45538=CARTESIAN_POINT('Ctrl Pts',(-1.66411849222326,-1.,3.54375747475014));
#45539=CARTESIAN_POINT('Ctrl Pts',(-1.66411849222326,1.,3.54375747475014));
#45540=CARTESIAN_POINT('Ctrl Pts',(-1.66525401568994,-1.,3.55118121342861));
#45541=CARTESIAN_POINT('Ctrl Pts',(-1.66525401568994,1.,3.55118121342861));
#45542=CARTESIAN_POINT('Ctrl Pts',(-1.66635023293114,-1.,3.55864015233602));
#45543=CARTESIAN_POINT('Ctrl Pts',(-1.66635023293114,1.,3.55864015233602));
#45544=CARTESIAN_POINT('Ctrl Pts',(-1.66740349220305,-1.,3.56612465179422));
#45545=CARTESIAN_POINT('Ctrl Pts',(-1.66740349220305,1.,3.56612465179422));
#45546=CARTESIAN_POINT('Ctrl Pts',(-1.668409574073,-1.,3.57362406285887));
#45547=CARTESIAN_POINT('Ctrl Pts',(-1.668409574073,1.,3.57362406285887));
#45548=CARTESIAN_POINT('Ctrl Pts',(-1.66936552908232,-1.,3.58113044183829));
#45549=CARTESIAN_POINT('Ctrl Pts',(-1.66936552908232,1.,3.58113044183829));
#45550=CARTESIAN_POINT('Ctrl Pts',(-1.67027110397604,-1.,3.58864143097834));
#45551=CARTESIAN_POINT('Ctrl Pts',(-1.67027110397604,1.,3.58864143097834));
#45552=CARTESIAN_POINT('Ctrl Pts',(-1.67112775290707,-1.,3.59615824388807));
#45553=CARTESIAN_POINT('Ctrl Pts',(-1.67112775290707,1.,3.59615824388807));
#45554=CARTESIAN_POINT('Ctrl Pts',(-1.67193797318597,-1.,3.603684308152));
#45555=CARTESIAN_POINT('Ctrl Pts',(-1.67193797318597,1.,3.603684308152));
#45556=CARTESIAN_POINT('Ctrl Pts',(-1.67270452466968,-1.,3.61122367156181));
#45557=CARTESIAN_POINT('Ctrl Pts',(-1.67270452466968,1.,3.61122367156181));
#45558=CARTESIAN_POINT('Ctrl Pts',(-1.67342968196224,-1.,3.61877947398184));
#45559=CARTESIAN_POINT('Ctrl Pts',(-1.67342968196224,1.,3.61877947398184));
#45560=CARTESIAN_POINT('Ctrl Pts',(-1.67411452372271,-1.,3.62635249450923));
#45561=CARTESIAN_POINT('Ctrl Pts',(-1.67411452372271,1.,3.62635249450923));
#45562=CARTESIAN_POINT('Ctrl Pts',(-1.67475929882971,-1.,3.63394189312924));
#45563=CARTESIAN_POINT('Ctrl Pts',(-1.67475929882971,1.,3.63394189312924));
#45564=CARTESIAN_POINT('Ctrl Pts',(-1.67536373264848,-1.,3.6415458297234));
#45565=CARTESIAN_POINT('Ctrl Pts',(-1.67536373264848,1.,3.6415458297234));
#45566=CARTESIAN_POINT('Ctrl Pts',(-1.67592735946692,-1.,3.64916213574667));
#45567=CARTESIAN_POINT('Ctrl Pts',(-1.67592735946692,1.,3.64916213574667));
#45568=CARTESIAN_POINT('Ctrl Pts',(-1.6764498346945,-1.,3.6567889441642));
#45569=CARTESIAN_POINT('Ctrl Pts',(-1.6764498346945,1.,3.6567889441642));
#45570=CARTESIAN_POINT('Ctrl Pts',(-1.67693128053132,-1.,3.66442538670968));
#45571=CARTESIAN_POINT('Ctrl Pts',(-1.67693128053132,1.,3.66442538670968));
#45572=CARTESIAN_POINT('Ctrl Pts',(-1.67737217414874,-1.,3.67207136294575));
#45573=CARTESIAN_POINT('Ctrl Pts',(-1.67737217414874,1.,3.67207136294575));
#45574=CARTESIAN_POINT('Ctrl Pts',(-1.67777320475848,-1.,3.67972724579124));
#45575=CARTESIAN_POINT('Ctrl Pts',(-1.67777320475848,1.,3.67972724579124));
#45576=CARTESIAN_POINT('Ctrl Pts',(-1.67813513867965,-1.,3.68739360236487));
#45577=CARTESIAN_POINT('Ctrl Pts',(-1.67813513867965,1.,3.68739360236487));
#45578=CARTESIAN_POINT('Ctrl Pts',(-1.67845869064323,-1.,3.6950709275959));
#45579=CARTESIAN_POINT('Ctrl Pts',(-1.67845869064323,1.,3.6950709275959));
#45580=CARTESIAN_POINT('Ctrl Pts',(-1.67874436948667,-1.,3.70275932351108));
#45581=CARTESIAN_POINT('Ctrl Pts',(-1.67874436948667,1.,3.70275932351108));
#45582=CARTESIAN_POINT('Ctrl Pts',(-1.67899249793462,-1.,3.71045854208343));
#45583=CARTESIAN_POINT('Ctrl Pts',(-1.67899249793462,1.,3.71045854208343));
#45584=CARTESIAN_POINT('Ctrl Pts',(-1.67920328071708,-1.,3.71816812842322));
#45585=CARTESIAN_POINT('Ctrl Pts',(-1.67920328071708,1.,3.71816812842322));
#45586=CARTESIAN_POINT('Ctrl Pts',(-1.67937685856652,-1.,3.72588753416396));
#45587=CARTESIAN_POINT('Ctrl Pts',(-1.67937685856652,1.,3.72588753416396));
#45588=CARTESIAN_POINT('Ctrl Pts',(-1.67951336376402,-1.,3.73361623282543));
#45589=CARTESIAN_POINT('Ctrl Pts',(-1.67951336376402,1.,3.73361623282543));
#45590=CARTESIAN_POINT('Ctrl Pts',(-1.6796129868522,-1.,3.74135385965401));
#45591=CARTESIAN_POINT('Ctrl Pts',(-1.6796129868522,1.,3.74135385965401));
#45592=CARTESIAN_POINT('Ctrl Pts',(-1.67967598599525,-1.,3.7491002239452));
#45593=CARTESIAN_POINT('Ctrl Pts',(-1.67967598599525,1.,3.7491002239452));
#45594=CARTESIAN_POINT('Ctrl Pts',(-1.67970265841239,-1.,3.75685523754493));
#45595=CARTESIAN_POINT('Ctrl Pts',(-1.67970265841239,1.,3.75685523754493));
#45596=CARTESIAN_POINT('Ctrl Pts',(-1.67969332319245,-1.,3.76461886684344));
#45597=CARTESIAN_POINT('Ctrl Pts',(-1.67969332319245,1.,3.76461886684344));
#45598=CARTESIAN_POINT('Ctrl Pts',(-1.67964830084993,-1.,3.77239107928502));
#45599=CARTESIAN_POINT('Ctrl Pts',(-1.67964830084993,1.,3.77239107928502));
#45600=CARTESIAN_POINT('Ctrl Pts',(-1.67956789212141,-1.,3.78017178197317));
#45601=CARTESIAN_POINT('Ctrl Pts',(-1.67956789212141,1.,3.78017178197317));
#45602=CARTESIAN_POINT('Ctrl Pts',(-1.67945236653493,-1.,3.7879608002176));
#45603=CARTESIAN_POINT('Ctrl Pts',(-1.67945236653493,1.,3.7879608002176));
#45604=CARTESIAN_POINT('Ctrl Pts',(-1.67930196625548,-1.,3.79575791578424));
#45605=CARTESIAN_POINT('Ctrl Pts',(-1.67930196625548,1.,3.79575791578424));
#45606=CARTESIAN_POINT('Ctrl Pts',(-1.67911690648355,-1.,3.80356289079005));
#45607=CARTESIAN_POINT('Ctrl Pts',(-1.67911690648355,1.,3.80356289079005));
#45608=CARTESIAN_POINT('Ctrl Pts',(-1.6788973773827,-1.,3.81137549624178));
#45609=CARTESIAN_POINT('Ctrl Pts',(-1.6788973773827,1.,3.81137549624178));
#45610=CARTESIAN_POINT('Ctrl Pts',(-1.67864354605954,-1.,3.81919554099578));
#45611=CARTESIAN_POINT('Ctrl Pts',(-1.67864354605954,1.,3.81919554099578));
#45612=CARTESIAN_POINT('Ctrl Pts',(-1.6783555575934,-1.,3.82702289286713));
#45613=CARTESIAN_POINT('Ctrl Pts',(-1.6783555575934,1.,3.82702289286713));
#45614=CARTESIAN_POINT('Ctrl Pts',(-1.67803353064351,-1.,3.83485746513989));
#45615=CARTESIAN_POINT('Ctrl Pts',(-1.67803353064351,1.,3.83485746513989));
#45616=CARTESIAN_POINT('Ctrl Pts',(-1.67774874946079,-1.,3.84113085985244));
#45617=CARTESIAN_POINT('Ctrl Pts',(-1.67774874946079,1.,3.84113085985244));
#45618=CARTESIAN_POINT('Ctrl Pts',(-1.6775199114018,-1.,3.84583912296459));
#45619=CARTESIAN_POINT('Ctrl Pts',(-1.6775199114018,1.,3.84583912296459));
#45620=CARTESIAN_POINT('Ctrl Pts',(-1.67736057656533,-1.,3.84897939430696));
#45621=CARTESIAN_POINT('Ctrl Pts',(-1.67736057656533,1.,3.84897939430696));
#45622=CARTESIAN_POINT('Ctrl Pts',(-1.67727921511438,-1.,3.85054988729471));
#45623=CARTESIAN_POINT('Ctrl Pts',(-1.67727921511438,1.,3.85054988729471));
#45624=CARTESIAN_POINT('',(-1.62064718014094,1.,3.38171594275765));
#45625=CARTESIAN_POINT('Ctrl Pts',(-1.62064718014094,-1.,3.38171594275765));
#45626=CARTESIAN_POINT('Ctrl Pts',(-1.62064718014094,-0.666666666666667,
3.38171594275765));
#45627=CARTESIAN_POINT('Ctrl Pts',(-1.62064718014094,-0.333333333333333,
3.38171594275765));
#45628=CARTESIAN_POINT('Ctrl Pts',(-1.62064718014094,0.333333333333333,
3.38171594275765));
#45629=CARTESIAN_POINT('Ctrl Pts',(-1.62064718014094,0.666666666666667,
3.38171594275765));
#45630=CARTESIAN_POINT('Ctrl Pts',(-1.62064718014094,1.,3.38171594275765));
#45631=CARTESIAN_POINT('',(-1.67727921511438,1.,3.85054988729471));
#45632=CARTESIAN_POINT('',(-1.67727921511438,0.,3.85054988729471));
#45633=CARTESIAN_POINT('Ctrl Pts',(-1.62064718014094,1.,3.38171594275765));
#45634=CARTESIAN_POINT('Ctrl Pts',(-1.62069086551492,1.,3.38173802621259));
#45635=CARTESIAN_POINT('Ctrl Pts',(-1.62083271135947,1.,3.38187506456922));
#45636=CARTESIAN_POINT('Ctrl Pts',(-1.62118047294498,1.,3.38243080602408));
#45637=CARTESIAN_POINT('Ctrl Pts',(-1.62192472202769,1.,3.38394285763222));
#45638=CARTESIAN_POINT('Ctrl Pts',(-1.6233278855625,1.,3.38715832179072));
#45639=CARTESIAN_POINT('Ctrl Pts',(-1.62533996116713,1.,3.39206617496906));
#45640=CARTESIAN_POINT('Ctrl Pts',(-1.62774916464408,1.,3.39818605297991));
#45641=CARTESIAN_POINT('Ctrl Pts',(-1.63041148964828,1.,3.40519422740235));
#45642=CARTESIAN_POINT('Ctrl Pts',(-1.63316667054044,1.,3.41272817148478));
#45643=CARTESIAN_POINT('Ctrl Pts',(-1.63586250099773,1.,3.42043974590882));
#45644=CARTESIAN_POINT('Ctrl Pts',(-1.63837876246926,1.,3.42804772926291));
#45645=CARTESIAN_POINT('Ctrl Pts',(-1.64065778702023,1.,3.43540451921548));
#45646=CARTESIAN_POINT('Ctrl Pts',(-1.64270733821113,1.,3.44250337701888));
#45647=CARTESIAN_POINT('Ctrl Pts',(-1.64457408708107,1.,3.44942242546795));
#45648=CARTESIAN_POINT('Ctrl Pts',(-1.64632429697521,1.,3.45628421062422));
#45649=CARTESIAN_POINT('Ctrl Pts',(-1.64802323352738,1.,3.46321237515));
#45650=CARTESIAN_POINT('Ctrl Pts',(-1.64971118698256,1.,3.47028140995992));
#45651=CARTESIAN_POINT('Ctrl Pts',(-1.65139534930322,1.,3.47749926256476));
#45652=CARTESIAN_POINT('Ctrl Pts',(-1.65306335367739,1.,3.48483492840894));
#45653=CARTESIAN_POINT('Ctrl Pts',(-1.65469162644468,1.,3.49223525300176));
#45654=CARTESIAN_POINT('Ctrl Pts',(-1.65625517961588,1.,3.4996447647794));
#45655=CARTESIAN_POINT('Ctrl Pts',(-1.65773832633632,1.,3.50702733146542));
#45656=CARTESIAN_POINT('Ctrl Pts',(-1.65913971687342,1.,3.5143763218894));
#45657=CARTESIAN_POINT('Ctrl Pts',(-1.66046645222279,1.,3.52170261543815));
#45658=CARTESIAN_POINT('Ctrl Pts',(-1.66173058912371,1.,3.52902746211093));
#45659=CARTESIAN_POINT('Ctrl Pts',(-1.66294490916111,1.,3.5363738506022));
#45660=CARTESIAN_POINT('Ctrl Pts',(-1.66411849222326,1.,3.54375747475014));
#45661=CARTESIAN_POINT('Ctrl Pts',(-1.66525401568994,1.,3.55118121342861));
#45662=CARTESIAN_POINT('Ctrl Pts',(-1.66635023293114,1.,3.55864015233602));
#45663=CARTESIAN_POINT('Ctrl Pts',(-1.66740349220305,1.,3.56612465179422));
#45664=CARTESIAN_POINT('Ctrl Pts',(-1.668409574073,1.,3.57362406285887));
#45665=CARTESIAN_POINT('Ctrl Pts',(-1.66936552908232,1.,3.58113044183829));
#45666=CARTESIAN_POINT('Ctrl Pts',(-1.67027110397604,1.,3.58864143097834));
#45667=CARTESIAN_POINT('Ctrl Pts',(-1.67112775290707,1.,3.59615824388807));
#45668=CARTESIAN_POINT('Ctrl Pts',(-1.67193797318597,1.,3.603684308152));
#45669=CARTESIAN_POINT('Ctrl Pts',(-1.67270452466968,1.,3.61122367156181));
#45670=CARTESIAN_POINT('Ctrl Pts',(-1.67342968196224,1.,3.61877947398184));
#45671=CARTESIAN_POINT('Ctrl Pts',(-1.67411452372271,1.,3.62635249450923));
#45672=CARTESIAN_POINT('Ctrl Pts',(-1.67475929882971,1.,3.63394189312924));
#45673=CARTESIAN_POINT('Ctrl Pts',(-1.67536373264848,1.,3.6415458297234));
#45674=CARTESIAN_POINT('Ctrl Pts',(-1.67592735946692,1.,3.64916213574667));
#45675=CARTESIAN_POINT('Ctrl Pts',(-1.6764498346945,1.,3.6567889441642));
#45676=CARTESIAN_POINT('Ctrl Pts',(-1.67693128053132,1.,3.66442538670968));
#45677=CARTESIAN_POINT('Ctrl Pts',(-1.67737217414874,1.,3.67207136294575));
#45678=CARTESIAN_POINT('Ctrl Pts',(-1.67777320475848,1.,3.67972724579124));
#45679=CARTESIAN_POINT('Ctrl Pts',(-1.67813513867965,1.,3.68739360236487));
#45680=CARTESIAN_POINT('Ctrl Pts',(-1.67845869064323,1.,3.6950709275959));
#45681=CARTESIAN_POINT('Ctrl Pts',(-1.67874436948667,1.,3.70275932351108));
#45682=CARTESIAN_POINT('Ctrl Pts',(-1.67899249793462,1.,3.71045854208343));
#45683=CARTESIAN_POINT('Ctrl Pts',(-1.67920328071708,1.,3.71816812842322));
#45684=CARTESIAN_POINT('Ctrl Pts',(-1.67937685856652,1.,3.72588753416396));
#45685=CARTESIAN_POINT('Ctrl Pts',(-1.67951336376402,1.,3.73361623282543));
#45686=CARTESIAN_POINT('Ctrl Pts',(-1.6796129868522,1.,3.74135385965401));
#45687=CARTESIAN_POINT('Ctrl Pts',(-1.67967598599525,1.,3.7491002239452));
#45688=CARTESIAN_POINT('Ctrl Pts',(-1.67970265841239,1.,3.75685523754493));
#45689=CARTESIAN_POINT('Ctrl Pts',(-1.67969332319245,1.,3.76461886684344));
#45690=CARTESIAN_POINT('Ctrl Pts',(-1.67964830084993,1.,3.77239107928502));
#45691=CARTESIAN_POINT('Ctrl Pts',(-1.67956789212141,1.,3.78017178197317));
#45692=CARTESIAN_POINT('Ctrl Pts',(-1.67945236653493,1.,3.7879608002176));
#45693=CARTESIAN_POINT('Ctrl Pts',(-1.67930196625548,1.,3.79575791578424));
#45694=CARTESIAN_POINT('Ctrl Pts',(-1.67911690648355,1.,3.80356289079005));
#45695=CARTESIAN_POINT('Ctrl Pts',(-1.6788973773827,1.,3.81137549624178));
#45696=CARTESIAN_POINT('Ctrl Pts',(-1.67864354605954,1.,3.81919554099578));
#45697=CARTESIAN_POINT('Ctrl Pts',(-1.6783555575934,1.,3.82702289286713));
#45698=CARTESIAN_POINT('Ctrl Pts',(-1.67803353064351,1.,3.83485746513989));
#45699=CARTESIAN_POINT('Ctrl Pts',(-1.67774874946079,1.,3.84113085985244));
#45700=CARTESIAN_POINT('Ctrl Pts',(-1.6775199114018,1.,3.84583912296459));
#45701=CARTESIAN_POINT('Ctrl Pts',(-1.67736057656533,1.,3.84897939430696));
#45702=CARTESIAN_POINT('Ctrl Pts',(-1.67727921511438,1.,3.85054988729471));
#45703=CARTESIAN_POINT('Origin',(-1.67727921511438,0.,3.85054988729471));
#45704=CARTESIAN_POINT('',(-1.53673442965256,1.,3.90876544355381));
#45705=CARTESIAN_POINT('Origin',(0.,0.,0.));
#45706=CARTESIAN_POINT('',(-1.78327315618183,1.,3.29885386921599));
#45707=CARTESIAN_POINT('Origin',(0.,1.,0.));
#45708=CARTESIAN_POINT('Ctrl Pts',(-1.78327315618183,1.,3.29885386921599));
#45709=CARTESIAN_POINT('Ctrl Pts',(-1.78327315618183,0.666666666666667,
3.29885386921599));
#45710=CARTESIAN_POINT('Ctrl Pts',(-1.78327315618183,0.333333333333333,
3.29885386921599));
#45711=CARTESIAN_POINT('Ctrl Pts',(-1.78327315618183,-0.333333333333333,
3.29885386921599));
#45712=CARTESIAN_POINT('Ctrl Pts',(-1.78327315618183,-0.666666666666667,
3.29885386921599));
#45713=CARTESIAN_POINT('Ctrl Pts',(-1.78327315618183,-1.,3.29885386921599));
#45714=CARTESIAN_POINT('Ctrl Pts',(-2.12928030988903,-1.,3.62024382630768));
#45715=CARTESIAN_POINT('Ctrl Pts',(-2.12928030988903,1.,3.62024382630768));
#45716=CARTESIAN_POINT('Ctrl Pts',(-2.12796193131368,-1.,3.61938653649098));
#45717=CARTESIAN_POINT('Ctrl Pts',(-2.12796193131368,1.,3.61938653649098));
#45718=CARTESIAN_POINT('Ctrl Pts',(-2.12532774376758,-1.,3.61766963590482));
#45719=CARTESIAN_POINT('Ctrl Pts',(-2.12532774376758,1.,3.61766963590482));
#45720=CARTESIAN_POINT('Ctrl Pts',(-2.12138417126355,-1.,3.61508732216891));
#45721=CARTESIAN_POINT('Ctrl Pts',(-2.12138417126355,1.,3.61508732216891));
#45722=CARTESIAN_POINT('Ctrl Pts',(-2.11614149815106,-1.,3.61163030609447));
#45723=CARTESIAN_POINT('Ctrl Pts',(-2.11614149815106,1.,3.61163030609447));
#45724=CARTESIAN_POINT('Ctrl Pts',(-2.10961391334462,-1.,3.60728578532601));
#45725=CARTESIAN_POINT('Ctrl Pts',(-2.10961391334462,1.,3.60728578532601));
#45726=CARTESIAN_POINT('Ctrl Pts',(-2.1031121772821,-1.,3.60291797088734));
#45727=CARTESIAN_POINT('Ctrl Pts',(-2.1031121772821,1.,3.60291797088734));
#45728=CARTESIAN_POINT('Ctrl Pts',(-2.09663642986631,-1.,3.59852681775485));
#45729=CARTESIAN_POINT('Ctrl Pts',(-2.09663642986631,1.,3.59852681775485));
#45730=CARTESIAN_POINT('Ctrl Pts',(-2.09018686331416,-1.,3.59411228625588));
#45731=CARTESIAN_POINT('Ctrl Pts',(-2.09018686331416,1.,3.59411228625588));
#45732=CARTESIAN_POINT('Ctrl Pts',(-2.08376373048756,-1.,3.58967435355088));
#45733=CARTESIAN_POINT('Ctrl Pts',(-2.08376373048756,1.,3.58967435355088));
#45734=CARTESIAN_POINT('Ctrl Pts',(-2.07736732842117,-1.,3.58521300039299));
#45735=CARTESIAN_POINT('Ctrl Pts',(-2.07736732842117,1.,3.58521300039299));
#45736=CARTESIAN_POINT('Ctrl Pts',(-2.07099797605747,-1.,3.58072819250442));
#45737=CARTESIAN_POINT('Ctrl Pts',(-2.07099797605747,1.,3.58072819250442));
#45738=CARTESIAN_POINT('Ctrl Pts',(-2.06465599229174,-1.,3.576219862243));
#45739=CARTESIAN_POINT('Ctrl Pts',(-2.06465599229174,1.,3.576219862243));
#45740=CARTESIAN_POINT('Ctrl Pts',(-2.05834167687523,-1.,3.57168789423507));
#45741=CARTESIAN_POINT('Ctrl Pts',(-2.05834167687523,1.,3.57168789423507));
#45742=CARTESIAN_POINT('Ctrl Pts',(-2.0520552817309,-1.,3.56713209978207));
#45743=CARTESIAN_POINT('Ctrl Pts',(-2.0520552817309,1.,3.56713209978207));
#45744=CARTESIAN_POINT('Ctrl Pts',(-2.04579702159056,-1.,3.5625522387181));
#45745=CARTESIAN_POINT('Ctrl Pts',(-2.04579702159056,1.,3.5625522387181));
#45746=CARTESIAN_POINT('Ctrl Pts',(-2.03956711120099,-1.,3.55794807265052));
#45747=CARTESIAN_POINT('Ctrl Pts',(-2.03956711120099,1.,3.55794807265052));
#45748=CARTESIAN_POINT('Ctrl Pts',(-2.03336579658174,-1.,3.55331941294018));
#45749=CARTESIAN_POINT('Ctrl Pts',(-2.03336579658174,1.,3.55331941294018));
#45750=CARTESIAN_POINT('Ctrl Pts',(-2.02719338376144,-1.,3.54866616282173));
#45751=CARTESIAN_POINT('Ctrl Pts',(-2.02719338376144,1.,3.54866616282173));
#45752=CARTESIAN_POINT('Ctrl Pts',(-2.0210502798303,-1.,3.54398838254011));
#45753=CARTESIAN_POINT('Ctrl Pts',(-2.0210502798303,1.,3.54398838254011));
#45754=CARTESIAN_POINT('Ctrl Pts',(-2.0149369884727,-1.,3.53928627453503));
#45755=CARTESIAN_POINT('Ctrl Pts',(-2.0149369884727,1.,3.53928627453503));
#45756=CARTESIAN_POINT('Ctrl Pts',(-2.00885403604685,-1.,3.53456004727321));
#45757=CARTESIAN_POINT('Ctrl Pts',(-2.00885403604685,1.,3.53456004727321));
#45758=CARTESIAN_POINT('Ctrl Pts',(-2.00280191090341,-1.,3.52980980250181));
#45759=CARTESIAN_POINT('Ctrl Pts',(-2.00280191090341,1.,3.52980980250181));
#45760=CARTESIAN_POINT('Ctrl Pts',(-1.99678100339305,-1.,3.52503542491745));
#45761=CARTESIAN_POINT('Ctrl Pts',(-1.99678100339305,1.,3.52503542491745));
#45762=CARTESIAN_POINT('Ctrl Pts',(-1.99079153006143,-1.,3.52023644289195));
#45763=CARTESIAN_POINT('Ctrl Pts',(-1.99079153006143,1.,3.52023644289195));
#45764=CARTESIAN_POINT('Ctrl Pts',(-1.98483351061066,-1.,3.51541198728362));
#45765=CARTESIAN_POINT('Ctrl Pts',(-1.98483351061066,1.,3.51541198728362));
#45766=CARTESIAN_POINT('Ctrl Pts',(-1.97890693666316,-1.,3.51056110478334));
#45767=CARTESIAN_POINT('Ctrl Pts',(-1.97890693666316,1.,3.51056110478334));
#45768=CARTESIAN_POINT('Ctrl Pts',(-1.9730119116298,-1.,3.505683018611));
#45769=CARTESIAN_POINT('Ctrl Pts',(-1.9730119116298,1.,3.505683018611));
#45770=CARTESIAN_POINT('Ctrl Pts',(-1.9671487972405,-1.,3.50077740176262));
#45771=CARTESIAN_POINT('Ctrl Pts',(-1.9671487972405,1.,3.50077740176262));
#45772=CARTESIAN_POINT('Ctrl Pts',(-1.96131836776489,-1.,3.49584466573045));
#45773=CARTESIAN_POINT('Ctrl Pts',(-1.96131836776489,1.,3.49584466573045));
#45774=CARTESIAN_POINT('Ctrl Pts',(-1.95552193112071,-1.,3.49088618670967));
#45775=CARTESIAN_POINT('Ctrl Pts',(-1.95552193112071,1.,3.49088618670967));
#45776=CARTESIAN_POINT('Ctrl Pts',(-1.94976096795902,-1.,3.485903616108));
#45777=CARTESIAN_POINT('Ctrl Pts',(-1.94976096795902,1.,3.485903616108));
#45778=CARTESIAN_POINT('Ctrl Pts',(-1.94403680554062,-1.,3.48089825770411));
#45779=CARTESIAN_POINT('Ctrl Pts',(-1.94403680554062,1.,3.48089825770411));
#45780=CARTESIAN_POINT('Ctrl Pts',(-1.93835026973888,-1.,3.47587040389916));
#45781=CARTESIAN_POINT('Ctrl Pts',(-1.93835026973888,1.,3.47587040389916));
#45782=CARTESIAN_POINT('Ctrl Pts',(-1.93270136427083,-1.,3.47081872409783));
#45783=CARTESIAN_POINT('Ctrl Pts',(-1.93270136427083,1.,3.47081872409783));
#45784=CARTESIAN_POINT('Ctrl Pts',(-1.92708888591159,-1.,3.46573953254084));
#45785=CARTESIAN_POINT('Ctrl Pts',(-1.92708888591159,1.,3.46573953254084));
#45786=CARTESIAN_POINT('Ctrl Pts',(-1.9215111821321,-1.,3.4606282172248));
#45787=CARTESIAN_POINT('Ctrl Pts',(-1.9215111821321,1.,3.4606282172248));
#45788=CARTESIAN_POINT('Ctrl Pts',(-1.9159669478406,-1.,3.45548074309943));
#45789=CARTESIAN_POINT('Ctrl Pts',(-1.9159669478406,1.,3.45548074309943));
#45790=CARTESIAN_POINT('Ctrl Pts',(-1.91045605593638,-1.,3.45029522038885));
#45791=CARTESIAN_POINT('Ctrl Pts',(-1.91045605593638,1.,3.45029522038885));
#45792=CARTESIAN_POINT('Ctrl Pts',(-1.90498026502308,-1.,3.44507323983374));
#45793=CARTESIAN_POINT('Ctrl Pts',(-1.90498026502308,1.,3.44507323983374));
#45794=CARTESIAN_POINT('Ctrl Pts',(-1.89954426803392,-1.,3.43982185678105));
#45795=CARTESIAN_POINT('Ctrl Pts',(-1.89954426803392,1.,3.43982185678105));
#45796=CARTESIAN_POINT('Ctrl Pts',(-1.89415420002553,-1.,3.43455074411591));
#45797=CARTESIAN_POINT('Ctrl Pts',(-1.89415420002553,1.,3.43455074411591));
#45798=CARTESIAN_POINT('Ctrl Pts',(-1.88881571322018,-1.,3.42926852222174));
#45799=CARTESIAN_POINT('Ctrl Pts',(-1.88881571322018,1.,3.42926852222174));
#45800=CARTESIAN_POINT('Ctrl Pts',(-1.88353205062063,-1.,3.42397908819741));
#45801=CARTESIAN_POINT('Ctrl Pts',(-1.88353205062063,1.,3.42397908819741));
#45802=CARTESIAN_POINT('Ctrl Pts',(-1.87830245689338,-1.,3.4186785838376));
#45803=CARTESIAN_POINT('Ctrl Pts',(-1.87830245689338,1.,3.4186785838376));
#45804=CARTESIAN_POINT('Ctrl Pts',(-1.87311957248106,-1.,3.41335043875182));
#45805=CARTESIAN_POINT('Ctrl Pts',(-1.87311957248106,1.,3.41335043875182));
#45806=CARTESIAN_POINT('Ctrl Pts',(-1.86797231196635,-1.,3.40797080000513));
#45807=CARTESIAN_POINT('Ctrl Pts',(-1.86797231196635,1.,3.40797080000513));
#45808=CARTESIAN_POINT('Ctrl Pts',(-1.86285057051228,-1.,3.40251742305445));
#45809=CARTESIAN_POINT('Ctrl Pts',(-1.86285057051228,1.,3.40251742305445));
#45810=CARTESIAN_POINT('Ctrl Pts',(-1.85774972037055,-1.,3.39697816833056));
#45811=CARTESIAN_POINT('Ctrl Pts',(-1.85774972037055,1.,3.39697816833056));
#45812=CARTESIAN_POINT('Ctrl Pts',(-1.85267433291778,-1.,3.39135802549415));
#45813=CARTESIAN_POINT('Ctrl Pts',(-1.85267433291778,1.,3.39135802549415));
#45814=CARTESIAN_POINT('Ctrl Pts',(-1.84764441927778,-1.,3.38569092349639));
#45815=CARTESIAN_POINT('Ctrl Pts',(-1.84764441927778,1.,3.38569092349639));
#45816=CARTESIAN_POINT('Ctrl Pts',(-1.84269016931679,-1.,3.38002968341222));
#45817=CARTESIAN_POINT('Ctrl Pts',(-1.84269016931679,1.,3.38002968341222));
#45818=CARTESIAN_POINT('Ctrl Pts',(-1.83784072967111,-1.,3.37442462015914));
#45819=CARTESIAN_POINT('Ctrl Pts',(-1.83784072967111,1.,3.37442462015914));
#45820=CARTESIAN_POINT('Ctrl Pts',(-1.83311391452338,-1.,3.36890396271864));
#45821=CARTESIAN_POINT('Ctrl Pts',(-1.83311391452338,1.,3.36890396271864));
#45822=CARTESIAN_POINT('Ctrl Pts',(-1.82850752153182,-1.,3.36345722124127));
#45823=CARTESIAN_POINT('Ctrl Pts',(-1.82850752153182,1.,3.36345722124127));
#45824=CARTESIAN_POINT('Ctrl Pts',(-1.82398496829247,-1.,3.35800801557326));
#45825=CARTESIAN_POINT('Ctrl Pts',(-1.82398496829247,1.,3.35800801557326));
#45826=CARTESIAN_POINT('Ctrl Pts',(-1.81948458796748,-1.,3.35243086937451));
#45827=CARTESIAN_POINT('Ctrl Pts',(-1.81948458796748,1.,3.35243086937451));
#45828=CARTESIAN_POINT('Ctrl Pts',(-1.81494618732772,-1.,3.34660014370527));
#45829=CARTESIAN_POINT('Ctrl Pts',(-1.81494618732772,1.,3.34660014370527));
#45830=CARTESIAN_POINT('Ctrl Pts',(-1.81033399625311,-1.,3.34043216147532));
#45831=CARTESIAN_POINT('Ctrl Pts',(-1.81033399625311,1.,3.34043216147532));
#45832=CARTESIAN_POINT('Ctrl Pts',(-1.80565802981138,-1.,3.33392460276874));
#45833=CARTESIAN_POINT('Ctrl Pts',(-1.80565802981138,1.,3.33392460276874));
#45834=CARTESIAN_POINT('Ctrl Pts',(-1.80100380443535,-1.,3.3272108803981));
#45835=CARTESIAN_POINT('Ctrl Pts',(-1.80100380443535,1.,3.3272108803981));
#45836=CARTESIAN_POINT('Ctrl Pts',(-1.79652817033444,-1.,3.32055355101168));
#45837=CARTESIAN_POINT('Ctrl Pts',(-1.79652817033444,1.,3.32055355101168));
#45838=CARTESIAN_POINT('Ctrl Pts',(-1.79242331350137,-1.,3.31428038326763));
#45839=CARTESIAN_POINT('Ctrl Pts',(-1.79242331350137,1.,3.31428038326763));
#45840=CARTESIAN_POINT('Ctrl Pts',(-1.78888832245965,-1.,3.30873412266954));
#45841=CARTESIAN_POINT('Ctrl Pts',(-1.78888832245965,1.,3.30873412266954));
#45842=CARTESIAN_POINT('Ctrl Pts',(-1.78610045419769,-1.,3.30422155558973));
#45843=CARTESIAN_POINT('Ctrl Pts',(-1.78610045419769,1.,3.30422155558973));
#45844=CARTESIAN_POINT('Ctrl Pts',(-1.78417972819696,-1.,3.30095096463082));
#45845=CARTESIAN_POINT('Ctrl Pts',(-1.78417972819696,1.,3.30095096463082));
#45846=CARTESIAN_POINT('Ctrl Pts',(-1.78338186555671,-1.,3.29940631673818));
#45847=CARTESIAN_POINT('Ctrl Pts',(-1.78338186555671,1.,3.29940631673818));
#45848=CARTESIAN_POINT('Ctrl Pts',(-1.78320756177191,-1.,3.29886572077303));
#45849=CARTESIAN_POINT('Ctrl Pts',(-1.78320756177191,1.,3.29886572077303));
#45850=CARTESIAN_POINT('Ctrl Pts',(-1.78327971836272,-1.,3.29877974053191));
#45851=CARTESIAN_POINT('Ctrl Pts',(-1.78327971836272,1.,3.29877974053191));
#45852=CARTESIAN_POINT('Ctrl Pts',(-1.7833628895577,-1.,3.2988053601491));
#45853=CARTESIAN_POINT('Ctrl Pts',(-1.7833628895577,1.,3.2988053601491));
#45854=CARTESIAN_POINT('',(-2.12928030988903,1.,3.62024382630768));
#45855=CARTESIAN_POINT('Ctrl Pts',(-2.12928030988903,1.,3.62024382630768));
#45856=CARTESIAN_POINT('Ctrl Pts',(-2.12796193131368,1.,3.61938653649098));
#45857=CARTESIAN_POINT('Ctrl Pts',(-2.12532774376758,1.,3.61766963590482));
#45858=CARTESIAN_POINT('Ctrl Pts',(-2.12138417126355,1.,3.61508732216891));
#45859=CARTESIAN_POINT('Ctrl Pts',(-2.11614149815106,1.,3.61163030609447));
#45860=CARTESIAN_POINT('Ctrl Pts',(-2.10961391334462,1.,3.60728578532601));
#45861=CARTESIAN_POINT('Ctrl Pts',(-2.1031121772821,1.,3.60291797088734));
#45862=CARTESIAN_POINT('Ctrl Pts',(-2.09663642986631,1.,3.59852681775485));
#45863=CARTESIAN_POINT('Ctrl Pts',(-2.09018686331416,1.,3.59411228625588));
#45864=CARTESIAN_POINT('Ctrl Pts',(-2.08376373048756,1.,3.58967435355088));
#45865=CARTESIAN_POINT('Ctrl Pts',(-2.07736732842117,1.,3.58521300039299));
#45866=CARTESIAN_POINT('Ctrl Pts',(-2.07099797605747,1.,3.58072819250442));
#45867=CARTESIAN_POINT('Ctrl Pts',(-2.06465599229174,1.,3.576219862243));
#45868=CARTESIAN_POINT('Ctrl Pts',(-2.05834167687523,1.,3.57168789423507));
#45869=CARTESIAN_POINT('Ctrl Pts',(-2.0520552817309,1.,3.56713209978207));
#45870=CARTESIAN_POINT('Ctrl Pts',(-2.04579702159056,1.,3.5625522387181));
#45871=CARTESIAN_POINT('Ctrl Pts',(-2.03956711120099,1.,3.55794807265052));
#45872=CARTESIAN_POINT('Ctrl Pts',(-2.03336579658174,1.,3.55331941294018));
#45873=CARTESIAN_POINT('Ctrl Pts',(-2.02719338376144,1.,3.54866616282173));
#45874=CARTESIAN_POINT('Ctrl Pts',(-2.0210502798303,1.,3.54398838254011));
#45875=CARTESIAN_POINT('Ctrl Pts',(-2.0149369884727,1.,3.53928627453503));
#45876=CARTESIAN_POINT('Ctrl Pts',(-2.00885403604685,1.,3.53456004727321));
#45877=CARTESIAN_POINT('Ctrl Pts',(-2.00280191090341,1.,3.52980980250181));
#45878=CARTESIAN_POINT('Ctrl Pts',(-1.99678100339305,1.,3.52503542491745));
#45879=CARTESIAN_POINT('Ctrl Pts',(-1.99079153006143,1.,3.52023644289195));
#45880=CARTESIAN_POINT('Ctrl Pts',(-1.98483351061066,1.,3.51541198728362));
#45881=CARTESIAN_POINT('Ctrl Pts',(-1.97890693666316,1.,3.51056110478334));
#45882=CARTESIAN_POINT('Ctrl Pts',(-1.9730119116298,1.,3.505683018611));
#45883=CARTESIAN_POINT('Ctrl Pts',(-1.9671487972405,1.,3.50077740176262));
#45884=CARTESIAN_POINT('Ctrl Pts',(-1.96131836776489,1.,3.49584466573045));
#45885=CARTESIAN_POINT('Ctrl Pts',(-1.95552193112071,1.,3.49088618670967));
#45886=CARTESIAN_POINT('Ctrl Pts',(-1.94976096795902,1.,3.485903616108));
#45887=CARTESIAN_POINT('Ctrl Pts',(-1.94403680554062,1.,3.48089825770411));
#45888=CARTESIAN_POINT('Ctrl Pts',(-1.93835026973888,1.,3.47587040389916));
#45889=CARTESIAN_POINT('Ctrl Pts',(-1.93270136427083,1.,3.47081872409783));
#45890=CARTESIAN_POINT('Ctrl Pts',(-1.92708888591159,1.,3.46573953254084));
#45891=CARTESIAN_POINT('Ctrl Pts',(-1.9215111821321,1.,3.4606282172248));
#45892=CARTESIAN_POINT('Ctrl Pts',(-1.9159669478406,1.,3.45548074309943));
#45893=CARTESIAN_POINT('Ctrl Pts',(-1.91045605593638,1.,3.45029522038885));
#45894=CARTESIAN_POINT('Ctrl Pts',(-1.90498026502308,1.,3.44507323983374));
#45895=CARTESIAN_POINT('Ctrl Pts',(-1.89954426803392,1.,3.43982185678105));
#45896=CARTESIAN_POINT('Ctrl Pts',(-1.89415420002553,1.,3.43455074411591));
#45897=CARTESIAN_POINT('Ctrl Pts',(-1.88881571322018,1.,3.42926852222174));
#45898=CARTESIAN_POINT('Ctrl Pts',(-1.88353205062063,1.,3.42397908819741));
#45899=CARTESIAN_POINT('Ctrl Pts',(-1.87830245689338,1.,3.4186785838376));
#45900=CARTESIAN_POINT('Ctrl Pts',(-1.87311957248106,1.,3.41335043875182));
#45901=CARTESIAN_POINT('Ctrl Pts',(-1.86797231196635,1.,3.40797080000513));
#45902=CARTESIAN_POINT('Ctrl Pts',(-1.86285057051228,1.,3.40251742305445));
#45903=CARTESIAN_POINT('Ctrl Pts',(-1.85774972037055,1.,3.39697816833056));
#45904=CARTESIAN_POINT('Ctrl Pts',(-1.85267433291778,1.,3.39135802549415));
#45905=CARTESIAN_POINT('Ctrl Pts',(-1.84764441927778,1.,3.38569092349639));
#45906=CARTESIAN_POINT('Ctrl Pts',(-1.84269016931679,1.,3.38002968341222));
#45907=CARTESIAN_POINT('Ctrl Pts',(-1.83784072967111,1.,3.37442462015914));
#45908=CARTESIAN_POINT('Ctrl Pts',(-1.83311391452338,1.,3.36890396271864));
#45909=CARTESIAN_POINT('Ctrl Pts',(-1.82850752153182,1.,3.36345722124127));
#45910=CARTESIAN_POINT('Ctrl Pts',(-1.82398496829247,1.,3.35800801557326));
#45911=CARTESIAN_POINT('Ctrl Pts',(-1.81948458796748,1.,3.35243086937451));
#45912=CARTESIAN_POINT('Ctrl Pts',(-1.81494618732772,1.,3.34660014370527));
#45913=CARTESIAN_POINT('Ctrl Pts',(-1.81033399625311,1.,3.34043216147532));
#45914=CARTESIAN_POINT('Ctrl Pts',(-1.80565802981138,1.,3.33392460276874));
#45915=CARTESIAN_POINT('Ctrl Pts',(-1.80100380443535,1.,3.3272108803981));
#45916=CARTESIAN_POINT('Ctrl Pts',(-1.79652817033444,1.,3.32055355101168));
#45917=CARTESIAN_POINT('Ctrl Pts',(-1.79242331350137,1.,3.31428038326763));
#45918=CARTESIAN_POINT('Ctrl Pts',(-1.78888832245965,1.,3.30873412266954));
#45919=CARTESIAN_POINT('Ctrl Pts',(-1.78610045419769,1.,3.30422155558973));
#45920=CARTESIAN_POINT('Ctrl Pts',(-1.7843238478823,1.,3.30119637003466));
#45921=CARTESIAN_POINT('Ctrl Pts',(-1.78353803106983,1.,3.29970549824337));
#45922=CARTESIAN_POINT('Ctrl Pts',(-1.78329283591903,1.,3.29909749657945));
#45923=CARTESIAN_POINT('Ctrl Pts',(-1.78326534445426,1.,3.29890219175522));
#45924=CARTESIAN_POINT('Ctrl Pts',(-1.78327315618183,1.,3.29885386921599));
#45925=CARTESIAN_POINT('',(-2.12928030988903,0.,3.62024382630768));
#45926=CARTESIAN_POINT('Ctrl Pts',(-2.12962728847315,-1.,3.08661426358891));
#45927=CARTESIAN_POINT('Ctrl Pts',(-2.12962728847315,1.,3.08661426358891));
#45928=CARTESIAN_POINT('Ctrl Pts',(-2.12964222016025,-1.,3.08652852644995));
#45929=CARTESIAN_POINT('Ctrl Pts',(-2.12964222016025,1.,3.08652852644995));
#45930=CARTESIAN_POINT('Ctrl Pts',(-2.12975158752407,-1.,3.08650326867133));
#45931=CARTESIAN_POINT('Ctrl Pts',(-2.12975158752407,1.,3.08650326867133));
#45932=CARTESIAN_POINT('Ctrl Pts',(-2.1301541297946,-1.,3.08690399991463));
#45933=CARTESIAN_POINT('Ctrl Pts',(-2.1301541297946,1.,3.08690399991463));
#45934=CARTESIAN_POINT('Ctrl Pts',(-2.13116819908542,-1.,3.08831615620074));
#45935=CARTESIAN_POINT('Ctrl Pts',(-2.13116819908542,1.,3.08831615620074));
#45936=CARTESIAN_POINT('Ctrl Pts',(-2.13321032560893,-1.,3.09151235281963));
#45937=CARTESIAN_POINT('Ctrl Pts',(-2.13321032560893,1.,3.09151235281963));
#45938=CARTESIAN_POINT('Ctrl Pts',(-2.13596538661048,-1.,3.0960450242104));
#45939=CARTESIAN_POINT('Ctrl Pts',(-2.13596538661048,1.,3.0960450242104));
#45940=CARTESIAN_POINT('Ctrl Pts',(-2.13930228863751,-1.,3.10171267391049));
#45941=CARTESIAN_POINT('Ctrl Pts',(-2.13930228863751,1.,3.10171267391049));
#45942=CARTESIAN_POINT('Ctrl Pts',(-2.14302815601973,-1.,3.10821808668859));
#45943=CARTESIAN_POINT('Ctrl Pts',(-2.14302815601973,1.,3.10821808668859));
#45944=CARTESIAN_POINT('Ctrl Pts',(-2.14692798457532,-1.,3.11522827016855));
#45945=CARTESIAN_POINT('Ctrl Pts',(-2.14692798457532,1.,3.11522827016855));
#45946=CARTESIAN_POINT('Ctrl Pts',(-2.15079698090585,-1.,3.12242318151938));
#45947=CARTESIAN_POINT('Ctrl Pts',(-2.15079698090585,1.,3.12242318151938));
#45948=CARTESIAN_POINT('Ctrl Pts',(-2.1544724138292,-1.,3.12954386795646));
#45949=CARTESIAN_POINT('Ctrl Pts',(-2.1544724138292,1.,3.12954386795646));
#45950=CARTESIAN_POINT('Ctrl Pts',(-2.15787423530676,-1.,3.13645356563038));
#45951=CARTESIAN_POINT('Ctrl Pts',(-2.15787423530676,1.,3.13645356563038));
#45952=CARTESIAN_POINT('Ctrl Pts',(-2.16100905914435,-1.,3.14314440427022));
#45953=CARTESIAN_POINT('Ctrl Pts',(-2.16100905914435,1.,3.14314440427022));
#45954=CARTESIAN_POINT('Ctrl Pts',(-2.16393520288072,-1.,3.14968624389054));
#45955=CARTESIAN_POINT('Ctrl Pts',(-2.16393520288072,1.,3.14968624389054));
#45956=CARTESIAN_POINT('Ctrl Pts',(-2.1667372844769,-1.,3.15618975593656));
#45957=CARTESIAN_POINT('Ctrl Pts',(-2.1667372844769,1.,3.15618975593656));
#45958=CARTESIAN_POINT('Ctrl Pts',(-2.16949910801219,-1.,3.16276685102972));
#45959=CARTESIAN_POINT('Ctrl Pts',(-2.16949910801219,1.,3.16276685102972));
#45960=CARTESIAN_POINT('Ctrl Pts',(-2.17227212063817,-1.,3.16948480019497));
#45961=CARTESIAN_POINT('Ctrl Pts',(-2.17227212063817,1.,3.16948480019497));
#45962=CARTESIAN_POINT('Ctrl Pts',(-2.17506466903694,-1.,3.17635032802523));
#45963=CARTESIAN_POINT('Ctrl Pts',(-2.17506466903694,1.,3.17635032802523));
#45964=CARTESIAN_POINT('Ctrl Pts',(-2.17785968847142,-1.,3.18333474627807));
#45965=CARTESIAN_POINT('Ctrl Pts',(-2.17785968847142,1.,3.18333474627807));
#45966=CARTESIAN_POINT('Ctrl Pts',(-2.18062558031778,-1.,3.19038924261573));
#45967=CARTESIAN_POINT('Ctrl Pts',(-2.18062558031778,1.,3.19038924261573));
#45968=CARTESIAN_POINT('Ctrl Pts',(-2.18332898656602,-1.,3.19746293740411));
#45969=CARTESIAN_POINT('Ctrl Pts',(-2.18332898656602,1.,3.19746293740411));
#45970=CARTESIAN_POINT('Ctrl Pts',(-2.18594876115934,-1.,3.20452259717976));
#45971=CARTESIAN_POINT('Ctrl Pts',(-2.18594876115934,1.,3.20452259717976));
#45972=CARTESIAN_POINT('Ctrl Pts',(-2.18848253363901,-1.,3.21156188355769));
#45973=CARTESIAN_POINT('Ctrl Pts',(-2.18848253363901,1.,3.21156188355769));
#45974=CARTESIAN_POINT('Ctrl Pts',(-2.19093901948667,-1.,3.21859043114095));
#45975=CARTESIAN_POINT('Ctrl Pts',(-2.19093901948667,1.,3.21859043114095));
#45976=CARTESIAN_POINT('Ctrl Pts',(-2.19333345123538,-1.,3.22562734221646));
#45977=CARTESIAN_POINT('Ctrl Pts',(-2.19333345123538,1.,3.22562734221646));
#45978=CARTESIAN_POINT('Ctrl Pts',(-2.19568204933168,-1.,3.23269332296933));
#45979=CARTESIAN_POINT('Ctrl Pts',(-2.19568204933168,1.,3.23269332296933));
#45980=CARTESIAN_POINT('Ctrl Pts',(-2.19799623693253,-1.,3.23980245361308));
#45981=CARTESIAN_POINT('Ctrl Pts',(-2.19799623693253,1.,3.23980245361308));
#45982=CARTESIAN_POINT('Ctrl Pts',(-2.20027910880981,-1.,3.24695715874338));
#45983=CARTESIAN_POINT('Ctrl Pts',(-2.20027910880981,1.,3.24695715874338));
#45984=CARTESIAN_POINT('Ctrl Pts',(-2.20252866491545,-1.,3.25415277957775));
#45985=CARTESIAN_POINT('Ctrl Pts',(-2.20252866491545,1.,3.25415277957775));
#45986=CARTESIAN_POINT('Ctrl Pts',(-2.20473979048678,-1.,3.26138036637705));
#45987=CARTESIAN_POINT('Ctrl Pts',(-2.20473979048678,1.,3.26138036637705));
#45988=CARTESIAN_POINT('Ctrl Pts',(-2.20690665217743,-1.,3.26863006136782));
#45989=CARTESIAN_POINT('Ctrl Pts',(-2.20690665217743,1.,3.26863006136782));
#45990=CARTESIAN_POINT('Ctrl Pts',(-2.2090250941743,-1.,3.2758944800554));
#45991=CARTESIAN_POINT('Ctrl Pts',(-2.2090250941743,1.,3.2758944800554));
#45992=CARTESIAN_POINT('Ctrl Pts',(-2.21109449750641,-1.,3.28317133333131));
#45993=CARTESIAN_POINT('Ctrl Pts',(-2.21109449750641,1.,3.28317133333131));
#45994=CARTESIAN_POINT('Ctrl Pts',(-2.21311648827391,-1.,3.29046159238343));
#45995=CARTESIAN_POINT('Ctrl Pts',(-2.21311648827391,1.,3.29046159238343));
#45996=CARTESIAN_POINT('Ctrl Pts',(-2.21509406923368,-1.,3.29776825193159));
#45997=CARTESIAN_POINT('Ctrl Pts',(-2.21509406923368,1.,3.29776825193159));
#45998=CARTESIAN_POINT('Ctrl Pts',(-2.21703059947836,-1.,3.30509487819569));
#45999=CARTESIAN_POINT('Ctrl Pts',(-2.21703059947836,1.,3.30509487819569));
#46000=CARTESIAN_POINT('Ctrl Pts',(-2.21892881679086,-1.,3.31244421655666));
#46001=CARTESIAN_POINT('Ctrl Pts',(-2.21892881679086,1.,3.31244421655666));
#46002=CARTESIAN_POINT('Ctrl Pts',(-2.22078990842776,-1.,3.31981686778022));
#46003=CARTESIAN_POINT('Ctrl Pts',(-2.22078990842776,1.,3.31981686778022));
#46004=CARTESIAN_POINT('Ctrl Pts',(-2.22261398879635,-1.,3.3272119632604));
#46005=CARTESIAN_POINT('Ctrl Pts',(-2.22261398879635,1.,3.3272119632604));
#46006=CARTESIAN_POINT('Ctrl Pts',(-2.22440049878511,-1.,3.33462772849598));
#46007=CARTESIAN_POINT('Ctrl Pts',(-2.22440049878511,1.,3.33462772849598));
#46008=CARTESIAN_POINT('Ctrl Pts',(-2.22614863918047,-1.,3.34206209449375));
#46009=CARTESIAN_POINT('Ctrl Pts',(-2.22614863918047,1.,3.34206209449375));
#46010=CARTESIAN_POINT('Ctrl Pts',(-2.22785777756576,-1.,3.34951327111096));
#46011=CARTESIAN_POINT('Ctrl Pts',(-2.22785777756576,1.,3.34951327111096));
#46012=CARTESIAN_POINT('Ctrl Pts',(-2.22952789880982,-1.,3.35698038165483));
#46013=CARTESIAN_POINT('Ctrl Pts',(-2.22952789880982,1.,3.35698038165483));
#46014=CARTESIAN_POINT('Ctrl Pts',(-2.23115945849739,-1.,3.36446325227848));
#46015=CARTESIAN_POINT('Ctrl Pts',(-2.23115945849739,1.,3.36446325227848));
#46016=CARTESIAN_POINT('Ctrl Pts',(-2.23275319569221,-1.,3.37196214349304));
#46017=CARTESIAN_POINT('Ctrl Pts',(-2.23275319569221,1.,3.37196214349304));
#46018=CARTESIAN_POINT('Ctrl Pts',(-2.23430995599561,-1.,3.37947749555632));
#46019=CARTESIAN_POINT('Ctrl Pts',(-2.23430995599561,1.,3.37947749555632));
#46020=CARTESIAN_POINT('Ctrl Pts',(-2.23583052276308,-1.,3.38700968549563));
#46021=CARTESIAN_POINT('Ctrl Pts',(-2.23583052276308,1.,3.38700968549563));
#46022=CARTESIAN_POINT('Ctrl Pts',(-2.23731541452791,-1.,3.39455873448189));
#46023=CARTESIAN_POINT('Ctrl Pts',(-2.23731541452791,1.,3.39455873448189));
#46024=CARTESIAN_POINT('Ctrl Pts',(-2.2387649112415,-1.,3.40212434705647));
#46025=CARTESIAN_POINT('Ctrl Pts',(-2.2387649112415,1.,3.40212434705647));
#46026=CARTESIAN_POINT('Ctrl Pts',(-2.24017914395289,-1.,3.40970604190328));
#46027=CARTESIAN_POINT('Ctrl Pts',(-2.24017914395289,1.,3.40970604190328));
#46028=CARTESIAN_POINT('Ctrl Pts',(-2.24155816587844,-1.,3.41730325539172));
#46029=CARTESIAN_POINT('Ctrl Pts',(-2.24155816587844,1.,3.41730325539172));
#46030=CARTESIAN_POINT('Ctrl Pts',(-2.24290202531101,-1.,3.42491544683008));
#46031=CARTESIAN_POINT('Ctrl Pts',(-2.24290202531101,1.,3.42491544683008));
#46032=CARTESIAN_POINT('Ctrl Pts',(-2.24421085338727,-1.,3.43254222614803));
#46033=CARTESIAN_POINT('Ctrl Pts',(-2.24421085338727,1.,3.43254222614803));
#46034=CARTESIAN_POINT('Ctrl Pts',(-2.24548487526022,-1.,3.4401833646032));
#46035=CARTESIAN_POINT('Ctrl Pts',(-2.24548487526022,1.,3.4401833646032));
#46036=CARTESIAN_POINT('Ctrl Pts',(-2.2467243706995,-1.,3.44783872863151));
#46037=CARTESIAN_POINT('Ctrl Pts',(-2.2467243706995,1.,3.44783872863151));
#46038=CARTESIAN_POINT('Ctrl Pts',(-2.2479296496077,-1.,3.45550823512049));
#46039=CARTESIAN_POINT('Ctrl Pts',(-2.2479296496077,1.,3.45550823512049));
#46040=CARTESIAN_POINT('Ctrl Pts',(-2.2491010234604,-1.,3.46319180177573));
#46041=CARTESIAN_POINT('Ctrl Pts',(-2.2491010234604,1.,3.46319180177573));
#46042=CARTESIAN_POINT('Ctrl Pts',(-2.25023877475942,-1.,3.47088928979888));
#46043=CARTESIAN_POINT('Ctrl Pts',(-2.25023877475942,1.,3.47088928979888));
#46044=CARTESIAN_POINT('Ctrl Pts',(-2.25134314238687,-1.,3.47860048448691));
#46045=CARTESIAN_POINT('Ctrl Pts',(-2.25134314238687,1.,3.47860048448691));
#46046=CARTESIAN_POINT('Ctrl Pts',(-2.25241433138695,-1.,3.48632513240961));
#46047=CARTESIAN_POINT('Ctrl Pts',(-2.25241433138695,1.,3.48632513240961));
#46048=CARTESIAN_POINT('Ctrl Pts',(-2.2534525170976,-1.,3.49406296494791));
#46049=CARTESIAN_POINT('Ctrl Pts',(-2.2534525170976,1.,3.49406296494791));
#46050=CARTESIAN_POINT('Ctrl Pts',(-2.25445785151868,-1.,3.50181372617971));
#46051=CARTESIAN_POINT('Ctrl Pts',(-2.25445785151868,1.,3.50181372617971));
#46052=CARTESIAN_POINT('Ctrl Pts',(-2.25543046979799,-1.,3.50957720117341));
#46053=CARTESIAN_POINT('Ctrl Pts',(-2.25543046979799,1.,3.50957720117341));
#46054=CARTESIAN_POINT('Ctrl Pts',(-2.25637049455044,-1.,3.51735323667612));
#46055=CARTESIAN_POINT('Ctrl Pts',(-2.25637049455044,1.,3.51735323667612));
#46056=CARTESIAN_POINT('Ctrl Pts',(-2.25727802940898,-1.,3.52514172847711));
#46057=CARTESIAN_POINT('Ctrl Pts',(-2.25727802940898,1.,3.52514172847711));
#46058=CARTESIAN_POINT('Ctrl Pts',(-2.25797812950104,-1.,3.53138243688262));
#46059=CARTESIAN_POINT('Ctrl Pts',(-2.25797812950104,1.,3.53138243688262));
#46060=CARTESIAN_POINT('Ctrl Pts',(-2.25848864343951,-1.,3.53606853162228));
#46061=CARTESIAN_POINT('Ctrl Pts',(-2.25848864343951,1.,3.53606853162228));
#46062=CARTESIAN_POINT('Ctrl Pts',(-2.2588225169468,-1.,3.53919506647335));
#46063=CARTESIAN_POINT('Ctrl Pts',(-2.2588225169468,1.,3.53919506647335));
#46064=CARTESIAN_POINT('Ctrl Pts',(-2.25898783642071,-1.,3.54075895182139));
#46065=CARTESIAN_POINT('Ctrl Pts',(-2.25898783642071,1.,3.54075895182139));
#46066=CARTESIAN_POINT('',(-2.1297112484669,1.,3.08655633322212));
#46067=CARTESIAN_POINT('Ctrl Pts',(-2.1297112484669,-1.,3.08655633322212));
#46068=CARTESIAN_POINT('Ctrl Pts',(-2.1297112484669,-0.666666666666667,
3.08655633322212));
#46069=CARTESIAN_POINT('Ctrl Pts',(-2.1297112484669,-0.333333333333333,
3.08655633322212));
#46070=CARTESIAN_POINT('Ctrl Pts',(-2.1297112484669,0.333333333333333,3.08655633322212));
#46071=CARTESIAN_POINT('Ctrl Pts',(-2.1297112484669,0.666666666666667,3.08655633322212));
#46072=CARTESIAN_POINT('Ctrl Pts',(-2.1297112484669,1.,3.08655633322212));
#46073=CARTESIAN_POINT('',(-2.25898783642071,1.,3.54075895182139));
#46074=CARTESIAN_POINT('',(-2.25898783642071,0.,3.54075895182139));
#46075=CARTESIAN_POINT('Ctrl Pts',(-2.1297112484669,1.,3.08655633322211));
#46076=CARTESIAN_POINT('Ctrl Pts',(-2.1297578506149,1.,3.08657131089497));
#46077=CARTESIAN_POINT('Ctrl Pts',(-2.12991938762374,1.,3.08668447250322));
#46078=CARTESIAN_POINT('Ctrl Pts',(-2.13034980480424,1.,3.08717896996098));
#46079=CARTESIAN_POINT('Ctrl Pts',(-2.13132142793017,1.,3.08855597949761));
#46080=CARTESIAN_POINT('Ctrl Pts',(-2.13321032560893,1.,3.09151235281963));
#46081=CARTESIAN_POINT('Ctrl Pts',(-2.13596538661048,1.,3.0960450242104));
#46082=CARTESIAN_POINT('Ctrl Pts',(-2.13930228863751,1.,3.10171267391049));
#46083=CARTESIAN_POINT('Ctrl Pts',(-2.14302815601973,1.,3.10821808668859));
#46084=CARTESIAN_POINT('Ctrl Pts',(-2.14692798457532,1.,3.11522827016855));
#46085=CARTESIAN_POINT('Ctrl Pts',(-2.15079698090585,1.,3.12242318151938));
#46086=CARTESIAN_POINT('Ctrl Pts',(-2.1544724138292,1.,3.12954386795646));
#46087=CARTESIAN_POINT('Ctrl Pts',(-2.15787423530676,1.,3.13645356563038));
#46088=CARTESIAN_POINT('Ctrl Pts',(-2.16100905914435,1.,3.14314440427022));
#46089=CARTESIAN_POINT('Ctrl Pts',(-2.16393520288072,1.,3.14968624389054));
#46090=CARTESIAN_POINT('Ctrl Pts',(-2.1667372844769,1.,3.15618975593656));
#46091=CARTESIAN_POINT('Ctrl Pts',(-2.16949910801219,1.,3.16276685102972));
#46092=CARTESIAN_POINT('Ctrl Pts',(-2.17227212063817,1.,3.16948480019497));
#46093=CARTESIAN_POINT('Ctrl Pts',(-2.17506466903694,1.,3.17635032802523));
#46094=CARTESIAN_POINT('Ctrl Pts',(-2.17785968847142,1.,3.18333474627807));
#46095=CARTESIAN_POINT('Ctrl Pts',(-2.18062558031778,1.,3.19038924261573));
#46096=CARTESIAN_POINT('Ctrl Pts',(-2.18332898656602,1.,3.19746293740411));
#46097=CARTESIAN_POINT('Ctrl Pts',(-2.18594876115934,1.,3.20452259717976));
#46098=CARTESIAN_POINT('Ctrl Pts',(-2.18848253363901,1.,3.21156188355769));
#46099=CARTESIAN_POINT('Ctrl Pts',(-2.19093901948667,1.,3.21859043114095));
#46100=CARTESIAN_POINT('Ctrl Pts',(-2.19333345123538,1.,3.22562734221646));
#46101=CARTESIAN_POINT('Ctrl Pts',(-2.19568204933168,1.,3.23269332296933));
#46102=CARTESIAN_POINT('Ctrl Pts',(-2.19799623693253,1.,3.23980245361308));
#46103=CARTESIAN_POINT('Ctrl Pts',(-2.20027910880981,1.,3.24695715874338));
#46104=CARTESIAN_POINT('Ctrl Pts',(-2.20252866491545,1.,3.25415277957775));
#46105=CARTESIAN_POINT('Ctrl Pts',(-2.20473979048678,1.,3.26138036637705));
#46106=CARTESIAN_POINT('Ctrl Pts',(-2.20690665217743,1.,3.26863006136782));
#46107=CARTESIAN_POINT('Ctrl Pts',(-2.2090250941743,1.,3.2758944800554));
#46108=CARTESIAN_POINT('Ctrl Pts',(-2.21109449750641,1.,3.28317133333131));
#46109=CARTESIAN_POINT('Ctrl Pts',(-2.21311648827391,1.,3.29046159238343));
#46110=CARTESIAN_POINT('Ctrl Pts',(-2.21509406923368,1.,3.29776825193159));
#46111=CARTESIAN_POINT('Ctrl Pts',(-2.21703059947836,1.,3.30509487819569));
#46112=CARTESIAN_POINT('Ctrl Pts',(-2.21892881679086,1.,3.31244421655666));
#46113=CARTESIAN_POINT('Ctrl Pts',(-2.22078990842776,1.,3.31981686778022));
#46114=CARTESIAN_POINT('Ctrl Pts',(-2.22261398879635,1.,3.3272119632604));
#46115=CARTESIAN_POINT('Ctrl Pts',(-2.22440049878511,1.,3.33462772849598));
#46116=CARTESIAN_POINT('Ctrl Pts',(-2.22614863918047,1.,3.34206209449375));
#46117=CARTESIAN_POINT('Ctrl Pts',(-2.22785777756576,1.,3.34951327111096));
#46118=CARTESIAN_POINT('Ctrl Pts',(-2.22952789880982,1.,3.35698038165483));
#46119=CARTESIAN_POINT('Ctrl Pts',(-2.23115945849739,1.,3.36446325227848));
#46120=CARTESIAN_POINT('Ctrl Pts',(-2.23275319569221,1.,3.37196214349304));
#46121=CARTESIAN_POINT('Ctrl Pts',(-2.23430995599561,1.,3.37947749555632));
#46122=CARTESIAN_POINT('Ctrl Pts',(-2.23583052276308,1.,3.38700968549563));
#46123=CARTESIAN_POINT('Ctrl Pts',(-2.23731541452791,1.,3.39455873448189));
#46124=CARTESIAN_POINT('Ctrl Pts',(-2.2387649112415,1.,3.40212434705647));
#46125=CARTESIAN_POINT('Ctrl Pts',(-2.24017914395289,1.,3.40970604190328));
#46126=CARTESIAN_POINT('Ctrl Pts',(-2.24155816587844,1.,3.41730325539172));
#46127=CARTESIAN_POINT('Ctrl Pts',(-2.24290202531101,1.,3.42491544683008));
#46128=CARTESIAN_POINT('Ctrl Pts',(-2.24421085338727,1.,3.43254222614803));
#46129=CARTESIAN_POINT('Ctrl Pts',(-2.24548487526022,1.,3.4401833646032));
#46130=CARTESIAN_POINT('Ctrl Pts',(-2.2467243706995,1.,3.44783872863151));
#46131=CARTESIAN_POINT('Ctrl Pts',(-2.2479296496077,1.,3.45550823512049));
#46132=CARTESIAN_POINT('Ctrl Pts',(-2.2491010234604,1.,3.46319180177573));
#46133=CARTESIAN_POINT('Ctrl Pts',(-2.25023877475942,1.,3.47088928979888));
#46134=CARTESIAN_POINT('Ctrl Pts',(-2.25134314238687,1.,3.47860048448691));
#46135=CARTESIAN_POINT('Ctrl Pts',(-2.25241433138695,1.,3.48632513240961));
#46136=CARTESIAN_POINT('Ctrl Pts',(-2.2534525170976,1.,3.49406296494791));
#46137=CARTESIAN_POINT('Ctrl Pts',(-2.25445785151868,1.,3.50181372617971));
#46138=CARTESIAN_POINT('Ctrl Pts',(-2.25543046979799,1.,3.50957720117341));
#46139=CARTESIAN_POINT('Ctrl Pts',(-2.25637049455044,1.,3.51735323667612));
#46140=CARTESIAN_POINT('Ctrl Pts',(-2.25727802940898,1.,3.52514172847711));
#46141=CARTESIAN_POINT('Ctrl Pts',(-2.25797812950104,1.,3.53138243688262));
#46142=CARTESIAN_POINT('Ctrl Pts',(-2.25848864343951,1.,3.53606853162228));
#46143=CARTESIAN_POINT('Ctrl Pts',(-2.2588225169468,1.,3.53919506647335));
#46144=CARTESIAN_POINT('Ctrl Pts',(-2.25898783642071,1.,3.54075895182139));
#46145=CARTESIAN_POINT('Origin',(-2.25898783642071,0.,3.54075895182139));
#46146=CARTESIAN_POINT('',(-2.12928030988903,1.,3.62024382630768));
#46147=CARTESIAN_POINT('Origin',(0.,0.,0.));
#46148=CARTESIAN_POINT('',(-2.27737254473378,1.,2.97927412174388));
#46149=CARTESIAN_POINT('Origin',(0.,1.,0.));
#46150=CARTESIAN_POINT('Ctrl Pts',(-2.27737254473378,1.,2.97927412174388));
#46151=CARTESIAN_POINT('Ctrl Pts',(-2.27737254473378,0.666666666666667,
2.97927412174388));
#46152=CARTESIAN_POINT('Ctrl Pts',(-2.27737254473378,0.333333333333333,
2.97927412174388));
#46153=CARTESIAN_POINT('Ctrl Pts',(-2.27737254473378,-0.333333333333333,
2.97927412174388));
#46154=CARTESIAN_POINT('Ctrl Pts',(-2.27737254473378,-0.666666666666667,
2.97927412174388));
#46155=CARTESIAN_POINT('Ctrl Pts',(-2.27737254473378,-1.,2.97927412174388));
#46156=CARTESIAN_POINT('Ctrl Pts',(-2.66939624221984,-1.,3.24257979115744));
#46157=CARTESIAN_POINT('Ctrl Pts',(-2.66939624221984,1.,3.24257979115744));
#46158=CARTESIAN_POINT('Ctrl Pts',(-2.66795998539861,-1.,3.24193929584813));
#46159=CARTESIAN_POINT('Ctrl Pts',(-2.66795998539861,1.,3.24193929584813));
#46160=CARTESIAN_POINT('Ctrl Pts',(-2.66508964664767,-1.,3.24065561087681));
#46161=CARTESIAN_POINT('Ctrl Pts',(-2.66508964664767,1.,3.24065561087681));
#46162=CARTESIAN_POINT('Ctrl Pts',(-2.6607906631973,-1.,3.23872200036311));
#46163=CARTESIAN_POINT('Ctrl Pts',(-2.6607906631973,1.,3.23872200036311));
#46164=CARTESIAN_POINT('Ctrl Pts',(-2.6550717396303,-1.,3.23612768065687));
#46165=CARTESIAN_POINT('Ctrl Pts',(-2.6550717396303,1.,3.23612768065687));
#46166=CARTESIAN_POINT('Ctrl Pts',(-2.64794488744246,-1.,3.23285778738558));
#46167=CARTESIAN_POINT('Ctrl Pts',(-2.64794488744246,1.,3.23285778738558));
#46168=CARTESIAN_POINT('Ctrl Pts',(-2.64083992182478,-1.,3.2295608435934));
#46169=CARTESIAN_POINT('Ctrl Pts',(-2.64083992182478,1.,3.2295608435934));
#46170=CARTESIAN_POINT('Ctrl Pts',(-2.63375697391438,-1.,3.22623678292539));
#46171=CARTESIAN_POINT('Ctrl Pts',(-2.63375697391438,1.,3.22623678292539));
#46172=CARTESIAN_POINT('Ctrl Pts',(-2.62669622735548,-1.,3.222885536128));
#46173=CARTESIAN_POINT('Ctrl Pts',(-2.62669622735548,1.,3.222885536128));
#46174=CARTESIAN_POINT('Ctrl Pts',(-2.61965792832396,-1.,3.21950704108654));
#46175=CARTESIAN_POINT('Ctrl Pts',(-2.61965792832396,1.,3.21950704108654));
#46176=CARTESIAN_POINT('Ctrl Pts',(-2.61264236718662,-1.,3.21610123232465));
#46177=CARTESIAN_POINT('Ctrl Pts',(-2.61264236718662,1.,3.21610123232465));
#46178=CARTESIAN_POINT('Ctrl Pts',(-2.60564985359699,-1.,3.21266802609297));
#46179=CARTESIAN_POINT('Ctrl Pts',(-2.60564985359699,1.,3.21266802609297));
#46180=CARTESIAN_POINT('Ctrl Pts',(-2.59868069194267,-1.,3.2092073056959));
#46181=CARTESIAN_POINT('Ctrl Pts',(-2.59868069194267,1.,3.2092073056959));
#46182=CARTESIAN_POINT('Ctrl Pts',(-2.59173516023605,-1.,3.20571891028879));
#46183=CARTESIAN_POINT('Ctrl Pts',(-2.59173516023605,1.,3.20571891028879));
#46184=CARTESIAN_POINT('Ctrl Pts',(-2.58481347777953,-1.,3.20220261408685));
#46185=CARTESIAN_POINT('Ctrl Pts',(-2.58481347777953,1.,3.20220261408685));
#46186=CARTESIAN_POINT('Ctrl Pts',(-2.577915819091,-1.,3.19865814628955));
#46187=CARTESIAN_POINT('Ctrl Pts',(-2.577915819091,1.,3.19865814628955));
#46188=CARTESIAN_POINT('Ctrl Pts',(-2.57104235898053,-1.,3.19508523784548));
#46189=CARTESIAN_POINT('Ctrl Pts',(-2.57104235898053,1.,3.19508523784548));
#46190=CARTESIAN_POINT('Ctrl Pts',(-2.56419331092909,-1.,3.19148366395201));
#46191=CARTESIAN_POINT('Ctrl Pts',(-2.56419331092909,1.,3.19148366395201));
#46192=CARTESIAN_POINT('Ctrl Pts',(-2.55736896206016,-1.,3.1878532811617));
#46193=CARTESIAN_POINT('Ctrl Pts',(-2.55736896206016,1.,3.1878532811617));
#46194=CARTESIAN_POINT('Ctrl Pts',(-2.55056972387638,-1.,3.18419408529482));
#46195=CARTESIAN_POINT('Ctrl Pts',(-2.55056972387638,1.,3.18419408529482));
#46196=CARTESIAN_POINT('Ctrl Pts',(-2.54379612552948,-1.,3.18050619750515));
#46197=CARTESIAN_POINT('Ctrl Pts',(-2.54379612552948,1.,3.18050619750515));
#46198=CARTESIAN_POINT('Ctrl Pts',(-2.53704871950871,-1.,3.17678974135225));
#46199=CARTESIAN_POINT('Ctrl Pts',(-2.53704871950871,1.,3.17678974135225));
#46200=CARTESIAN_POINT('Ctrl Pts',(-2.5303280040691,-1.,3.17304474093574));
#46201=CARTESIAN_POINT('Ctrl Pts',(-2.5303280040691,1.,3.17304474093574));
#46202=CARTESIAN_POINT('Ctrl Pts',(-2.523634346718,-1.,3.16927102130751));
#46203=CARTESIAN_POINT('Ctrl Pts',(-2.523634346718,1.,3.16927102130751));
#46204=CARTESIAN_POINT('Ctrl Pts',(-2.51696788755616,-1.,3.16546808277069));
#46205=CARTESIAN_POINT('Ctrl Pts',(-2.51696788755616,1.,3.16546808277069));
#46206=CARTESIAN_POINT('Ctrl Pts',(-2.51032851007939,-1.,3.16163506380211));
#46207=CARTESIAN_POINT('Ctrl Pts',(-2.51032851007939,1.,3.16163506380211));
#46208=CARTESIAN_POINT('Ctrl Pts',(-2.50371605688287,-1.,3.15777102413998));
#46209=CARTESIAN_POINT('Ctrl Pts',(-2.50371605688287,1.,3.15777102413998));
#46210=CARTESIAN_POINT('Ctrl Pts',(-2.49713050858911,-1.,3.15387518039064));
#46211=CARTESIAN_POINT('Ctrl Pts',(-2.49713050858911,1.,3.15387518039064));
#46212=CARTESIAN_POINT('Ctrl Pts',(-2.49057217131985,-1.,3.14994715298903));
#46213=CARTESIAN_POINT('Ctrl Pts',(-2.49057217131985,1.,3.14994715298903));
#46214=CARTESIAN_POINT('Ctrl Pts',(-2.48404187418376,-1.,3.1459872272388));
#46215=CARTESIAN_POINT('Ctrl Pts',(-2.48404187418376,1.,3.1459872272388));
#46216=CARTESIAN_POINT('Ctrl Pts',(-2.47754112428028,-1.,3.14199655778845));
#46217=CARTESIAN_POINT('Ctrl Pts',(-2.47754112428028,1.,3.14199655778845));
#46218=CARTESIAN_POINT('Ctrl Pts',(-2.47107164236827,-1.,3.13797654408931));
#46219=CARTESIAN_POINT('Ctrl Pts',(-2.47107164236827,1.,3.13797654408931));
#46220=CARTESIAN_POINT('Ctrl Pts',(-2.4646349433237,-1.,3.13392826623902));
#46221=CARTESIAN_POINT('Ctrl Pts',(-2.4646349433237,1.,3.13392826623902));
#46222=CARTESIAN_POINT('Ctrl Pts',(-2.45823188859367,-1.,3.12985188384372));
#46223=CARTESIAN_POINT('Ctrl Pts',(-2.45823188859367,1.,3.12985188384372));
#46224=CARTESIAN_POINT('Ctrl Pts',(-2.45186227369848,-1.,3.12574608210849));
#46225=CARTESIAN_POINT('Ctrl Pts',(-2.45186227369848,1.,3.12574608210849));
#46226=CARTESIAN_POINT('Ctrl Pts',(-2.44552433364716,-1.,3.12160740887768));
#46227=CARTESIAN_POINT('Ctrl Pts',(-2.44552433364716,1.,3.12160740887768));
#46228=CARTESIAN_POINT('Ctrl Pts',(-2.43921571477975,-1.,3.11743156744182));
#46229=CARTESIAN_POINT('Ctrl Pts',(-2.43921571477975,1.,3.11743156744182));
#46230=CARTESIAN_POINT('Ctrl Pts',(-2.4329344968514,-1.,3.11321477659012));
#46231=CARTESIAN_POINT('Ctrl Pts',(-2.4329344968514,1.,3.11321477659012));
#46232=CARTESIAN_POINT('Ctrl Pts',(-2.42668025870013,-1.,3.10895518969592));
#46233=CARTESIAN_POINT('Ctrl Pts',(-2.42668025870013,1.,3.10895518969592));
#46234=CARTESIAN_POINT('Ctrl Pts',(-2.42045498612494,-1.,3.10465410280902));
#46235=CARTESIAN_POINT('Ctrl Pts',(-2.42045498612494,1.,3.10465410280902));
#46236=CARTESIAN_POINT('Ctrl Pts',(-2.41426441798067,-1.,3.10031775027683));
#46237=CARTESIAN_POINT('Ctrl Pts',(-2.41426441798067,1.,3.10031775027683));
#46238=CARTESIAN_POINT('Ctrl Pts',(-2.40811612696382,-1.,3.09595472616093));
#46239=CARTESIAN_POINT('Ctrl Pts',(-2.40811612696382,1.,3.09595472616093));
#46240=CARTESIAN_POINT('Ctrl Pts',(-2.40201704423352,-1.,3.09157266051115));
#46241=CARTESIAN_POINT('Ctrl Pts',(-2.40201704423352,1.,3.09157266051115));
#46242=CARTESIAN_POINT('Ctrl Pts',(-2.39597098250635,-1.,3.08717489512919));
#46243=CARTESIAN_POINT('Ctrl Pts',(-2.39597098250635,1.,3.08717489512919));
#46244=CARTESIAN_POINT('Ctrl Pts',(-2.38997659219192,-1.,3.08275773747083));
#46245=CARTESIAN_POINT('Ctrl Pts',(-2.38997659219192,1.,3.08275773747083));
#46246=CARTESIAN_POINT('Ctrl Pts',(-2.38402401216107,-1.,3.07830597244301));
#46247=CARTESIAN_POINT('Ctrl Pts',(-2.38402401216107,1.,3.07830597244301));
#46248=CARTESIAN_POINT('Ctrl Pts',(-2.37809856205524,-1.,3.07379777492133));
#46249=CARTESIAN_POINT('Ctrl Pts',(-2.37809856205524,1.,3.07379777492133));
#46250=CARTESIAN_POINT('Ctrl Pts',(-2.37218678163157,-1.,3.06921275497472));
#46251=CARTESIAN_POINT('Ctrl Pts',(-2.37218678163157,1.,3.06921275497472));
#46252=CARTESIAN_POINT('Ctrl Pts',(-2.36628220107001,-1.,3.06453964643152));
#46253=CARTESIAN_POINT('Ctrl Pts',(-2.36628220107001,1.,3.06453964643152));
#46254=CARTESIAN_POINT('Ctrl Pts',(-2.36039011602084,-1.,3.05978266240056));
#46255=CARTESIAN_POINT('Ctrl Pts',(-2.36039011602084,1.,3.05978266240056));
#46256=CARTESIAN_POINT('Ctrl Pts',(-2.35453559889506,-1.,3.05497218368188));
#46257=CARTESIAN_POINT('Ctrl Pts',(-2.35453559889506,1.,3.05497218368188));
#46258=CARTESIAN_POINT('Ctrl Pts',(-2.34875673090816,-1.,3.05015565829976));
#46259=CARTESIAN_POINT('Ctrl Pts',(-2.34875673090816,1.,3.05015565829976));
#46260=CARTESIAN_POINT('Ctrl Pts',(-2.3430901708402,-1.,3.04537822217311));
#46261=CARTESIAN_POINT('Ctrl Pts',(-2.3430901708402,1.,3.04537822217311));
#46262=CARTESIAN_POINT('Ctrl Pts',(-2.33755792953726,-1.,3.04066496998569));
#46263=CARTESIAN_POINT('Ctrl Pts',(-2.33755792953726,1.,3.04066496998569));
#46264=CARTESIAN_POINT('Ctrl Pts',(-2.33215619079807,-1.,3.03600588555765));
#46265=CARTESIAN_POINT('Ctrl Pts',(-2.33215619079807,1.,3.03600588555765));
#46266=CARTESIAN_POINT('Ctrl Pts',(-2.32683687412027,-1.,3.03133125185047));
#46267=CARTESIAN_POINT('Ctrl Pts',(-2.32683687412027,1.,3.03133125185047));
#46268=CARTESIAN_POINT('Ctrl Pts',(-2.32151944306299,-1.,3.02652678416478));
#46269=CARTESIAN_POINT('Ctrl Pts',(-2.32151944306299,1.,3.02652678416478));
#46270=CARTESIAN_POINT('Ctrl Pts',(-2.31612479121528,-1.,3.02147780668029));
#46271=CARTESIAN_POINT('Ctrl Pts',(-2.31612479121528,1.,3.02147780668029));
#46272=CARTESIAN_POINT('Ctrl Pts',(-2.31060449886577,-1.,3.01610726819019));
#46273=CARTESIAN_POINT('Ctrl Pts',(-2.31060449886577,1.,3.01610726819019));
#46274=CARTESIAN_POINT('Ctrl Pts',(-2.30496809486529,-1.,3.01041131063882));
#46275=CARTESIAN_POINT('Ctrl Pts',(-2.30496809486529,1.,3.01041131063882));
#46276=CARTESIAN_POINT('Ctrl Pts',(-2.29932091315939,-1.,3.00450832658822));
#46277=CARTESIAN_POINT('Ctrl Pts',(-2.29932091315939,1.,3.00450832658822));
#46278=CARTESIAN_POINT('Ctrl Pts',(-2.29385894577999,-1.,2.99863310340004));
#46279=CARTESIAN_POINT('Ctrl Pts',(-2.29385894577999,1.,2.99863310340004));
#46280=CARTESIAN_POINT('Ctrl Pts',(-2.28882328690601,-1.,2.9930793098434));
#46281=CARTESIAN_POINT('Ctrl Pts',(-2.28882328690601,1.,2.9930793098434));
#46282=CARTESIAN_POINT('Ctrl Pts',(-2.28446419116036,-1.,2.98815432734929));
#46283=CARTESIAN_POINT('Ctrl Pts',(-2.28446419116036,1.,2.98815432734929));
#46284=CARTESIAN_POINT('Ctrl Pts',(-2.28100472516582,-1.,2.98413343613858));
#46285=CARTESIAN_POINT('Ctrl Pts',(-2.28100472516582,1.,2.98413343613858));
#46286=CARTESIAN_POINT('Ctrl Pts',(-2.2785960133424,-1.,2.98120357932601));
#46287=CARTESIAN_POINT('Ctrl Pts',(-2.2785960133424,1.,2.98120357932601));
#46288=CARTESIAN_POINT('Ctrl Pts',(-2.27756633754846,-1.,2.97980276182744));
#46289=CARTESIAN_POINT('Ctrl Pts',(-2.27756633754846,1.,2.97980276182744));
#46290=CARTESIAN_POINT('Ctrl Pts',(-2.27730961189188,-1.,2.97929608861502));
#46291=CARTESIAN_POINT('Ctrl Pts',(-2.27730961189188,1.,2.97929608861502));
#46292=CARTESIAN_POINT('Ctrl Pts',(-2.2773674298423,-1.,2.97919987915565));
#46293=CARTESIAN_POINT('Ctrl Pts',(-2.2773674298423,1.,2.97919987915565));
#46294=CARTESIAN_POINT('Ctrl Pts',(-2.27745358485296,-1.,2.97921217251145));
#46295=CARTESIAN_POINT('Ctrl Pts',(-2.27745358485296,1.,2.97921217251145));
#46296=CARTESIAN_POINT('',(-2.66939624221984,1.,3.24257979115744));
#46297=CARTESIAN_POINT('Ctrl Pts',(-2.66939624221984,1.,3.24257979115744));
#46298=CARTESIAN_POINT('Ctrl Pts',(-2.66795998539861,1.,3.24193929584813));
#46299=CARTESIAN_POINT('Ctrl Pts',(-2.66508964664767,1.,3.24065561087681));
#46300=CARTESIAN_POINT('Ctrl Pts',(-2.6607906631973,1.,3.23872200036311));
#46301=CARTESIAN_POINT('Ctrl Pts',(-2.6550717396303,1.,3.23612768065687));
#46302=CARTESIAN_POINT('Ctrl Pts',(-2.64794488744246,1.,3.23285778738558));
#46303=CARTESIAN_POINT('Ctrl Pts',(-2.64083992182478,1.,3.2295608435934));
#46304=CARTESIAN_POINT('Ctrl Pts',(-2.63375697391438,1.,3.22623678292539));
#46305=CARTESIAN_POINT('Ctrl Pts',(-2.62669622735548,1.,3.222885536128));
#46306=CARTESIAN_POINT('Ctrl Pts',(-2.61965792832396,1.,3.21950704108654));
#46307=CARTESIAN_POINT('Ctrl Pts',(-2.61264236718662,1.,3.21610123232465));
#46308=CARTESIAN_POINT('Ctrl Pts',(-2.60564985359699,1.,3.21266802609297));
#46309=CARTESIAN_POINT('Ctrl Pts',(-2.59868069194267,1.,3.2092073056959));
#46310=CARTESIAN_POINT('Ctrl Pts',(-2.59173516023605,1.,3.20571891028879));
#46311=CARTESIAN_POINT('Ctrl Pts',(-2.58481347777953,1.,3.20220261408685));
#46312=CARTESIAN_POINT('Ctrl Pts',(-2.577915819091,1.,3.19865814628955));
#46313=CARTESIAN_POINT('Ctrl Pts',(-2.57104235898053,1.,3.19508523784548));
#46314=CARTESIAN_POINT('Ctrl Pts',(-2.56419331092909,1.,3.19148366395201));
#46315=CARTESIAN_POINT('Ctrl Pts',(-2.55736896206016,1.,3.1878532811617));
#46316=CARTESIAN_POINT('Ctrl Pts',(-2.55056972387638,1.,3.18419408529482));
#46317=CARTESIAN_POINT('Ctrl Pts',(-2.54379612552948,1.,3.18050619750515));
#46318=CARTESIAN_POINT('Ctrl Pts',(-2.53704871950871,1.,3.17678974135225));
#46319=CARTESIAN_POINT('Ctrl Pts',(-2.5303280040691,1.,3.17304474093574));
#46320=CARTESIAN_POINT('Ctrl Pts',(-2.523634346718,1.,3.16927102130751));
#46321=CARTESIAN_POINT('Ctrl Pts',(-2.51696788755616,1.,3.16546808277069));
#46322=CARTESIAN_POINT('Ctrl Pts',(-2.51032851007939,1.,3.16163506380211));
#46323=CARTESIAN_POINT('Ctrl Pts',(-2.50371605688287,1.,3.15777102413998));
#46324=CARTESIAN_POINT('Ctrl Pts',(-2.49713050858911,1.,3.15387518039064));
#46325=CARTESIAN_POINT('Ctrl Pts',(-2.49057217131985,1.,3.14994715298903));
#46326=CARTESIAN_POINT('Ctrl Pts',(-2.48404187418376,1.,3.1459872272388));
#46327=CARTESIAN_POINT('Ctrl Pts',(-2.47754112428028,1.,3.14199655778845));
#46328=CARTESIAN_POINT('Ctrl Pts',(-2.47107164236827,1.,3.13797654408931));
#46329=CARTESIAN_POINT('Ctrl Pts',(-2.4646349433237,1.,3.13392826623902));
#46330=CARTESIAN_POINT('Ctrl Pts',(-2.45823188859367,1.,3.12985188384372));
#46331=CARTESIAN_POINT('Ctrl Pts',(-2.45186227369848,1.,3.12574608210849));
#46332=CARTESIAN_POINT('Ctrl Pts',(-2.44552433364716,1.,3.12160740887768));
#46333=CARTESIAN_POINT('Ctrl Pts',(-2.43921571477975,1.,3.11743156744182));
#46334=CARTESIAN_POINT('Ctrl Pts',(-2.4329344968514,1.,3.11321477659012));
#46335=CARTESIAN_POINT('Ctrl Pts',(-2.42668025870013,1.,3.10895518969592));
#46336=CARTESIAN_POINT('Ctrl Pts',(-2.42045498612494,1.,3.10465410280902));
#46337=CARTESIAN_POINT('Ctrl Pts',(-2.41426441798067,1.,3.10031775027683));
#46338=CARTESIAN_POINT('Ctrl Pts',(-2.40811612696382,1.,3.09595472616093));
#46339=CARTESIAN_POINT('Ctrl Pts',(-2.40201704423352,1.,3.09157266051115));
#46340=CARTESIAN_POINT('Ctrl Pts',(-2.39597098250635,1.,3.08717489512919));
#46341=CARTESIAN_POINT('Ctrl Pts',(-2.38997659219192,1.,3.08275773747083));
#46342=CARTESIAN_POINT('Ctrl Pts',(-2.38402401216107,1.,3.07830597244301));
#46343=CARTESIAN_POINT('Ctrl Pts',(-2.37809856205524,1.,3.07379777492133));
#46344=CARTESIAN_POINT('Ctrl Pts',(-2.37218678163157,1.,3.06921275497472));
#46345=CARTESIAN_POINT('Ctrl Pts',(-2.36628220107001,1.,3.06453964643152));
#46346=CARTESIAN_POINT('Ctrl Pts',(-2.36039011602084,1.,3.05978266240056));
#46347=CARTESIAN_POINT('Ctrl Pts',(-2.35453559889506,1.,3.05497218368188));
#46348=CARTESIAN_POINT('Ctrl Pts',(-2.34875673090816,1.,3.05015565829976));
#46349=CARTESIAN_POINT('Ctrl Pts',(-2.3430901708402,1.,3.04537822217311));
#46350=CARTESIAN_POINT('Ctrl Pts',(-2.33755792953726,1.,3.04066496998569));
#46351=CARTESIAN_POINT('Ctrl Pts',(-2.33215619079807,1.,3.03600588555765));
#46352=CARTESIAN_POINT('Ctrl Pts',(-2.32683687412027,1.,3.03133125185047));
#46353=CARTESIAN_POINT('Ctrl Pts',(-2.32151944306299,1.,3.02652678416478));
#46354=CARTESIAN_POINT('Ctrl Pts',(-2.31612479121528,1.,3.02147780668029));
#46355=CARTESIAN_POINT('Ctrl Pts',(-2.31060449886577,1.,3.01610726819019));
#46356=CARTESIAN_POINT('Ctrl Pts',(-2.30496809486529,1.,3.01041131063882));
#46357=CARTESIAN_POINT('Ctrl Pts',(-2.29932091315939,1.,3.00450832658822));
#46358=CARTESIAN_POINT('Ctrl Pts',(-2.29385894577999,1.,2.99863310340004));
#46359=CARTESIAN_POINT('Ctrl Pts',(-2.28882328690601,1.,2.9930793098434));
#46360=CARTESIAN_POINT('Ctrl Pts',(-2.28446419116036,1.,2.98815432734929));
#46361=CARTESIAN_POINT('Ctrl Pts',(-2.28100472516582,1.,2.98413343613858));
#46362=CARTESIAN_POINT('Ctrl Pts',(-2.27877674853833,1.,2.98142341809623));
#46363=CARTESIAN_POINT('Ctrl Pts',(-2.27776738270369,1.,2.98007383024333));
#46364=CARTESIAN_POINT('Ctrl Pts',(-2.27743009389704,1.,2.97951167106106));
#46365=CARTESIAN_POINT('Ctrl Pts',(-2.27737238849212,1.,2.97932307137589));
#46366=CARTESIAN_POINT('Ctrl Pts',(-2.27737254473378,1.,2.97927412174388));
#46367=CARTESIAN_POINT('',(-2.66939624221984,0.,3.24257979115744));
#46368=CARTESIAN_POINT('Ctrl Pts',(-2.58626089374824,-1.,2.71546581445404));
#46369=CARTESIAN_POINT('Ctrl Pts',(-2.58626089374824,1.,2.71546581445404));
#46370=CARTESIAN_POINT('Ctrl Pts',(-2.58626222935804,-1.,2.71537879705104));
#46371=CARTESIAN_POINT('Ctrl Pts',(-2.58626222935804,1.,2.71537879705104));
#46372=CARTESIAN_POINT('Ctrl Pts',(-2.58636629904103,-1.,2.71533674141254));
#46373=CARTESIAN_POINT('Ctrl Pts',(-2.58636629904103,1.,2.71533674141254));
#46374=CARTESIAN_POINT('Ctrl Pts',(-2.5868265735259,-1.,2.71566956750452));
#46375=CARTESIAN_POINT('Ctrl Pts',(-2.5868265735259,1.,2.71566956750452));
#46376=CARTESIAN_POINT('Ctrl Pts',(-2.58804906785417,-1.,2.71690570241638));
#46377=CARTESIAN_POINT('Ctrl Pts',(-2.58804906785417,1.,2.71690570241638));
#46378=CARTESIAN_POINT('Ctrl Pts',(-2.59056604771971,-1.,2.71974308958086));
#46379=CARTESIAN_POINT('Ctrl Pts',(-2.59056604771971,1.,2.71974308958086));
#46380=CARTESIAN_POINT('Ctrl Pts',(-2.59399625537278,-1.,2.72378896977134));
#46381=CARTESIAN_POINT('Ctrl Pts',(-2.59399625537278,1.,2.72378896977134));
#46382=CARTESIAN_POINT('Ctrl Pts',(-2.59817869034746,-1.,2.7288648348152));
#46383=CARTESIAN_POINT('Ctrl Pts',(-2.59817869034746,1.,2.7288648348152));
#46384=CARTESIAN_POINT('Ctrl Pts',(-2.60287635688728,-1.,2.73470730109615));
#46385=CARTESIAN_POINT('Ctrl Pts',(-2.60287635688728,1.,2.73470730109615));
#46386=CARTESIAN_POINT('Ctrl Pts',(-2.60782480638448,-1.,2.7410211099909));
#46387=CARTESIAN_POINT('Ctrl Pts',(-2.60782480638448,1.,2.7410211099909));
#46388=CARTESIAN_POINT('Ctrl Pts',(-2.61277170105813,-1.,2.74752219567252));
#46389=CARTESIAN_POINT('Ctrl Pts',(-2.61277170105813,1.,2.74752219567252));
#46390=CARTESIAN_POINT('Ctrl Pts',(-2.61751580407667,-1.,2.7539802502603));
#46391=CARTESIAN_POINT('Ctrl Pts',(-2.61751580407667,1.,2.7539802502603));
#46392=CARTESIAN_POINT('Ctrl Pts',(-2.62195665834605,-1.,2.76027271596686));
#46393=CARTESIAN_POINT('Ctrl Pts',(-2.62195665834605,1.,2.76027271596686));
#46394=CARTESIAN_POINT('Ctrl Pts',(-2.62609956506355,-1.,2.76639078479021));
#46395=CARTESIAN_POINT('Ctrl Pts',(-2.62609956506355,1.,2.76639078479021));
#46396=CARTESIAN_POINT('Ctrl Pts',(-2.63001305229625,-1.,2.77239433377921));
#46397=CARTESIAN_POINT('Ctrl Pts',(-2.63001305229625,1.,2.77239433377921));
#46398=CARTESIAN_POINT('Ctrl Pts',(-2.63379800904599,-1.,2.77837943466449));
#46399=CARTESIAN_POINT('Ctrl Pts',(-2.63379800904599,1.,2.77837943466449));
#46400=CARTESIAN_POINT('Ctrl Pts',(-2.637554714303,-1.,2.78444351041571));
#46401=CARTESIAN_POINT('Ctrl Pts',(-2.637554714303,1.,2.78444351041571));
#46402=CARTESIAN_POINT('Ctrl Pts',(-2.64134450532584,-1.,2.79064495573224));
#46403=CARTESIAN_POINT('Ctrl Pts',(-2.64134450532584,1.,2.79064495573224));
#46404=CARTESIAN_POINT('Ctrl Pts',(-2.6451766779932,-1.,2.79698910670736));
#46405=CARTESIAN_POINT('Ctrl Pts',(-2.6451766779932,1.,2.79698910670736));
#46406=CARTESIAN_POINT('Ctrl Pts',(-2.64902988983337,-1.,2.80345029781152));
#46407=CARTESIAN_POINT('Ctrl Pts',(-2.64902988983337,1.,2.80345029781152));
#46408=CARTESIAN_POINT('Ctrl Pts',(-2.65286529532208,-1.,2.80998526078165));
#46409=CARTESIAN_POINT('Ctrl Pts',(-2.65286529532208,1.,2.80998526078165));
#46410=CARTESIAN_POINT('Ctrl Pts',(-2.65664198781344,-1.,2.81654896073883));
#46411=CARTESIAN_POINT('Ctrl Pts',(-2.65664198781344,1.,2.81654896073883));
#46412=CARTESIAN_POINT('Ctrl Pts',(-2.66033388273461,-1.,2.82311188135078));
#46413=CARTESIAN_POINT('Ctrl Pts',(-2.66033388273461,1.,2.82311188135078));
#46414=CARTESIAN_POINT('Ctrl Pts',(-2.6639376472693,-1.,2.82966813308998));
#46415=CARTESIAN_POINT('Ctrl Pts',(-2.6639376472693,1.,2.82966813308998));
#46416=CARTESIAN_POINT('Ctrl Pts',(-2.66746339678107,-1.,2.83622586853982));
#46417=CARTESIAN_POINT('Ctrl Pts',(-2.66746339678107,1.,2.83622586853982));
#46418=CARTESIAN_POINT('Ctrl Pts',(-2.67092916452125,-1.,2.84280157191323));
#46419=CARTESIAN_POINT('Ctrl Pts',(-2.67092916452125,1.,2.84280157191323));
#46420=CARTESIAN_POINT('Ctrl Pts',(-2.67435421039677,-1.,2.84941315703092));
#46421=CARTESIAN_POINT('Ctrl Pts',(-2.67435421039677,1.,2.84941315703092));
#46422=CARTESIAN_POINT('Ctrl Pts',(-2.67775201955724,-1.,2.85607274378018));
#46423=CARTESIAN_POINT('Ctrl Pts',(-2.67775201955724,1.,2.85607274378018));
#46424=CARTESIAN_POINT('Ctrl Pts',(-2.68112602796308,-1.,2.86278224277689));
#46425=CARTESIAN_POINT('Ctrl Pts',(-2.68112602796308,1.,2.86278224277689));
#46426=CARTESIAN_POINT('Ctrl Pts',(-2.68447353139599,-1.,2.86953736547238));
#46427=CARTESIAN_POINT('Ctrl Pts',(-2.68447353139599,1.,2.86953736547238));
#46428=CARTESIAN_POINT('Ctrl Pts',(-2.68778807801686,-1.,2.8763300724388));
#46429=CARTESIAN_POINT('Ctrl Pts',(-2.68778807801686,1.,2.8763300724388));
#46430=CARTESIAN_POINT('Ctrl Pts',(-2.69106236420198,-1.,2.88315153980466));
#46431=CARTESIAN_POINT('Ctrl Pts',(-2.69106236420198,1.,2.88315153980466));
#46432=CARTESIAN_POINT('Ctrl Pts',(-2.69429113011374,-1.,2.88999512410309));
#46433=CARTESIAN_POINT('Ctrl Pts',(-2.69429113011374,1.,2.88999512410309));
#46434=CARTESIAN_POINT('Ctrl Pts',(-2.69747340630625,-1.,2.89685866123671));
#46435=CARTESIAN_POINT('Ctrl Pts',(-2.69747340630625,1.,2.89685866123671));
#46436=CARTESIAN_POINT('Ctrl Pts',(-2.70061095078692,-1.,2.90374285605838));
#46437=CARTESIAN_POINT('Ctrl Pts',(-2.70061095078692,1.,2.90374285605838));
#46438=CARTESIAN_POINT('Ctrl Pts',(-2.70370719782113,-1.,2.91065019668329));
#46439=CARTESIAN_POINT('Ctrl Pts',(-2.70370719782113,1.,2.91065019668329));
#46440=CARTESIAN_POINT('Ctrl Pts',(-2.70676602302518,-1.,2.91758367994737));
#46441=CARTESIAN_POINT('Ctrl Pts',(-2.70676602302518,1.,2.91758367994737));
#46442=CARTESIAN_POINT('Ctrl Pts',(-2.70979055994754,-1.,2.92454558914778));
#46443=CARTESIAN_POINT('Ctrl Pts',(-2.70979055994754,1.,2.92454558914778));
#46444=CARTESIAN_POINT('Ctrl Pts',(-2.71278207520817,-1.,2.93153633192595));
#46445=CARTESIAN_POINT('Ctrl Pts',(-2.71278207520817,1.,2.93153633192595));
#46446=CARTESIAN_POINT('Ctrl Pts',(-2.71574054592591,-1.,2.93855503247266));
#46447=CARTESIAN_POINT('Ctrl Pts',(-2.71574054592591,1.,2.93855503247266));
#46448=CARTESIAN_POINT('Ctrl Pts',(-2.71866514227965,-1.,2.94560002559806));
#46449=CARTESIAN_POINT('Ctrl Pts',(-2.71866514227965,1.,2.94560002559806));
#46450=CARTESIAN_POINT('Ctrl Pts',(-2.72155475123364,-1.,2.95266939280621));
#46451=CARTESIAN_POINT('Ctrl Pts',(-2.72155475123364,1.,2.95266939280621));
#46452=CARTESIAN_POINT('Ctrl Pts',(-2.72440846811729,-1.,2.95976146492576));
#46453=CARTESIAN_POINT('Ctrl Pts',(-2.72440846811729,1.,2.95976146492576));
#46454=CARTESIAN_POINT('Ctrl Pts',(-2.72722614084076,-1.,2.96687537842451));
#46455=CARTESIAN_POINT('Ctrl Pts',(-2.72722614084076,1.,2.96687537842451));
#46456=CARTESIAN_POINT('Ctrl Pts',(-2.73000819218414,-1.,2.97401089032677));
#46457=CARTESIAN_POINT('Ctrl Pts',(-2.73000819218414,1.,2.97401089032677));
#46458=CARTESIAN_POINT('Ctrl Pts',(-2.73275539286497,-1.,2.98116814232129));
#46459=CARTESIAN_POINT('Ctrl Pts',(-2.73275539286497,1.,2.98116814232129));
#46460=CARTESIAN_POINT('Ctrl Pts',(-2.73546864694536,-1.,2.9883474369644));
#46461=CARTESIAN_POINT('Ctrl Pts',(-2.73546864694536,1.,2.9883474369644));
#46462=CARTESIAN_POINT('Ctrl Pts',(-2.73814878711641,-1.,2.99554902409778));
#46463=CARTESIAN_POINT('Ctrl Pts',(-2.73814878711641,1.,2.99554902409778));
#46464=CARTESIAN_POINT('Ctrl Pts',(-2.74079632883931,-1.,3.00277284351521));
#46465=CARTESIAN_POINT('Ctrl Pts',(-2.74079632883931,1.,3.00277284351521));
#46466=CARTESIAN_POINT('Ctrl Pts',(-2.74341150239887,-1.,3.01001855960162));
#46467=CARTESIAN_POINT('Ctrl Pts',(-2.74341150239887,1.,3.01001855960162));
#46468=CARTESIAN_POINT('Ctrl Pts',(-2.74599436193625,-1.,3.01728567646611));
#46469=CARTESIAN_POINT('Ctrl Pts',(-2.74599436193625,1.,3.01728567646611));
#46470=CARTESIAN_POINT('Ctrl Pts',(-2.7485448718414,-1.,3.02457362909245));
#46471=CARTESIAN_POINT('Ctrl Pts',(-2.7485448718414,1.,3.02457362909245));
#46472=CARTESIAN_POINT('Ctrl Pts',(-2.75106299522979,-1.,3.03188187589107));
#46473=CARTESIAN_POINT('Ctrl Pts',(-2.75106299522979,1.,3.03188187589107));
#46474=CARTESIAN_POINT('Ctrl Pts',(-2.75354880060314,-1.,3.03921001107977));
#46475=CARTESIAN_POINT('Ctrl Pts',(-2.75354880060314,1.,3.03921001107977));
#46476=CARTESIAN_POINT('Ctrl Pts',(-2.75600247455925,-1.,3.04655777351067));
#46477=CARTESIAN_POINT('Ctrl Pts',(-2.75600247455925,1.,3.04655777351067));
#46478=CARTESIAN_POINT('Ctrl Pts',(-2.75842427252931,-1.,3.05392498749847));
#46479=CARTESIAN_POINT('Ctrl Pts',(-2.75842427252931,1.,3.05392498749847));
#46480=CARTESIAN_POINT('Ctrl Pts',(-2.76081448759882,-1.,3.06131152247454));
#46481=CARTESIAN_POINT('Ctrl Pts',(-2.76081448759882,1.,3.06131152247454));
#46482=CARTESIAN_POINT('Ctrl Pts',(-2.76317341453493,-1.,3.0687172484321));
#46483=CARTESIAN_POINT('Ctrl Pts',(-2.76317341453493,1.,3.0687172484321));
#46484=CARTESIAN_POINT('Ctrl Pts',(-2.76550131064852,-1.,3.07614198408862));
#46485=CARTESIAN_POINT('Ctrl Pts',(-2.76550131064852,1.,3.07614198408862));
#46486=CARTESIAN_POINT('Ctrl Pts',(-2.76779837829373,-1.,3.08358548001504));
#46487=CARTESIAN_POINT('Ctrl Pts',(-2.76779837829373,1.,3.08358548001504));
#46488=CARTESIAN_POINT('Ctrl Pts',(-2.7700647803451,-1.,3.09104745382531));
#46489=CARTESIAN_POINT('Ctrl Pts',(-2.7700647803451,1.,3.09104745382531));
#46490=CARTESIAN_POINT('Ctrl Pts',(-2.77230064796057,-1.,3.0985276127786));
#46491=CARTESIAN_POINT('Ctrl Pts',(-2.77230064796057,1.,3.0985276127786));
#46492=CARTESIAN_POINT('Ctrl Pts',(-2.77450609123362,-1.,3.10602568032564));
#46493=CARTESIAN_POINT('Ctrl Pts',(-2.77450609123362,1.,3.10602568032564));
#46494=CARTESIAN_POINT('Ctrl Pts',(-2.77668121002545,-1.,3.11354142303921));
#46495=CARTESIAN_POINT('Ctrl Pts',(-2.77668121002545,1.,3.11354142303921));
#46496=CARTESIAN_POINT('Ctrl Pts',(-2.77882610146731,-1.,3.12107467037201));
#46497=CARTESIAN_POINT('Ctrl Pts',(-2.77882610146731,1.,3.12107467037201));
#46498=CARTESIAN_POINT('Ctrl Pts',(-2.78094085161413,-1.,3.12862530318457));
#46499=CARTESIAN_POINT('Ctrl Pts',(-2.78094085161413,1.,3.12862530318457));
#46500=CARTESIAN_POINT('Ctrl Pts',(-2.78260859419319,-1.,3.13467965833037));
#46501=CARTESIAN_POINT('Ctrl Pts',(-2.78260859419319,1.,3.13467965833037));
#46502=CARTESIAN_POINT('Ctrl Pts',(-2.78384588958166,-1.,3.13922819749279));
#46503=CARTESIAN_POINT('Ctrl Pts',(-2.78384588958166,1.,3.13922819749279));
#46504=CARTESIAN_POINT('Ctrl Pts',(-2.7846647503589,-1.,3.14226401018816));
#46505=CARTESIAN_POINT('Ctrl Pts',(-2.7846647503589,1.,3.14226401018816));
#46506=CARTESIAN_POINT('Ctrl Pts',(-2.78507268004356,-1.,3.14378277984898));
#46507=CARTESIAN_POINT('Ctrl Pts',(-2.78507268004356,1.,3.14378277984898));
#46508=CARTESIAN_POINT('',(-2.58633475774921,1.,2.71539546306948));
#46509=CARTESIAN_POINT('Ctrl Pts',(-2.58633475774921,-1.,2.71539546306948));
#46510=CARTESIAN_POINT('Ctrl Pts',(-2.58633475774921,-0.666666666666667,
2.71539546306948));
#46511=CARTESIAN_POINT('Ctrl Pts',(-2.58633475774921,-0.333333333333333,
2.71539546306948));
#46512=CARTESIAN_POINT('Ctrl Pts',(-2.58633475774921,0.333333333333333,
2.71539546306948));
#46513=CARTESIAN_POINT('Ctrl Pts',(-2.58633475774921,0.666666666666667,
2.71539546306948));
#46514=CARTESIAN_POINT('Ctrl Pts',(-2.58633475774921,1.,2.71539546306948));
#46515=CARTESIAN_POINT('',(-2.78507268004356,1.,3.14378277984898));
#46516=CARTESIAN_POINT('',(-2.78507268004356,0.,3.14378277984898));
#46517=CARTESIAN_POINT('Ctrl Pts',(-2.58633475774921,1.,2.71539546306948));
#46518=CARTESIAN_POINT('Ctrl Pts',(-2.58638312917167,1.,2.71540296616024));
#46519=CARTESIAN_POINT('Ctrl Pts',(-2.58656037976753,1.,2.71548946460575));
#46520=CARTESIAN_POINT('Ctrl Pts',(-2.58706285424358,1.,2.71591054189786));
#46521=CARTESIAN_POINT('Ctrl Pts',(-2.58823792682672,1.,2.71711860281815));
#46522=CARTESIAN_POINT('Ctrl Pts',(-2.59056604771971,1.,2.71974308958086));
#46523=CARTESIAN_POINT('Ctrl Pts',(-2.59399625537278,1.,2.72378896977134));
#46524=CARTESIAN_POINT('Ctrl Pts',(-2.59817869034746,1.,2.7288648348152));
#46525=CARTESIAN_POINT('Ctrl Pts',(-2.60287635688728,1.,2.73470730109615));
#46526=CARTESIAN_POINT('Ctrl Pts',(-2.60782480638448,1.,2.7410211099909));
#46527=CARTESIAN_POINT('Ctrl Pts',(-2.61277170105813,1.,2.74752219567252));
#46528=CARTESIAN_POINT('Ctrl Pts',(-2.61751580407667,1.,2.7539802502603));
#46529=CARTESIAN_POINT('Ctrl Pts',(-2.62195665834605,1.,2.76027271596686));
#46530=CARTESIAN_POINT('Ctrl Pts',(-2.62609956506355,1.,2.76639078479021));
#46531=CARTESIAN_POINT('Ctrl Pts',(-2.63001305229625,1.,2.77239433377921));
#46532=CARTESIAN_POINT('Ctrl Pts',(-2.63379800904599,1.,2.77837943466449));
#46533=CARTESIAN_POINT('Ctrl Pts',(-2.637554714303,1.,2.78444351041571));
#46534=CARTESIAN_POINT('Ctrl Pts',(-2.64134450532584,1.,2.79064495573224));
#46535=CARTESIAN_POINT('Ctrl Pts',(-2.6451766779932,1.,2.79698910670736));
#46536=CARTESIAN_POINT('Ctrl Pts',(-2.64902988983337,1.,2.80345029781152));
#46537=CARTESIAN_POINT('Ctrl Pts',(-2.65286529532208,1.,2.80998526078165));
#46538=CARTESIAN_POINT('Ctrl Pts',(-2.65664198781344,1.,2.81654896073883));
#46539=CARTESIAN_POINT('Ctrl Pts',(-2.66033388273461,1.,2.82311188135078));
#46540=CARTESIAN_POINT('Ctrl Pts',(-2.6639376472693,1.,2.82966813308998));
#46541=CARTESIAN_POINT('Ctrl Pts',(-2.66746339678107,1.,2.83622586853982));
#46542=CARTESIAN_POINT('Ctrl Pts',(-2.67092916452125,1.,2.84280157191323));
#46543=CARTESIAN_POINT('Ctrl Pts',(-2.67435421039677,1.,2.84941315703092));
#46544=CARTESIAN_POINT('Ctrl Pts',(-2.67775201955724,1.,2.85607274378018));
#46545=CARTESIAN_POINT('Ctrl Pts',(-2.68112602796308,1.,2.86278224277689));
#46546=CARTESIAN_POINT('Ctrl Pts',(-2.68447353139599,1.,2.86953736547238));
#46547=CARTESIAN_POINT('Ctrl Pts',(-2.68778807801686,1.,2.8763300724388));
#46548=CARTESIAN_POINT('Ctrl Pts',(-2.69106236420198,1.,2.88315153980466));
#46549=CARTESIAN_POINT('Ctrl Pts',(-2.69429113011374,1.,2.88999512410309));
#46550=CARTESIAN_POINT('Ctrl Pts',(-2.69747340630625,1.,2.89685866123671));
#46551=CARTESIAN_POINT('Ctrl Pts',(-2.70061095078692,1.,2.90374285605838));
#46552=CARTESIAN_POINT('Ctrl Pts',(-2.70370719782113,1.,2.91065019668329));
#46553=CARTESIAN_POINT('Ctrl Pts',(-2.70676602302518,1.,2.91758367994737));
#46554=CARTESIAN_POINT('Ctrl Pts',(-2.70979055994754,1.,2.92454558914778));
#46555=CARTESIAN_POINT('Ctrl Pts',(-2.71278207520817,1.,2.93153633192595));
#46556=CARTESIAN_POINT('Ctrl Pts',(-2.71574054592591,1.,2.93855503247266));
#46557=CARTESIAN_POINT('Ctrl Pts',(-2.71866514227965,1.,2.94560002559806));
#46558=CARTESIAN_POINT('Ctrl Pts',(-2.72155475123364,1.,2.95266939280621));
#46559=CARTESIAN_POINT('Ctrl Pts',(-2.72440846811729,1.,2.95976146492576));
#46560=CARTESIAN_POINT('Ctrl Pts',(-2.72722614084076,1.,2.96687537842451));
#46561=CARTESIAN_POINT('Ctrl Pts',(-2.73000819218414,1.,2.97401089032677));
#46562=CARTESIAN_POINT('Ctrl Pts',(-2.73275539286497,1.,2.98116814232129));
#46563=CARTESIAN_POINT('Ctrl Pts',(-2.73546864694536,1.,2.9883474369644));
#46564=CARTESIAN_POINT('Ctrl Pts',(-2.73814878711641,1.,2.99554902409778));
#46565=CARTESIAN_POINT('Ctrl Pts',(-2.74079632883931,1.,3.00277284351521));
#46566=CARTESIAN_POINT('Ctrl Pts',(-2.74341150239887,1.,3.01001855960162));
#46567=CARTESIAN_POINT('Ctrl Pts',(-2.74599436193625,1.,3.01728567646611));
#46568=CARTESIAN_POINT('Ctrl Pts',(-2.7485448718414,1.,3.02457362909245));
#46569=CARTESIAN_POINT('Ctrl Pts',(-2.75106299522979,1.,3.03188187589107));
#46570=CARTESIAN_POINT('Ctrl Pts',(-2.75354880060314,1.,3.03921001107977));
#46571=CARTESIAN_POINT('Ctrl Pts',(-2.75600247455925,1.,3.04655777351067));
#46572=CARTESIAN_POINT('Ctrl Pts',(-2.75842427252931,1.,3.05392498749847));
#46573=CARTESIAN_POINT('Ctrl Pts',(-2.76081448759882,1.,3.06131152247454));
#46574=CARTESIAN_POINT('Ctrl Pts',(-2.76317341453493,1.,3.0687172484321));
#46575=CARTESIAN_POINT('Ctrl Pts',(-2.76550131064852,1.,3.07614198408862));
#46576=CARTESIAN_POINT('Ctrl Pts',(-2.76779837829373,1.,3.08358548001504));
#46577=CARTESIAN_POINT('Ctrl Pts',(-2.7700647803451,1.,3.09104745382531));
#46578=CARTESIAN_POINT('Ctrl Pts',(-2.77230064796057,1.,3.0985276127786));
#46579=CARTESIAN_POINT('Ctrl Pts',(-2.77450609123362,1.,3.10602568032564));
#46580=CARTESIAN_POINT('Ctrl Pts',(-2.77668121002545,1.,3.11354142303921));
#46581=CARTESIAN_POINT('Ctrl Pts',(-2.77882610146731,1.,3.12107467037201));
#46582=CARTESIAN_POINT('Ctrl Pts',(-2.78094085161413,1.,3.12862530318457));
#46583=CARTESIAN_POINT('Ctrl Pts',(-2.78260859419319,1.,3.13467965833037));
#46584=CARTESIAN_POINT('Ctrl Pts',(-2.78384588958166,1.,3.13922819749279));
#46585=CARTESIAN_POINT('Ctrl Pts',(-2.7846647503589,1.,3.14226401018816));
#46586=CARTESIAN_POINT('Ctrl Pts',(-2.78507268004356,1.,3.14378277984898));
#46587=CARTESIAN_POINT('Origin',(-2.78507268004356,0.,3.14378277984898));
#46588=CARTESIAN_POINT('',(-2.66939624221984,1.,3.24257979115744));
#46589=CARTESIAN_POINT('Origin',(0.,0.,0.));
#46590=CARTESIAN_POINT('',(-2.71539546306824,1.,2.58633475775051));
#46591=CARTESIAN_POINT('Origin',(0.,1.,0.));
#46592=CARTESIAN_POINT('Ctrl Pts',(-2.71539546306824,1.,2.58633475775051));
#46593=CARTESIAN_POINT('Ctrl Pts',(-2.71539546306824,0.666666666666667,
2.58633475775051));
#46594=CARTESIAN_POINT('Ctrl Pts',(-2.71539546306824,0.333333333333333,
2.58633475775051));
#46595=CARTESIAN_POINT('Ctrl Pts',(-2.71539546306824,-0.333333333333333,
2.58633475775051));
#46596=CARTESIAN_POINT('Ctrl Pts',(-2.71539546306824,-0.666666666666667,
2.58633475775051));
#46597=CARTESIAN_POINT('Ctrl Pts',(-2.71539546306824,-1.,2.58633475775051));
#46598=CARTESIAN_POINT('Ctrl Pts',(-3.14378277984898,-1.,2.78507268004356));
#46599=CARTESIAN_POINT('Ctrl Pts',(-3.14378277984898,1.,2.78507268004356));
#46600=CARTESIAN_POINT('Ctrl Pts',(-3.14226401019149,-1.,2.78466475036183));
#46601=CARTESIAN_POINT('Ctrl Pts',(-3.14226401019149,1.,2.78466475036183));
#46602=CARTESIAN_POINT('Ctrl Pts',(-3.13922819750185,-1.,2.78384588958965));
#46603=CARTESIAN_POINT('Ctrl Pts',(-3.13922819750185,1.,2.78384588958965));
#46604=CARTESIAN_POINT('Ctrl Pts',(-3.1346796583452,-1.,2.78260859420629));
#46605=CARTESIAN_POINT('Ctrl Pts',(-3.1346796583452,1.,2.78260859420629));
#46606=CARTESIAN_POINT('Ctrl Pts',(-3.12862530320194,-1.,2.78094085162947));
#46607=CARTESIAN_POINT('Ctrl Pts',(-3.12862530320194,1.,2.78094085162947));
#46608=CARTESIAN_POINT('Ctrl Pts',(-3.12107467038623,-1.,2.77882610147986));
#46609=CARTESIAN_POINT('Ctrl Pts',(-3.12107467038623,1.,2.77882610147986));
#46610=CARTESIAN_POINT('Ctrl Pts',(-3.11354142304692,-1.,2.77668121003225));
#46611=CARTESIAN_POINT('Ctrl Pts',(-3.11354142304692,1.,2.77668121003225));
#46612=CARTESIAN_POINT('Ctrl Pts',(-3.10602568032641,-1.,2.7745060912343));
#46613=CARTESIAN_POINT('Ctrl Pts',(-3.10602568032641,1.,2.7745060912343));
#46614=CARTESIAN_POINT('Ctrl Pts',(-3.09852761277432,-1.,2.77230064795679));
#46615=CARTESIAN_POINT('Ctrl Pts',(-3.09852761277432,1.,2.77230064795679));
#46616=CARTESIAN_POINT('Ctrl Pts',(-3.09104745381882,-1.,2.77006478033937));
#46617=CARTESIAN_POINT('Ctrl Pts',(-3.09104745381882,1.,2.77006478033937));
#46618=CARTESIAN_POINT('Ctrl Pts',(-3.08358548000904,-1.,2.76779837828843));
#46619=CARTESIAN_POINT('Ctrl Pts',(-3.08358548000904,1.,2.76779837828843));
#46620=CARTESIAN_POINT('Ctrl Pts',(-3.07614198408488,-1.,2.76550131064522));
#46621=CARTESIAN_POINT('Ctrl Pts',(-3.07614198408488,1.,2.76550131064522));
#46622=CARTESIAN_POINT('Ctrl Pts',(-3.06871724843121,-1.,2.76317341453415));
#46623=CARTESIAN_POINT('Ctrl Pts',(-3.06871724843121,1.,2.76317341453415));
#46624=CARTESIAN_POINT('Ctrl Pts',(-3.06131152247599,-1.,2.76081448760011));
#46625=CARTESIAN_POINT('Ctrl Pts',(-3.06131152247599,1.,2.76081448760011));
#46626=CARTESIAN_POINT('Ctrl Pts',(-3.05392498750112,-1.,2.75842427253164));
#46627=CARTESIAN_POINT('Ctrl Pts',(-3.05392498750112,1.,2.75842427253164));
#46628=CARTESIAN_POINT('Ctrl Pts',(-3.04655777351333,-1.,2.7560024745616));
#46629=CARTESIAN_POINT('Ctrl Pts',(-3.04655777351333,1.,2.7560024745616));
#46630=CARTESIAN_POINT('Ctrl Pts',(-3.03921001108158,-1.,2.75354880060473));
#46631=CARTESIAN_POINT('Ctrl Pts',(-3.03921001108158,1.,2.75354880060473));
#46632=CARTESIAN_POINT('Ctrl Pts',(-3.03188187589168,-1.,2.75106299523032));
#46633=CARTESIAN_POINT('Ctrl Pts',(-3.03188187589168,1.,2.75106299523032));
#46634=CARTESIAN_POINT('Ctrl Pts',(-3.02457362909199,-1.,2.74854487184099));
#46635=CARTESIAN_POINT('Ctrl Pts',(-3.02457362909199,1.,2.74854487184099));
#46636=CARTESIAN_POINT('Ctrl Pts',(-3.01728567646502,-1.,2.74599436193528));
#46637=CARTESIAN_POINT('Ctrl Pts',(-3.01728567646502,1.,2.74599436193528));
#46638=CARTESIAN_POINT('Ctrl Pts',(-3.01001855960041,-1.,2.7434115023978));
#46639=CARTESIAN_POINT('Ctrl Pts',(-3.01001855960041,1.,2.7434115023978));
#46640=CARTESIAN_POINT('Ctrl Pts',(-3.00277284351431,-1.,2.74079632883852));
#46641=CARTESIAN_POINT('Ctrl Pts',(-3.00277284351431,1.,2.74079632883852));
#46642=CARTESIAN_POINT('Ctrl Pts',(-2.99554902409741,-1.,2.73814878711609));
#46643=CARTESIAN_POINT('Ctrl Pts',(-2.99554902409741,1.,2.73814878711609));
#46644=CARTESIAN_POINT('Ctrl Pts',(-2.98834743696455,-1.,2.73546864694548));
#46645=CARTESIAN_POINT('Ctrl Pts',(-2.98834743696455,1.,2.73546864694548));
#46646=CARTESIAN_POINT('Ctrl Pts',(-2.98116814232175,-1.,2.73275539286537));
#46647=CARTESIAN_POINT('Ctrl Pts',(-2.98116814232175,1.,2.73275539286537));
#46648=CARTESIAN_POINT('Ctrl Pts',(-2.97401089032729,-1.,2.7300081921846));
#46649=CARTESIAN_POINT('Ctrl Pts',(-2.97401089032729,1.,2.7300081921846));
#46650=CARTESIAN_POINT('Ctrl Pts',(-2.96687537842492,-1.,2.72722614084112));
#46651=CARTESIAN_POINT('Ctrl Pts',(-2.96687537842492,1.,2.72722614084112));
#46652=CARTESIAN_POINT('Ctrl Pts',(-2.95976146492595,-1.,2.72440846811745));
#46653=CARTESIAN_POINT('Ctrl Pts',(-2.95976146492595,1.,2.72440846811745));
#46654=CARTESIAN_POINT('Ctrl Pts',(-2.95266939280617,-1.,2.72155475123361));
#46655=CARTESIAN_POINT('Ctrl Pts',(-2.95266939280617,1.,2.72155475123361));
#46656=CARTESIAN_POINT('Ctrl Pts',(-2.94560002559789,-1.,2.71866514227952));
#46657=CARTESIAN_POINT('Ctrl Pts',(-2.94560002559789,1.,2.71866514227952));
#46658=CARTESIAN_POINT('Ctrl Pts',(-2.93855503247248,-1.,2.71574054592575));
#46659=CARTESIAN_POINT('Ctrl Pts',(-2.93855503247248,1.,2.71574054592575));
#46660=CARTESIAN_POINT('Ctrl Pts',(-2.93153633192583,-1.,2.71278207520807));
#46661=CARTESIAN_POINT('Ctrl Pts',(-2.93153633192583,1.,2.71278207520807));
#46662=CARTESIAN_POINT('Ctrl Pts',(-2.92454558914774,-1.,2.70979055994751));
#46663=CARTESIAN_POINT('Ctrl Pts',(-2.92454558914774,1.,2.70979055994751));
#46664=CARTESIAN_POINT('Ctrl Pts',(-2.91758367994738,-1.,2.70676602302518));
#46665=CARTESIAN_POINT('Ctrl Pts',(-2.91758367994738,1.,2.70676602302518));
#46666=CARTESIAN_POINT('Ctrl Pts',(-2.91065019668331,-1.,2.70370719782114));
#46667=CARTESIAN_POINT('Ctrl Pts',(-2.91065019668331,1.,2.70370719782114));
#46668=CARTESIAN_POINT('Ctrl Pts',(-2.90374285605839,-1.,2.70061095078692));
#46669=CARTESIAN_POINT('Ctrl Pts',(-2.90374285605839,1.,2.70061095078692));
#46670=CARTESIAN_POINT('Ctrl Pts',(-2.89685866123668,-1.,2.69747340630621));
#46671=CARTESIAN_POINT('Ctrl Pts',(-2.89685866123668,1.,2.69747340630621));
#46672=CARTESIAN_POINT('Ctrl Pts',(-2.88999512410304,-1.,2.69429113011369));
#46673=CARTESIAN_POINT('Ctrl Pts',(-2.88999512410304,1.,2.69429113011369));
#46674=CARTESIAN_POINT('Ctrl Pts',(-2.88315153980464,-1.,2.69106236420197));
#46675=CARTESIAN_POINT('Ctrl Pts',(-2.88315153980464,1.,2.69106236420197));
#46676=CARTESIAN_POINT('Ctrl Pts',(-2.87633007243885,-1.,2.68778807801691));
#46677=CARTESIAN_POINT('Ctrl Pts',(-2.87633007243885,1.,2.68778807801691));
#46678=CARTESIAN_POINT('Ctrl Pts',(-2.8695373654725,-1.,2.68447353139611));
#46679=CARTESIAN_POINT('Ctrl Pts',(-2.8695373654725,1.,2.68447353139611));
#46680=CARTESIAN_POINT('Ctrl Pts',(-2.86278224277705,-1.,2.68112602796323));
#46681=CARTESIAN_POINT('Ctrl Pts',(-2.86278224277705,1.,2.68112602796323));
#46682=CARTESIAN_POINT('Ctrl Pts',(-2.85607274378031,-1.,2.67775201955736));
#46683=CARTESIAN_POINT('Ctrl Pts',(-2.85607274378031,1.,2.67775201955736));
#46684=CARTESIAN_POINT('Ctrl Pts',(-2.84941315703096,-1.,2.67435421039682));
#46685=CARTESIAN_POINT('Ctrl Pts',(-2.84941315703096,1.,2.67435421039682));
#46686=CARTESIAN_POINT('Ctrl Pts',(-2.84280157191314,-1.,2.67092916452117));
#46687=CARTESIAN_POINT('Ctrl Pts',(-2.84280157191314,1.,2.67092916452117));
#46688=CARTESIAN_POINT('Ctrl Pts',(-2.8362258685396,-1.,2.66746339678085));
#46689=CARTESIAN_POINT('Ctrl Pts',(-2.8362258685396,1.,2.66746339678085));
#46690=CARTESIAN_POINT('Ctrl Pts',(-2.82966813308969,-1.,2.66393764726902));
#46691=CARTESIAN_POINT('Ctrl Pts',(-2.82966813308969,1.,2.66393764726902));
#46692=CARTESIAN_POINT('Ctrl Pts',(-2.82311188135053,-1.,2.66033388273437));
#46693=CARTESIAN_POINT('Ctrl Pts',(-2.82311188135053,1.,2.66033388273437));
#46694=CARTESIAN_POINT('Ctrl Pts',(-2.81654896073874,-1.,2.65664198781335));
#46695=CARTESIAN_POINT('Ctrl Pts',(-2.81654896073874,1.,2.65664198781335));
#46696=CARTESIAN_POINT('Ctrl Pts',(-2.80998526078179,-1.,2.65286529532221));
#46697=CARTESIAN_POINT('Ctrl Pts',(-2.80998526078179,1.,2.65286529532221));
#46698=CARTESIAN_POINT('Ctrl Pts',(-2.80345029781191,-1.,2.64902988983373));
#46699=CARTESIAN_POINT('Ctrl Pts',(-2.80345029781191,1.,2.64902988983373));
#46700=CARTESIAN_POINT('Ctrl Pts',(-2.7969891067079,-1.,2.6451766779937));
#46701=CARTESIAN_POINT('Ctrl Pts',(-2.7969891067079,1.,2.6451766779937));
#46702=CARTESIAN_POINT('Ctrl Pts',(-2.79064495573275,-1.,2.64134450532632));
#46703=CARTESIAN_POINT('Ctrl Pts',(-2.79064495573275,1.,2.64134450532632));
#46704=CARTESIAN_POINT('Ctrl Pts',(-2.78444351041594,-1.,2.63755471430322));
#46705=CARTESIAN_POINT('Ctrl Pts',(-2.78444351041594,1.,2.63755471430322));
#46706=CARTESIAN_POINT('Ctrl Pts',(-2.77837943466423,-1.,2.63379800904575));
#46707=CARTESIAN_POINT('Ctrl Pts',(-2.77837943466423,1.,2.63379800904575));
#46708=CARTESIAN_POINT('Ctrl Pts',(-2.77239433377839,-1.,2.63001305229548));
#46709=CARTESIAN_POINT('Ctrl Pts',(-2.77239433377839,1.,2.63001305229548));
#46710=CARTESIAN_POINT('Ctrl Pts',(-2.76639078478898,-1.,2.6260995650624));
#46711=CARTESIAN_POINT('Ctrl Pts',(-2.76639078478898,1.,2.6260995650624));
#46712=CARTESIAN_POINT('Ctrl Pts',(-2.76027271596564,-1.,2.62195665834491));
#46713=CARTESIAN_POINT('Ctrl Pts',(-2.76027271596564,1.,2.62195665834491));
#46714=CARTESIAN_POINT('Ctrl Pts',(-2.75398025025967,-1.,2.61751580407608));
#46715=CARTESIAN_POINT('Ctrl Pts',(-2.75398025025967,1.,2.61751580407608));
#46716=CARTESIAN_POINT('Ctrl Pts',(-2.74752219567307,-1.,2.61277170105864));
#46717=CARTESIAN_POINT('Ctrl Pts',(-2.74752219567307,1.,2.61277170105864));
#46718=CARTESIAN_POINT('Ctrl Pts',(-2.74102110999284,-1.,2.60782480638629));
#46719=CARTESIAN_POINT('Ctrl Pts',(-2.74102110999284,1.,2.60782480638629));
#46720=CARTESIAN_POINT('Ctrl Pts',(-2.73470730109906,-1.,2.60287635689));
#46721=CARTESIAN_POINT('Ctrl Pts',(-2.73470730109906,1.,2.60287635689));
#46722=CARTESIAN_POINT('Ctrl Pts',(-2.72886483481804,-1.,2.5981786903501));
#46723=CARTESIAN_POINT('Ctrl Pts',(-2.72886483481804,1.,2.5981786903501));
#46724=CARTESIAN_POINT('Ctrl Pts',(-2.72378896977273,-1.,2.59399625537407));
#46725=CARTESIAN_POINT('Ctrl Pts',(-2.72378896977273,1.,2.59399625537407));
#46726=CARTESIAN_POINT('Ctrl Pts',(-2.7197430895797,-1.,2.59056604771863));
#46727=CARTESIAN_POINT('Ctrl Pts',(-2.7197430895797,1.,2.59056604771863));
#46728=CARTESIAN_POINT('Ctrl Pts',(-2.71690570241274,-1.,2.58804906785078));
#46729=CARTESIAN_POINT('Ctrl Pts',(-2.71690570241274,1.,2.58804906785078));
#46730=CARTESIAN_POINT('Ctrl Pts',(-2.71566956750046,-1.,2.58682657352212));
#46731=CARTESIAN_POINT('Ctrl Pts',(-2.71566956750046,1.,2.58682657352212));
#46732=CARTESIAN_POINT('Ctrl Pts',(-2.71533674140979,-1.,2.58636629903847));
#46733=CARTESIAN_POINT('Ctrl Pts',(-2.71533674140979,1.,2.58636629903847));
#46734=CARTESIAN_POINT('Ctrl Pts',(-2.71537879705,-1.,2.58626222935706));
#46735=CARTESIAN_POINT('Ctrl Pts',(-2.71537879705,1.,2.58626222935706));
#46736=CARTESIAN_POINT('Ctrl Pts',(-2.71546581445404,-1.,2.58626089374824));
#46737=CARTESIAN_POINT('Ctrl Pts',(-2.71546581445404,1.,2.58626089374824));
#46738=CARTESIAN_POINT('',(-3.14378277984898,1.,2.78507268004356));
#46739=CARTESIAN_POINT('Ctrl Pts',(-3.14378277984898,1.,2.78507268004356));
#46740=CARTESIAN_POINT('Ctrl Pts',(-3.14226401019149,1.,2.78466475036183));
#46741=CARTESIAN_POINT('Ctrl Pts',(-3.13922819750185,1.,2.78384588958965));
#46742=CARTESIAN_POINT('Ctrl Pts',(-3.1346796583452,1.,2.78260859420629));
#46743=CARTESIAN_POINT('Ctrl Pts',(-3.12862530320194,1.,2.78094085162947));
#46744=CARTESIAN_POINT('Ctrl Pts',(-3.12107467038623,1.,2.77882610147986));
#46745=CARTESIAN_POINT('Ctrl Pts',(-3.11354142304692,1.,2.77668121003225));
#46746=CARTESIAN_POINT('Ctrl Pts',(-3.10602568032641,1.,2.7745060912343));
#46747=CARTESIAN_POINT('Ctrl Pts',(-3.09852761277432,1.,2.77230064795679));
#46748=CARTESIAN_POINT('Ctrl Pts',(-3.09104745381882,1.,2.77006478033937));
#46749=CARTESIAN_POINT('Ctrl Pts',(-3.08358548000904,1.,2.76779837828843));
#46750=CARTESIAN_POINT('Ctrl Pts',(-3.07614198408488,1.,2.76550131064522));
#46751=CARTESIAN_POINT('Ctrl Pts',(-3.06871724843121,1.,2.76317341453415));
#46752=CARTESIAN_POINT('Ctrl Pts',(-3.06131152247599,1.,2.76081448760011));
#46753=CARTESIAN_POINT('Ctrl Pts',(-3.05392498750112,1.,2.75842427253164));
#46754=CARTESIAN_POINT('Ctrl Pts',(-3.04655777351333,1.,2.7560024745616));
#46755=CARTESIAN_POINT('Ctrl Pts',(-3.03921001108158,1.,2.75354880060473));
#46756=CARTESIAN_POINT('Ctrl Pts',(-3.03188187589168,1.,2.75106299523032));
#46757=CARTESIAN_POINT('Ctrl Pts',(-3.02457362909199,1.,2.74854487184099));
#46758=CARTESIAN_POINT('Ctrl Pts',(-3.01728567646502,1.,2.74599436193528));
#46759=CARTESIAN_POINT('Ctrl Pts',(-3.01001855960041,1.,2.7434115023978));
#46760=CARTESIAN_POINT('Ctrl Pts',(-3.00277284351431,1.,2.74079632883852));
#46761=CARTESIAN_POINT('Ctrl Pts',(-2.99554902409741,1.,2.73814878711609));
#46762=CARTESIAN_POINT('Ctrl Pts',(-2.98834743696455,1.,2.73546864694548));
#46763=CARTESIAN_POINT('Ctrl Pts',(-2.98116814232175,1.,2.73275539286537));
#46764=CARTESIAN_POINT('Ctrl Pts',(-2.97401089032729,1.,2.7300081921846));
#46765=CARTESIAN_POINT('Ctrl Pts',(-2.96687537842492,1.,2.72722614084112));
#46766=CARTESIAN_POINT('Ctrl Pts',(-2.95976146492595,1.,2.72440846811745));
#46767=CARTESIAN_POINT('Ctrl Pts',(-2.95266939280617,1.,2.72155475123361));
#46768=CARTESIAN_POINT('Ctrl Pts',(-2.94560002559789,1.,2.71866514227952));
#46769=CARTESIAN_POINT('Ctrl Pts',(-2.93855503247248,1.,2.71574054592575));
#46770=CARTESIAN_POINT('Ctrl Pts',(-2.93153633192583,1.,2.71278207520807));
#46771=CARTESIAN_POINT('Ctrl Pts',(-2.92454558914774,1.,2.70979055994751));
#46772=CARTESIAN_POINT('Ctrl Pts',(-2.91758367994738,1.,2.70676602302518));
#46773=CARTESIAN_POINT('Ctrl Pts',(-2.91065019668331,1.,2.70370719782114));
#46774=CARTESIAN_POINT('Ctrl Pts',(-2.90374285605839,1.,2.70061095078692));
#46775=CARTESIAN_POINT('Ctrl Pts',(-2.89685866123668,1.,2.69747340630621));
#46776=CARTESIAN_POINT('Ctrl Pts',(-2.88999512410304,1.,2.69429113011369));
#46777=CARTESIAN_POINT('Ctrl Pts',(-2.88315153980464,1.,2.69106236420197));
#46778=CARTESIAN_POINT('Ctrl Pts',(-2.87633007243885,1.,2.68778807801691));
#46779=CARTESIAN_POINT('Ctrl Pts',(-2.8695373654725,1.,2.68447353139611));
#46780=CARTESIAN_POINT('Ctrl Pts',(-2.86278224277705,1.,2.68112602796323));
#46781=CARTESIAN_POINT('Ctrl Pts',(-2.85607274378031,1.,2.67775201955736));
#46782=CARTESIAN_POINT('Ctrl Pts',(-2.84941315703096,1.,2.67435421039682));
#46783=CARTESIAN_POINT('Ctrl Pts',(-2.84280157191314,1.,2.67092916452117));
#46784=CARTESIAN_POINT('Ctrl Pts',(-2.8362258685396,1.,2.66746339678085));
#46785=CARTESIAN_POINT('Ctrl Pts',(-2.82966813308969,1.,2.66393764726902));
#46786=CARTESIAN_POINT('Ctrl Pts',(-2.82311188135053,1.,2.66033388273437));
#46787=CARTESIAN_POINT('Ctrl Pts',(-2.81654896073874,1.,2.65664198781335));
#46788=CARTESIAN_POINT('Ctrl Pts',(-2.80998526078179,1.,2.65286529532221));
#46789=CARTESIAN_POINT('Ctrl Pts',(-2.80345029781191,1.,2.64902988983373));
#46790=CARTESIAN_POINT('Ctrl Pts',(-2.7969891067079,1.,2.6451766779937));
#46791=CARTESIAN_POINT('Ctrl Pts',(-2.79064495573275,1.,2.64134450532632));
#46792=CARTESIAN_POINT('Ctrl Pts',(-2.78444351041594,1.,2.63755471430322));
#46793=CARTESIAN_POINT('Ctrl Pts',(-2.77837943466423,1.,2.63379800904575));
#46794=CARTESIAN_POINT('Ctrl Pts',(-2.77239433377839,1.,2.63001305229548));
#46795=CARTESIAN_POINT('Ctrl Pts',(-2.76639078478898,1.,2.6260995650624));
#46796=CARTESIAN_POINT('Ctrl Pts',(-2.76027271596564,1.,2.62195665834491));
#46797=CARTESIAN_POINT('Ctrl Pts',(-2.75398025025967,1.,2.61751580407608));
#46798=CARTESIAN_POINT('Ctrl Pts',(-2.74752219567307,1.,2.61277170105864));
#46799=CARTESIAN_POINT('Ctrl Pts',(-2.74102110999284,1.,2.60782480638629));
#46800=CARTESIAN_POINT('Ctrl Pts',(-2.73470730109906,1.,2.60287635689));
#46801=CARTESIAN_POINT('Ctrl Pts',(-2.72886483481804,1.,2.5981786903501));
#46802=CARTESIAN_POINT('Ctrl Pts',(-2.72378896977273,1.,2.59399625537407));
#46803=CARTESIAN_POINT('Ctrl Pts',(-2.7197430895797,1.,2.59056604771863));
#46804=CARTESIAN_POINT('Ctrl Pts',(-2.7171186028189,1.,2.58823792682724));
#46805=CARTESIAN_POINT('Ctrl Pts',(-2.71591054189884,1.,2.58706285424469));
#46806=CARTESIAN_POINT('Ctrl Pts',(-2.71548946460616,1.,2.58656037976884));
#46807=CARTESIAN_POINT('Ctrl Pts',(-2.71540296615967,1.,2.58638312917291));
#46808=CARTESIAN_POINT('Ctrl Pts',(-2.71539546306824,1.,2.58633475775051));
#46809=CARTESIAN_POINT('',(-3.14378277984898,0.,2.78507268004356));
#46810=CARTESIAN_POINT('Ctrl Pts',(-2.97921217251145,-1.,2.27745358485296));
#46811=CARTESIAN_POINT('Ctrl Pts',(-2.97921217251145,1.,2.27745358485296));
#46812=CARTESIAN_POINT('Ctrl Pts',(-2.97919987915679,-1.,2.27736742984319));
#46813=CARTESIAN_POINT('Ctrl Pts',(-2.97919987915679,1.,2.27736742984319));
#46814=CARTESIAN_POINT('Ctrl Pts',(-2.97929608861798,-1.,2.2773096118942));
#46815=CARTESIAN_POINT('Ctrl Pts',(-2.97929608861798,1.,2.2773096118942));
#46816=CARTESIAN_POINT('Ctrl Pts',(-2.97980276183181,-1.,2.27756633755188));
#46817=CARTESIAN_POINT('Ctrl Pts',(-2.97980276183181,1.,2.27756633755188));
#46818=CARTESIAN_POINT('Ctrl Pts',(-2.98120357932994,-1.,2.27859601334547));
#46819=CARTESIAN_POINT('Ctrl Pts',(-2.98120357932994,1.,2.27859601334547));
#46820=CARTESIAN_POINT('Ctrl Pts',(-2.98413343613983,-1.,2.28100472516679));
#46821=CARTESIAN_POINT('Ctrl Pts',(-2.98413343613983,1.,2.28100472516679));
#46822=CARTESIAN_POINT('Ctrl Pts',(-2.9881543273478,-1.,2.28446419115919));
#46823=CARTESIAN_POINT('Ctrl Pts',(-2.9881543273478,1.,2.28446419115919));
#46824=CARTESIAN_POINT('Ctrl Pts',(-2.99307930984034,-1.,2.28882328690362));
#46825=CARTESIAN_POINT('Ctrl Pts',(-2.99307930984034,1.,2.28882328690362));
#46826=CARTESIAN_POINT('Ctrl Pts',(-2.99863310339691,-1.,2.29385894577754));
#46827=CARTESIAN_POINT('Ctrl Pts',(-2.99863310339691,1.,2.29385894577754));
#46828=CARTESIAN_POINT('Ctrl Pts',(-3.00450832658613,-1.,2.29932091315775));
#46829=CARTESIAN_POINT('Ctrl Pts',(-3.00450832658613,1.,2.29932091315775));
#46830=CARTESIAN_POINT('Ctrl Pts',(-3.01041131063823,-1.,2.30496809486482));
#46831=CARTESIAN_POINT('Ctrl Pts',(-3.01041131063823,1.,2.30496809486482));
#46832=CARTESIAN_POINT('Ctrl Pts',(-3.01610726819086,-1.,2.31060449886629));
#46833=CARTESIAN_POINT('Ctrl Pts',(-3.01610726819086,1.,2.31060449886629));
#46834=CARTESIAN_POINT('Ctrl Pts',(-3.02147780668161,-1.,2.31612479121631));
#46835=CARTESIAN_POINT('Ctrl Pts',(-3.02147780668161,1.,2.31612479121631));
#46836=CARTESIAN_POINT('Ctrl Pts',(-3.02652678416611,-1.,2.32151944306402));
#46837=CARTESIAN_POINT('Ctrl Pts',(-3.02652678416611,1.,2.32151944306402));
#46838=CARTESIAN_POINT('Ctrl Pts',(-3.03133125185136,-1.,2.32683687412097));
#46839=CARTESIAN_POINT('Ctrl Pts',(-3.03133125185136,1.,2.32683687412097));
#46840=CARTESIAN_POINT('Ctrl Pts',(-3.03600588555793,-1.,2.33215619079829));
#46841=CARTESIAN_POINT('Ctrl Pts',(-3.03600588555793,1.,2.33215619079829));
#46842=CARTESIAN_POINT('Ctrl Pts',(-3.04066496998544,-1.,2.33755792953706));
#46843=CARTESIAN_POINT('Ctrl Pts',(-3.04066496998544,1.,2.33755792953706));
#46844=CARTESIAN_POINT('Ctrl Pts',(-3.04537822217256,-1.,2.34309017083977));
#46845=CARTESIAN_POINT('Ctrl Pts',(-3.04537822217256,1.,2.34309017083977));
#46846=CARTESIAN_POINT('Ctrl Pts',(-3.05015565829918,-1.,2.34875673090771));
#46847=CARTESIAN_POINT('Ctrl Pts',(-3.05015565829918,1.,2.34875673090771));
#46848=CARTESIAN_POINT('Ctrl Pts',(-3.05497218368146,-1.,2.35453559889474));
#46849=CARTESIAN_POINT('Ctrl Pts',(-3.05497218368146,1.,2.35453559889474));
#46850=CARTESIAN_POINT('Ctrl Pts',(-3.0597826624004,-1.,2.36039011602072));
#46851=CARTESIAN_POINT('Ctrl Pts',(-3.0597826624004,1.,2.36039011602072));
#46852=CARTESIAN_POINT('Ctrl Pts',(-3.06453964643162,-1.,2.36628220107009));
#46853=CARTESIAN_POINT('Ctrl Pts',(-3.06453964643162,1.,2.36628220107009));
#46854=CARTESIAN_POINT('Ctrl Pts',(-3.069212754975,-1.,2.37218678163178));
#46855=CARTESIAN_POINT('Ctrl Pts',(-3.069212754975,1.,2.37218678163178));
#46856=CARTESIAN_POINT('Ctrl Pts',(-3.07379777492165,-1.,2.37809856205548));
#46857=CARTESIAN_POINT('Ctrl Pts',(-3.07379777492165,1.,2.37809856205548));
#46858=CARTESIAN_POINT('Ctrl Pts',(-3.07830597244326,-1.,2.38402401216126));
#46859=CARTESIAN_POINT('Ctrl Pts',(-3.07830597244326,1.,2.38402401216126));
#46860=CARTESIAN_POINT('Ctrl Pts',(-3.08275773747093,-1.,2.38997659219199));
#46861=CARTESIAN_POINT('Ctrl Pts',(-3.08275773747093,1.,2.38997659219199));
#46862=CARTESIAN_POINT('Ctrl Pts',(-3.08717489512914,-1.,2.39597098250631));
#46863=CARTESIAN_POINT('Ctrl Pts',(-3.08717489512914,1.,2.39597098250631));
#46864=CARTESIAN_POINT('Ctrl Pts',(-3.091572660511,-1.,2.40201704423341));
#46865=CARTESIAN_POINT('Ctrl Pts',(-3.091572660511,1.,2.40201704423341));
#46866=CARTESIAN_POINT('Ctrl Pts',(-3.09595472616076,-1.,2.40811612696369));
#46867=CARTESIAN_POINT('Ctrl Pts',(-3.09595472616076,1.,2.40811612696369));
#46868=CARTESIAN_POINT('Ctrl Pts',(-3.1003177502767,-1.,2.41426441798057));
#46869=CARTESIAN_POINT('Ctrl Pts',(-3.1003177502767,1.,2.41426441798057));
#46870=CARTESIAN_POINT('Ctrl Pts',(-3.10465410280896,-1.,2.42045498612489));
#46871=CARTESIAN_POINT('Ctrl Pts',(-3.10465410280896,1.,2.42045498612489));
#46872=CARTESIAN_POINT('Ctrl Pts',(-3.10895518969595,-1.,2.42668025870015));
#46873=CARTESIAN_POINT('Ctrl Pts',(-3.10895518969595,1.,2.42668025870015));
#46874=CARTESIAN_POINT('Ctrl Pts',(-3.11321477659018,-1.,2.43293449685144));
#46875=CARTESIAN_POINT('Ctrl Pts',(-3.11321477659018,1.,2.43293449685144));
#46876=CARTESIAN_POINT('Ctrl Pts',(-3.11743156744186,-1.,2.43921571477977));
#46877=CARTESIAN_POINT('Ctrl Pts',(-3.11743156744186,1.,2.43921571477977));
#46878=CARTESIAN_POINT('Ctrl Pts',(-3.12160740887768,-1.,2.44552433364715));
#46879=CARTESIAN_POINT('Ctrl Pts',(-3.12160740887768,1.,2.44552433364715));
#46880=CARTESIAN_POINT('Ctrl Pts',(-3.12574608210847,-1.,2.45186227369846));
#46881=CARTESIAN_POINT('Ctrl Pts',(-3.12574608210847,1.,2.45186227369846));
#46882=CARTESIAN_POINT('Ctrl Pts',(-3.12985188384371,-1.,2.45823188859366));
#46883=CARTESIAN_POINT('Ctrl Pts',(-3.12985188384371,1.,2.45823188859366));
#46884=CARTESIAN_POINT('Ctrl Pts',(-3.13392826623906,-1.,2.46463494332374));
#46885=CARTESIAN_POINT('Ctrl Pts',(-3.13392826623906,1.,2.46463494332374));
#46886=CARTESIAN_POINT('Ctrl Pts',(-3.13797654408943,-1.,2.47107164236838));
#46887=CARTESIAN_POINT('Ctrl Pts',(-3.13797654408943,1.,2.47107164236838));
#46888=CARTESIAN_POINT('Ctrl Pts',(-3.14199655778863,-1.,2.47754112428043));
#46889=CARTESIAN_POINT('Ctrl Pts',(-3.14199655778863,1.,2.47754112428043));
#46890=CARTESIAN_POINT('Ctrl Pts',(-3.14598722723896,-1.,2.4840418741839));
#46891=CARTESIAN_POINT('Ctrl Pts',(-3.14598722723896,1.,2.4840418741839));
#46892=CARTESIAN_POINT('Ctrl Pts',(-3.14994715298907,-1.,2.49057217131988));
#46893=CARTESIAN_POINT('Ctrl Pts',(-3.14994715298907,1.,2.49057217131988));
#46894=CARTESIAN_POINT('Ctrl Pts',(-3.15387518039046,-1.,2.49713050858896));
#46895=CARTESIAN_POINT('Ctrl Pts',(-3.15387518039046,1.,2.49713050858896));
#46896=CARTESIAN_POINT('Ctrl Pts',(-3.15777102413957,-1.,2.50371605688252));
#46897=CARTESIAN_POINT('Ctrl Pts',(-3.15777102413957,1.,2.50371605688252));
#46898=CARTESIAN_POINT('Ctrl Pts',(-3.16163506380157,-1.,2.51032851007894));
#46899=CARTESIAN_POINT('Ctrl Pts',(-3.16163506380157,1.,2.51032851007894));
#46900=CARTESIAN_POINT('Ctrl Pts',(-3.16546808277023,-1.,2.51696788755577));
#46901=CARTESIAN_POINT('Ctrl Pts',(-3.16546808277023,1.,2.51696788755577));
#46902=CARTESIAN_POINT('Ctrl Pts',(-3.16927102130736,-1.,2.52363434671788));
#46903=CARTESIAN_POINT('Ctrl Pts',(-3.16927102130736,1.,2.52363434671788));
#46904=CARTESIAN_POINT('Ctrl Pts',(-3.17304474093612,-1.,2.53032800406941));
#46905=CARTESIAN_POINT('Ctrl Pts',(-3.17304474093612,1.,2.53032800406941));
#46906=CARTESIAN_POINT('Ctrl Pts',(-3.17678974135318,-1.,2.53704871950948));
#46907=CARTESIAN_POINT('Ctrl Pts',(-3.17678974135318,1.,2.53704871950948));
#46908=CARTESIAN_POINT('Ctrl Pts',(-3.1805061975064,-1.,2.54379612553051));
#46909=CARTESIAN_POINT('Ctrl Pts',(-3.1805061975064,1.,2.54379612553051));
#46910=CARTESIAN_POINT('Ctrl Pts',(-3.18419408529594,-1.,2.55056972387731));
#46911=CARTESIAN_POINT('Ctrl Pts',(-3.18419408529594,1.,2.55056972387731));
#46912=CARTESIAN_POINT('Ctrl Pts',(-3.18785328116218,-1.,2.55736896206056));
#46913=CARTESIAN_POINT('Ctrl Pts',(-3.18785328116218,1.,2.55736896206056));
#46914=CARTESIAN_POINT('Ctrl Pts',(-3.19148366395139,-1.,2.56419331092858));
#46915=CARTESIAN_POINT('Ctrl Pts',(-3.19148366395139,1.,2.56419331092858));
#46916=CARTESIAN_POINT('Ctrl Pts',(-3.19508523784363,-1.,2.57104235897899));
#46917=CARTESIAN_POINT('Ctrl Pts',(-3.19508523784363,1.,2.57104235897899));
#46918=CARTESIAN_POINT('Ctrl Pts',(-3.19865814628682,-1.,2.57791581908875));
#46919=CARTESIAN_POINT('Ctrl Pts',(-3.19865814628682,1.,2.57791581908875));
#46920=CARTESIAN_POINT('Ctrl Pts',(-3.20220261408414,-1.,2.58481347777729));
#46921=CARTESIAN_POINT('Ctrl Pts',(-3.20220261408414,1.,2.58481347777729));
#46922=CARTESIAN_POINT('Ctrl Pts',(-3.2057189102873,-1.,2.59173516023481));
#46923=CARTESIAN_POINT('Ctrl Pts',(-3.2057189102873,1.,2.59173516023481));
#46924=CARTESIAN_POINT('Ctrl Pts',(-3.20920730569681,-1.,2.59868069194342));
#46925=CARTESIAN_POINT('Ctrl Pts',(-3.20920730569681,1.,2.59868069194342));
#46926=CARTESIAN_POINT('Ctrl Pts',(-3.21266802609682,-1.,2.60564985360017));
#46927=CARTESIAN_POINT('Ctrl Pts',(-3.21266802609682,1.,2.60564985360017));
#46928=CARTESIAN_POINT('Ctrl Pts',(-3.21610123233082,-1.,2.61264236719171));
#46929=CARTESIAN_POINT('Ctrl Pts',(-3.21610123233082,1.,2.61264236719171));
#46930=CARTESIAN_POINT('Ctrl Pts',(-3.21950704109321,-1.,2.61965792832947));
#46931=CARTESIAN_POINT('Ctrl Pts',(-3.21950704109321,1.,2.61965792832947));
#46932=CARTESIAN_POINT('Ctrl Pts',(-3.2228855361324,-1.,2.62669622735912));
#46933=CARTESIAN_POINT('Ctrl Pts',(-3.2228855361324,1.,2.62669622735912));
#46934=CARTESIAN_POINT('Ctrl Pts',(-3.2262367829246,-1.,2.63375697391372));
#46935=CARTESIAN_POINT('Ctrl Pts',(-3.2262367829246,1.,2.63375697391372));
#46936=CARTESIAN_POINT('Ctrl Pts',(-3.22956084358547,-1.,2.64083992181823));
#46937=CARTESIAN_POINT('Ctrl Pts',(-3.22956084358547,1.,2.64083992181823));
#46938=CARTESIAN_POINT('Ctrl Pts',(-3.23285778737096,-1.,2.64794488743038));
#46939=CARTESIAN_POINT('Ctrl Pts',(-3.23285778737096,1.,2.64794488743038));
#46940=CARTESIAN_POINT('Ctrl Pts',(-3.236127680639,-1.,2.65507173961555));
#46941=CARTESIAN_POINT('Ctrl Pts',(-3.236127680639,1.,2.65507173961555));
#46942=CARTESIAN_POINT('Ctrl Pts',(-3.23872200034785,-1.,2.6607906631847));
#46943=CARTESIAN_POINT('Ctrl Pts',(-3.23872200034785,1.,2.6607906631847));
#46944=CARTESIAN_POINT('Ctrl Pts',(-3.24065561086749,-1.,2.66508964663997));
#46945=CARTESIAN_POINT('Ctrl Pts',(-3.24065561086749,1.,2.66508964663997));
#46946=CARTESIAN_POINT('Ctrl Pts',(-3.24193929584471,-1.,2.66795998539579));
#46947=CARTESIAN_POINT('Ctrl Pts',(-3.24193929584471,1.,2.66795998539579));
#46948=CARTESIAN_POINT('Ctrl Pts',(-3.24257979115744,-1.,2.66939624221984));
#46949=CARTESIAN_POINT('Ctrl Pts',(-3.24257979115744,1.,2.66939624221984));
#46950=CARTESIAN_POINT('',(-2.97927412174279,1.,2.27737254473521));
#46951=CARTESIAN_POINT('Ctrl Pts',(-2.97927412174279,-1.,2.27737254473521));
#46952=CARTESIAN_POINT('Ctrl Pts',(-2.97927412174279,-0.666666666666667,
2.27737254473521));
#46953=CARTESIAN_POINT('Ctrl Pts',(-2.97927412174279,-0.333333333333333,
2.27737254473521));
#46954=CARTESIAN_POINT('Ctrl Pts',(-2.97927412174279,0.333333333333333,
2.27737254473521));
#46955=CARTESIAN_POINT('Ctrl Pts',(-2.97927412174279,0.666666666666667,
2.27737254473521));
#46956=CARTESIAN_POINT('Ctrl Pts',(-2.97927412174279,1.,2.27737254473521));
#46957=CARTESIAN_POINT('',(-3.24257979115744,1.,2.66939624221984));
#46958=CARTESIAN_POINT('',(-3.24257979115744,0.,2.66939624221984));
#46959=CARTESIAN_POINT('Ctrl Pts',(-2.97927412174279,1.,2.27737254473521));
#46960=CARTESIAN_POINT('Ctrl Pts',(-2.97932307137476,1.,2.27737238849287));
#46961=CARTESIAN_POINT('Ctrl Pts',(-2.9795116710597,1.,2.27743009389684));
#46962=CARTESIAN_POINT('Ctrl Pts',(-2.98007383024207,1.,2.27776738270289));
#46963=CARTESIAN_POINT('Ctrl Pts',(-2.9814234180956,1.,2.27877674853766));
#46964=CARTESIAN_POINT('Ctrl Pts',(-2.98413343613983,1.,2.28100472516679));
#46965=CARTESIAN_POINT('Ctrl Pts',(-2.9881543273478,1.,2.28446419115919));
#46966=CARTESIAN_POINT('Ctrl Pts',(-2.99307930984034,1.,2.28882328690362));
#46967=CARTESIAN_POINT('Ctrl Pts',(-2.99863310339691,1.,2.29385894577754));
#46968=CARTESIAN_POINT('Ctrl Pts',(-3.00450832658613,1.,2.29932091315775));
#46969=CARTESIAN_POINT('Ctrl Pts',(-3.01041131063823,1.,2.30496809486482));
#46970=CARTESIAN_POINT('Ctrl Pts',(-3.01610726819086,1.,2.31060449886629));
#46971=CARTESIAN_POINT('Ctrl Pts',(-3.02147780668161,1.,2.31612479121631));
#46972=CARTESIAN_POINT('Ctrl Pts',(-3.02652678416611,1.,2.32151944306402));
#46973=CARTESIAN_POINT('Ctrl Pts',(-3.03133125185136,1.,2.32683687412097));
#46974=CARTESIAN_POINT('Ctrl Pts',(-3.03600588555793,1.,2.33215619079829));
#46975=CARTESIAN_POINT('Ctrl Pts',(-3.04066496998544,1.,2.33755792953706));
#46976=CARTESIAN_POINT('Ctrl Pts',(-3.04537822217256,1.,2.34309017083977));
#46977=CARTESIAN_POINT('Ctrl Pts',(-3.05015565829918,1.,2.34875673090771));
#46978=CARTESIAN_POINT('Ctrl Pts',(-3.05497218368146,1.,2.35453559889474));
#46979=CARTESIAN_POINT('Ctrl Pts',(-3.0597826624004,1.,2.36039011602072));
#46980=CARTESIAN_POINT('Ctrl Pts',(-3.06453964643162,1.,2.36628220107009));
#46981=CARTESIAN_POINT('Ctrl Pts',(-3.069212754975,1.,2.37218678163178));
#46982=CARTESIAN_POINT('Ctrl Pts',(-3.07379777492165,1.,2.37809856205548));
#46983=CARTESIAN_POINT('Ctrl Pts',(-3.07830597244326,1.,2.38402401216126));
#46984=CARTESIAN_POINT('Ctrl Pts',(-3.08275773747093,1.,2.38997659219199));
#46985=CARTESIAN_POINT('Ctrl Pts',(-3.08717489512914,1.,2.39597098250631));
#46986=CARTESIAN_POINT('Ctrl Pts',(-3.091572660511,1.,2.40201704423341));
#46987=CARTESIAN_POINT('Ctrl Pts',(-3.09595472616076,1.,2.40811612696369));
#46988=CARTESIAN_POINT('Ctrl Pts',(-3.1003177502767,1.,2.41426441798057));
#46989=CARTESIAN_POINT('Ctrl Pts',(-3.10465410280896,1.,2.42045498612489));
#46990=CARTESIAN_POINT('Ctrl Pts',(-3.10895518969595,1.,2.42668025870015));
#46991=CARTESIAN_POINT('Ctrl Pts',(-3.11321477659018,1.,2.43293449685144));
#46992=CARTESIAN_POINT('Ctrl Pts',(-3.11743156744186,1.,2.43921571477977));
#46993=CARTESIAN_POINT('Ctrl Pts',(-3.12160740887768,1.,2.44552433364715));
#46994=CARTESIAN_POINT('Ctrl Pts',(-3.12574608210847,1.,2.45186227369846));
#46995=CARTESIAN_POINT('Ctrl Pts',(-3.12985188384371,1.,2.45823188859366));
#46996=CARTESIAN_POINT('Ctrl Pts',(-3.13392826623906,1.,2.46463494332374));
#46997=CARTESIAN_POINT('Ctrl Pts',(-3.13797654408943,1.,2.47107164236838));
#46998=CARTESIAN_POINT('Ctrl Pts',(-3.14199655778863,1.,2.47754112428043));
#46999=CARTESIAN_POINT('Ctrl Pts',(-3.14598722723896,1.,2.4840418741839));
#47000=CARTESIAN_POINT('Ctrl Pts',(-3.14994715298907,1.,2.49057217131988));
#47001=CARTESIAN_POINT('Ctrl Pts',(-3.15387518039046,1.,2.49713050858896));
#47002=CARTESIAN_POINT('Ctrl Pts',(-3.15777102413957,1.,2.50371605688252));
#47003=CARTESIAN_POINT('Ctrl Pts',(-3.16163506380157,1.,2.51032851007894));
#47004=CARTESIAN_POINT('Ctrl Pts',(-3.16546808277023,1.,2.51696788755577));
#47005=CARTESIAN_POINT('Ctrl Pts',(-3.16927102130736,1.,2.52363434671788));
#47006=CARTESIAN_POINT('Ctrl Pts',(-3.17304474093612,1.,2.53032800406941));
#47007=CARTESIAN_POINT('Ctrl Pts',(-3.17678974135318,1.,2.53704871950948));
#47008=CARTESIAN_POINT('Ctrl Pts',(-3.1805061975064,1.,2.54379612553051));
#47009=CARTESIAN_POINT('Ctrl Pts',(-3.18419408529594,1.,2.55056972387731));
#47010=CARTESIAN_POINT('Ctrl Pts',(-3.18785328116218,1.,2.55736896206056));
#47011=CARTESIAN_POINT('Ctrl Pts',(-3.19148366395139,1.,2.56419331092858));
#47012=CARTESIAN_POINT('Ctrl Pts',(-3.19508523784363,1.,2.57104235897899));
#47013=CARTESIAN_POINT('Ctrl Pts',(-3.19865814628682,1.,2.57791581908875));
#47014=CARTESIAN_POINT('Ctrl Pts',(-3.20220261408414,1.,2.58481347777729));
#47015=CARTESIAN_POINT('Ctrl Pts',(-3.2057189102873,1.,2.59173516023481));
#47016=CARTESIAN_POINT('Ctrl Pts',(-3.20920730569681,1.,2.59868069194342));
#47017=CARTESIAN_POINT('Ctrl Pts',(-3.21266802609682,1.,2.60564985360017));
#47018=CARTESIAN_POINT('Ctrl Pts',(-3.21610123233082,1.,2.61264236719171));
#47019=CARTESIAN_POINT('Ctrl Pts',(-3.21950704109321,1.,2.61965792832947));
#47020=CARTESIAN_POINT('Ctrl Pts',(-3.2228855361324,1.,2.62669622735912));
#47021=CARTESIAN_POINT('Ctrl Pts',(-3.2262367829246,1.,2.63375697391372));
#47022=CARTESIAN_POINT('Ctrl Pts',(-3.22956084358547,1.,2.64083992181823));
#47023=CARTESIAN_POINT('Ctrl Pts',(-3.23285778737096,1.,2.64794488743038));
#47024=CARTESIAN_POINT('Ctrl Pts',(-3.236127680639,1.,2.65507173961555));
#47025=CARTESIAN_POINT('Ctrl Pts',(-3.23872200034785,1.,2.6607906631847));
#47026=CARTESIAN_POINT('Ctrl Pts',(-3.24065561086749,1.,2.66508964663997));
#47027=CARTESIAN_POINT('Ctrl Pts',(-3.24193929584471,1.,2.66795998539579));
#47028=CARTESIAN_POINT('Ctrl Pts',(-3.24257979115744,1.,2.66939624221984));
#47029=CARTESIAN_POINT('Origin',(-3.24257979115744,0.,2.66939624221984));
#47030=CARTESIAN_POINT('',(-3.14378277984898,1.,2.78507268004356));
#47031=CARTESIAN_POINT('Origin',(0.,0.,0.));
#47032=CARTESIAN_POINT('',(-3.08655633322109,1.,2.12971124846838));
#47033=CARTESIAN_POINT('Origin',(0.,1.,0.));
#47034=CARTESIAN_POINT('Ctrl Pts',(-3.08655633322109,1.,2.12971124846838));
#47035=CARTESIAN_POINT('Ctrl Pts',(-3.08655633322109,0.666666666666667,
2.12971124846838));
#47036=CARTESIAN_POINT('Ctrl Pts',(-3.08655633322109,0.333333333333333,
2.12971124846838));
#47037=CARTESIAN_POINT('Ctrl Pts',(-3.08655633322109,-0.333333333333333,
2.12971124846838));
#47038=CARTESIAN_POINT('Ctrl Pts',(-3.08655633322109,-0.666666666666667,
2.12971124846838));
#47039=CARTESIAN_POINT('Ctrl Pts',(-3.08655633322109,-1.,2.12971124846838));
#47040=CARTESIAN_POINT('Ctrl Pts',(-3.54075895182139,-1.,2.25898783642071));
#47041=CARTESIAN_POINT('Ctrl Pts',(-3.54075895182139,1.,2.25898783642071));
#47042=CARTESIAN_POINT('Ctrl Pts',(-3.5391950664771,-1.,2.25882251694918));
#47043=CARTESIAN_POINT('Ctrl Pts',(-3.5391950664771,1.,2.25882251694918));
#47044=CARTESIAN_POINT('Ctrl Pts',(-3.53606853163247,-1.,2.25848864344599));
#47045=CARTESIAN_POINT('Ctrl Pts',(-3.53606853163247,1.,2.25848864344599));
#47046=CARTESIAN_POINT('Ctrl Pts',(-3.53138243689932,-1.,2.25797812951166));
#47047=CARTESIAN_POINT('Ctrl Pts',(-3.53138243689932,1.,2.25797812951166));
#47048=CARTESIAN_POINT('Ctrl Pts',(-3.52514172849666,-1.,2.25727802942141));
#47049=CARTESIAN_POINT('Ctrl Pts',(-3.52514172849666,1.,2.25727802942141));
#47050=CARTESIAN_POINT('Ctrl Pts',(-3.51735323669213,-1.,2.25637049456061));
#47051=CARTESIAN_POINT('Ctrl Pts',(-3.51735323669213,1.,2.25637049456061));
#47052=CARTESIAN_POINT('Ctrl Pts',(-3.50957720118209,-1.,2.25543046980351));
#47053=CARTESIAN_POINT('Ctrl Pts',(-3.50957720118209,1.,2.25543046980351));
#47054=CARTESIAN_POINT('Ctrl Pts',(-3.50181372618058,-1.,2.25445785151923));
#47055=CARTESIAN_POINT('Ctrl Pts',(-3.50181372618058,1.,2.25445785151923));
#47056=CARTESIAN_POINT('Ctrl Pts',(-3.49406296494309,-1.,2.25345251709453));
#47057=CARTESIAN_POINT('Ctrl Pts',(-3.49406296494309,1.,2.25345251709453));
#47058=CARTESIAN_POINT('Ctrl Pts',(-3.48632513240231,-1.,2.25241433138231));
#47059=CARTESIAN_POINT('Ctrl Pts',(-3.48632513240231,1.,2.25241433138231));
#47060=CARTESIAN_POINT('Ctrl Pts',(-3.47860048448015,-1.,2.25134314238258));
#47061=CARTESIAN_POINT('Ctrl Pts',(-3.47860048448015,1.,2.25134314238258));
#47062=CARTESIAN_POINT('Ctrl Pts',(-3.47088928979467,-1.,2.25023877475674));
#47063=CARTESIAN_POINT('Ctrl Pts',(-3.47088928979467,1.,2.25023877475674));
#47064=CARTESIAN_POINT('Ctrl Pts',(-3.46319180177474,-1.,2.24910102345977));
#47065=CARTESIAN_POINT('Ctrl Pts',(-3.46319180177474,1.,2.24910102345977));
#47066=CARTESIAN_POINT('Ctrl Pts',(-3.45550823512213,-1.,2.24792964960874));
#47067=CARTESIAN_POINT('Ctrl Pts',(-3.45550823512213,1.,2.24792964960874));
#47068=CARTESIAN_POINT('Ctrl Pts',(-3.44783872863448,-1.,2.24672437070139));
#47069=CARTESIAN_POINT('Ctrl Pts',(-3.44783872863448,1.,2.24672437070139));
#47070=CARTESIAN_POINT('Ctrl Pts',(-3.44018336460619,-1.,2.24548487526212));
#47071=CARTESIAN_POINT('Ctrl Pts',(-3.44018336460619,1.,2.24548487526212));
#47072=CARTESIAN_POINT('Ctrl Pts',(-3.43254222615007,-1.,2.24421085338856));
#47073=CARTESIAN_POINT('Ctrl Pts',(-3.43254222615007,1.,2.24421085338856));
#47074=CARTESIAN_POINT('Ctrl Pts',(-3.42491544683075,-1.,2.24290202531144));
#47075=CARTESIAN_POINT('Ctrl Pts',(-3.42491544683075,1.,2.24290202531144));
#47076=CARTESIAN_POINT('Ctrl Pts',(-3.41730325539119,-1.,2.24155816587811));
#47077=CARTESIAN_POINT('Ctrl Pts',(-3.41730325539119,1.,2.24155816587811));
#47078=CARTESIAN_POINT('Ctrl Pts',(-3.40970604190205,-1.,2.24017914395211));
#47079=CARTESIAN_POINT('Ctrl Pts',(-3.40970604190205,1.,2.24017914395211));
#47080=CARTESIAN_POINT('Ctrl Pts',(-3.40212434705511,-1.,2.23876491124064));
#47081=CARTESIAN_POINT('Ctrl Pts',(-3.40212434705511,1.,2.23876491124064));
#47082=CARTESIAN_POINT('Ctrl Pts',(-3.39455873448088,-1.,2.23731541452727));
#47083=CARTESIAN_POINT('Ctrl Pts',(-3.39455873448088,1.,2.23731541452727));
#47084=CARTESIAN_POINT('Ctrl Pts',(-3.38700968549522,-1.,2.23583052276281));
#47085=CARTESIAN_POINT('Ctrl Pts',(-3.38700968549522,1.,2.23583052276281));
#47086=CARTESIAN_POINT('Ctrl Pts',(-3.37947749555649,-1.,2.23430995599572));
#47087=CARTESIAN_POINT('Ctrl Pts',(-3.37947749555649,1.,2.23430995599572));
#47088=CARTESIAN_POINT('Ctrl Pts',(-3.37196214349356,-1.,2.23275319569253));
#47089=CARTESIAN_POINT('Ctrl Pts',(-3.37196214349356,1.,2.23275319569253));
#47090=CARTESIAN_POINT('Ctrl Pts',(-3.36446325227908,-1.,2.23115945849777));
#47091=CARTESIAN_POINT('Ctrl Pts',(-3.36446325227908,1.,2.23115945849777));
#47092=CARTESIAN_POINT('Ctrl Pts',(-3.35698038165529,-1.,2.22952789881011));
#47093=CARTESIAN_POINT('Ctrl Pts',(-3.35698038165529,1.,2.22952789881011));
#47094=CARTESIAN_POINT('Ctrl Pts',(-3.34951327111117,-1.,2.22785777756588));
#47095=CARTESIAN_POINT('Ctrl Pts',(-3.34951327111117,1.,2.22785777756588));
#47096=CARTESIAN_POINT('Ctrl Pts',(-3.34206209449371,-1.,2.22614863918044));
#47097=CARTESIAN_POINT('Ctrl Pts',(-3.34206209449371,1.,2.22614863918044));
#47098=CARTESIAN_POINT('Ctrl Pts',(-3.3346277284958,-1.,2.224400498785));
#47099=CARTESIAN_POINT('Ctrl Pts',(-3.3346277284958,1.,2.224400498785));
#47100=CARTESIAN_POINT('Ctrl Pts',(-3.32721196326019,-1.,2.22261398879623));
#47101=CARTESIAN_POINT('Ctrl Pts',(-3.32721196326019,1.,2.22261398879623));
#47102=CARTESIAN_POINT('Ctrl Pts',(-3.31981686778008,-1.,2.22078990842768));
#47103=CARTESIAN_POINT('Ctrl Pts',(-3.31981686778008,1.,2.22078990842768));
#47104=CARTESIAN_POINT('Ctrl Pts',(-3.31244421655662,-1.,2.21892881679083));
#47105=CARTESIAN_POINT('Ctrl Pts',(-3.31244421655662,1.,2.21892881679083));
#47106=CARTESIAN_POINT('Ctrl Pts',(-3.3050948781957,-1.,2.21703059947837));
#47107=CARTESIAN_POINT('Ctrl Pts',(-3.3050948781957,1.,2.21703059947837));
#47108=CARTESIAN_POINT('Ctrl Pts',(-3.29776825193162,-1.,2.21509406923369));
#47109=CARTESIAN_POINT('Ctrl Pts',(-3.29776825193162,1.,2.21509406923369));
#47110=CARTESIAN_POINT('Ctrl Pts',(-3.29046159238344,-1.,2.21311648827391));
#47111=CARTESIAN_POINT('Ctrl Pts',(-3.29046159238344,1.,2.21311648827391));
#47112=CARTESIAN_POINT('Ctrl Pts',(-3.28317133333127,-1.,2.21109449750638));
#47113=CARTESIAN_POINT('Ctrl Pts',(-3.28317133333127,1.,2.21109449750638));
#47114=CARTESIAN_POINT('Ctrl Pts',(-3.27589448005534,-1.,2.20902509417425));
#47115=CARTESIAN_POINT('Ctrl Pts',(-3.27589448005534,1.,2.20902509417425));
#47116=CARTESIAN_POINT('Ctrl Pts',(-3.2686300613678,-1.,2.20690665217741));
#47117=CARTESIAN_POINT('Ctrl Pts',(-3.2686300613678,1.,2.20690665217741));
#47118=CARTESIAN_POINT('Ctrl Pts',(-3.26138036637711,-1.,2.20473979048682));
#47119=CARTESIAN_POINT('Ctrl Pts',(-3.26138036637711,1.,2.20473979048682));
#47120=CARTESIAN_POINT('Ctrl Pts',(-3.25415277957789,-1.,2.20252866491554));
#47121=CARTESIAN_POINT('Ctrl Pts',(-3.25415277957789,1.,2.20252866491554));
#47122=CARTESIAN_POINT('Ctrl Pts',(-3.24695715874356,-1.,2.20027910880993));
#47123=CARTESIAN_POINT('Ctrl Pts',(-3.24695715874356,1.,2.20027910880993));
#47124=CARTESIAN_POINT('Ctrl Pts',(-3.23980245361323,-1.,2.19799623693263));
#47125=CARTESIAN_POINT('Ctrl Pts',(-3.23980245361323,1.,2.19799623693263));
#47126=CARTESIAN_POINT('Ctrl Pts',(-3.23269332296938,-1.,2.19568204933172));
#47127=CARTESIAN_POINT('Ctrl Pts',(-3.23269332296938,1.,2.19568204933172));
#47128=CARTESIAN_POINT('Ctrl Pts',(-3.22562734221636,-1.,2.19333345123531));
#47129=CARTESIAN_POINT('Ctrl Pts',(-3.22562734221636,1.,2.19333345123531));
#47130=CARTESIAN_POINT('Ctrl Pts',(-3.21859043114069,-1.,2.1909390194865));
#47131=CARTESIAN_POINT('Ctrl Pts',(-3.21859043114069,1.,2.1909390194865));
#47132=CARTESIAN_POINT('Ctrl Pts',(-3.21156188355736,-1.,2.18848253363878));
#47133=CARTESIAN_POINT('Ctrl Pts',(-3.21156188355736,1.,2.18848253363878));
#47134=CARTESIAN_POINT('Ctrl Pts',(-3.20452259717947,-1.,2.18594876115914));
#47135=CARTESIAN_POINT('Ctrl Pts',(-3.20452259717947,1.,2.18594876115914));
#47136=CARTESIAN_POINT('Ctrl Pts',(-3.197462937404,-1.,2.18332898656595));
#47137=CARTESIAN_POINT('Ctrl Pts',(-3.197462937404,1.,2.18332898656595));
#47138=CARTESIAN_POINT('Ctrl Pts',(-3.19038924261589,-1.,2.18062558031789));
#47139=CARTESIAN_POINT('Ctrl Pts',(-3.19038924261589,1.,2.18062558031789));
#47140=CARTESIAN_POINT('Ctrl Pts',(-3.18333474627851,-1.,2.17785968847172));
#47141=CARTESIAN_POINT('Ctrl Pts',(-3.18333474627851,1.,2.17785968847172));
#47142=CARTESIAN_POINT('Ctrl Pts',(-3.17635032802584,-1.,2.17506466903736));
#47143=CARTESIAN_POINT('Ctrl Pts',(-3.17635032802584,1.,2.17506466903736));
#47144=CARTESIAN_POINT('Ctrl Pts',(-3.16948480019555,-1.,2.17227212063857));
#47145=CARTESIAN_POINT('Ctrl Pts',(-3.16948480019555,1.,2.17227212063857));
#47146=CARTESIAN_POINT('Ctrl Pts',(-3.16276685102999,-1.,2.16949910801237));
#47147=CARTESIAN_POINT('Ctrl Pts',(-3.16276685102999,1.,2.16949910801237));
#47148=CARTESIAN_POINT('Ctrl Pts',(-3.15618975593627,-1.,2.1667372844767));
#47149=CARTESIAN_POINT('Ctrl Pts',(-3.15618975593627,1.,2.1667372844767));
#47150=CARTESIAN_POINT('Ctrl Pts',(-3.14968624388961,-1.,2.16393520288009));
#47151=CARTESIAN_POINT('Ctrl Pts',(-3.14968624388961,1.,2.16393520288009));
#47152=CARTESIAN_POINT('Ctrl Pts',(-3.14314440426882,-1.,2.16100905914341));
#47153=CARTESIAN_POINT('Ctrl Pts',(-3.14314440426882,1.,2.16100905914341));
#47154=CARTESIAN_POINT('Ctrl Pts',(-3.136453565629,-1.,2.15787423530583));
#47155=CARTESIAN_POINT('Ctrl Pts',(-3.136453565629,1.,2.15787423530583));
#47156=CARTESIAN_POINT('Ctrl Pts',(-3.12954386795575,-1.,2.15447241382872));
#47157=CARTESIAN_POINT('Ctrl Pts',(-3.12954386795575,1.,2.15447241382872));
#47158=CARTESIAN_POINT('Ctrl Pts',(-3.12242318152001,-1.,2.15079698090627));
#47159=CARTESIAN_POINT('Ctrl Pts',(-3.12242318152001,1.,2.15079698090627));
#47160=CARTESIAN_POINT('Ctrl Pts',(-3.11522827017075,-1.,2.1469279845768));
#47161=CARTESIAN_POINT('Ctrl Pts',(-3.11522827017075,1.,2.1469279845768));
#47162=CARTESIAN_POINT('Ctrl Pts',(-3.10821808669189,-1.,2.14302815602195));
#47163=CARTESIAN_POINT('Ctrl Pts',(-3.10821808669189,1.,2.14302815602195));
#47164=CARTESIAN_POINT('Ctrl Pts',(-3.1017126739137,-1.,2.13930228863968));
#47165=CARTESIAN_POINT('Ctrl Pts',(-3.1017126739137,1.,2.13930228863968));
#47166=CARTESIAN_POINT('Ctrl Pts',(-3.09604502421197,-1.,2.13596538661154));
#47167=CARTESIAN_POINT('Ctrl Pts',(-3.09604502421197,1.,2.13596538661154));
#47168=CARTESIAN_POINT('Ctrl Pts',(-3.09151235281832,-1.,2.13321032560805));
#47169=CARTESIAN_POINT('Ctrl Pts',(-3.09151235281832,1.,2.13321032560805));
#47170=CARTESIAN_POINT('Ctrl Pts',(-3.08831615619661,-1.,2.13116819908263));
#47171=CARTESIAN_POINT('Ctrl Pts',(-3.08831615619661,1.,2.13116819908263));
#47172=CARTESIAN_POINT('Ctrl Pts',(-3.08690399991003,-1.,2.1301541297915));
#47173=CARTESIAN_POINT('Ctrl Pts',(-3.08690399991003,1.,2.1301541297915));
#47174=CARTESIAN_POINT('Ctrl Pts',(-3.08650326866821,-1.,2.12975158752197));
#47175=CARTESIAN_POINT('Ctrl Pts',(-3.08650326866821,1.,2.12975158752197));
#47176=CARTESIAN_POINT('Ctrl Pts',(-3.08652852644876,-1.,2.12964222015945));
#47177=CARTESIAN_POINT('Ctrl Pts',(-3.08652852644876,1.,2.12964222015945));
#47178=CARTESIAN_POINT('Ctrl Pts',(-3.08661426358891,-1.,2.12962728847314));
#47179=CARTESIAN_POINT('Ctrl Pts',(-3.08661426358891,1.,2.12962728847314));
#47180=CARTESIAN_POINT('',(-3.54075895182139,1.,2.25898783642071));
#47181=CARTESIAN_POINT('Ctrl Pts',(-3.54075895182139,1.,2.25898783642071));
#47182=CARTESIAN_POINT('Ctrl Pts',(-3.5391950664771,1.,2.25882251694918));
#47183=CARTESIAN_POINT('Ctrl Pts',(-3.53606853163247,1.,2.25848864344599));
#47184=CARTESIAN_POINT('Ctrl Pts',(-3.53138243689932,1.,2.25797812951166));
#47185=CARTESIAN_POINT('Ctrl Pts',(-3.52514172849666,1.,2.25727802942141));
#47186=CARTESIAN_POINT('Ctrl Pts',(-3.51735323669213,1.,2.25637049456061));
#47187=CARTESIAN_POINT('Ctrl Pts',(-3.50957720118209,1.,2.25543046980351));
#47188=CARTESIAN_POINT('Ctrl Pts',(-3.50181372618058,1.,2.25445785151923));
#47189=CARTESIAN_POINT('Ctrl Pts',(-3.49406296494309,1.,2.25345251709453));
#47190=CARTESIAN_POINT('Ctrl Pts',(-3.48632513240231,1.,2.25241433138231));
#47191=CARTESIAN_POINT('Ctrl Pts',(-3.47860048448015,1.,2.25134314238258));
#47192=CARTESIAN_POINT('Ctrl Pts',(-3.47088928979467,1.,2.25023877475674));
#47193=CARTESIAN_POINT('Ctrl Pts',(-3.46319180177474,1.,2.24910102345977));
#47194=CARTESIAN_POINT('Ctrl Pts',(-3.45550823512213,1.,2.24792964960874));
#47195=CARTESIAN_POINT('Ctrl Pts',(-3.44783872863448,1.,2.24672437070139));
#47196=CARTESIAN_POINT('Ctrl Pts',(-3.44018336460619,1.,2.24548487526212));
#47197=CARTESIAN_POINT('Ctrl Pts',(-3.43254222615007,1.,2.24421085338856));
#47198=CARTESIAN_POINT('Ctrl Pts',(-3.42491544683075,1.,2.24290202531144));
#47199=CARTESIAN_POINT('Ctrl Pts',(-3.41730325539119,1.,2.24155816587811));
#47200=CARTESIAN_POINT('Ctrl Pts',(-3.40970604190205,1.,2.24017914395211));
#47201=CARTESIAN_POINT('Ctrl Pts',(-3.40212434705511,1.,2.23876491124064));
#47202=CARTESIAN_POINT('Ctrl Pts',(-3.39455873448088,1.,2.23731541452727));
#47203=CARTESIAN_POINT('Ctrl Pts',(-3.38700968549522,1.,2.23583052276281));
#47204=CARTESIAN_POINT('Ctrl Pts',(-3.37947749555649,1.,2.23430995599572));
#47205=CARTESIAN_POINT('Ctrl Pts',(-3.37196214349356,1.,2.23275319569253));
#47206=CARTESIAN_POINT('Ctrl Pts',(-3.36446325227908,1.,2.23115945849777));
#47207=CARTESIAN_POINT('Ctrl Pts',(-3.35698038165529,1.,2.22952789881011));
#47208=CARTESIAN_POINT('Ctrl Pts',(-3.34951327111117,1.,2.22785777756588));
#47209=CARTESIAN_POINT('Ctrl Pts',(-3.34206209449371,1.,2.22614863918044));
#47210=CARTESIAN_POINT('Ctrl Pts',(-3.3346277284958,1.,2.224400498785));
#47211=CARTESIAN_POINT('Ctrl Pts',(-3.32721196326019,1.,2.22261398879623));
#47212=CARTESIAN_POINT('Ctrl Pts',(-3.31981686778008,1.,2.22078990842768));
#47213=CARTESIAN_POINT('Ctrl Pts',(-3.31244421655662,1.,2.21892881679083));
#47214=CARTESIAN_POINT('Ctrl Pts',(-3.3050948781957,1.,2.21703059947837));
#47215=CARTESIAN_POINT('Ctrl Pts',(-3.29776825193162,1.,2.21509406923369));
#47216=CARTESIAN_POINT('Ctrl Pts',(-3.29046159238344,1.,2.21311648827391));
#47217=CARTESIAN_POINT('Ctrl Pts',(-3.28317133333127,1.,2.21109449750638));
#47218=CARTESIAN_POINT('Ctrl Pts',(-3.27589448005534,1.,2.20902509417425));
#47219=CARTESIAN_POINT('Ctrl Pts',(-3.2686300613678,1.,2.20690665217741));
#47220=CARTESIAN_POINT('Ctrl Pts',(-3.26138036637711,1.,2.20473979048682));
#47221=CARTESIAN_POINT('Ctrl Pts',(-3.25415277957789,1.,2.20252866491554));
#47222=CARTESIAN_POINT('Ctrl Pts',(-3.24695715874356,1.,2.20027910880993));
#47223=CARTESIAN_POINT('Ctrl Pts',(-3.23980245361323,1.,2.19799623693263));
#47224=CARTESIAN_POINT('Ctrl Pts',(-3.23269332296938,1.,2.19568204933172));
#47225=CARTESIAN_POINT('Ctrl Pts',(-3.22562734221636,1.,2.19333345123531));
#47226=CARTESIAN_POINT('Ctrl Pts',(-3.21859043114069,1.,2.1909390194865));
#47227=CARTESIAN_POINT('Ctrl Pts',(-3.21156188355736,1.,2.18848253363878));
#47228=CARTESIAN_POINT('Ctrl Pts',(-3.20452259717947,1.,2.18594876115914));
#47229=CARTESIAN_POINT('Ctrl Pts',(-3.197462937404,1.,2.18332898656595));
#47230=CARTESIAN_POINT('Ctrl Pts',(-3.19038924261589,1.,2.18062558031789));
#47231=CARTESIAN_POINT('Ctrl Pts',(-3.18333474627851,1.,2.17785968847172));
#47232=CARTESIAN_POINT('Ctrl Pts',(-3.17635032802584,1.,2.17506466903736));
#47233=CARTESIAN_POINT('Ctrl Pts',(-3.16948480019555,1.,2.17227212063857));
#47234=CARTESIAN_POINT('Ctrl Pts',(-3.16276685102999,1.,2.16949910801237));
#47235=CARTESIAN_POINT('Ctrl Pts',(-3.15618975593627,1.,2.1667372844767));
#47236=CARTESIAN_POINT('Ctrl Pts',(-3.14968624388961,1.,2.16393520288009));
#47237=CARTESIAN_POINT('Ctrl Pts',(-3.14314440426882,1.,2.16100905914341));
#47238=CARTESIAN_POINT('Ctrl Pts',(-3.136453565629,1.,2.15787423530583));
#47239=CARTESIAN_POINT('Ctrl Pts',(-3.12954386795575,1.,2.15447241382872));
#47240=CARTESIAN_POINT('Ctrl Pts',(-3.12242318152001,1.,2.15079698090627));
#47241=CARTESIAN_POINT('Ctrl Pts',(-3.11522827017075,1.,2.1469279845768));
#47242=CARTESIAN_POINT('Ctrl Pts',(-3.10821808669189,1.,2.14302815602195));
#47243=CARTESIAN_POINT('Ctrl Pts',(-3.1017126739137,1.,2.13930228863968));
#47244=CARTESIAN_POINT('Ctrl Pts',(-3.09604502421197,1.,2.13596538661154));
#47245=CARTESIAN_POINT('Ctrl Pts',(-3.09151235281832,1.,2.13321032560805));
#47246=CARTESIAN_POINT('Ctrl Pts',(-3.08855597949844,1.,2.13132142793056));
#47247=CARTESIAN_POINT('Ctrl Pts',(-3.08717896996213,1.,2.13034980480519));
#47248=CARTESIAN_POINT('Ctrl Pts',(-3.08668447250383,1.,2.12991938762497));
#47249=CARTESIAN_POINT('Ctrl Pts',(-3.0865713108946,1.,2.1297578506162));
#47250=CARTESIAN_POINT('Ctrl Pts',(-3.0865563332211,1.,2.12971124846838));
#47251=CARTESIAN_POINT('',(-3.54075895182139,0.,2.25898783642071));
#47252=CARTESIAN_POINT('Ctrl Pts',(-3.2988053601491,-1.,1.7833628895577));
#47253=CARTESIAN_POINT('Ctrl Pts',(-3.2988053601491,1.,1.7833628895577));
#47254=CARTESIAN_POINT('Ctrl Pts',(-3.29877974053316,-1.,1.78327971836342));
#47255=CARTESIAN_POINT('Ctrl Pts',(-3.29877974053316,1.,1.78327971836342));
#47256=CARTESIAN_POINT('Ctrl Pts',(-3.29886572077632,-1.,1.78320756177373));
#47257=CARTESIAN_POINT('Ctrl Pts',(-3.29886572077632,1.,1.78320756177373));
#47258=CARTESIAN_POINT('Ctrl Pts',(-3.29940631674303,-1.,1.7833818655594));
#47259=CARTESIAN_POINT('Ctrl Pts',(-3.29940631674303,1.,1.7833818655594));
#47260=CARTESIAN_POINT('Ctrl Pts',(-3.30095096463517,-1.,1.78417972819938));
#47261=CARTESIAN_POINT('Ctrl Pts',(-3.30095096463517,1.,1.78417972819938));
#47262=CARTESIAN_POINT('Ctrl Pts',(-3.30422155559112,-1.,1.78610045419846));
#47263=CARTESIAN_POINT('Ctrl Pts',(-3.30422155559112,1.,1.78610045419846));
#47264=CARTESIAN_POINT('Ctrl Pts',(-3.30873412266788,-1.,1.78888832245873));
#47265=CARTESIAN_POINT('Ctrl Pts',(-3.30873412266788,1.,1.78888832245873));
#47266=CARTESIAN_POINT('Ctrl Pts',(-3.31428038326424,-1.,1.79242331349949));
#47267=CARTESIAN_POINT('Ctrl Pts',(-3.31428038326424,1.,1.79242331349949));
#47268=CARTESIAN_POINT('Ctrl Pts',(-3.3205535510082,-1.,1.79652817033251));
#47269=CARTESIAN_POINT('Ctrl Pts',(-3.3205535510082,1.,1.79652817033251));
#47270=CARTESIAN_POINT('Ctrl Pts',(-3.32721088039578,-1.,1.80100380443406));
#47271=CARTESIAN_POINT('Ctrl Pts',(-3.32721088039578,1.,1.80100380443406));
#47272=CARTESIAN_POINT('Ctrl Pts',(-3.33392460276808,-1.,1.80565802981102));
#47273=CARTESIAN_POINT('Ctrl Pts',(-3.33392460276808,1.,1.80565802981102));
#47274=CARTESIAN_POINT('Ctrl Pts',(-3.34043216147606,-1.,1.81033399625352));
#47275=CARTESIAN_POINT('Ctrl Pts',(-3.34043216147606,1.,1.81033399625352));
#47276=CARTESIAN_POINT('Ctrl Pts',(-3.34660014370673,-1.,1.81494618732853));
#47277=CARTESIAN_POINT('Ctrl Pts',(-3.34660014370673,1.,1.81494618732853));
#47278=CARTESIAN_POINT('Ctrl Pts',(-3.35243086937598,-1.,1.81948458796829));
#47279=CARTESIAN_POINT('Ctrl Pts',(-3.35243086937598,1.,1.81948458796829));
#47280=CARTESIAN_POINT('Ctrl Pts',(-3.35800801557424,-1.,1.82398496829301));
#47281=CARTESIAN_POINT('Ctrl Pts',(-3.35800801557424,1.,1.82398496829301));
#47282=CARTESIAN_POINT('Ctrl Pts',(-3.36345722124158,-1.,1.82850752153199));
#47283=CARTESIAN_POINT('Ctrl Pts',(-3.36345722124158,1.,1.82850752153199));
#47284=CARTESIAN_POINT('Ctrl Pts',(-3.36890396271836,-1.,1.83311391452322));
#47285=CARTESIAN_POINT('Ctrl Pts',(-3.36890396271836,1.,1.83311391452322));
#47286=CARTESIAN_POINT('Ctrl Pts',(-3.37442462015853,-1.,1.83784072967077));
#47287=CARTESIAN_POINT('Ctrl Pts',(-3.37442462015853,1.,1.83784072967077));
#47288=CARTESIAN_POINT('Ctrl Pts',(-3.38002968341157,-1.,1.84269016931643));
#47289=CARTESIAN_POINT('Ctrl Pts',(-3.38002968341157,1.,1.84269016931643));
#47290=CARTESIAN_POINT('Ctrl Pts',(-3.38569092349592,-1.,1.84764441927753));
#47291=CARTESIAN_POINT('Ctrl Pts',(-3.38569092349592,1.,1.84764441927753));
#47292=CARTESIAN_POINT('Ctrl Pts',(-3.39135802549398,-1.,1.85267433291769));
#47293=CARTESIAN_POINT('Ctrl Pts',(-3.39135802549398,1.,1.85267433291769));
#47294=CARTESIAN_POINT('Ctrl Pts',(-3.39697816833067,-1.,1.85774972037062));
#47295=CARTESIAN_POINT('Ctrl Pts',(-3.39697816833067,1.,1.85774972037062));
#47296=CARTESIAN_POINT('Ctrl Pts',(-3.40251742305476,-1.,1.86285057051245));
#47297=CARTESIAN_POINT('Ctrl Pts',(-3.40251742305476,1.,1.86285057051245));
#47298=CARTESIAN_POINT('Ctrl Pts',(-3.40797080000549,-1.,1.86797231196654));
#47299=CARTESIAN_POINT('Ctrl Pts',(-3.40797080000549,1.,1.86797231196654));
#47300=CARTESIAN_POINT('Ctrl Pts',(-3.41335043875209,-1.,1.87311957248121));
#47301=CARTESIAN_POINT('Ctrl Pts',(-3.41335043875209,1.,1.87311957248121));
#47302=CARTESIAN_POINT('Ctrl Pts',(-3.41867858383771,-1.,1.87830245689344));
#47303=CARTESIAN_POINT('Ctrl Pts',(-3.41867858383771,1.,1.87830245689344));
#47304=CARTESIAN_POINT('Ctrl Pts',(-3.42397908819736,-1.,1.8835320506206));
#47305=CARTESIAN_POINT('Ctrl Pts',(-3.42397908819736,1.,1.8835320506206));
#47306=CARTESIAN_POINT('Ctrl Pts',(-3.42926852222158,-1.,1.88881571322009));
#47307=CARTESIAN_POINT('Ctrl Pts',(-3.42926852222158,1.,1.88881571322009));
#47308=CARTESIAN_POINT('Ctrl Pts',(-3.43455074411571,-1.,1.89415420002542));
#47309=CARTESIAN_POINT('Ctrl Pts',(-3.43455074411571,1.,1.89415420002542));
#47310=CARTESIAN_POINT('Ctrl Pts',(-3.4398218567809,-1.,1.89954426803384));
#47311=CARTESIAN_POINT('Ctrl Pts',(-3.4398218567809,1.,1.89954426803384));
#47312=CARTESIAN_POINT('Ctrl Pts',(-3.44507323983367,-1.,1.90498026502304));
#47313=CARTESIAN_POINT('Ctrl Pts',(-3.44507323983367,1.,1.90498026502304));
#47314=CARTESIAN_POINT('Ctrl Pts',(-3.45029522038888,-1.,1.91045605593639));
#47315=CARTESIAN_POINT('Ctrl Pts',(-3.45029522038888,1.,1.91045605593639));
#47316=CARTESIAN_POINT('Ctrl Pts',(-3.4554807430995,-1.,1.91596694784063));
#47317=CARTESIAN_POINT('Ctrl Pts',(-3.4554807430995,1.,1.91596694784063));
#47318=CARTESIAN_POINT('Ctrl Pts',(-3.46062821722485,-1.,1.92151118213212));
#47319=CARTESIAN_POINT('Ctrl Pts',(-3.46062821722485,1.,1.92151118213212));
#47320=CARTESIAN_POINT('Ctrl Pts',(-3.46573953254084,-1.,1.92708888591158));
#47321=CARTESIAN_POINT('Ctrl Pts',(-3.46573953254084,1.,1.92708888591158));
#47322=CARTESIAN_POINT('Ctrl Pts',(-3.47081872409781,-1.,1.93270136427081));
#47323=CARTESIAN_POINT('Ctrl Pts',(-3.47081872409781,1.,1.93270136427081));
#47324=CARTESIAN_POINT('Ctrl Pts',(-3.47587040389915,-1.,1.93835026973887));
#47325=CARTESIAN_POINT('Ctrl Pts',(-3.47587040389915,1.,1.93835026973887));
#47326=CARTESIAN_POINT('Ctrl Pts',(-3.48089825770416,-1.,1.94403680554065));
#47327=CARTESIAN_POINT('Ctrl Pts',(-3.48089825770416,1.,1.94403680554065));
#47328=CARTESIAN_POINT('Ctrl Pts',(-3.48590361610814,-1.,1.94976096795911));
#47329=CARTESIAN_POINT('Ctrl Pts',(-3.48590361610814,1.,1.94976096795911));
#47330=CARTESIAN_POINT('Ctrl Pts',(-3.49088618670987,-1.,1.95552193112084));
#47331=CARTESIAN_POINT('Ctrl Pts',(-3.49088618670987,1.,1.95552193112084));
#47332=CARTESIAN_POINT('Ctrl Pts',(-3.49584466573064,-1.,1.961318367765));
#47333=CARTESIAN_POINT('Ctrl Pts',(-3.49584466573064,1.,1.961318367765));
#47334=CARTESIAN_POINT('Ctrl Pts',(-3.50077740176267,-1.,1.96714879724052));
#47335=CARTESIAN_POINT('Ctrl Pts',(-3.50077740176267,1.,1.96714879724052));
#47336=CARTESIAN_POINT('Ctrl Pts',(-3.5056830186108,-1.,1.97301191162968));
#47337=CARTESIAN_POINT('Ctrl Pts',(-3.5056830186108,1.,1.97301191162968));
#47338=CARTESIAN_POINT('Ctrl Pts',(-3.51056110478287,-1.,1.97890693666288));
#47339=CARTESIAN_POINT('Ctrl Pts',(-3.51056110478287,1.,1.97890693666288));
#47340=CARTESIAN_POINT('Ctrl Pts',(-3.51541198728301,-1.,1.9848335106103));
#47341=CARTESIAN_POINT('Ctrl Pts',(-3.51541198728301,1.,1.9848335106103));
#47342=CARTESIAN_POINT('Ctrl Pts',(-3.52023644289142,-1.,1.99079153006112));
#47343=CARTESIAN_POINT('Ctrl Pts',(-3.52023644289142,1.,1.99079153006112));
#47344=CARTESIAN_POINT('Ctrl Pts',(-3.52503542491728,-1.,1.99678100339295));
#47345=CARTESIAN_POINT('Ctrl Pts',(-3.52503542491728,1.,1.99678100339295));
#47346=CARTESIAN_POINT('Ctrl Pts',(-3.52980980250224,-1.,2.00280191090366));
#47347=CARTESIAN_POINT('Ctrl Pts',(-3.52980980250224,1.,2.00280191090366));
#47348=CARTESIAN_POINT('Ctrl Pts',(-3.53456004727424,-1.,2.00885403604746));
#47349=CARTESIAN_POINT('Ctrl Pts',(-3.53456004727424,1.,2.00885403604746));
#47350=CARTESIAN_POINT('Ctrl Pts',(-3.53928627453642,-1.,2.01493698847351));
#47351=CARTESIAN_POINT('Ctrl Pts',(-3.53928627453642,1.,2.01493698847351));
#47352=CARTESIAN_POINT('Ctrl Pts',(-3.54398838254136,-1.,2.02105027983104));
#47353=CARTESIAN_POINT('Ctrl Pts',(-3.54398838254136,1.,2.02105027983104));
#47354=CARTESIAN_POINT('Ctrl Pts',(-3.54866616282227,-1.,2.02719338376175));
#47355=CARTESIAN_POINT('Ctrl Pts',(-3.54866616282227,1.,2.02719338376175));
#47356=CARTESIAN_POINT('Ctrl Pts',(-3.55331941293949,-1.,2.03336579658133));
#47357=CARTESIAN_POINT('Ctrl Pts',(-3.55331941293949,1.,2.03336579658133));
#47358=CARTESIAN_POINT('Ctrl Pts',(-3.55794807264844,-1.,2.03956711119976));
#47359=CARTESIAN_POINT('Ctrl Pts',(-3.55794807264844,1.,2.03956711119976));
#47360=CARTESIAN_POINT('Ctrl Pts',(-3.56255223871505,-1.,2.04579702158876));
#47361=CARTESIAN_POINT('Ctrl Pts',(-3.56255223871505,1.,2.04579702158876));
#47362=CARTESIAN_POINT('Ctrl Pts',(-3.56713209977904,-1.,2.05205528172911));
#47363=CARTESIAN_POINT('Ctrl Pts',(-3.56713209977904,1.,2.05205528172911));
#47364=CARTESIAN_POINT('Ctrl Pts',(-3.5716878942334,-1.,2.05834167687425));
#47365=CARTESIAN_POINT('Ctrl Pts',(-3.5716878942334,1.,2.05834167687425));
#47366=CARTESIAN_POINT('Ctrl Pts',(-3.57621986224402,-1.,2.06465599229234));
#47367=CARTESIAN_POINT('Ctrl Pts',(-3.57621986224402,1.,2.06465599229234));
#47368=CARTESIAN_POINT('Ctrl Pts',(-3.58072819250872,-1.,2.07099797606));
#47369=CARTESIAN_POINT('Ctrl Pts',(-3.58072819250872,1.,2.07099797606));
#47370=CARTESIAN_POINT('Ctrl Pts',(-3.58521300039988,-1.,2.07736732842524));
#47371=CARTESIAN_POINT('Ctrl Pts',(-3.58521300039988,1.,2.07736732842524));
#47372=CARTESIAN_POINT('Ctrl Pts',(-3.58967435355834,-1.,2.08376373049196));
#47373=CARTESIAN_POINT('Ctrl Pts',(-3.58967435355834,1.,2.08376373049196));
#47374=CARTESIAN_POINT('Ctrl Pts',(-3.5941122862608,-1.,2.09018686331706));
#47375=CARTESIAN_POINT('Ctrl Pts',(-3.5941122862608,1.,2.09018686331706));
#47376=CARTESIAN_POINT('Ctrl Pts',(-3.59852681775396,-1.,2.09663642986579));
#47377=CARTESIAN_POINT('Ctrl Pts',(-3.59852681775396,1.,2.09663642986579));
#47378=CARTESIAN_POINT('Ctrl Pts',(-3.60291797087849,-1.,2.10311217727687));
#47379=CARTESIAN_POINT('Ctrl Pts',(-3.60291797087849,1.,2.10311217727687));
#47380=CARTESIAN_POINT('Ctrl Pts',(-3.60728578530968,-1.,2.10961391333497));
#47381=CARTESIAN_POINT('Ctrl Pts',(-3.60728578530968,1.,2.10961391333497));
#47382=CARTESIAN_POINT('Ctrl Pts',(-3.61163030607452,-1.,2.11614149813928));
#47383=CARTESIAN_POINT('Ctrl Pts',(-3.61163030607452,1.,2.11614149813928));
#47384=CARTESIAN_POINT('Ctrl Pts',(-3.61508732215187,-1.,2.12138417125349));
#47385=CARTESIAN_POINT('Ctrl Pts',(-3.61508732215187,1.,2.12138417125349));
#47386=CARTESIAN_POINT('Ctrl Pts',(-3.61766963589442,-1.,2.12532774376144));
#47387=CARTESIAN_POINT('Ctrl Pts',(-3.61766963589442,1.,2.12532774376144));
#47388=CARTESIAN_POINT('Ctrl Pts',(-3.61938653648716,-1.,2.12796193131142));
#47389=CARTESIAN_POINT('Ctrl Pts',(-3.61938653648716,1.,2.12796193131142));
#47390=CARTESIAN_POINT('Ctrl Pts',(-3.62024382630768,-1.,2.12928030988903));
#47391=CARTESIAN_POINT('Ctrl Pts',(-3.62024382630768,1.,2.12928030988903));
#47392=CARTESIAN_POINT('',(-3.29885386921513,1.,1.78327315618341));
#47393=CARTESIAN_POINT('Ctrl Pts',(-3.29885386921513,-1.,1.78327315618341));
#47394=CARTESIAN_POINT('Ctrl Pts',(-3.29885386921513,-0.666666666666667,
1.78327315618341));
#47395=CARTESIAN_POINT('Ctrl Pts',(-3.29885386921513,-0.333333333333333,
1.78327315618341));
#47396=CARTESIAN_POINT('Ctrl Pts',(-3.29885386921513,0.333333333333333,
1.78327315618341));
#47397=CARTESIAN_POINT('Ctrl Pts',(-3.29885386921513,0.666666666666667,
1.78327315618341));
#47398=CARTESIAN_POINT('Ctrl Pts',(-3.29885386921513,1.,1.78327315618341));
#47399=CARTESIAN_POINT('',(-3.62024382630768,1.,2.12928030988903));
#47400=CARTESIAN_POINT('',(-3.62024382630768,0.,2.12928030988903));
#47401=CARTESIAN_POINT('Ctrl Pts',(-3.29885386921513,1.,1.78327315618341));
#47402=CARTESIAN_POINT('Ctrl Pts',(-3.29890219175423,1.,1.78326534445518));
#47403=CARTESIAN_POINT('Ctrl Pts',(-3.29909749657808,1.,1.78329283591905));
#47404=CARTESIAN_POINT('Ctrl Pts',(-3.299705498242,1.,1.78353803106924));
#47405=CARTESIAN_POINT('Ctrl Pts',(-3.30119637003393,1.,1.78432384788174));
#47406=CARTESIAN_POINT('Ctrl Pts',(-3.30422155559112,1.,1.78610045419846));
#47407=CARTESIAN_POINT('Ctrl Pts',(-3.30873412266788,1.,1.78888832245873));
#47408=CARTESIAN_POINT('Ctrl Pts',(-3.31428038326424,1.,1.79242331349949));
#47409=CARTESIAN_POINT('Ctrl Pts',(-3.3205535510082,1.,1.79652817033251));
#47410=CARTESIAN_POINT('Ctrl Pts',(-3.32721088039578,1.,1.80100380443406));
#47411=CARTESIAN_POINT('Ctrl Pts',(-3.33392460276808,1.,1.80565802981102));
#47412=CARTESIAN_POINT('Ctrl Pts',(-3.34043216147606,1.,1.81033399625352));
#47413=CARTESIAN_POINT('Ctrl Pts',(-3.34660014370673,1.,1.81494618732853));
#47414=CARTESIAN_POINT('Ctrl Pts',(-3.35243086937598,1.,1.81948458796829));
#47415=CARTESIAN_POINT('Ctrl Pts',(-3.35800801557424,1.,1.82398496829301));
#47416=CARTESIAN_POINT('Ctrl Pts',(-3.36345722124158,1.,1.82850752153199));
#47417=CARTESIAN_POINT('Ctrl Pts',(-3.36890396271836,1.,1.83311391452322));
#47418=CARTESIAN_POINT('Ctrl Pts',(-3.37442462015853,1.,1.83784072967077));
#47419=CARTESIAN_POINT('Ctrl Pts',(-3.38002968341157,1.,1.84269016931643));
#47420=CARTESIAN_POINT('Ctrl Pts',(-3.38569092349592,1.,1.84764441927753));
#47421=CARTESIAN_POINT('Ctrl Pts',(-3.39135802549398,1.,1.85267433291769));
#47422=CARTESIAN_POINT('Ctrl Pts',(-3.39697816833067,1.,1.85774972037062));
#47423=CARTESIAN_POINT('Ctrl Pts',(-3.40251742305476,1.,1.86285057051245));
#47424=CARTESIAN_POINT('Ctrl Pts',(-3.40797080000549,1.,1.86797231196654));
#47425=CARTESIAN_POINT('Ctrl Pts',(-3.41335043875209,1.,1.87311957248121));
#47426=CARTESIAN_POINT('Ctrl Pts',(-3.41867858383771,1.,1.87830245689344));
#47427=CARTESIAN_POINT('Ctrl Pts',(-3.42397908819736,1.,1.8835320506206));
#47428=CARTESIAN_POINT('Ctrl Pts',(-3.42926852222158,1.,1.88881571322009));
#47429=CARTESIAN_POINT('Ctrl Pts',(-3.43455074411571,1.,1.89415420002542));
#47430=CARTESIAN_POINT('Ctrl Pts',(-3.4398218567809,1.,1.89954426803384));
#47431=CARTESIAN_POINT('Ctrl Pts',(-3.44507323983367,1.,1.90498026502304));
#47432=CARTESIAN_POINT('Ctrl Pts',(-3.45029522038888,1.,1.91045605593639));
#47433=CARTESIAN_POINT('Ctrl Pts',(-3.4554807430995,1.,1.91596694784063));
#47434=CARTESIAN_POINT('Ctrl Pts',(-3.46062821722485,1.,1.92151118213212));
#47435=CARTESIAN_POINT('Ctrl Pts',(-3.46573953254084,1.,1.92708888591158));
#47436=CARTESIAN_POINT('Ctrl Pts',(-3.47081872409781,1.,1.93270136427081));
#47437=CARTESIAN_POINT('Ctrl Pts',(-3.47587040389915,1.,1.93835026973887));
#47438=CARTESIAN_POINT('Ctrl Pts',(-3.48089825770416,1.,1.94403680554065));
#47439=CARTESIAN_POINT('Ctrl Pts',(-3.48590361610814,1.,1.94976096795911));
#47440=CARTESIAN_POINT('Ctrl Pts',(-3.49088618670987,1.,1.95552193112084));
#47441=CARTESIAN_POINT('Ctrl Pts',(-3.49584466573064,1.,1.961318367765));
#47442=CARTESIAN_POINT('Ctrl Pts',(-3.50077740176267,1.,1.96714879724052));
#47443=CARTESIAN_POINT('Ctrl Pts',(-3.5056830186108,1.,1.97301191162968));
#47444=CARTESIAN_POINT('Ctrl Pts',(-3.51056110478287,1.,1.97890693666288));
#47445=CARTESIAN_POINT('Ctrl Pts',(-3.51541198728301,1.,1.9848335106103));
#47446=CARTESIAN_POINT('Ctrl Pts',(-3.52023644289142,1.,1.99079153006112));
#47447=CARTESIAN_POINT('Ctrl Pts',(-3.52503542491728,1.,1.99678100339295));
#47448=CARTESIAN_POINT('Ctrl Pts',(-3.52980980250224,1.,2.00280191090366));
#47449=CARTESIAN_POINT('Ctrl Pts',(-3.53456004727424,1.,2.00885403604746));
#47450=CARTESIAN_POINT('Ctrl Pts',(-3.53928627453642,1.,2.01493698847351));
#47451=CARTESIAN_POINT('Ctrl Pts',(-3.54398838254136,1.,2.02105027983104));
#47452=CARTESIAN_POINT('Ctrl Pts',(-3.54866616282227,1.,2.02719338376175));
#47453=CARTESIAN_POINT('Ctrl Pts',(-3.55331941293949,1.,2.03336579658133));
#47454=CARTESIAN_POINT('Ctrl Pts',(-3.55794807264844,1.,2.03956711119976));
#47455=CARTESIAN_POINT('Ctrl Pts',(-3.56255223871505,1.,2.04579702158876));
#47456=CARTESIAN_POINT('Ctrl Pts',(-3.56713209977904,1.,2.05205528172911));
#47457=CARTESIAN_POINT('Ctrl Pts',(-3.5716878942334,1.,2.05834167687425));
#47458=CARTESIAN_POINT('Ctrl Pts',(-3.57621986224402,1.,2.06465599229234));
#47459=CARTESIAN_POINT('Ctrl Pts',(-3.58072819250872,1.,2.07099797606));
#47460=CARTESIAN_POINT('Ctrl Pts',(-3.58521300039988,1.,2.07736732842524));
#47461=CARTESIAN_POINT('Ctrl Pts',(-3.58967435355834,1.,2.08376373049196));
#47462=CARTESIAN_POINT('Ctrl Pts',(-3.5941122862608,1.,2.09018686331706));
#47463=CARTESIAN_POINT('Ctrl Pts',(-3.59852681775396,1.,2.09663642986579));
#47464=CARTESIAN_POINT('Ctrl Pts',(-3.60291797087849,1.,2.10311217727687));
#47465=CARTESIAN_POINT('Ctrl Pts',(-3.60728578530968,1.,2.10961391333497));
#47466=CARTESIAN_POINT('Ctrl Pts',(-3.61163030607452,1.,2.11614149813928));
#47467=CARTESIAN_POINT('Ctrl Pts',(-3.61508732215187,1.,2.12138417125349));
#47468=CARTESIAN_POINT('Ctrl Pts',(-3.61766963589442,1.,2.12532774376144));
#47469=CARTESIAN_POINT('Ctrl Pts',(-3.61938653648716,1.,2.12796193131142));
#47470=CARTESIAN_POINT('Ctrl Pts',(-3.62024382630768,1.,2.12928030988903));
#47471=CARTESIAN_POINT('Origin',(-3.62024382630768,0.,2.12928030988903));
#47472=CARTESIAN_POINT('',(-3.54075895182139,1.,2.25898783642071));
#47473=CARTESIAN_POINT('Origin',(0.,0.,0.));
#47474=CARTESIAN_POINT('',(-3.38171594275687,1.,1.62064718014256));
#47475=CARTESIAN_POINT('Origin',(0.,1.,0.));
#47476=CARTESIAN_POINT('Ctrl Pts',(-3.38171594275687,1.,1.62064718014256));
#47477=CARTESIAN_POINT('Ctrl Pts',(-3.38171594275687,0.666666666666667,
1.62064718014256));
#47478=CARTESIAN_POINT('Ctrl Pts',(-3.38171594275687,0.333333333333333,
1.62064718014256));
#47479=CARTESIAN_POINT('Ctrl Pts',(-3.38171594275687,-0.333333333333333,
1.62064718014256));
#47480=CARTESIAN_POINT('Ctrl Pts',(-3.38171594275687,-0.666666666666667,
1.62064718014256));
#47481=CARTESIAN_POINT('Ctrl Pts',(-3.38171594275687,-1.,1.62064718014256));
#47482=CARTESIAN_POINT('Ctrl Pts',(-3.85054988729471,-1.,1.67727921511438));
#47483=CARTESIAN_POINT('Ctrl Pts',(-3.85054988729471,1.,1.67727921511438));
#47484=CARTESIAN_POINT('Ctrl Pts',(-3.84897939431104,-1.,1.6773605765671));
#47485=CARTESIAN_POINT('Ctrl Pts',(-3.84897939431104,1.,1.6773605765671));
#47486=CARTESIAN_POINT('Ctrl Pts',(-3.84583912297567,-1.,1.67751991140661));
#47487=CARTESIAN_POINT('Ctrl Pts',(-3.84583912297567,1.,1.67751991140661));
#47488=CARTESIAN_POINT('Ctrl Pts',(-3.8411308598706,-1.,1.67774874946867));
#47489=CARTESIAN_POINT('Ctrl Pts',(-3.8411308598706,1.,1.67774874946867));
#47490=CARTESIAN_POINT('Ctrl Pts',(-3.83485746516115,-1.,1.67803353065273));
#47491=CARTESIAN_POINT('Ctrl Pts',(-3.83485746516115,1.,1.67803353065273));
#47492=CARTESIAN_POINT('Ctrl Pts',(-3.82702289288453,-1.,1.67835555760094));
#47493=CARTESIAN_POINT('Ctrl Pts',(-3.82702289288453,1.,1.67835555760094));
#47494=CARTESIAN_POINT('Ctrl Pts',(-3.81919554100522,-1.,1.67864354606363));
#47495=CARTESIAN_POINT('Ctrl Pts',(-3.81919554100522,1.,1.67864354606363));
#47496=CARTESIAN_POINT('Ctrl Pts',(-3.81137549624273,-1.,1.67889737738311));
#47497=CARTESIAN_POINT('Ctrl Pts',(-3.81137549624273,1.,1.67889737738311));
#47498=CARTESIAN_POINT('Ctrl Pts',(-3.80356289078481,-1.,1.67911690648128));
#47499=CARTESIAN_POINT('Ctrl Pts',(-3.80356289078481,1.,1.67911690648128));
#47500=CARTESIAN_POINT('Ctrl Pts',(-3.7957579157763,-1.,1.67930196625203));
#47501=CARTESIAN_POINT('Ctrl Pts',(-3.7957579157763,1.,1.67930196625203));
#47502=CARTESIAN_POINT('Ctrl Pts',(-3.78796080021026,-1.,1.67945236653175));
#47503=CARTESIAN_POINT('Ctrl Pts',(-3.78796080021026,1.,1.67945236653175));
#47504=CARTESIAN_POINT('Ctrl Pts',(-3.78017178196859,-1.,1.67956789211943));
#47505=CARTESIAN_POINT('Ctrl Pts',(-3.78017178196859,1.,1.67956789211943));
#47506=CARTESIAN_POINT('Ctrl Pts',(-3.77239107928394,-1.,1.67964830084946));
#47507=CARTESIAN_POINT('Ctrl Pts',(-3.77239107928394,1.,1.67964830084946));
#47508=CARTESIAN_POINT('Ctrl Pts',(-3.76461886684523,-1.,1.67969332319322));
#47509=CARTESIAN_POINT('Ctrl Pts',(-3.76461886684523,1.,1.67969332319322));
#47510=CARTESIAN_POINT('Ctrl Pts',(-3.75685523754816,-1.,1.67970265841379));
#47511=CARTESIAN_POINT('Ctrl Pts',(-3.75685523754816,1.,1.67970265841379));
#47512=CARTESIAN_POINT('Ctrl Pts',(-3.74910022394845,-1.,1.67967598599665));
#47513=CARTESIAN_POINT('Ctrl Pts',(-3.74910022394845,1.,1.67967598599665));
#47514=CARTESIAN_POINT('Ctrl Pts',(-3.74135385965622,-1.,1.67961298685316));
#47515=CARTESIAN_POINT('Ctrl Pts',(-3.74135385965622,1.,1.67961298685316));
#47516=CARTESIAN_POINT('Ctrl Pts',(-3.73361623282617,-1.,1.67951336376434));
#47517=CARTESIAN_POINT('Ctrl Pts',(-3.73361623282617,1.,1.67951336376434));
#47518=CARTESIAN_POINT('Ctrl Pts',(-3.72588753416339,-1.,1.67937685856627));
#47519=CARTESIAN_POINT('Ctrl Pts',(-3.72588753416339,1.,1.67937685856627));
#47520=CARTESIAN_POINT('Ctrl Pts',(-3.71816812842188,-1.,1.6792032807165));
#47521=CARTESIAN_POINT('Ctrl Pts',(-3.71816812842188,1.,1.6792032807165));
#47522=CARTESIAN_POINT('Ctrl Pts',(-3.71045854208195,-1.,1.67899249793398));
#47523=CARTESIAN_POINT('Ctrl Pts',(-3.71045854208195,1.,1.67899249793398));
#47524=CARTESIAN_POINT('Ctrl Pts',(-3.70275932350998,-1.,1.6787443694862));
#47525=CARTESIAN_POINT('Ctrl Pts',(-3.70275932350998,1.,1.6787443694862));
#47526=CARTESIAN_POINT('Ctrl Pts',(-3.69507092759545,-1.,1.67845869064304));
#47527=CARTESIAN_POINT('Ctrl Pts',(-3.69507092759545,1.,1.67845869064304));
#47528=CARTESIAN_POINT('Ctrl Pts',(-3.68739360236505,-1.,1.67813513867973));
#47529=CARTESIAN_POINT('Ctrl Pts',(-3.68739360236505,1.,1.67813513867973));
#47530=CARTESIAN_POINT('Ctrl Pts',(-3.6797272457918,-1.,1.67777320475872));
#47531=CARTESIAN_POINT('Ctrl Pts',(-3.6797272457918,1.,1.67777320475872));
#47532=CARTESIAN_POINT('Ctrl Pts',(-3.67207136294639,-1.,1.67737217414901));
#47533=CARTESIAN_POINT('Ctrl Pts',(-3.67207136294639,1.,1.67737217414901));
#47534=CARTESIAN_POINT('Ctrl Pts',(-3.66442538671018,-1.,1.67693128053153));
#47535=CARTESIAN_POINT('Ctrl Pts',(-3.66442538671018,1.,1.67693128053153));
#47536=CARTESIAN_POINT('Ctrl Pts',(-3.65678894416442,-1.,1.67644983469459));
#47537=CARTESIAN_POINT('Ctrl Pts',(-3.65678894416442,1.,1.67644983469459));
#47538=CARTESIAN_POINT('Ctrl Pts',(-3.64916213574663,-1.,1.6759273594669));
#47539=CARTESIAN_POINT('Ctrl Pts',(-3.64916213574663,1.,1.6759273594669));
#47540=CARTESIAN_POINT('Ctrl Pts',(-3.6415458297232,-1.,1.67536373264839));
#47541=CARTESIAN_POINT('Ctrl Pts',(-3.6415458297232,1.,1.67536373264839));
#47542=CARTESIAN_POINT('Ctrl Pts',(-3.63394189312902,-1.,1.67475929882962));
#47543=CARTESIAN_POINT('Ctrl Pts',(-3.63394189312902,1.,1.67475929882962));
#47544=CARTESIAN_POINT('Ctrl Pts',(-3.62635249450908,-1.,1.67411452372265));
#47545=CARTESIAN_POINT('Ctrl Pts',(-3.62635249450908,1.,1.67411452372265));
#47546=CARTESIAN_POINT('Ctrl Pts',(-3.61877947398179,-1.,1.67342968196223));
#47547=CARTESIAN_POINT('Ctrl Pts',(-3.61877947398179,1.,1.67342968196223));
#47548=CARTESIAN_POINT('Ctrl Pts',(-3.61122367156182,-1.,1.67270452466968));
#47549=CARTESIAN_POINT('Ctrl Pts',(-3.61122367156182,1.,1.67270452466968));
#47550=CARTESIAN_POINT('Ctrl Pts',(-3.60368430815203,-1.,1.67193797318598));
#47551=CARTESIAN_POINT('Ctrl Pts',(-3.60368430815203,1.,1.67193797318598));
#47552=CARTESIAN_POINT('Ctrl Pts',(-3.59615824388808,-1.,1.67112775290706));
#47553=CARTESIAN_POINT('Ctrl Pts',(-3.59615824388808,1.,1.67112775290706));
#47554=CARTESIAN_POINT('Ctrl Pts',(-3.5886414309783,-1.,1.67027110397601));
#47555=CARTESIAN_POINT('Ctrl Pts',(-3.5886414309783,1.,1.67027110397601));
#47556=CARTESIAN_POINT('Ctrl Pts',(-3.58113044183823,-1.,1.66936552908228));
#47557=CARTESIAN_POINT('Ctrl Pts',(-3.58113044183823,1.,1.66936552908228));
#47558=CARTESIAN_POINT('Ctrl Pts',(-3.57362406285884,-1.,1.66840957407299));
#47559=CARTESIAN_POINT('Ctrl Pts',(-3.57362406285884,1.,1.66840957407299));
#47560=CARTESIAN_POINT('Ctrl Pts',(-3.56612465179429,-1.,1.66740349220308));
#47561=CARTESIAN_POINT('Ctrl Pts',(-3.56612465179429,1.,1.66740349220308));
#47562=CARTESIAN_POINT('Ctrl Pts',(-3.55864015233617,-1.,1.66635023293121));
#47563=CARTESIAN_POINT('Ctrl Pts',(-3.55864015233617,1.,1.66635023293121));
#47564=CARTESIAN_POINT('Ctrl Pts',(-3.5511812134288,-1.,1.66525401569004));
#47565=CARTESIAN_POINT('Ctrl Pts',(-3.5511812134288,1.,1.66525401569004));
#47566=CARTESIAN_POINT('Ctrl Pts',(-3.5437574747503,-1.,1.66411849222334));
#47567=CARTESIAN_POINT('Ctrl Pts',(-3.5437574747503,1.,1.66411849222334));
#47568=CARTESIAN_POINT('Ctrl Pts',(-3.53637385060225,-1.,1.66294490916113));
#47569=CARTESIAN_POINT('Ctrl Pts',(-3.53637385060225,1.,1.66294490916113));
#47570=CARTESIAN_POINT('Ctrl Pts',(-3.52902746211081,-1.,1.66173058912365));
#47571=CARTESIAN_POINT('Ctrl Pts',(-3.52902746211081,1.,1.66173058912365));
#47572=CARTESIAN_POINT('Ctrl Pts',(-3.52170261543787,-1.,1.66046645222266));
#47573=CARTESIAN_POINT('Ctrl Pts',(-3.52170261543787,1.,1.66046645222266));
#47574=CARTESIAN_POINT('Ctrl Pts',(-3.51437632188903,-1.,1.65913971687324));
#47575=CARTESIAN_POINT('Ctrl Pts',(-3.51437632188903,1.,1.65913971687324));
#47576=CARTESIAN_POINT('Ctrl Pts',(-3.5070273314651,-1.,1.65773832633617));
#47577=CARTESIAN_POINT('Ctrl Pts',(-3.5070273314651,1.,1.65773832633617));
#47578=CARTESIAN_POINT('Ctrl Pts',(-3.49964476477929,-1.,1.65625517961583));
#47579=CARTESIAN_POINT('Ctrl Pts',(-3.49964476477929,1.,1.65625517961583));
#47580=CARTESIAN_POINT('Ctrl Pts',(-3.49223525300194,-1.,1.65469162644476));
#47581=CARTESIAN_POINT('Ctrl Pts',(-3.49223525300194,1.,1.65469162644476));
#47582=CARTESIAN_POINT('Ctrl Pts',(-3.48483492840942,-1.,1.65306335367762));
#47583=CARTESIAN_POINT('Ctrl Pts',(-3.48483492840942,1.,1.65306335367762));
#47584=CARTESIAN_POINT('Ctrl Pts',(-3.47749926256543,-1.,1.65139534930353));
#47585=CARTESIAN_POINT('Ctrl Pts',(-3.47749926256543,1.,1.65139534930353));
#47586=CARTESIAN_POINT('Ctrl Pts',(-3.47028140996055,-1.,1.64971118698285));
#47587=CARTESIAN_POINT('Ctrl Pts',(-3.47028140996055,1.,1.64971118698285));
#47588=CARTESIAN_POINT('Ctrl Pts',(-3.46321237515029,-1.,1.64802323352752));
#47589=CARTESIAN_POINT('Ctrl Pts',(-3.46321237515029,1.,1.64802323352752));
#47590=CARTESIAN_POINT('Ctrl Pts',(-3.4562842106239,-1.,1.64632429697506));
#47591=CARTESIAN_POINT('Ctrl Pts',(-3.4562842106239,1.,1.64632429697506));
#47592=CARTESIAN_POINT('Ctrl Pts',(-3.44942242546693,-1.,1.64457408708059));
#47593=CARTESIAN_POINT('Ctrl Pts',(-3.44942242546693,1.,1.64457408708059));
#47594=CARTESIAN_POINT('Ctrl Pts',(-3.44250337701736,-1.,1.64270733821042));
#47595=CARTESIAN_POINT('Ctrl Pts',(-3.44250337701736,1.,1.64270733821042));
#47596=CARTESIAN_POINT('Ctrl Pts',(-3.43540451921397,-1.,1.64065778701952));
#47597=CARTESIAN_POINT('Ctrl Pts',(-3.43540451921397,1.,1.64065778701952));
#47598=CARTESIAN_POINT('Ctrl Pts',(-3.42804772926213,-1.,1.6383787624689));
#47599=CARTESIAN_POINT('Ctrl Pts',(-3.42804772926213,1.,1.6383787624689));
#47600=CARTESIAN_POINT('Ctrl Pts',(-3.4204397459095,-1.,1.63586250099804));
#47601=CARTESIAN_POINT('Ctrl Pts',(-3.4204397459095,1.,1.63586250099804));
#47602=CARTESIAN_POINT('Ctrl Pts',(-3.41272817148719,-1.,1.63316667054156));
#47603=CARTESIAN_POINT('Ctrl Pts',(-3.41272817148719,1.,1.63316667054156));
#47604=CARTESIAN_POINT('Ctrl Pts',(-3.40519422740596,-1.,1.63041148964996));
#47605=CARTESIAN_POINT('Ctrl Pts',(-3.40519422740596,1.,1.63041148964996));
#47606=CARTESIAN_POINT('Ctrl Pts',(-3.39818605298342,-1.,1.62774916464571));
#47607=CARTESIAN_POINT('Ctrl Pts',(-3.39818605298342,1.,1.62774916464571));
#47608=CARTESIAN_POINT('Ctrl Pts',(-3.39206617497078,-1.,1.62533996116793));
#47609=CARTESIAN_POINT('Ctrl Pts',(-3.39206617497078,1.,1.62533996116793));
#47610=CARTESIAN_POINT('Ctrl Pts',(-3.38715832178929,-1.,1.62332788556183));
#47611=CARTESIAN_POINT('Ctrl Pts',(-3.38715832178929,1.,1.62332788556183));
#47612=CARTESIAN_POINT('Ctrl Pts',(-3.38368201668123,-1.,1.62181089631134));
#47613=CARTESIAN_POINT('Ctrl Pts',(-3.38368201668123,1.,1.62181089631134));
#47614=CARTESIAN_POINT('Ctrl Pts',(-3.38212861099481,-1.,1.62103022180917));
#47615=CARTESIAN_POINT('Ctrl Pts',(-3.38212861099481,1.,1.62103022180917));
#47616=CARTESIAN_POINT('Ctrl Pts',(-3.38166984193496,-1.,1.6206953236804));
#47617=CARTESIAN_POINT('Ctrl Pts',(-3.38166984193496,1.,1.6206953236804));
#47618=CARTESIAN_POINT('Ctrl Pts',(-3.38167767992546,-1.,1.62058335162421));
#47619=CARTESIAN_POINT('Ctrl Pts',(-3.38167767992546,1.,1.62058335162421));
#47620=CARTESIAN_POINT('Ctrl Pts',(-3.38176002566879,-1.,1.62055519152808));
#47621=CARTESIAN_POINT('Ctrl Pts',(-3.38176002566879,1.,1.62055519152808));
#47622=CARTESIAN_POINT('',(-3.85054988729471,1.,1.67727921511438));
#47623=CARTESIAN_POINT('Ctrl Pts',(-3.85054988729471,1.,1.67727921511438));
#47624=CARTESIAN_POINT('Ctrl Pts',(-3.84897939431104,1.,1.6773605765671));
#47625=CARTESIAN_POINT('Ctrl Pts',(-3.84583912297567,1.,1.67751991140661));
#47626=CARTESIAN_POINT('Ctrl Pts',(-3.8411308598706,1.,1.67774874946867));
#47627=CARTESIAN_POINT('Ctrl Pts',(-3.83485746516115,1.,1.67803353065273));
#47628=CARTESIAN_POINT('Ctrl Pts',(-3.82702289288453,1.,1.67835555760094));
#47629=CARTESIAN_POINT('Ctrl Pts',(-3.81919554100522,1.,1.67864354606363));
#47630=CARTESIAN_POINT('Ctrl Pts',(-3.81137549624273,1.,1.67889737738311));
#47631=CARTESIAN_POINT('Ctrl Pts',(-3.80356289078481,1.,1.67911690648128));
#47632=CARTESIAN_POINT('Ctrl Pts',(-3.7957579157763,1.,1.67930196625203));
#47633=CARTESIAN_POINT('Ctrl Pts',(-3.78796080021026,1.,1.67945236653175));
#47634=CARTESIAN_POINT('Ctrl Pts',(-3.78017178196859,1.,1.67956789211943));
#47635=CARTESIAN_POINT('Ctrl Pts',(-3.77239107928394,1.,1.67964830084946));
#47636=CARTESIAN_POINT('Ctrl Pts',(-3.76461886684523,1.,1.67969332319322));
#47637=CARTESIAN_POINT('Ctrl Pts',(-3.75685523754816,1.,1.67970265841379));
#47638=CARTESIAN_POINT('Ctrl Pts',(-3.74910022394845,1.,1.67967598599665));
#47639=CARTESIAN_POINT('Ctrl Pts',(-3.74135385965622,1.,1.67961298685316));
#47640=CARTESIAN_POINT('Ctrl Pts',(-3.73361623282617,1.,1.67951336376434));
#47641=CARTESIAN_POINT('Ctrl Pts',(-3.72588753416339,1.,1.67937685856627));
#47642=CARTESIAN_POINT('Ctrl Pts',(-3.71816812842188,1.,1.6792032807165));
#47643=CARTESIAN_POINT('Ctrl Pts',(-3.71045854208195,1.,1.67899249793398));
#47644=CARTESIAN_POINT('Ctrl Pts',(-3.70275932350998,1.,1.6787443694862));
#47645=CARTESIAN_POINT('Ctrl Pts',(-3.69507092759545,1.,1.67845869064304));
#47646=CARTESIAN_POINT('Ctrl Pts',(-3.68739360236505,1.,1.67813513867973));
#47647=CARTESIAN_POINT('Ctrl Pts',(-3.6797272457918,1.,1.67777320475872));
#47648=CARTESIAN_POINT('Ctrl Pts',(-3.67207136294639,1.,1.67737217414901));
#47649=CARTESIAN_POINT('Ctrl Pts',(-3.66442538671018,1.,1.67693128053153));
#47650=CARTESIAN_POINT('Ctrl Pts',(-3.65678894416442,1.,1.67644983469459));
#47651=CARTESIAN_POINT('Ctrl Pts',(-3.64916213574663,1.,1.6759273594669));
#47652=CARTESIAN_POINT('Ctrl Pts',(-3.6415458297232,1.,1.67536373264839));
#47653=CARTESIAN_POINT('Ctrl Pts',(-3.63394189312902,1.,1.67475929882962));
#47654=CARTESIAN_POINT('Ctrl Pts',(-3.62635249450908,1.,1.67411452372265));
#47655=CARTESIAN_POINT('Ctrl Pts',(-3.61877947398179,1.,1.67342968196223));
#47656=CARTESIAN_POINT('Ctrl Pts',(-3.61122367156182,1.,1.67270452466968));
#47657=CARTESIAN_POINT('Ctrl Pts',(-3.60368430815203,1.,1.67193797318598));
#47658=CARTESIAN_POINT('Ctrl Pts',(-3.59615824388808,1.,1.67112775290706));
#47659=CARTESIAN_POINT('Ctrl Pts',(-3.5886414309783,1.,1.67027110397601));
#47660=CARTESIAN_POINT('Ctrl Pts',(-3.58113044183823,1.,1.66936552908228));
#47661=CARTESIAN_POINT('Ctrl Pts',(-3.57362406285884,1.,1.66840957407299));
#47662=CARTESIAN_POINT('Ctrl Pts',(-3.56612465179429,1.,1.66740349220308));
#47663=CARTESIAN_POINT('Ctrl Pts',(-3.55864015233617,1.,1.66635023293121));
#47664=CARTESIAN_POINT('Ctrl Pts',(-3.5511812134288,1.,1.66525401569004));
#47665=CARTESIAN_POINT('Ctrl Pts',(-3.5437574747503,1.,1.66411849222334));
#47666=CARTESIAN_POINT('Ctrl Pts',(-3.53637385060225,1.,1.66294490916113));
#47667=CARTESIAN_POINT('Ctrl Pts',(-3.52902746211081,1.,1.66173058912365));
#47668=CARTESIAN_POINT('Ctrl Pts',(-3.52170261543787,1.,1.66046645222266));
#47669=CARTESIAN_POINT('Ctrl Pts',(-3.51437632188903,1.,1.65913971687324));
#47670=CARTESIAN_POINT('Ctrl Pts',(-3.5070273314651,1.,1.65773832633617));
#47671=CARTESIAN_POINT('Ctrl Pts',(-3.49964476477929,1.,1.65625517961583));
#47672=CARTESIAN_POINT('Ctrl Pts',(-3.49223525300194,1.,1.65469162644476));
#47673=CARTESIAN_POINT('Ctrl Pts',(-3.48483492840942,1.,1.65306335367762));
#47674=CARTESIAN_POINT('Ctrl Pts',(-3.47749926256543,1.,1.65139534930353));
#47675=CARTESIAN_POINT('Ctrl Pts',(-3.47028140996055,1.,1.64971118698285));
#47676=CARTESIAN_POINT('Ctrl Pts',(-3.46321237515029,1.,1.64802323352752));
#47677=CARTESIAN_POINT('Ctrl Pts',(-3.4562842106239,1.,1.64632429697506));
#47678=CARTESIAN_POINT('Ctrl Pts',(-3.44942242546693,1.,1.64457408708059));
#47679=CARTESIAN_POINT('Ctrl Pts',(-3.44250337701736,1.,1.64270733821042));
#47680=CARTESIAN_POINT('Ctrl Pts',(-3.43540451921397,1.,1.64065778701952));
#47681=CARTESIAN_POINT('Ctrl Pts',(-3.42804772926213,1.,1.6383787624689));
#47682=CARTESIAN_POINT('Ctrl Pts',(-3.4204397459095,1.,1.63586250099804));
#47683=CARTESIAN_POINT('Ctrl Pts',(-3.41272817148719,1.,1.63316667054156));
#47684=CARTESIAN_POINT('Ctrl Pts',(-3.40519422740596,1.,1.63041148964996));
#47685=CARTESIAN_POINT('Ctrl Pts',(-3.39818605298342,1.,1.62774916464571));
#47686=CARTESIAN_POINT('Ctrl Pts',(-3.39206617497078,1.,1.62533996116793));
#47687=CARTESIAN_POINT('Ctrl Pts',(-3.38715832178929,1.,1.62332788556183));
#47688=CARTESIAN_POINT('Ctrl Pts',(-3.3839428576331,1.,1.62192472202795));
#47689=CARTESIAN_POINT('Ctrl Pts',(-3.38243080602536,1.,1.62118047294574));
#47690=CARTESIAN_POINT('Ctrl Pts',(-3.38187506457001,1.,1.62083271136059));
#47691=CARTESIAN_POINT('Ctrl Pts',(-3.38173802621243,1.,1.62069086551626));
#47692=CARTESIAN_POINT('Ctrl Pts',(-3.38171594275687,1.,1.62064718014256));
#47693=CARTESIAN_POINT('',(-3.85054988729471,0.,1.67727921511438));
#47694=CARTESIAN_POINT('Ctrl Pts',(-3.53717101171257,-1.,1.24535988127942));
#47695=CARTESIAN_POINT('Ctrl Pts',(-3.53717101171257,1.,1.24535988127942));
#47696=CARTESIAN_POINT('Ctrl Pts',(-3.53713269667534,-1.,1.24528174185147));
#47697=CARTESIAN_POINT('Ctrl Pts',(-3.53713269667534,1.,1.24528174185147));
#47698=CARTESIAN_POINT('Ctrl Pts',(-3.53720633058152,-1.,1.2451970233558));
#47699=CARTESIAN_POINT('Ctrl Pts',(-3.53720633058152,1.,1.2451970233558));
#47700=CARTESIAN_POINT('Ctrl Pts',(-3.53776753803428,-1.,1.24528461333177));
#47701=CARTESIAN_POINT('Ctrl Pts',(-3.53776753803428,1.,1.24528461333177));
#47702=CARTESIAN_POINT('Ctrl Pts',(-3.53941798196293,-1.,1.24583101679199));
#47703=CARTESIAN_POINT('Ctrl Pts',(-3.53941798196293,1.,1.24583101679199));
#47704=CARTESIAN_POINT('Ctrl Pts',(-3.54294877426113,-1.,1.2472164623202));
#47705=CARTESIAN_POINT('Ctrl Pts',(-3.54294877426113,1.,1.2472164623202));
#47706=CARTESIAN_POINT('Ctrl Pts',(-3.54784190282889,-1.,1.24926408627938));
#47707=CARTESIAN_POINT('Ctrl Pts',(-3.54784190282889,1.,1.24926408627938));
#47708=CARTESIAN_POINT('Ctrl Pts',(-3.5538728741862,-1.,1.25188792940508));
#47709=CARTESIAN_POINT('Ctrl Pts',(-3.5538728741862,1.,1.25188792940508));
#47710=CARTESIAN_POINT('Ctrl Pts',(-3.56071094990825,-1.,1.25496090899873));
#47711=CARTESIAN_POINT('Ctrl Pts',(-3.56071094990825,1.,1.25496090899873));
#47712=CARTESIAN_POINT('Ctrl Pts',(-3.56798645995025,-1.,1.25834000485626));
#47713=CARTESIAN_POINT('Ctrl Pts',(-3.56798645995025,1.,1.25834000485626));
#47714=CARTESIAN_POINT('Ctrl Pts',(-3.5753456065164,-1.,1.26188667142784));
#47715=CARTESIAN_POINT('Ctrl Pts',(-3.5753456065164,1.,1.26188667142784));
#47716=CARTESIAN_POINT('Ctrl Pts',(-3.58250452868699,-1.,1.26548706249891));
#47717=CARTESIAN_POINT('Ctrl Pts',(-3.58250452868699,1.,1.26548706249891));
#47718=CARTESIAN_POINT('Ctrl Pts',(-3.5893180784647,-1.,1.26907758484766));
#47719=CARTESIAN_POINT('Ctrl Pts',(-3.5893180784647,1.,1.26907758484766));
#47720=CARTESIAN_POINT('Ctrl Pts',(-3.59578698050164,-1.,1.27264798379365));
#47721=CARTESIAN_POINT('Ctrl Pts',(-3.59578698050164,1.,1.27264798379365));
#47722=CARTESIAN_POINT('Ctrl Pts',(-3.60199947736404,-1.,1.27622049908664));
#47723=CARTESIAN_POINT('Ctrl Pts',(-3.60199947736404,1.,1.27622049908664));
#47724=CARTESIAN_POINT('Ctrl Pts',(-3.60808907746372,-1.,1.27983492861703));
#47725=CARTESIAN_POINT('Ctrl Pts',(-3.60808907746372,1.,1.27983492861703));
#47726=CARTESIAN_POINT('Ctrl Pts',(-3.61418935913793,-1.,1.28353255117754));
#47727=CARTESIAN_POINT('Ctrl Pts',(-3.61418935913793,1.,1.28353255117754));
#47728=CARTESIAN_POINT('Ctrl Pts',(-3.62038148492295,-1.,1.2873375502936));
#47729=CARTESIAN_POINT('Ctrl Pts',(-3.62038148492295,1.,1.2873375502936));
#47730=CARTESIAN_POINT('Ctrl Pts',(-3.62667616004299,-1.,1.29125046021853));
#47731=CARTESIAN_POINT('Ctrl Pts',(-3.62667616004299,1.,1.29125046021853));
#47732=CARTESIAN_POINT('Ctrl Pts',(-3.63304271630995,-1.,1.29525810207744));
#47733=CARTESIAN_POINT('Ctrl Pts',(-3.63304271630995,1.,1.29525810207744));
#47734=CARTESIAN_POINT('Ctrl Pts',(-3.6394268987279,-1.,1.29933955906463));
#47735=CARTESIAN_POINT('Ctrl Pts',(-3.6394268987279,1.,1.29933955906463));
#47736=CARTESIAN_POINT('Ctrl Pts',(-3.64577181380125,-1.,1.30347327603778));
#47737=CARTESIAN_POINT('Ctrl Pts',(-3.64577181380125,1.,1.30347327603778));
#47738=CARTESIAN_POINT('Ctrl Pts',(-3.65204081987101,-1.,1.30764479590051));
#47739=CARTESIAN_POINT('Ctrl Pts',(-3.65204081987101,1.,1.30764479590051));
#47740=CARTESIAN_POINT('Ctrl Pts',(-3.65822827358655,-1.,1.31185038411231));
#47741=CARTESIAN_POINT('Ctrl Pts',(-3.65822827358655,1.,1.31185038411231));
#47742=CARTESIAN_POINT('Ctrl Pts',(-3.66434688899822,-1.,1.31609271239922));
#47743=CARTESIAN_POINT('Ctrl Pts',(-3.66434688899822,1.,1.31609271239922));
#47744=CARTESIAN_POINT('Ctrl Pts',(-3.67042021752668,-1.,1.3203782813777));
#47745=CARTESIAN_POINT('Ctrl Pts',(-3.67042021752668,1.,1.3203782813777));
#47746=CARTESIAN_POINT('Ctrl Pts',(-3.67647355257906,-1.,1.32471430856413));
#47747=CARTESIAN_POINT('Ctrl Pts',(-3.67647355257906,1.,1.32471430856413));
#47748=CARTESIAN_POINT('Ctrl Pts',(-3.68252441182534,-1.,1.32910547072734));
#47749=CARTESIAN_POINT('Ctrl Pts',(-3.68252441182534,1.,1.32910547072734));
#47750=CARTESIAN_POINT('Ctrl Pts',(-3.68857672413013,-1.,1.33355191034515));
#47751=CARTESIAN_POINT('Ctrl Pts',(-3.68857672413013,1.,1.33355191034515));
#47752=CARTESIAN_POINT('Ctrl Pts',(-3.69462613305692,-1.,1.33805103398214));
#47753=CARTESIAN_POINT('Ctrl Pts',(-3.69462613305692,1.,1.33805103398214));
#47754=CARTESIAN_POINT('Ctrl Pts',(-3.70066324015112,-1.,1.3425986075293));
#47755=CARTESIAN_POINT('Ctrl Pts',(-3.70066324015112,1.,1.3425986075293));
#47756=CARTESIAN_POINT('Ctrl Pts',(-3.7066775318825,-1.,1.34719008463535));
#47757=CARTESIAN_POINT('Ctrl Pts',(-3.7066775318825,1.,1.34719008463535));
#47758=CARTESIAN_POINT('Ctrl Pts',(-3.71266130563061,-1.,1.35182193384426));
#47759=CARTESIAN_POINT('Ctrl Pts',(-3.71266130563061,1.,1.35182193384426));
#47760=CARTESIAN_POINT('Ctrl Pts',(-3.71861271513318,-1.,1.35649266705038));
#47761=CARTESIAN_POINT('Ctrl Pts',(-3.71861271513318,1.,1.35649266705038));
#47762=CARTESIAN_POINT('Ctrl Pts',(-3.72453364678279,-1.,1.36120211416353));
#47763=CARTESIAN_POINT('Ctrl Pts',(-3.72453364678279,1.,1.36120211416353));
#47764=CARTESIAN_POINT('Ctrl Pts',(-3.73042829011293,-1.,1.36595093298674));
#47765=CARTESIAN_POINT('Ctrl Pts',(-3.73042829011293,1.,1.36595093298674));
#47766=CARTESIAN_POINT('Ctrl Pts',(-3.73630145885809,-1.,1.37074003422739));
#47767=CARTESIAN_POINT('Ctrl Pts',(-3.73630145885809,1.,1.37074003422739));
#47768=CARTESIAN_POINT('Ctrl Pts',(-3.7421569816256,-1.,1.3755700297169));
#47769=CARTESIAN_POINT('Ctrl Pts',(-3.7421569816256,1.,1.3755700297169));
#47770=CARTESIAN_POINT('Ctrl Pts',(-3.74799617204744,-1.,1.38044070763302));
#47771=CARTESIAN_POINT('Ctrl Pts',(-3.74799617204744,1.,1.38044070763302));
#47772=CARTESIAN_POINT('Ctrl Pts',(-3.75381861212728,-1.,1.38535129801185));
#47773=CARTESIAN_POINT('Ctrl Pts',(-3.75381861212728,1.,1.38535129801185));
#47774=CARTESIAN_POINT('Ctrl Pts',(-3.75962280650875,-1.,1.39030069388926));
#47775=CARTESIAN_POINT('Ctrl Pts',(-3.75962280650875,1.,1.39030069388926));
#47776=CARTESIAN_POINT('Ctrl Pts',(-3.76540689249078,-1.,1.39528769118054));
#47777=CARTESIAN_POINT('Ctrl Pts',(-3.76540689249078,1.,1.39528769118054));
#47778=CARTESIAN_POINT('Ctrl Pts',(-3.77116930621804,-1.,1.40031121335495));
#47779=CARTESIAN_POINT('Ctrl Pts',(-3.77116930621804,1.,1.40031121335495));
#47780=CARTESIAN_POINT('Ctrl Pts',(-3.77690952014209,-1.,1.40537056004702));
#47781=CARTESIAN_POINT('Ctrl Pts',(-3.77690952014209,1.,1.40537056004702));
#47782=CARTESIAN_POINT('Ctrl Pts',(-3.78262780065406,-1.,1.41046532282567));
#47783=CARTESIAN_POINT('Ctrl Pts',(-3.78262780065406,1.,1.41046532282567));
#47784=CARTESIAN_POINT('Ctrl Pts',(-3.78832489879369,-1.,1.41559527803808));
#47785=CARTESIAN_POINT('Ctrl Pts',(-3.78832489879369,1.,1.41559527803808));
#47786=CARTESIAN_POINT('Ctrl Pts',(-3.7940017574439,-1.,1.42076028482828));
#47787=CARTESIAN_POINT('Ctrl Pts',(-3.7940017574439,1.,1.42076028482828));
#47788=CARTESIAN_POINT('Ctrl Pts',(-3.79965923196365,-1.,1.42596018777301));
#47789=CARTESIAN_POINT('Ctrl Pts',(-3.79965923196365,1.,1.42596018777301));
#47790=CARTESIAN_POINT('Ctrl Pts',(-3.80529775429916,-1.,1.43119469921364));
#47791=CARTESIAN_POINT('Ctrl Pts',(-3.80529775429916,1.,1.43119469921364));
#47792=CARTESIAN_POINT('Ctrl Pts',(-3.81091737726965,-1.,1.43646341556783));
#47793=CARTESIAN_POINT('Ctrl Pts',(-3.81091737726965,1.,1.43646341556783));
#47794=CARTESIAN_POINT('Ctrl Pts',(-3.8165179239855,-1.,1.441765870414));
#47795=CARTESIAN_POINT('Ctrl Pts',(-3.8165179239855,1.,1.441765870414));
#47796=CARTESIAN_POINT('Ctrl Pts',(-3.82209910620591,-1.,1.44710157648562));
#47797=CARTESIAN_POINT('Ctrl Pts',(-3.82209910620591,1.,1.44710157648562));
#47798=CARTESIAN_POINT('Ctrl Pts',(-3.82766064519,-1.,1.45247006796807));
#47799=CARTESIAN_POINT('Ctrl Pts',(-3.82766064519,1.,1.45247006796807));
#47800=CARTESIAN_POINT('Ctrl Pts',(-3.83320241775199,-1.,1.45787095220763));
#47801=CARTESIAN_POINT('Ctrl Pts',(-3.83320241775199,1.,1.45787095220763));
#47802=CARTESIAN_POINT('Ctrl Pts',(-3.83872447159309,-1.,1.46330391180621));
#47803=CARTESIAN_POINT('Ctrl Pts',(-3.83872447159309,1.,1.46330391180621));
#47804=CARTESIAN_POINT('Ctrl Pts',(-3.84422695454469,-1.,1.46876867426374));
#47805=CARTESIAN_POINT('Ctrl Pts',(-3.84422695454469,1.,1.46876867426374));
#47806=CARTESIAN_POINT('Ctrl Pts',(-3.84971006847096,-1.,1.47426499018467));
#47807=CARTESIAN_POINT('Ctrl Pts',(-3.84971006847096,1.,1.47426499018467));
#47808=CARTESIAN_POINT('Ctrl Pts',(-3.85517401698952,-1.,1.47979260991063));
#47809=CARTESIAN_POINT('Ctrl Pts',(-3.85517401698952,1.,1.47979260991063));
#47810=CARTESIAN_POINT('Ctrl Pts',(-3.86061894706551,-1.,1.48535125510102));
#47811=CARTESIAN_POINT('Ctrl Pts',(-3.86061894706551,1.,1.48535125510102));
#47812=CARTESIAN_POINT('Ctrl Pts',(-3.86604492575933,-1.,1.49094061164604));
#47813=CARTESIAN_POINT('Ctrl Pts',(-3.86604492575933,1.,1.49094061164604));
#47814=CARTESIAN_POINT('Ctrl Pts',(-3.8714519699927,-1.,1.4965603539944));
#47815=CARTESIAN_POINT('Ctrl Pts',(-3.8714519699927,1.,1.4965603539944));
#47816=CARTESIAN_POINT('Ctrl Pts',(-3.87684006372665,-1.,1.50221016176766));
#47817=CARTESIAN_POINT('Ctrl Pts',(-3.87684006372665,1.,1.50221016176766));
#47818=CARTESIAN_POINT('Ctrl Pts',(-3.88220917950443,-1.,1.50788973857719));
#47819=CARTESIAN_POINT('Ctrl Pts',(-3.88220917950443,1.,1.50788973857719));
#47820=CARTESIAN_POINT('Ctrl Pts',(-3.88755930032927,-1.,1.51359883110181));
#47821=CARTESIAN_POINT('Ctrl Pts',(-3.88755930032927,1.,1.51359883110181));
#47822=CARTESIAN_POINT('Ctrl Pts',(-3.89289043531893,-1.,1.51933724328609));
#47823=CARTESIAN_POINT('Ctrl Pts',(-3.89289043531893,1.,1.51933724328609));
#47824=CARTESIAN_POINT('Ctrl Pts',(-3.8982026070607,-1.,1.52510482990784));
#47825=CARTESIAN_POINT('Ctrl Pts',(-3.8982026070607,1.,1.52510482990784));
#47826=CARTESIAN_POINT('Ctrl Pts',(-3.90243719629755,-1.,1.5297421605556));
#47827=CARTESIAN_POINT('Ctrl Pts',(-3.90243719629755,1.,1.5297421605556));
#47828=CARTESIAN_POINT('Ctrl Pts',(-3.90560462812846,-1.,1.53323321827311));
#47829=CARTESIAN_POINT('Ctrl Pts',(-3.90560462812846,1.,1.53323321827311));
#47830=CARTESIAN_POINT('Ctrl Pts',(-3.90771246854607,-1.,1.53556639217742));
#47831=CARTESIAN_POINT('Ctrl Pts',(-3.90771246854607,1.,1.53556639217742));
#47832=CARTESIAN_POINT('Ctrl Pts',(-3.90876544355381,-1.,1.53673442965255));
#47833=CARTESIAN_POINT('Ctrl Pts',(-3.90876544355381,1.,1.53673442965255));
#47834=CARTESIAN_POINT('',(-3.5372048861591,1.,1.24526366418208));
#47835=CARTESIAN_POINT('Ctrl Pts',(-3.5372048861591,-1.,1.24526366418208));
#47836=CARTESIAN_POINT('Ctrl Pts',(-3.5372048861591,-0.666666666666667,
1.24526366418208));
#47837=CARTESIAN_POINT('Ctrl Pts',(-3.5372048861591,-0.333333333333333,
1.24526366418208));
#47838=CARTESIAN_POINT('Ctrl Pts',(-3.5372048861591,0.333333333333333,1.24526366418208));
#47839=CARTESIAN_POINT('Ctrl Pts',(-3.5372048861591,0.666666666666667,1.24526366418208));
#47840=CARTESIAN_POINT('Ctrl Pts',(-3.5372048861591,1.,1.24526366418208));
#47841=CARTESIAN_POINT('',(-3.90876544355381,1.,1.53673442965255));
#47842=CARTESIAN_POINT('',(-3.90876544355381,0.,1.53673442965255));
#47843=CARTESIAN_POINT('Ctrl Pts',(-3.5372048861591,1.,1.24526366418208));
#47844=CARTESIAN_POINT('Ctrl Pts',(-3.53725139174402,1.,1.24524838931864));
#47845=CARTESIAN_POINT('Ctrl Pts',(-3.53744859265385,1.,1.24524498991133));
#47846=CARTESIAN_POINT('Ctrl Pts',(-3.53808746578052,1.,1.2453920538873));
#47847=CARTESIAN_POINT('Ctrl Pts',(-3.53968291129942,1.,1.24593497225964));
#47848=CARTESIAN_POINT('Ctrl Pts',(-3.54294877426113,1.,1.2472164623202));
#47849=CARTESIAN_POINT('Ctrl Pts',(-3.54784190282889,1.,1.24926408627938));
#47850=CARTESIAN_POINT('Ctrl Pts',(-3.5538728741862,1.,1.25188792940508));
#47851=CARTESIAN_POINT('Ctrl Pts',(-3.56071094990825,1.,1.25496090899873));
#47852=CARTESIAN_POINT('Ctrl Pts',(-3.56798645995025,1.,1.25834000485626));
#47853=CARTESIAN_POINT('Ctrl Pts',(-3.5753456065164,1.,1.26188667142784));
#47854=CARTESIAN_POINT('Ctrl Pts',(-3.58250452868699,1.,1.26548706249891));
#47855=CARTESIAN_POINT('Ctrl Pts',(-3.5893180784647,1.,1.26907758484766));
#47856=CARTESIAN_POINT('Ctrl Pts',(-3.59578698050164,1.,1.27264798379365));
#47857=CARTESIAN_POINT('Ctrl Pts',(-3.60199947736404,1.,1.27622049908664));
#47858=CARTESIAN_POINT('Ctrl Pts',(-3.60808907746372,1.,1.27983492861703));
#47859=CARTESIAN_POINT('Ctrl Pts',(-3.61418935913793,1.,1.28353255117754));
#47860=CARTESIAN_POINT('Ctrl Pts',(-3.62038148492295,1.,1.2873375502936));
#47861=CARTESIAN_POINT('Ctrl Pts',(-3.62667616004299,1.,1.29125046021853));
#47862=CARTESIAN_POINT('Ctrl Pts',(-3.63304271630995,1.,1.29525810207744));
#47863=CARTESIAN_POINT('Ctrl Pts',(-3.6394268987279,1.,1.29933955906463));
#47864=CARTESIAN_POINT('Ctrl Pts',(-3.64577181380125,1.,1.30347327603778));
#47865=CARTESIAN_POINT('Ctrl Pts',(-3.65204081987101,1.,1.30764479590051));
#47866=CARTESIAN_POINT('Ctrl Pts',(-3.65822827358655,1.,1.31185038411231));
#47867=CARTESIAN_POINT('Ctrl Pts',(-3.66434688899822,1.,1.31609271239922));
#47868=CARTESIAN_POINT('Ctrl Pts',(-3.67042021752668,1.,1.3203782813777));
#47869=CARTESIAN_POINT('Ctrl Pts',(-3.67647355257906,1.,1.32471430856413));
#47870=CARTESIAN_POINT('Ctrl Pts',(-3.68252441182534,1.,1.32910547072734));
#47871=CARTESIAN_POINT('Ctrl Pts',(-3.68857672413013,1.,1.33355191034515));
#47872=CARTESIAN_POINT('Ctrl Pts',(-3.69462613305692,1.,1.33805103398214));
#47873=CARTESIAN_POINT('Ctrl Pts',(-3.70066324015112,1.,1.3425986075293));
#47874=CARTESIAN_POINT('Ctrl Pts',(-3.7066775318825,1.,1.34719008463535));
#47875=CARTESIAN_POINT('Ctrl Pts',(-3.71266130563061,1.,1.35182193384426));
#47876=CARTESIAN_POINT('Ctrl Pts',(-3.71861271513318,1.,1.35649266705038));
#47877=CARTESIAN_POINT('Ctrl Pts',(-3.72453364678279,1.,1.36120211416353));
#47878=CARTESIAN_POINT('Ctrl Pts',(-3.73042829011293,1.,1.36595093298674));
#47879=CARTESIAN_POINT('Ctrl Pts',(-3.73630145885809,1.,1.37074003422739));
#47880=CARTESIAN_POINT('Ctrl Pts',(-3.7421569816256,1.,1.3755700297169));
#47881=CARTESIAN_POINT('Ctrl Pts',(-3.74799617204744,1.,1.38044070763302));
#47882=CARTESIAN_POINT('Ctrl Pts',(-3.75381861212728,1.,1.38535129801185));
#47883=CARTESIAN_POINT('Ctrl Pts',(-3.75962280650875,1.,1.39030069388926));
#47884=CARTESIAN_POINT('Ctrl Pts',(-3.76540689249078,1.,1.39528769118054));
#47885=CARTESIAN_POINT('Ctrl Pts',(-3.77116930621804,1.,1.40031121335495));
#47886=CARTESIAN_POINT('Ctrl Pts',(-3.77690952014209,1.,1.40537056004702));
#47887=CARTESIAN_POINT('Ctrl Pts',(-3.78262780065406,1.,1.41046532282567));
#47888=CARTESIAN_POINT('Ctrl Pts',(-3.78832489879369,1.,1.41559527803808));
#47889=CARTESIAN_POINT('Ctrl Pts',(-3.7940017574439,1.,1.42076028482828));
#47890=CARTESIAN_POINT('Ctrl Pts',(-3.79965923196365,1.,1.42596018777301));
#47891=CARTESIAN_POINT('Ctrl Pts',(-3.80529775429916,1.,1.43119469921364));
#47892=CARTESIAN_POINT('Ctrl Pts',(-3.81091737726965,1.,1.43646341556783));
#47893=CARTESIAN_POINT('Ctrl Pts',(-3.8165179239855,1.,1.441765870414));
#47894=CARTESIAN_POINT('Ctrl Pts',(-3.82209910620591,1.,1.44710157648562));
#47895=CARTESIAN_POINT('Ctrl Pts',(-3.82766064519,1.,1.45247006796807));
#47896=CARTESIAN_POINT('Ctrl Pts',(-3.83320241775199,1.,1.45787095220763));
#47897=CARTESIAN_POINT('Ctrl Pts',(-3.83872447159309,1.,1.46330391180621));
#47898=CARTESIAN_POINT('Ctrl Pts',(-3.84422695454469,1.,1.46876867426374));
#47899=CARTESIAN_POINT('Ctrl Pts',(-3.84971006847096,1.,1.47426499018467));
#47900=CARTESIAN_POINT('Ctrl Pts',(-3.85517401698952,1.,1.47979260991063));
#47901=CARTESIAN_POINT('Ctrl Pts',(-3.86061894706551,1.,1.48535125510102));
#47902=CARTESIAN_POINT('Ctrl Pts',(-3.86604492575933,1.,1.49094061164604));
#47903=CARTESIAN_POINT('Ctrl Pts',(-3.8714519699927,1.,1.4965603539944));
#47904=CARTESIAN_POINT('Ctrl Pts',(-3.87684006372665,1.,1.50221016176766));
#47905=CARTESIAN_POINT('Ctrl Pts',(-3.88220917950443,1.,1.50788973857719));
#47906=CARTESIAN_POINT('Ctrl Pts',(-3.88755930032927,1.,1.51359883110181));
#47907=CARTESIAN_POINT('Ctrl Pts',(-3.89289043531893,1.,1.51933724328609));
#47908=CARTESIAN_POINT('Ctrl Pts',(-3.8982026070607,1.,1.52510482990784));
#47909=CARTESIAN_POINT('Ctrl Pts',(-3.90243719629755,1.,1.5297421605556));
#47910=CARTESIAN_POINT('Ctrl Pts',(-3.90560462812846,1.,1.53323321827311));
#47911=CARTESIAN_POINT('Ctrl Pts',(-3.90771246854607,1.,1.53556639217742));
#47912=CARTESIAN_POINT('Ctrl Pts',(-3.90876544355381,1.,1.53673442965255));
#47913=CARTESIAN_POINT('Origin',(-3.90876544355381,0.,1.53673442965255));
#47914=CARTESIAN_POINT('',(-3.85054988729471,1.,1.67727921511438));
#47915=CARTESIAN_POINT('Origin',(0.,0.,0.));
#47916=CARTESIAN_POINT('',(-3.59360648251021,1.,1.071677399622));
#47917=CARTESIAN_POINT('Origin',(0.,1.,0.));
#47918=CARTESIAN_POINT('Ctrl Pts',(-3.59360648251021,1.,1.071677399622));
#47919=CARTESIAN_POINT('Ctrl Pts',(-3.59360648251021,0.666666666666667,
1.071677399622));
#47920=CARTESIAN_POINT('Ctrl Pts',(-3.59360648251021,0.333333333333333,
1.071677399622));
#47921=CARTESIAN_POINT('Ctrl Pts',(-3.59360648251021,-0.333333333333333,
1.071677399622));
#47922=CARTESIAN_POINT('Ctrl Pts',(-3.59360648251021,-0.666666666666667,
1.071677399622));
#47923=CARTESIAN_POINT('Ctrl Pts',(-3.59360648251021,-1.,1.071677399622));
#47924=CARTESIAN_POINT('Ctrl Pts',(-4.06552750530042,-1.,1.05427041296137));
#47925=CARTESIAN_POINT('Ctrl Pts',(-4.06552750530042,1.,1.05427041296137));
#47926=CARTESIAN_POINT('Ctrl Pts',(-4.06398907542679,-1.,1.05459645194934));
#47927=CARTESIAN_POINT('Ctrl Pts',(-4.06398907542679,1.,1.05459645194934));
#47928=CARTESIAN_POINT('Ctrl Pts',(-4.06091239150293,-1.,1.05524507177901));
#47929=CARTESIAN_POINT('Ctrl Pts',(-4.06091239150293,1.,1.05524507177901));
#47930=CARTESIAN_POINT('Ctrl Pts',(-4.05629789308941,-1.,1.0562076270849));
#47931=CARTESIAN_POINT('Ctrl Pts',(-4.05629789308941,1.,1.0562076270849));
#47932=CARTESIAN_POINT('Ctrl Pts',(-4.05014628387112,-1.,1.05747027728537));
#47933=CARTESIAN_POINT('Ctrl Pts',(-4.05014628387112,1.,1.05747027728537));
#47934=CARTESIAN_POINT('Ctrl Pts',(-4.04245854429333,-1.,1.05901393667039));
#47935=CARTESIAN_POINT('Ctrl Pts',(-4.04245854429333,1.,1.05901393667039));
#47936=CARTESIAN_POINT('Ctrl Pts',(-4.03477261142549,-1.,1.06052284712114));
#47937=CARTESIAN_POINT('Ctrl Pts',(-4.03477261142549,1.,1.06052284712114));
#47938=CARTESIAN_POINT('Ctrl Pts',(-4.02708855235732,-1.,1.06199687787488));
#47939=CARTESIAN_POINT('Ctrl Pts',(-4.02708855235732,1.,1.06199687787488));
#47940=CARTESIAN_POINT('Ctrl Pts',(-4.0194064749539,-1.,1.06343586496094));
#47941=CARTESIAN_POINT('Ctrl Pts',(-4.0194064749539,1.,1.06343586496094));
#47942=CARTESIAN_POINT('Ctrl Pts',(-4.0117265418656,-1.,1.06483961342894));
#47943=CARTESIAN_POINT('Ctrl Pts',(-4.0117265418656,1.,1.06483961342894));
#47944=CARTESIAN_POINT('Ctrl Pts',(-4.00404894951804,-1.,1.06620789963406));
#47945=CARTESIAN_POINT('Ctrl Pts',(-4.00404894951804,1.,1.06620789963406));
#47946=CARTESIAN_POINT('Ctrl Pts',(-3.99637389919958,-1.,1.06754047381188));
#47947=CARTESIAN_POINT('Ctrl Pts',(-3.99637389919958,1.,1.06754047381188));
#47948=CARTESIAN_POINT('Ctrl Pts',(-3.98870156857298,-1.,1.06883706263912));
#47949=CARTESIAN_POINT('Ctrl Pts',(-3.98870156857298,1.,1.06883706263912));
#47950=CARTESIAN_POINT('Ctrl Pts',(-3.98103208801289,-1.,1.07009737257815));
#47951=CARTESIAN_POINT('Ctrl Pts',(-3.98103208801289,1.,1.07009737257815));
#47952=CARTESIAN_POINT('Ctrl Pts',(-3.97336550222571,-1.,1.07132109206252));
#47953=CARTESIAN_POINT('Ctrl Pts',(-3.97336550222571,1.,1.07132109206252));
#47954=CARTESIAN_POINT('Ctrl Pts',(-3.96570179322681,-1.,1.07250789943095));
#47955=CARTESIAN_POINT('Ctrl Pts',(-3.96570179322681,1.,1.07250789943095));
#47956=CARTESIAN_POINT('Ctrl Pts',(-3.95804094429606,-1.,1.07365747426551));
#47957=CARTESIAN_POINT('Ctrl Pts',(-3.95804094429606,1.,1.07365747426551));
#47958=CARTESIAN_POINT('Ctrl Pts',(-3.95038299600754,-1.,1.07476950921607));
#47959=CARTESIAN_POINT('Ctrl Pts',(-3.95038299600754,1.,1.07476950921607));
#47960=CARTESIAN_POINT('Ctrl Pts',(-3.94272809633271,-1.,1.07584371946428));
#47961=CARTESIAN_POINT('Ctrl Pts',(-3.94272809633271,1.,1.07584371946428));
#47962=CARTESIAN_POINT('Ctrl Pts',(-3.93507657572743,-1.,1.07687985975348));
#47963=CARTESIAN_POINT('Ctrl Pts',(-3.93507657572743,1.,1.07687985975348));
#47964=CARTESIAN_POINT('Ctrl Pts',(-3.92742893349684,-1.,1.07787771707155));
#47965=CARTESIAN_POINT('Ctrl Pts',(-3.92742893349684,1.,1.07787771707155));
#47966=CARTESIAN_POINT('Ctrl Pts',(-3.91978568924062,-1.,1.07883706663524));
#47967=CARTESIAN_POINT('Ctrl Pts',(-3.91978568924062,1.,1.07883706663524));
#47968=CARTESIAN_POINT('Ctrl Pts',(-3.91214726022096,-1.,1.0797576350746));
#47969=CARTESIAN_POINT('Ctrl Pts',(-3.91214726022096,1.,1.0797576350746));
#47970=CARTESIAN_POINT('Ctrl Pts',(-3.90451384092564,-1.,1.08063906483822));
#47971=CARTESIAN_POINT('Ctrl Pts',(-3.90451384092564,1.,1.08063906483822));
#47972=CARTESIAN_POINT('Ctrl Pts',(-3.89688525098408,-1.,1.08148086931373));
#47973=CARTESIAN_POINT('Ctrl Pts',(-3.89688525098408,1.,1.08148086931373));
#47974=CARTESIAN_POINT('Ctrl Pts',(-3.88926088975182,-1.,1.08228241999363));
#47975=CARTESIAN_POINT('Ctrl Pts',(-3.88926088975182,1.,1.08228241999363));
#47976=CARTESIAN_POINT('Ctrl Pts',(-3.88164007721365,-1.,1.08304304871042));
#47977=CARTESIAN_POINT('Ctrl Pts',(-3.88164007721365,1.,1.08304304871042));
#47978=CARTESIAN_POINT('Ctrl Pts',(-3.87402233722563,-1.,1.0837621330751));
#47979=CARTESIAN_POINT('Ctrl Pts',(-3.87402233722563,1.,1.0837621330751));
#47980=CARTESIAN_POINT('Ctrl Pts',(-3.86640769434269,-1.,1.08443918607926));
#47981=CARTESIAN_POINT('Ctrl Pts',(-3.86640769434269,1.,1.08443918607926));
#47982=CARTESIAN_POINT('Ctrl Pts',(-3.85879698702511,-1.,1.08507395120054));
#47983=CARTESIAN_POINT('Ctrl Pts',(-3.85879698702511,1.,1.08507395120054));
#47984=CARTESIAN_POINT('Ctrl Pts',(-3.85119211322732,-1.,1.08566647671838));
#47985=CARTESIAN_POINT('Ctrl Pts',(-3.85119211322732,1.,1.08566647671838));
#47986=CARTESIAN_POINT('Ctrl Pts',(-3.84359528764934,-1.,1.08621688337601));
#47987=CARTESIAN_POINT('Ctrl Pts',(-3.84359528764934,1.,1.08621688337601));
#47988=CARTESIAN_POINT('Ctrl Pts',(-3.83600837071702,-1.,1.08672515456901));
#47989=CARTESIAN_POINT('Ctrl Pts',(-3.83600837071702,1.,1.08672515456901));
#47990=CARTESIAN_POINT('Ctrl Pts',(-3.82843215316985,-1.,1.08719091307558));
#47991=CARTESIAN_POINT('Ctrl Pts',(-3.82843215316985,1.,1.08719091307558));
#47992=CARTESIAN_POINT('Ctrl Pts',(-3.82086569676321,-1.,1.08761321539442));
#47993=CARTESIAN_POINT('Ctrl Pts',(-3.82086569676321,1.,1.08761321539442));
#47994=CARTESIAN_POINT('Ctrl Pts',(-3.81330554446324,-1.,1.08799030610861));
#47995=CARTESIAN_POINT('Ctrl Pts',(-3.81330554446324,1.,1.08799030610861));
#47996=CARTESIAN_POINT('Ctrl Pts',(-3.80574726657656,-1.,1.08832009255378));
#47997=CARTESIAN_POINT('Ctrl Pts',(-3.80574726657656,1.,1.08832009255378));
#47998=CARTESIAN_POINT('Ctrl Pts',(-3.79818708705252,-1.,1.08860064435776));
#47999=CARTESIAN_POINT('Ctrl Pts',(-3.79818708705252,1.,1.08860064435776));
#48000=CARTESIAN_POINT('Ctrl Pts',(-3.79062357974401,-1.,1.08883071512097));
#48001=CARTESIAN_POINT('Ctrl Pts',(-3.79062357974401,1.,1.08883071512097));
#48002=CARTESIAN_POINT('Ctrl Pts',(-3.78305911299511,-1.,1.08901018614638));
#48003=CARTESIAN_POINT('Ctrl Pts',(-3.78305911299511,1.,1.08901018614638));
#48004=CARTESIAN_POINT('Ctrl Pts',(-3.7755019940944,-1.,1.08914072791275));
#48005=CARTESIAN_POINT('Ctrl Pts',(-3.7755019940944,1.,1.08914072791275));
#48006=CARTESIAN_POINT('Ctrl Pts',(-3.76796340094469,-1.,1.08922484204263));
#48007=CARTESIAN_POINT('Ctrl Pts',(-3.76796340094469,1.,1.08922484204263));
#48008=CARTESIAN_POINT('Ctrl Pts',(-3.76045342580226,-1.,1.08926462734287));
#48009=CARTESIAN_POINT('Ctrl Pts',(-3.76045342580226,1.,1.08926462734287));
#48010=CARTESIAN_POINT('Ctrl Pts',(-3.75297711748138,-1.,1.08926054632927));
#48011=CARTESIAN_POINT('Ctrl Pts',(-3.75297711748138,1.,1.08926054632927));
#48012=CARTESIAN_POINT('Ctrl Pts',(-3.74553121371745,-1.,1.08921040494013));
#48013=CARTESIAN_POINT('Ctrl Pts',(-3.74553121371745,1.,1.08921040494013));
#48014=CARTESIAN_POINT('Ctrl Pts',(-3.73809879348209,-1.,1.08910769013288));
#48015=CARTESIAN_POINT('Ctrl Pts',(-3.73809879348209,1.,1.08910769013288));
#48016=CARTESIAN_POINT('Ctrl Pts',(-3.73065515162949,-1.,1.08894337390925));
#48017=CARTESIAN_POINT('Ctrl Pts',(-3.73065515162949,1.,1.08894337390925));
#48018=CARTESIAN_POINT('Ctrl Pts',(-3.72317741369364,-1.,1.08870887220072));
#48019=CARTESIAN_POINT('Ctrl Pts',(-3.72317741369364,1.,1.08870887220072));
#48020=CARTESIAN_POINT('Ctrl Pts',(-3.71565372339063,-1.,1.08839887334776));
#48021=CARTESIAN_POINT('Ctrl Pts',(-3.71565372339063,1.,1.08839887334776));
#48022=CARTESIAN_POINT('Ctrl Pts',(-3.70809084139476,-1.,1.0880136731219));
#48023=CARTESIAN_POINT('Ctrl Pts',(-3.70809084139476,1.,1.0880136731219));
#48024=CARTESIAN_POINT('Ctrl Pts',(-3.70052690909884,-1.,1.08756311291324));
#48025=CARTESIAN_POINT('Ctrl Pts',(-3.70052690909884,1.,1.08756311291324));
#48026=CARTESIAN_POINT('Ctrl Pts',(-3.69302062410229,-1.,1.08706319540291));
#48027=CARTESIAN_POINT('Ctrl Pts',(-3.69302062410229,1.,1.08706319540291));
#48028=CARTESIAN_POINT('Ctrl Pts',(-3.68562817420864,-1.,1.08652888882609));
#48029=CARTESIAN_POINT('Ctrl Pts',(-3.68562817420864,1.,1.08652888882609));
#48030=CARTESIAN_POINT('Ctrl Pts',(-3.67838211685148,-1.,1.08596755755768));
#48031=CARTESIAN_POINT('Ctrl Pts',(-3.67838211685148,1.,1.08596755755768));
#48032=CARTESIAN_POINT('Ctrl Pts',(-3.67127347729632,-1.,1.0853733414448));
#48033=CARTESIAN_POINT('Ctrl Pts',(-3.67127347729632,1.,1.0853733414448));
#48034=CARTESIAN_POINT('Ctrl Pts',(-3.66422237895256,-1.,1.0847180992287));
#48035=CARTESIAN_POINT('Ctrl Pts',(-3.66422237895256,1.,1.0847180992287));
#48036=CARTESIAN_POINT('Ctrl Pts',(-3.65709649161004,-1.,1.08395671077761));
#48037=CARTESIAN_POINT('Ctrl Pts',(-3.65709649161004,1.,1.08395671077761));
#48038=CARTESIAN_POINT('Ctrl Pts',(-3.64976441208197,-1.,1.08304289898577));
#48039=CARTESIAN_POINT('Ctrl Pts',(-3.64976441208197,1.,1.08304289898577));
#48040=CARTESIAN_POINT('Ctrl Pts',(-3.64214167843595,-1.,1.08194278850972));
#48041=CARTESIAN_POINT('Ctrl Pts',(-3.64214167843595,1.,1.08194278850972));
#48042=CARTESIAN_POINT('Ctrl Pts',(-3.63423373196602,-1.,1.08064765719887));
#48043=CARTESIAN_POINT('Ctrl Pts',(-3.63423373196602,1.,1.08064765719887));
#48044=CARTESIAN_POINT('Ctrl Pts',(-3.62619537902616,-1.,1.07919137290815));
#48045=CARTESIAN_POINT('Ctrl Pts',(-3.62619537902616,1.,1.07919137290815));
#48046=CARTESIAN_POINT('Ctrl Pts',(-3.61832318504957,-1.,1.07764868137729));
#48047=CARTESIAN_POINT('Ctrl Pts',(-3.61832318504957,1.,1.07764868137729));
#48048=CARTESIAN_POINT('Ctrl Pts',(-3.61098481349577,-1.,1.07611545402841));
#48049=CARTESIAN_POINT('Ctrl Pts',(-3.61098481349577,1.,1.07611545402841));
#48050=CARTESIAN_POINT('Ctrl Pts',(-3.6045633988796,-1.,1.0746932716863));
#48051=CARTESIAN_POINT('Ctrl Pts',(-3.6045633988796,1.,1.0746932716863));
#48052=CARTESIAN_POINT('Ctrl Pts',(-3.59940121154383,-1.,1.0734737254567));
#48053=CARTESIAN_POINT('Ctrl Pts',(-3.59940121154383,1.,1.0734737254567));
#48054=CARTESIAN_POINT('Ctrl Pts',(-3.59573039611837,-1.,1.07251922679108));
#48055=CARTESIAN_POINT('Ctrl Pts',(-3.59573039611837,1.,1.07251922679108));
#48056=CARTESIAN_POINT('Ctrl Pts',(-3.59407399103556,-1.,1.07199116987503));
#48057=CARTESIAN_POINT('Ctrl Pts',(-3.59407399103556,1.,1.07199116987503));
#48058=CARTESIAN_POINT('Ctrl Pts',(-3.59356848057451,-1.,1.07173216219041));
#48059=CARTESIAN_POINT('Ctrl Pts',(-3.59356848057451,1.,1.07173216219041));
#48060=CARTESIAN_POINT('Ctrl Pts',(-3.59355870577763,-1.,1.07162034256419));
#48061=CARTESIAN_POINT('Ctrl Pts',(-3.59355870577763,1.,1.07162034256419));
#48062=CARTESIAN_POINT('Ctrl Pts',(-3.59363563249864,-1.,1.07157964745328));
#48063=CARTESIAN_POINT('Ctrl Pts',(-3.59363563249864,1.,1.07157964745328));
#48064=CARTESIAN_POINT('',(-4.06552750530042,1.,1.05427041296137));
#48065=CARTESIAN_POINT('Ctrl Pts',(-4.06552750530042,1.,1.05427041296137));
#48066=CARTESIAN_POINT('Ctrl Pts',(-4.06398907542679,1.,1.05459645194934));
#48067=CARTESIAN_POINT('Ctrl Pts',(-4.06091239150293,1.,1.05524507177901));
#48068=CARTESIAN_POINT('Ctrl Pts',(-4.05629789308941,1.,1.0562076270849));
#48069=CARTESIAN_POINT('Ctrl Pts',(-4.05014628387112,1.,1.05747027728537));
#48070=CARTESIAN_POINT('Ctrl Pts',(-4.04245854429333,1.,1.05901393667039));
#48071=CARTESIAN_POINT('Ctrl Pts',(-4.03477261142549,1.,1.06052284712114));
#48072=CARTESIAN_POINT('Ctrl Pts',(-4.02708855235732,1.,1.06199687787488));
#48073=CARTESIAN_POINT('Ctrl Pts',(-4.0194064749539,1.,1.06343586496094));
#48074=CARTESIAN_POINT('Ctrl Pts',(-4.0117265418656,1.,1.06483961342894));
#48075=CARTESIAN_POINT('Ctrl Pts',(-4.00404894951804,1.,1.06620789963406));
#48076=CARTESIAN_POINT('Ctrl Pts',(-3.99637389919958,1.,1.06754047381188));
#48077=CARTESIAN_POINT('Ctrl Pts',(-3.98870156857298,1.,1.06883706263912));
#48078=CARTESIAN_POINT('Ctrl Pts',(-3.98103208801289,1.,1.07009737257815));
#48079=CARTESIAN_POINT('Ctrl Pts',(-3.97336550222571,1.,1.07132109206252));
#48080=CARTESIAN_POINT('Ctrl Pts',(-3.96570179322681,1.,1.07250789943095));
#48081=CARTESIAN_POINT('Ctrl Pts',(-3.95804094429606,1.,1.07365747426551));
#48082=CARTESIAN_POINT('Ctrl Pts',(-3.95038299600754,1.,1.07476950921607));
#48083=CARTESIAN_POINT('Ctrl Pts',(-3.94272809633271,1.,1.07584371946428));
#48084=CARTESIAN_POINT('Ctrl Pts',(-3.93507657572743,1.,1.07687985975348));
#48085=CARTESIAN_POINT('Ctrl Pts',(-3.92742893349684,1.,1.07787771707155));
#48086=CARTESIAN_POINT('Ctrl Pts',(-3.91978568924062,1.,1.07883706663524));
#48087=CARTESIAN_POINT('Ctrl Pts',(-3.91214726022096,1.,1.0797576350746));
#48088=CARTESIAN_POINT('Ctrl Pts',(-3.90451384092564,1.,1.08063906483822));
#48089=CARTESIAN_POINT('Ctrl Pts',(-3.89688525098408,1.,1.08148086931373));
#48090=CARTESIAN_POINT('Ctrl Pts',(-3.88926088975182,1.,1.08228241999363));
#48091=CARTESIAN_POINT('Ctrl Pts',(-3.88164007721365,1.,1.08304304871042));
#48092=CARTESIAN_POINT('Ctrl Pts',(-3.87402233722563,1.,1.0837621330751));
#48093=CARTESIAN_POINT('Ctrl Pts',(-3.86640769434269,1.,1.08443918607926));
#48094=CARTESIAN_POINT('Ctrl Pts',(-3.85879698702511,1.,1.08507395120054));
#48095=CARTESIAN_POINT('Ctrl Pts',(-3.85119211322732,1.,1.08566647671838));
#48096=CARTESIAN_POINT('Ctrl Pts',(-3.84359528764934,1.,1.08621688337601));
#48097=CARTESIAN_POINT('Ctrl Pts',(-3.83600837071702,1.,1.08672515456901));
#48098=CARTESIAN_POINT('Ctrl Pts',(-3.82843215316985,1.,1.08719091307558));
#48099=CARTESIAN_POINT('Ctrl Pts',(-3.82086569676321,1.,1.08761321539442));
#48100=CARTESIAN_POINT('Ctrl Pts',(-3.81330554446324,1.,1.08799030610861));
#48101=CARTESIAN_POINT('Ctrl Pts',(-3.80574726657656,1.,1.08832009255378));
#48102=CARTESIAN_POINT('Ctrl Pts',(-3.79818708705252,1.,1.08860064435776));
#48103=CARTESIAN_POINT('Ctrl Pts',(-3.79062357974401,1.,1.08883071512097));
#48104=CARTESIAN_POINT('Ctrl Pts',(-3.78305911299511,1.,1.08901018614638));
#48105=CARTESIAN_POINT('Ctrl Pts',(-3.7755019940944,1.,1.08914072791275));
#48106=CARTESIAN_POINT('Ctrl Pts',(-3.76796340094469,1.,1.08922484204263));
#48107=CARTESIAN_POINT('Ctrl Pts',(-3.76045342580226,1.,1.08926462734287));
#48108=CARTESIAN_POINT('Ctrl Pts',(-3.75297711748138,1.,1.08926054632927));
#48109=CARTESIAN_POINT('Ctrl Pts',(-3.74553121371745,1.,1.08921040494013));
#48110=CARTESIAN_POINT('Ctrl Pts',(-3.73809879348209,1.,1.08910769013288));
#48111=CARTESIAN_POINT('Ctrl Pts',(-3.73065515162949,1.,1.08894337390925));
#48112=CARTESIAN_POINT('Ctrl Pts',(-3.72317741369364,1.,1.08870887220072));
#48113=CARTESIAN_POINT('Ctrl Pts',(-3.71565372339063,1.,1.08839887334776));
#48114=CARTESIAN_POINT('Ctrl Pts',(-3.70809084139476,1.,1.0880136731219));
#48115=CARTESIAN_POINT('Ctrl Pts',(-3.70052690909884,1.,1.08756311291324));
#48116=CARTESIAN_POINT('Ctrl Pts',(-3.69302062410229,1.,1.08706319540291));
#48117=CARTESIAN_POINT('Ctrl Pts',(-3.68562817420864,1.,1.08652888882609));
#48118=CARTESIAN_POINT('Ctrl Pts',(-3.67838211685148,1.,1.08596755755768));
#48119=CARTESIAN_POINT('Ctrl Pts',(-3.67127347729632,1.,1.0853733414448));
#48120=CARTESIAN_POINT('Ctrl Pts',(-3.66422237895256,1.,1.0847180992287));
#48121=CARTESIAN_POINT('Ctrl Pts',(-3.65709649161004,1.,1.08395671077761));
#48122=CARTESIAN_POINT('Ctrl Pts',(-3.64976441208197,1.,1.08304289898577));
#48123=CARTESIAN_POINT('Ctrl Pts',(-3.64214167843595,1.,1.08194278850972));
#48124=CARTESIAN_POINT('Ctrl Pts',(-3.63423373196602,1.,1.08064765719887));
#48125=CARTESIAN_POINT('Ctrl Pts',(-3.62619537902616,1.,1.07919137290815));
#48126=CARTESIAN_POINT('Ctrl Pts',(-3.61832318504957,1.,1.07764868137729));
#48127=CARTESIAN_POINT('Ctrl Pts',(-3.61098481349577,1.,1.07611545402841));
#48128=CARTESIAN_POINT('Ctrl Pts',(-3.6045633988796,1.,1.0746932716863));
#48129=CARTESIAN_POINT('Ctrl Pts',(-3.59940121154383,1.,1.0734737254567));
#48130=CARTESIAN_POINT('Ctrl Pts',(-3.59600583195037,1.,1.07259084660947));
#48131=CARTESIAN_POINT('Ctrl Pts',(-3.59439597,1.,1.07209229745284));
#48132=CARTESIAN_POINT('Ctrl Pts',(-3.59379266874663,1.,1.07183575450716));
#48133=CARTESIAN_POINT('Ctrl Pts',(-3.59363512797985,1.,1.07171709254271));
#48134=CARTESIAN_POINT('Ctrl Pts',(-3.59360648251021,1.,1.071677399622));
#48135=CARTESIAN_POINT('',(-4.06552750530042,0.,1.05427041296137));
#48136=CARTESIAN_POINT('Ctrl Pts',(-3.68843977377012,-1.,0.676691979611561));
#48137=CARTESIAN_POINT('Ctrl Pts',(-3.68843977377012,1.,0.676691979611561));
#48138=CARTESIAN_POINT('Ctrl Pts',(-3.68838970675497,-1.,0.676620796001989));
#48139=CARTESIAN_POINT('Ctrl Pts',(-3.68838970675497,1.,0.676620796001989));
#48140=CARTESIAN_POINT('Ctrl Pts',(-3.68844918121303,-1.,0.676525601650855));
#48141=CARTESIAN_POINT('Ctrl Pts',(-3.68844918121303,1.,0.676525601650855));
#48142=CARTESIAN_POINT('Ctrl Pts',(-3.68901718136181,-1.,0.676524321061226));
#48143=CARTESIAN_POINT('Ctrl Pts',(-3.68901718136181,1.,0.676524321061226));
#48144=CARTESIAN_POINT('Ctrl Pts',(-3.69073278191994,-1.,0.67680581107509));
#48145=CARTESIAN_POINT('Ctrl Pts',(-3.69073278191994,1.,0.67680581107509));
#48146=CARTESIAN_POINT('Ctrl Pts',(-3.69443683573598,-1.,0.677621861865498));
#48147=CARTESIAN_POINT('Ctrl Pts',(-3.69443683573598,1.,0.677621861865498));
#48148=CARTESIAN_POINT('Ctrl Pts',(-3.69959004073005,-1.,0.678878822226026));
#48149=CARTESIAN_POINT('Ctrl Pts',(-3.69959004073005,1.,0.678878822226026));
#48150=CARTESIAN_POINT('Ctrl Pts',(-3.70595722031785,-1.,0.680526909710877));
#48151=CARTESIAN_POINT('Ctrl Pts',(-3.70595722031785,1.,0.680526909710877));
#48152=CARTESIAN_POINT('Ctrl Pts',(-3.71319182789943,-1.,0.68249234510893));
#48153=CARTESIAN_POINT('Ctrl Pts',(-3.71319182789943,1.,0.68249234510893));
#48154=CARTESIAN_POINT('Ctrl Pts',(-3.7209063713926,-1.,0.684691698167848));
#48155=CARTESIAN_POINT('Ctrl Pts',(-3.7209063713926,1.,0.684691698167848));
#48156=CARTESIAN_POINT('Ctrl Pts',(-3.72872973554051,-1.,0.687043475232354));
#48157=CARTESIAN_POINT('Ctrl Pts',(-3.72872973554051,1.,0.687043475232354));
#48158=CARTESIAN_POINT('Ctrl Pts',(-3.73636374475077,-1.,0.689479637354813));
#48159=CARTESIAN_POINT('Ctrl Pts',(-3.73636374475077,1.,0.689479637354813));
#48160=CARTESIAN_POINT('Ctrl Pts',(-3.74365508986712,-1.,0.69196008040082));
#48161=CARTESIAN_POINT('Ctrl Pts',(-3.74365508986712,1.,0.69196008040082));
#48162=CARTESIAN_POINT('Ctrl Pts',(-3.75060288243455,-1.,0.694474562581492));
#48163=CARTESIAN_POINT('Ctrl Pts',(-3.75060288243455,1.,0.694474562581492));
#48164=CARTESIAN_POINT('Ctrl Pts',(-3.75729775767023,-1.,0.697031245659743));
#48165=CARTESIAN_POINT('Ctrl Pts',(-3.75729775767023,1.,0.697031245659743));
#48166=CARTESIAN_POINT('Ctrl Pts',(-3.76387780603759,-1.,0.699648552230917));
#48167=CARTESIAN_POINT('Ctrl Pts',(-3.76387780603759,1.,0.699648552230917));
#48168=CARTESIAN_POINT('Ctrl Pts',(-3.77048141872872,-1.,0.702346356621551));
#48169=CARTESIAN_POINT('Ctrl Pts',(-3.77048141872872,1.,0.702346356621551));
#48170=CARTESIAN_POINT('Ctrl Pts',(-3.77719254217129,-1.,0.705135847999816));
#48171=CARTESIAN_POINT('Ctrl Pts',(-3.77719254217129,1.,0.705135847999816));
#48172=CARTESIAN_POINT('Ctrl Pts',(-3.78402183336605,-1.,0.708015879375459));
#48173=CARTESIAN_POINT('Ctrl Pts',(-3.78402183336605,1.,0.708015879375459));
#48174=CARTESIAN_POINT('Ctrl Pts',(-3.79093694007094,-1.,0.710978231689017));
#48175=CARTESIAN_POINT('Ctrl Pts',(-3.79093694007094,1.,0.710978231689017));
#48176=CARTESIAN_POINT('Ctrl Pts',(-3.79788100314975,-1.,0.71401073300664));
#48177=CARTESIAN_POINT('Ctrl Pts',(-3.79788100314975,1.,0.71401073300664));
#48178=CARTESIAN_POINT('Ctrl Pts',(-3.80479445759309,-1.,0.717100993669114));
#48179=CARTESIAN_POINT('Ctrl Pts',(-3.80479445759309,1.,0.717100993669114));
#48180=CARTESIAN_POINT('Ctrl Pts',(-3.81163885127344,-1.,0.720240466589236));
#48181=CARTESIAN_POINT('Ctrl Pts',(-3.81163885127344,1.,0.720240466589236));
#48182=CARTESIAN_POINT('Ctrl Pts',(-3.81840802610835,-1.,0.723426346019422));
#48183=CARTESIAN_POINT('Ctrl Pts',(-3.81840802610835,1.,0.723426346019422));
#48184=CARTESIAN_POINT('Ctrl Pts',(-3.82511495756713,-1.,0.726659281876664));
#48185=CARTESIAN_POINT('Ctrl Pts',(-3.82511495756713,1.,0.726659281876664));
#48186=CARTESIAN_POINT('Ctrl Pts',(-3.83178392403383,-1.,0.729942010490167));
#48187=CARTESIAN_POINT('Ctrl Pts',(-3.83178392403383,1.,0.729942010490167));
#48188=CARTESIAN_POINT('Ctrl Pts',(-3.83844103658009,-1.,0.733277703756078));
#48189=CARTESIAN_POINT('Ctrl Pts',(-3.83844103658009,1.,0.733277703756078));
#48190=CARTESIAN_POINT('Ctrl Pts',(-3.84510432881213,-1.,0.736668240497117));
#48191=CARTESIAN_POINT('Ctrl Pts',(-3.84510432881213,1.,0.736668240497117));
#48192=CARTESIAN_POINT('Ctrl Pts',(-3.85177770351216,-1.,0.740113146827137));
#48193=CARTESIAN_POINT('Ctrl Pts',(-3.85177770351216,1.,0.740113146827137));
#48194=CARTESIAN_POINT('Ctrl Pts',(-3.85845645217594,-1.,0.743610542737012));
#48195=CARTESIAN_POINT('Ctrl Pts',(-3.85845645217594,1.,0.743610542737012));
#48196=CARTESIAN_POINT('Ctrl Pts',(-3.86513062969889,-1.,0.747157716488871));
#48197=CARTESIAN_POINT('Ctrl Pts',(-3.86513062969889,1.,0.747157716488871));
#48198=CARTESIAN_POINT('Ctrl Pts',(-3.87178914078374,-1.,0.750751822383027));
#48199=CARTESIAN_POINT('Ctrl Pts',(-3.87178914078374,1.,0.750751822383027));
#48200=CARTESIAN_POINT('Ctrl Pts',(-3.87842382520065,-1.,0.754390577396856));
#48201=CARTESIAN_POINT('Ctrl Pts',(-3.87842382520065,1.,0.754390577396856));
#48202=CARTESIAN_POINT('Ctrl Pts',(-3.88503262662689,-1.,0.758072800564801));
#48203=CARTESIAN_POINT('Ctrl Pts',(-3.88503262662689,1.,0.758072800564801));
#48204=CARTESIAN_POINT('Ctrl Pts',(-3.89161738162245,-1.,0.761798028793969));
#48205=CARTESIAN_POINT('Ctrl Pts',(-3.89161738162245,1.,0.761798028793969));
#48206=CARTESIAN_POINT('Ctrl Pts',(-3.89818233104378,-1.,0.765566256401295));
#48207=CARTESIAN_POINT('Ctrl Pts',(-3.89818233104378,1.,0.765566256401295));
#48208=CARTESIAN_POINT('Ctrl Pts',(-3.90473237182633,-1.,0.769377629847874));
#48209=CARTESIAN_POINT('Ctrl Pts',(-3.90473237182633,1.,0.769377629847874));
#48210=CARTESIAN_POINT('Ctrl Pts',(-3.91127138115243,-1.,0.773232154506321));
#48211=CARTESIAN_POINT('Ctrl Pts',(-3.91127138115243,1.,0.773232154506321));
#48212=CARTESIAN_POINT('Ctrl Pts',(-3.9178006233448,-1.,0.777129415664956));
#48213=CARTESIAN_POINT('Ctrl Pts',(-3.9178006233448,1.,0.777129415664956));
#48214=CARTESIAN_POINT('Ctrl Pts',(-3.92431956510441,-1.,0.781068718228451));
#48215=CARTESIAN_POINT('Ctrl Pts',(-3.92431956510441,1.,0.781068718228451));
#48216=CARTESIAN_POINT('Ctrl Pts',(-3.93082655631789,-1.,0.785049202786507));
#48217=CARTESIAN_POINT('Ctrl Pts',(-3.93082655631789,1.,0.785049202786507));
#48218=CARTESIAN_POINT('Ctrl Pts',(-3.93731956885676,-1.,0.789069971469333));
#48219=CARTESIAN_POINT('Ctrl Pts',(-3.93731956885676,1.,0.789069971469333));
#48220=CARTESIAN_POINT('Ctrl Pts',(-3.94379688971283,-1.,0.793130205640961));
#48221=CARTESIAN_POINT('Ctrl Pts',(-3.94379688971283,1.,0.793130205640961));
#48222=CARTESIAN_POINT('Ctrl Pts',(-3.95025788827136,-1.,0.797229296085315));
#48223=CARTESIAN_POINT('Ctrl Pts',(-3.95025788827136,1.,0.797229296085315));
#48224=CARTESIAN_POINT('Ctrl Pts',(-3.95670276375108,-1.,0.801366797727049));
#48225=CARTESIAN_POINT('Ctrl Pts',(-3.95670276375108,1.,0.801366797727049));
#48226=CARTESIAN_POINT('Ctrl Pts',(-3.96313222295815,-1.,0.805542372178361));
#48227=CARTESIAN_POINT('Ctrl Pts',(-3.96313222295815,1.,0.805542372178361));
#48228=CARTESIAN_POINT('Ctrl Pts',(-3.96954717513232,-1.,0.80975573281809));
#48229=CARTESIAN_POINT('Ctrl Pts',(-3.96954717513232,1.,0.80975573281809));
#48230=CARTESIAN_POINT('Ctrl Pts',(-3.97594844078811,-1.,0.814006592328843));
#48231=CARTESIAN_POINT('Ctrl Pts',(-3.97594844078811,1.,0.814006592328843));
#48232=CARTESIAN_POINT('Ctrl Pts',(-3.98233640155404,-1.,0.818294599022293));
#48233=CARTESIAN_POINT('Ctrl Pts',(-3.98233640155404,1.,0.818294599022293));
#48234=CARTESIAN_POINT('Ctrl Pts',(-3.98871104646485,-1.,0.822619346022119));
#48235=CARTESIAN_POINT('Ctrl Pts',(-3.98871104646485,1.,0.822619346022119));
#48236=CARTESIAN_POINT('Ctrl Pts',(-3.99507212784431,-1.,0.826980400320789));
#48237=CARTESIAN_POINT('Ctrl Pts',(-3.99507212784431,1.,0.826980400320789));
#48238=CARTESIAN_POINT('Ctrl Pts',(-4.00141928477507,-1.,0.831377325741622));
#48239=CARTESIAN_POINT('Ctrl Pts',(-4.00141928477507,1.,0.831377325741622));
#48240=CARTESIAN_POINT('Ctrl Pts',(-4.00775216907856,-1.,0.835809705809646));
#48241=CARTESIAN_POINT('Ctrl Pts',(-4.00775216907856,1.,0.835809705809646));
#48242=CARTESIAN_POINT('Ctrl Pts',(-4.01407059766103,-1.,0.840277171975855));
#48243=CARTESIAN_POINT('Ctrl Pts',(-4.01407059766103,1.,0.840277171975855));
#48244=CARTESIAN_POINT('Ctrl Pts',(-4.02037456798441,-1.,0.844779403287745));
#48245=CARTESIAN_POINT('Ctrl Pts',(-4.02037456798441,1.,0.844779403287745));
#48246=CARTESIAN_POINT('Ctrl Pts',(-4.02666418343164,-1.,0.849316107474245));
#48247=CARTESIAN_POINT('Ctrl Pts',(-4.02666418343164,1.,0.849316107474245));
#48248=CARTESIAN_POINT('Ctrl Pts',(-4.03293960436756,-1.,0.853887006631755));
#48249=CARTESIAN_POINT('Ctrl Pts',(-4.03293960436756,1.,0.853887006631755));
#48250=CARTESIAN_POINT('Ctrl Pts',(-4.03920099284773,-1.,0.858491822322827));
#48251=CARTESIAN_POINT('Ctrl Pts',(-4.03920099284773,1.,0.858491822322827));
#48252=CARTESIAN_POINT('Ctrl Pts',(-4.04544845048584,-1.,0.863130256643259));
#48253=CARTESIAN_POINT('Ctrl Pts',(-4.04544845048584,1.,0.863130256643259));
#48254=CARTESIAN_POINT('Ctrl Pts',(-4.05168199437909,-1.,0.867801988859917));
#48255=CARTESIAN_POINT('Ctrl Pts',(-4.05168199437909,1.,0.867801988859917));
#48256=CARTESIAN_POINT('Ctrl Pts',(-4.0579015903134,-1.,0.872506694782446));
#48257=CARTESIAN_POINT('Ctrl Pts',(-4.0579015903134,1.,0.872506694782446));
#48258=CARTESIAN_POINT('Ctrl Pts',(-4.06410717232905,-1.,0.877244060485837));
#48259=CARTESIAN_POINT('Ctrl Pts',(-4.06410717232905,1.,0.877244060485837));
#48260=CARTESIAN_POINT('Ctrl Pts',(-4.07029866694192,-1.,0.882013797525692));
#48261=CARTESIAN_POINT('Ctrl Pts',(-4.07029866694192,1.,0.882013797525692));
#48262=CARTESIAN_POINT('Ctrl Pts',(-4.07647601773635,-1.,0.886815658358501));
#48263=CARTESIAN_POINT('Ctrl Pts',(-4.07647601773635,1.,0.886815658358501));
#48264=CARTESIAN_POINT('Ctrl Pts',(-4.08263920304799,-1.,0.891649447916277));
#48265=CARTESIAN_POINT('Ctrl Pts',(-4.08263920304799,1.,0.891649447916277));
#48266=CARTESIAN_POINT('Ctrl Pts',(-4.08878822246833,-1.,0.896515019231333));
#48267=CARTESIAN_POINT('Ctrl Pts',(-4.08878822246833,1.,0.896515019231333));
#48268=CARTESIAN_POINT('Ctrl Pts',(-4.09369611522387,-1.,0.900432820941674));
#48269=CARTESIAN_POINT('Ctrl Pts',(-4.09369611522387,1.,0.900432820941674));
#48270=CARTESIAN_POINT('Ctrl Pts',(-4.09737067245935,-1.,0.903385402441587));
#48271=CARTESIAN_POINT('Ctrl Pts',(-4.09737067245935,1.,0.903385402441587));
#48272=CARTESIAN_POINT('Ctrl Pts',(-4.09981755067523,-1.,0.905360112215337));
#48273=CARTESIAN_POINT('Ctrl Pts',(-4.09981755067523,1.,0.905360112215337));
#48274=CARTESIAN_POINT('Ctrl Pts',(-4.10104028313088,-1.,0.906349047628866));
#48275=CARTESIAN_POINT('Ctrl Pts',(-4.10104028313088,1.,0.906349047628866));
#48276=CARTESIAN_POINT('',(-3.68845817949586,1.,0.676591647975429));
#48277=CARTESIAN_POINT('Ctrl Pts',(-3.68845817949586,-1.,0.676591647975428));
#48278=CARTESIAN_POINT('Ctrl Pts',(-3.68845817949586,-0.666666666666667,
0.676591647975428));
#48279=CARTESIAN_POINT('Ctrl Pts',(-3.68845817949586,-0.333333333333333,
0.676591647975428));
#48280=CARTESIAN_POINT('Ctrl Pts',(-3.68845817949586,0.333333333333333,
0.676591647975428));
#48281=CARTESIAN_POINT('Ctrl Pts',(-3.68845817949586,0.666666666666667,
0.676591647975429));
#48282=CARTESIAN_POINT('Ctrl Pts',(-3.68845817949586,1.,0.676591647975429));
#48283=CARTESIAN_POINT('',(-4.10104028313088,1.,0.906349047628866));
#48284=CARTESIAN_POINT('',(-4.10104028313088,0.,0.906349047628866));
#48285=CARTESIAN_POINT('Ctrl Pts',(-3.68845817949586,1.,0.676591647975428));
#48286=CARTESIAN_POINT('Ctrl Pts',(-3.68850172300477,1.,0.676569286094606));
#48287=CARTESIAN_POINT('Ctrl Pts',(-3.68869596425969,1.,0.676535079520806));
#48288=CARTESIAN_POINT('Ctrl Pts',(-3.68934997767243,1.,0.676580391119396));
#48289=CARTESIAN_POINT('Ctrl Pts',(-3.69101071175464,1.,0.676867042599401));
#48290=CARTESIAN_POINT('Ctrl Pts',(-3.69443683573598,1.,0.677621861865498));
#48291=CARTESIAN_POINT('Ctrl Pts',(-3.69959004073005,1.,0.678878822226026));
#48292=CARTESIAN_POINT('Ctrl Pts',(-3.70595722031785,1.,0.680526909710877));
#48293=CARTESIAN_POINT('Ctrl Pts',(-3.71319182789943,1.,0.68249234510893));
#48294=CARTESIAN_POINT('Ctrl Pts',(-3.7209063713926,1.,0.684691698167848));
#48295=CARTESIAN_POINT('Ctrl Pts',(-3.72872973554051,1.,0.687043475232354));
#48296=CARTESIAN_POINT('Ctrl Pts',(-3.73636374475077,1.,0.689479637354813));
#48297=CARTESIAN_POINT('Ctrl Pts',(-3.74365508986712,1.,0.69196008040082));
#48298=CARTESIAN_POINT('Ctrl Pts',(-3.75060288243455,1.,0.694474562581492));
#48299=CARTESIAN_POINT('Ctrl Pts',(-3.75729775767023,1.,0.697031245659743));
#48300=CARTESIAN_POINT('Ctrl Pts',(-3.76387780603759,1.,0.699648552230917));
#48301=CARTESIAN_POINT('Ctrl Pts',(-3.77048141872872,1.,0.702346356621551));
#48302=CARTESIAN_POINT('Ctrl Pts',(-3.77719254217129,1.,0.705135847999816));
#48303=CARTESIAN_POINT('Ctrl Pts',(-3.78402183336605,1.,0.708015879375459));
#48304=CARTESIAN_POINT('Ctrl Pts',(-3.79093694007094,1.,0.710978231689017));
#48305=CARTESIAN_POINT('Ctrl Pts',(-3.79788100314975,1.,0.71401073300664));
#48306=CARTESIAN_POINT('Ctrl Pts',(-3.80479445759309,1.,0.717100993669114));
#48307=CARTESIAN_POINT('Ctrl Pts',(-3.81163885127344,1.,0.720240466589236));
#48308=CARTESIAN_POINT('Ctrl Pts',(-3.81840802610835,1.,0.723426346019422));
#48309=CARTESIAN_POINT('Ctrl Pts',(-3.82511495756713,1.,0.726659281876664));
#48310=CARTESIAN_POINT('Ctrl Pts',(-3.83178392403383,1.,0.729942010490167));
#48311=CARTESIAN_POINT('Ctrl Pts',(-3.83844103658009,1.,0.733277703756078));
#48312=CARTESIAN_POINT('Ctrl Pts',(-3.84510432881213,1.,0.736668240497117));
#48313=CARTESIAN_POINT('Ctrl Pts',(-3.85177770351216,1.,0.740113146827137));
#48314=CARTESIAN_POINT('Ctrl Pts',(-3.85845645217594,1.,0.743610542737012));
#48315=CARTESIAN_POINT('Ctrl Pts',(-3.86513062969889,1.,0.747157716488871));
#48316=CARTESIAN_POINT('Ctrl Pts',(-3.87178914078374,1.,0.750751822383027));
#48317=CARTESIAN_POINT('Ctrl Pts',(-3.87842382520065,1.,0.754390577396856));
#48318=CARTESIAN_POINT('Ctrl Pts',(-3.88503262662689,1.,0.758072800564801));
#48319=CARTESIAN_POINT('Ctrl Pts',(-3.89161738162245,1.,0.761798028793969));
#48320=CARTESIAN_POINT('Ctrl Pts',(-3.89818233104378,1.,0.765566256401295));
#48321=CARTESIAN_POINT('Ctrl Pts',(-3.90473237182633,1.,0.769377629847874));
#48322=CARTESIAN_POINT('Ctrl Pts',(-3.91127138115243,1.,0.773232154506321));
#48323=CARTESIAN_POINT('Ctrl Pts',(-3.9178006233448,1.,0.777129415664956));
#48324=CARTESIAN_POINT('Ctrl Pts',(-3.92431956510441,1.,0.781068718228451));
#48325=CARTESIAN_POINT('Ctrl Pts',(-3.93082655631789,1.,0.785049202786507));
#48326=CARTESIAN_POINT('Ctrl Pts',(-3.93731956885676,1.,0.789069971469333));
#48327=CARTESIAN_POINT('Ctrl Pts',(-3.94379688971283,1.,0.793130205640961));
#48328=CARTESIAN_POINT('Ctrl Pts',(-3.95025788827136,1.,0.797229296085315));
#48329=CARTESIAN_POINT('Ctrl Pts',(-3.95670276375108,1.,0.801366797727049));
#48330=CARTESIAN_POINT('Ctrl Pts',(-3.96313222295815,1.,0.805542372178361));
#48331=CARTESIAN_POINT('Ctrl Pts',(-3.96954717513232,1.,0.80975573281809));
#48332=CARTESIAN_POINT('Ctrl Pts',(-3.97594844078811,1.,0.814006592328843));
#48333=CARTESIAN_POINT('Ctrl Pts',(-3.98233640155404,1.,0.818294599022293));
#48334=CARTESIAN_POINT('Ctrl Pts',(-3.98871104646485,1.,0.822619346022119));
#48335=CARTESIAN_POINT('Ctrl Pts',(-3.99507212784431,1.,0.826980400320789));
#48336=CARTESIAN_POINT('Ctrl Pts',(-4.00141928477507,1.,0.831377325741622));
#48337=CARTESIAN_POINT('Ctrl Pts',(-4.00775216907856,1.,0.835809705809646));
#48338=CARTESIAN_POINT('Ctrl Pts',(-4.01407059766103,1.,0.840277171975855));
#48339=CARTESIAN_POINT('Ctrl Pts',(-4.02037456798441,1.,0.844779403287745));
#48340=CARTESIAN_POINT('Ctrl Pts',(-4.02666418343164,1.,0.849316107474245));
#48341=CARTESIAN_POINT('Ctrl Pts',(-4.03293960436756,1.,0.853887006631755));
#48342=CARTESIAN_POINT('Ctrl Pts',(-4.03920099284773,1.,0.858491822322827));
#48343=CARTESIAN_POINT('Ctrl Pts',(-4.04544845048584,1.,0.863130256643259));
#48344=CARTESIAN_POINT('Ctrl Pts',(-4.05168199437909,1.,0.867801988859917));
#48345=CARTESIAN_POINT('Ctrl Pts',(-4.0579015903134,1.,0.872506694782446));
#48346=CARTESIAN_POINT('Ctrl Pts',(-4.06410717232905,1.,0.877244060485837));
#48347=CARTESIAN_POINT('Ctrl Pts',(-4.07029866694192,1.,0.882013797525692));
#48348=CARTESIAN_POINT('Ctrl Pts',(-4.07647601773635,1.,0.886815658358501));
#48349=CARTESIAN_POINT('Ctrl Pts',(-4.08263920304799,1.,0.891649447916277));
#48350=CARTESIAN_POINT('Ctrl Pts',(-4.08878822246833,1.,0.896515019231333));
#48351=CARTESIAN_POINT('Ctrl Pts',(-4.09369611522387,1.,0.900432820941674));
#48352=CARTESIAN_POINT('Ctrl Pts',(-4.09737067245935,1.,0.903385402441587));
#48353=CARTESIAN_POINT('Ctrl Pts',(-4.09981755067523,1.,0.905360112215337));
#48354=CARTESIAN_POINT('Ctrl Pts',(-4.10104028313088,1.,0.906349047628866));
#48355=CARTESIAN_POINT('Origin',(-4.10104028313088,0.,0.906349047628866));
#48356=CARTESIAN_POINT('',(-4.06552750530042,1.,1.05427041296137));
#48357=CARTESIAN_POINT('Origin',(0.,0.,0.));
#48358=CARTESIAN_POINT('',(-3.71701050416802,1.,0.496319364829374));
#48359=CARTESIAN_POINT('Origin',(0.,1.,0.));
#48360=CARTESIAN_POINT('Ctrl Pts',(-3.71701050416802,1.,0.496319364829374));
#48361=CARTESIAN_POINT('Ctrl Pts',(-3.71701050416802,0.666666666666667,
0.496319364829374));
#48362=CARTESIAN_POINT('Ctrl Pts',(-3.71701050416802,0.333333333333333,
0.496319364829374));
#48363=CARTESIAN_POINT('Ctrl Pts',(-3.71701050416802,-0.333333333333333,
0.496319364829374));
#48364=CARTESIAN_POINT('Ctrl Pts',(-3.71701050416802,-0.666666666666667,
0.496319364829374));
#48365=CARTESIAN_POINT('Ctrl Pts',(-3.71701050416802,-1.,0.496319364829374));
#48366=CARTESIAN_POINT('Ctrl Pts',(-4.18039834341342,-1.,0.405301974318349));
#48367=CARTESIAN_POINT('Ctrl Pts',(-4.18039834341342,1.,0.405301974318349));
#48368=CARTESIAN_POINT('Ctrl Pts',(-4.17892985789908,-1.,0.40586466267963));
#48369=CARTESIAN_POINT('Ctrl Pts',(-4.17892985789908,1.,0.40586466267963));
#48370=CARTESIAN_POINT('Ctrl Pts',(-4.17599251955585,-1.,0.406986596326602));
#48371=CARTESIAN_POINT('Ctrl Pts',(-4.17599251955585,1.,0.406986596326602));
#48372=CARTESIAN_POINT('Ctrl Pts',(-4.17158541009947,-1.,0.408659167570153));
#48373=CARTESIAN_POINT('Ctrl Pts',(-4.17158541009947,1.,0.408659167570153));
#48374=CARTESIAN_POINT('Ctrl Pts',(-4.16570705940731,-1.,0.410868596148613));
#48375=CARTESIAN_POINT('Ctrl Pts',(-4.16570705940731,1.,0.410868596148613));
#48376=CARTESIAN_POINT('Ctrl Pts',(-4.1583554501909,-1.,0.413595877953269));
#48377=CARTESIAN_POINT('Ctrl Pts',(-4.1583554501909,1.,0.413595877953269));
#48378=CARTESIAN_POINT('Ctrl Pts',(-4.15100018950989,-1.,0.416288556008986));
#48379=CARTESIAN_POINT('Ctrl Pts',(-4.15100018950989,1.,0.416288556008986));
#48380=CARTESIAN_POINT('Ctrl Pts',(-4.14364132317223,-1.,0.418946490667799));
#48381=CARTESIAN_POINT('Ctrl Pts',(-4.14364132317223,1.,0.418946490667799));
#48382=CARTESIAN_POINT('Ctrl Pts',(-4.13627893206433,-1.,0.421569503103971));
#48383=CARTESIAN_POINT('Ctrl Pts',(-4.13627893206433,1.,0.421569503103971));
#48384=CARTESIAN_POINT('Ctrl Pts',(-4.1289131463371,-1.,0.424157375323155));
#48385=CARTESIAN_POINT('Ctrl Pts',(-4.1289131463371,1.,0.424157375323155));
#48386=CARTESIAN_POINT('Ctrl Pts',(-4.1215441250121,-1.,0.426709855706243));
#48387=CARTESIAN_POINT('Ctrl Pts',(-4.1215441250121,1.,0.426709855706243));
#48388=CARTESIAN_POINT('Ctrl Pts',(-4.1141720278277,-1.,0.429226666075372));
#48389=CARTESIAN_POINT('Ctrl Pts',(-4.1141720278277,1.,0.429226666075372));
#48390=CARTESIAN_POINT('Ctrl Pts',(-4.10679698750219,-1.,0.431707508679772));
#48391=CARTESIAN_POINT('Ctrl Pts',(-4.10679698750219,1.,0.431707508679772));
#48392=CARTESIAN_POINT('Ctrl Pts',(-4.09941908688567,-1.,0.434152073200642));
#48393=CARTESIAN_POINT('Ctrl Pts',(-4.09941908688567,1.,0.434152073200642));
#48394=CARTESIAN_POINT('Ctrl Pts',(-4.09203832139439,-1.,0.436560044913814));
#48395=CARTESIAN_POINT('Ctrl Pts',(-4.09203832139439,1.,0.436560044913814));
#48396=CARTESIAN_POINT('Ctrl Pts',(-4.08465462294625,-1.,0.438931108931613));
#48397=CARTESIAN_POINT('Ctrl Pts',(-4.08465462294625,1.,0.438931108931613));
#48398=CARTESIAN_POINT('Ctrl Pts',(-4.07726792490256,-1.,0.441264951396587));
#48399=CARTESIAN_POINT('Ctrl Pts',(-4.07726792490256,1.,0.441264951396587));
#48400=CARTESIAN_POINT('Ctrl Pts',(-4.0698782192577,-1.,0.443561262395408));
#48401=CARTESIAN_POINT('Ctrl Pts',(-4.0698782192577,1.,0.443561262395408));
#48402=CARTESIAN_POINT('Ctrl Pts',(-4.06248560760596,-1.,0.445819737468478));
#48403=CARTESIAN_POINT('Ctrl Pts',(-4.06248560760596,1.,0.445819737468478));
#48404=CARTESIAN_POINT('Ctrl Pts',(-4.05509037796815,-1.,0.448040082683976));
#48405=CARTESIAN_POINT('Ctrl Pts',(-4.05509037796815,1.,0.448040082683976));
#48406=CARTESIAN_POINT('Ctrl Pts',(-4.0476929901797,-1.,0.450222009543774));
#48407=CARTESIAN_POINT('Ctrl Pts',(-4.0476929901797,1.,0.450222009543774));
#48408=CARTESIAN_POINT('Ctrl Pts',(-4.0402939222793,-1.,0.452365214748779));
#48409=CARTESIAN_POINT('Ctrl Pts',(-4.0402939222793,1.,0.452365214748779));
#48410=CARTESIAN_POINT('Ctrl Pts',(-4.03289354362745,-1.,0.454469363020495));
#48411=CARTESIAN_POINT('Ctrl Pts',(-4.03289354362745,1.,0.454469363020495));
#48412=CARTESIAN_POINT('Ctrl Pts',(-4.02549199038414,-1.,0.456534070784968));
#48413=CARTESIAN_POINT('Ctrl Pts',(-4.02549199038414,1.,0.456534070784968));
#48414=CARTESIAN_POINT('Ctrl Pts',(-4.01808900827647,-1.,0.458558885637001));
#48415=CARTESIAN_POINT('Ctrl Pts',(-4.01808900827647,1.,0.458558885637001));
#48416=CARTESIAN_POINT('Ctrl Pts',(-4.01068390573469,-1.,0.460543280768577));
#48417=CARTESIAN_POINT('Ctrl Pts',(-4.01068390573469,1.,0.460543280768577));
#48418=CARTESIAN_POINT('Ctrl Pts',(-4.00327590659129,-1.,0.462486702616252));
#48419=CARTESIAN_POINT('Ctrl Pts',(-4.00327590659129,1.,0.462486702616252));
#48420=CARTESIAN_POINT('Ctrl Pts',(-3.99586444320135,-1.,0.464388610938995));
#48421=CARTESIAN_POINT('Ctrl Pts',(-3.99586444320135,1.,0.464388610938995));
#48422=CARTESIAN_POINT('Ctrl Pts',(-3.98844946363258,-1.,0.466248520883034));
#48423=CARTESIAN_POINT('Ctrl Pts',(-3.98844946363258,1.,0.466248520883034));
#48424=CARTESIAN_POINT('Ctrl Pts',(-3.98103175589349,-1.,0.468066047920139));
#48425=CARTESIAN_POINT('Ctrl Pts',(-3.98103175589349,1.,0.468066047920139));
#48426=CARTESIAN_POINT('Ctrl Pts',(-3.97361320212413,-1.,0.469840942829878));
#48427=CARTESIAN_POINT('Ctrl Pts',(-3.97361320212413,1.,0.469840942829878));
#48428=CARTESIAN_POINT('Ctrl Pts',(-3.96619600864626,-1.,0.471572978413493));
#48429=CARTESIAN_POINT('Ctrl Pts',(-3.96619600864626,1.,0.471572978413493));
#48430=CARTESIAN_POINT('Ctrl Pts',(-3.95878201038332,-1.,0.473261847236296));
#48431=CARTESIAN_POINT('Ctrl Pts',(-3.95878201038332,1.,0.473261847236296));
#48432=CARTESIAN_POINT('Ctrl Pts',(-3.95137192932898,-1.,0.47490705302179));
#48433=CARTESIAN_POINT('Ctrl Pts',(-3.95137192932898,1.,0.47490705302179));
#48434=CARTESIAN_POINT('Ctrl Pts',(-3.94396469119385,-1.,0.476507810658534));
#48435=CARTESIAN_POINT('Ctrl Pts',(-3.94396469119385,1.,0.476507810658534));
#48436=CARTESIAN_POINT('Ctrl Pts',(-3.93655660689819,-1.,0.478062927140957));
#48437=CARTESIAN_POINT('Ctrl Pts',(-3.93655660689819,1.,0.478062927140957));
#48438=CARTESIAN_POINT('Ctrl Pts',(-3.92914297392067,-1.,0.479571028525566));
#48439=CARTESIAN_POINT('Ctrl Pts',(-3.92914297392067,1.,0.479571028525566));
#48440=CARTESIAN_POINT('Ctrl Pts',(-3.92171976072334,-1.,0.481030798910735));
#48441=CARTESIAN_POINT('Ctrl Pts',(-3.92171976072334,1.,0.481030798910735));
#48442=CARTESIAN_POINT('Ctrl Pts',(-3.91428536373749,-1.,0.482441230340708));
#48443=CARTESIAN_POINT('Ctrl Pts',(-3.91428536373749,1.,0.482441230340708));
#48444=CARTESIAN_POINT('Ctrl Pts',(-3.90684210358063,-1.,0.48380183508916));
#48445=CARTESIAN_POINT('Ctrl Pts',(-3.90684210358063,1.,0.48380183508916));
#48446=CARTESIAN_POINT('Ctrl Pts',(-3.89939844658529,-1.,0.485112963522246));
#48447=CARTESIAN_POINT('Ctrl Pts',(-3.89939844658529,1.,0.485112963522246));
#48448=CARTESIAN_POINT('Ctrl Pts',(-3.89196582437574,-1.,0.486375337854133));
#48449=CARTESIAN_POINT('Ctrl Pts',(-3.89196582437574,1.,0.486375337854133));
#48450=CARTESIAN_POINT('Ctrl Pts',(-3.88455453328156,-1.,0.487589452275179));
#48451=CARTESIAN_POINT('Ctrl Pts',(-3.88455453328156,1.,0.487589452275179));
#48452=CARTESIAN_POINT('Ctrl Pts',(-3.87716963231115,-1.,0.488754973798281));
#48453=CARTESIAN_POINT('Ctrl Pts',(-3.87716963231115,1.,0.488754973798281));
#48454=CARTESIAN_POINT('Ctrl Pts',(-3.86980755613694,-1.,0.489870245704899));
#48455=CARTESIAN_POINT('Ctrl Pts',(-3.86980755613694,1.,0.489870245704899));
#48456=CARTESIAN_POINT('Ctrl Pts',(-3.86245057319215,-1.,0.490931482170849));
#48457=CARTESIAN_POINT('Ctrl Pts',(-3.86245057319215,1.,0.490931482170849));
#48458=CARTESIAN_POINT('Ctrl Pts',(-3.85507287020223,-1.,0.49193363108376));
#48459=CARTESIAN_POINT('Ctrl Pts',(-3.85507287020223,1.,0.49193363108376));
#48460=CARTESIAN_POINT('Ctrl Pts',(-3.84765051147965,-1.,0.492871792414095));
#48461=CARTESIAN_POINT('Ctrl Pts',(-3.84765051147965,1.,0.492871792414095));
#48462=CARTESIAN_POINT('Ctrl Pts',(-3.84017095578438,-1.,0.493742574629117));
#48463=CARTESIAN_POINT('Ctrl Pts',(-3.84017095578438,1.,0.493742574629117));
#48464=CARTESIAN_POINT('Ctrl Pts',(-3.8326409268245,-1.,0.494545212256425));
#48465=CARTESIAN_POINT('Ctrl Pts',(-3.8326409268245,1.,0.494545212256425));
#48466=CARTESIAN_POINT('Ctrl Pts',(-3.82509963594156,-1.,0.495283458893903));
#48467=CARTESIAN_POINT('Ctrl Pts',(-3.82509963594156,1.,0.495283458893903));
#48468=CARTESIAN_POINT('Ctrl Pts',(-3.81760756144099,-1.,0.495963937875572));
#48469=CARTESIAN_POINT('Ctrl Pts',(-3.81760756144099,1.,0.495963937875572));
#48470=CARTESIAN_POINT('Ctrl Pts',(-3.81022254090909,-1.,0.496592643443789));
#48471=CARTESIAN_POINT('Ctrl Pts',(-3.81022254090909,1.,0.496592643443789));
#48472=CARTESIAN_POINT('Ctrl Pts',(-3.80297788298545,-1.,0.49717175620109));
#48473=CARTESIAN_POINT('Ctrl Pts',(-3.80297788298545,1.,0.49717175620109));
#48474=CARTESIAN_POINT('Ctrl Pts',(-3.79586380669959,-1.,0.49769689210058));
#48475=CARTESIAN_POINT('Ctrl Pts',(-3.79586380669959,1.,0.49769689210058));
#48476=CARTESIAN_POINT('Ctrl Pts',(-3.78879701661152,-1.,0.498152751800819));
#48477=CARTESIAN_POINT('Ctrl Pts',(-3.78879701661152,1.,0.498152751800819));
#48478=CARTESIAN_POINT('Ctrl Pts',(-3.78163975337189,-1.,0.498515471679378));
#48479=CARTESIAN_POINT('Ctrl Pts',(-3.78163975337189,1.,0.498515471679378));
#48480=CARTESIAN_POINT('Ctrl Pts',(-3.77425499225089,-1.,0.498759900365687));
#48481=CARTESIAN_POINT('Ctrl Pts',(-3.77425499225089,1.,0.498759900365687));
#48482=CARTESIAN_POINT('Ctrl Pts',(-3.76655401191144,-1.,0.498865792335185));
#48483=CARTESIAN_POINT('Ctrl Pts',(-3.76655401191144,1.,0.498865792335185));
#48484=CARTESIAN_POINT('Ctrl Pts',(-3.75854082221127,-1.,0.498823681615513));
#48485=CARTESIAN_POINT('Ctrl Pts',(-3.75854082221127,1.,0.498823681615513));
#48486=CARTESIAN_POINT('Ctrl Pts',(-3.75037362168103,-1.,0.498642802042929));
#48487=CARTESIAN_POINT('Ctrl Pts',(-3.75037362168103,1.,0.498642802042929));
#48488=CARTESIAN_POINT('Ctrl Pts',(-3.74235701735109,-1.,0.498350586058176));
#48489=CARTESIAN_POINT('Ctrl Pts',(-3.74235701735109,1.,0.498350586058176));
#48490=CARTESIAN_POINT('Ctrl Pts',(-3.73486914372834,-1.,0.497984209510495));
#48491=CARTESIAN_POINT('Ctrl Pts',(-3.73486914372834,1.,0.497984209510495));
#48492=CARTESIAN_POINT('Ctrl Pts',(-3.72830430904794,-1.,0.497584067153279));
#48493=CARTESIAN_POINT('Ctrl Pts',(-3.72830430904794,1.,0.497584067153279));
#48494=CARTESIAN_POINT('Ctrl Pts',(-3.72301489774241,-1.,0.497187079575794));
#48495=CARTESIAN_POINT('Ctrl Pts',(-3.72301489774241,1.,0.497187079575794));
#48496=CARTESIAN_POINT('Ctrl Pts',(-3.71923995965807,-1.,0.496818574419988));
#48497=CARTESIAN_POINT('Ctrl Pts',(-3.71923995965807,1.,0.496818574419988));
#48498=CARTESIAN_POINT('Ctrl Pts',(-3.71752134136931,-1.,0.496556137603856));
#48499=CARTESIAN_POINT('Ctrl Pts',(-3.71752134136931,1.,0.496556137603856));
#48500=CARTESIAN_POINT('Ctrl Pts',(-3.71698153685229,-1.,0.496379397992181));
#48501=CARTESIAN_POINT('Ctrl Pts',(-3.71698153685229,1.,0.496379397992181));
#48502=CARTESIAN_POINT('Ctrl Pts',(-3.71695438995598,-1.,0.496270484166233));
#48503=CARTESIAN_POINT('Ctrl Pts',(-3.71695438995598,1.,0.496270484166233));
#48504=CARTESIAN_POINT('Ctrl Pts',(-3.71702400346349,-1.,0.496218256089211));
#48505=CARTESIAN_POINT('Ctrl Pts',(-3.71702400346349,1.,0.496218256089211));
#48506=CARTESIAN_POINT('',(-4.18039834341342,1.,0.405301974318349));
#48507=CARTESIAN_POINT('Ctrl Pts',(-4.18039834341342,1.,0.405301974318349));
#48508=CARTESIAN_POINT('Ctrl Pts',(-4.17892985789908,1.,0.40586466267963));
#48509=CARTESIAN_POINT('Ctrl Pts',(-4.17599251955585,1.,0.406986596326602));
#48510=CARTESIAN_POINT('Ctrl Pts',(-4.17158541009947,1.,0.408659167570153));
#48511=CARTESIAN_POINT('Ctrl Pts',(-4.16570705940731,1.,0.410868596148613));
#48512=CARTESIAN_POINT('Ctrl Pts',(-4.1583554501909,1.,0.413595877953269));
#48513=CARTESIAN_POINT('Ctrl Pts',(-4.15100018950989,1.,0.416288556008986));
#48514=CARTESIAN_POINT('Ctrl Pts',(-4.14364132317223,1.,0.418946490667799));
#48515=CARTESIAN_POINT('Ctrl Pts',(-4.13627893206433,1.,0.421569503103971));
#48516=CARTESIAN_POINT('Ctrl Pts',(-4.1289131463371,1.,0.424157375323155));
#48517=CARTESIAN_POINT('Ctrl Pts',(-4.1215441250121,1.,0.426709855706243));
#48518=CARTESIAN_POINT('Ctrl Pts',(-4.1141720278277,1.,0.429226666075372));
#48519=CARTESIAN_POINT('Ctrl Pts',(-4.10679698750219,1.,0.431707508679772));
#48520=CARTESIAN_POINT('Ctrl Pts',(-4.09941908688567,1.,0.434152073200642));
#48521=CARTESIAN_POINT('Ctrl Pts',(-4.09203832139439,1.,0.436560044913814));
#48522=CARTESIAN_POINT('Ctrl Pts',(-4.08465462294625,1.,0.438931108931613));
#48523=CARTESIAN_POINT('Ctrl Pts',(-4.07726792490256,1.,0.441264951396587));
#48524=CARTESIAN_POINT('Ctrl Pts',(-4.0698782192577,1.,0.443561262395408));
#48525=CARTESIAN_POINT('Ctrl Pts',(-4.06248560760596,1.,0.445819737468478));
#48526=CARTESIAN_POINT('Ctrl Pts',(-4.05509037796815,1.,0.448040082683976));
#48527=CARTESIAN_POINT('Ctrl Pts',(-4.0476929901797,1.,0.450222009543774));
#48528=CARTESIAN_POINT('Ctrl Pts',(-4.0402939222793,1.,0.452365214748779));
#48529=CARTESIAN_POINT('Ctrl Pts',(-4.03289354362745,1.,0.454469363020495));
#48530=CARTESIAN_POINT('Ctrl Pts',(-4.02549199038414,1.,0.456534070784968));
#48531=CARTESIAN_POINT('Ctrl Pts',(-4.01808900827647,1.,0.458558885637001));
#48532=CARTESIAN_POINT('Ctrl Pts',(-4.01068390573469,1.,0.460543280768577));
#48533=CARTESIAN_POINT('Ctrl Pts',(-4.00327590659129,1.,0.462486702616252));
#48534=CARTESIAN_POINT('Ctrl Pts',(-3.99586444320135,1.,0.464388610938995));
#48535=CARTESIAN_POINT('Ctrl Pts',(-3.98844946363258,1.,0.466248520883034));
#48536=CARTESIAN_POINT('Ctrl Pts',(-3.98103175589349,1.,0.468066047920139));
#48537=CARTESIAN_POINT('Ctrl Pts',(-3.97361320212413,1.,0.469840942829878));
#48538=CARTESIAN_POINT('Ctrl Pts',(-3.96619600864626,1.,0.471572978413493));
#48539=CARTESIAN_POINT('Ctrl Pts',(-3.95878201038332,1.,0.473261847236296));
#48540=CARTESIAN_POINT('Ctrl Pts',(-3.95137192932898,1.,0.47490705302179));
#48541=CARTESIAN_POINT('Ctrl Pts',(-3.94396469119385,1.,0.476507810658534));
#48542=CARTESIAN_POINT('Ctrl Pts',(-3.93655660689819,1.,0.478062927140957));
#48543=CARTESIAN_POINT('Ctrl Pts',(-3.92914297392067,1.,0.479571028525566));
#48544=CARTESIAN_POINT('Ctrl Pts',(-3.92171976072334,1.,0.481030798910735));
#48545=CARTESIAN_POINT('Ctrl Pts',(-3.91428536373749,1.,0.482441230340708));
#48546=CARTESIAN_POINT('Ctrl Pts',(-3.90684210358063,1.,0.48380183508916));
#48547=CARTESIAN_POINT('Ctrl Pts',(-3.89939844658529,1.,0.485112963522246));
#48548=CARTESIAN_POINT('Ctrl Pts',(-3.89196582437574,1.,0.486375337854133));
#48549=CARTESIAN_POINT('Ctrl Pts',(-3.88455453328156,1.,0.487589452275179));
#48550=CARTESIAN_POINT('Ctrl Pts',(-3.87716963231115,1.,0.488754973798281));
#48551=CARTESIAN_POINT('Ctrl Pts',(-3.86980755613694,1.,0.489870245704899));
#48552=CARTESIAN_POINT('Ctrl Pts',(-3.86245057319215,1.,0.490931482170849));
#48553=CARTESIAN_POINT('Ctrl Pts',(-3.85507287020223,1.,0.49193363108376));
#48554=CARTESIAN_POINT('Ctrl Pts',(-3.84765051147965,1.,0.492871792414095));
#48555=CARTESIAN_POINT('Ctrl Pts',(-3.84017095578438,1.,0.493742574629117));
#48556=CARTESIAN_POINT('Ctrl Pts',(-3.8326409268245,1.,0.494545212256425));
#48557=CARTESIAN_POINT('Ctrl Pts',(-3.82509963594156,1.,0.495283458893903));
#48558=CARTESIAN_POINT('Ctrl Pts',(-3.81760756144099,1.,0.495963937875572));
#48559=CARTESIAN_POINT('Ctrl Pts',(-3.81022254090909,1.,0.496592643443789));
#48560=CARTESIAN_POINT('Ctrl Pts',(-3.80297788298545,1.,0.49717175620109));
#48561=CARTESIAN_POINT('Ctrl Pts',(-3.79586380669959,1.,0.49769689210058));
#48562=CARTESIAN_POINT('Ctrl Pts',(-3.78879701661152,1.,0.498152751800819));
#48563=CARTESIAN_POINT('Ctrl Pts',(-3.78163975337189,1.,0.498515471679378));
#48564=CARTESIAN_POINT('Ctrl Pts',(-3.77425499225089,1.,0.498759900365687));
#48565=CARTESIAN_POINT('Ctrl Pts',(-3.76655401191144,1.,0.498865792335185));
#48566=CARTESIAN_POINT('Ctrl Pts',(-3.75854082221127,1.,0.498823681615513));
#48567=CARTESIAN_POINT('Ctrl Pts',(-3.75037362168103,1.,0.498642802042929));
#48568=CARTESIAN_POINT('Ctrl Pts',(-3.74235701735109,1.,0.498350586058176));
#48569=CARTESIAN_POINT('Ctrl Pts',(-3.73486914372834,1.,0.497984209510495));
#48570=CARTESIAN_POINT('Ctrl Pts',(-3.72830430904794,1.,0.497584067153279));
#48571=CARTESIAN_POINT('Ctrl Pts',(-3.72301489774241,1.,0.497187079575794));
#48572=CARTESIAN_POINT('Ctrl Pts',(-3.7195232082259,1.,0.496846224822535));
#48573=CARTESIAN_POINT('Ctrl Pts',(-3.71785517607694,1.,0.496605651526313));
#48574=CARTESIAN_POINT('Ctrl Pts',(-3.71721917030465,1.,0.496446644158827));
#48575=CARTESIAN_POINT('Ctrl Pts',(-3.71704500630521,1.,0.496354087925645));
#48576=CARTESIAN_POINT('Ctrl Pts',(-3.71701050416802,1.,0.496319364829374));
#48577=CARTESIAN_POINT('',(-4.18039834341342,0.,0.405301974318349));
#48578=CARTESIAN_POINT('Ctrl Pts',(-3.74888690736767,-1.,0.091361675593742));
#48579=CARTESIAN_POINT('Ctrl Pts',(-3.74888690736767,1.,0.091361675593742));
#48580=CARTESIAN_POINT('Ctrl Pts',(-3.74882632119067,-1.,0.0912992005792584));
#48581=CARTESIAN_POINT('Ctrl Pts',(-3.74882632119067,1.,0.0912992005792584));
#48582=CARTESIAN_POINT('Ctrl Pts',(-3.74887017174206,-1.,0.0911958743735234));
#48583=CARTESIAN_POINT('Ctrl Pts',(-3.74887017174206,1.,0.0911958743735234));
#48584=CARTESIAN_POINT('Ctrl Pts',(-3.74943097853811,-1.,0.0911057547506599));
#48585=CARTESIAN_POINT('Ctrl Pts',(-3.74943097853811,1.,0.0911057547506599));
#48586=CARTESIAN_POINT('Ctrl Pts',(-3.75116949194623,-1.,0.0911154000998141));
#48587=CARTESIAN_POINT('Ctrl Pts',(-3.75116949194623,1.,0.0911154000998141));
#48588=CARTESIAN_POINT('Ctrl Pts',(-3.75495560118212,-1.,0.0913419622736397));
#48589=CARTESIAN_POINT('Ctrl Pts',(-3.75495560118212,1.,0.0913419622736397));
#48590=CARTESIAN_POINT('Ctrl Pts',(-3.76024199359303,-1.,0.0917773084998334));
#48591=CARTESIAN_POINT('Ctrl Pts',(-3.76024199359303,1.,0.0917773084998334));
#48592=CARTESIAN_POINT('Ctrl Pts',(-3.76678860031841,-1.,0.092409058960269));
#48593=CARTESIAN_POINT('Ctrl Pts',(-3.76678860031841,1.,0.092409058960269));
#48594=CARTESIAN_POINT('Ctrl Pts',(-3.77424159971059,-1.,0.0932185546203178));
#48595=CARTESIAN_POINT('Ctrl Pts',(-3.77424159971059,1.,0.0932185546203178));
#48596=CARTESIAN_POINT('Ctrl Pts',(-3.782205218991,-1.,0.0941840095090813));
#48597=CARTESIAN_POINT('Ctrl Pts',(-3.782205218991,1.,0.0941840095090813));
#48598=CARTESIAN_POINT('Ctrl Pts',(-3.79030016353111,-1.,0.09528298851008));
#48599=CARTESIAN_POINT('Ctrl Pts',(-3.79030016353111,1.,0.09528298851008));
#48600=CARTESIAN_POINT('Ctrl Pts',(-3.79822128513845,-1.,0.0964949352873131));
#48601=CARTESIAN_POINT('Ctrl Pts',(-3.79822128513845,1.,0.0964949352873131));
#48602=CARTESIAN_POINT('Ctrl Pts',(-3.80581088847809,-1.,0.0978042222906642));
#48603=CARTESIAN_POINT('Ctrl Pts',(-3.80581088847809,1.,0.0978042222906642));
#48604=CARTESIAN_POINT('Ctrl Pts',(-3.81306649386461,-1.,0.0992008728096513));
#48605=CARTESIAN_POINT('Ctrl Pts',(-3.81306649386461,1.,0.0992008728096513));
#48606=CARTESIAN_POINT('Ctrl Pts',(-3.82007889742625,-1.,0.100678769650632));
#48607=CARTESIAN_POINT('Ctrl Pts',(-3.82007889742625,1.,0.100678769650632));
#48608=CARTESIAN_POINT('Ctrl Pts',(-3.82698737143255,-1.,0.102234506488456));
#48609=CARTESIAN_POINT('Ctrl Pts',(-3.82698737143255,1.,0.102234506488456));
#48610=CARTESIAN_POINT('Ctrl Pts',(-3.83393171228002,-1.,0.103866063811622));
#48611=CARTESIAN_POINT('Ctrl Pts',(-3.83393171228002,1.,0.103866063811622));
#48612=CARTESIAN_POINT('Ctrl Pts',(-3.84099658324803,-1.,0.105571360916569));
#48613=CARTESIAN_POINT('Ctrl Pts',(-3.84099658324803,1.,0.105571360916569));
#48614=CARTESIAN_POINT('Ctrl Pts',(-3.84819233070317,-1.,0.107347597812183));
#48615=CARTESIAN_POINT('Ctrl Pts',(-3.84819233070317,1.,0.107347597812183));
#48616=CARTESIAN_POINT('Ctrl Pts',(-3.855485714969,-1.,0.109191717634943));
#48617=CARTESIAN_POINT('Ctrl Pts',(-3.855485714969,1.,0.109191717634943));
#48618=CARTESIAN_POINT('Ctrl Pts',(-3.86281867282965,-1.,0.11110059303626));
#48619=CARTESIAN_POINT('Ctrl Pts',(-3.86281867282965,1.,0.11110059303626));
#48620=CARTESIAN_POINT('Ctrl Pts',(-3.87013043445014,-1.,0.113071304914561));
#48621=CARTESIAN_POINT('Ctrl Pts',(-3.87013043445014,1.,0.113071304914561));
#48622=CARTESIAN_POINT('Ctrl Pts',(-3.87738168405343,-1.,0.11510142664947));
#48623=CARTESIAN_POINT('Ctrl Pts',(-3.87738168405343,1.,0.11510142664947));
#48624=CARTESIAN_POINT('Ctrl Pts',(-3.88456590045767,-1.,0.117189150373144));
#48625=CARTESIAN_POINT('Ctrl Pts',(-3.88456590045767,1.,0.117189150373144));
#48626=CARTESIAN_POINT('Ctrl Pts',(-3.89169600105201,-1.,0.119333088190417));
#48627=CARTESIAN_POINT('Ctrl Pts',(-3.89169600105201,1.,0.119333088190417));
#48628=CARTESIAN_POINT('Ctrl Pts',(-3.89879639336952,-1.,0.121532144765723));
#48629=CARTESIAN_POINT('Ctrl Pts',(-3.89879639336952,1.,0.121532144765723));
#48630=CARTESIAN_POINT('Ctrl Pts',(-3.90589336320508,-1.,0.123785368272377));
#48631=CARTESIAN_POINT('Ctrl Pts',(-3.90589336320508,1.,0.123785368272377));
#48632=CARTESIAN_POINT('Ctrl Pts',(-3.91300501605392,-1.,0.126091793324136));
#48633=CARTESIAN_POINT('Ctrl Pts',(-3.91300501605392,1.,0.126091793324136));
#48634=CARTESIAN_POINT('Ctrl Pts',(-3.92013513251642,-1.,0.128450341339528));
#48635=CARTESIAN_POINT('Ctrl Pts',(-3.92013513251642,1.,0.128450341339528));
#48636=CARTESIAN_POINT('Ctrl Pts',(-3.9272787679596,-1.,0.130859892027798));
#48637=CARTESIAN_POINT('Ctrl Pts',(-3.9272787679596,1.,0.130859892027798));
#48638=CARTESIAN_POINT('Ctrl Pts',(-3.93442567551035,-1.,0.133319322794189));
#48639=CARTESIAN_POINT('Ctrl Pts',(-3.93442567551035,1.,0.133319322794189));
#48640=CARTESIAN_POINT('Ctrl Pts',(-3.94156445130744,-1.,0.135827558661188));
#48641=CARTESIAN_POINT('Ctrl Pts',(-3.94156445130744,1.,0.135827558661188));
#48642=CARTESIAN_POINT('Ctrl Pts',(-3.94868667844355,-1.,0.138383621255159));
#48643=CARTESIAN_POINT('Ctrl Pts',(-3.94868667844355,1.,0.138383621255159));
#48644=CARTESIAN_POINT('Ctrl Pts',(-3.95579014116899,-1.,0.140986665829937));
#48645=CARTESIAN_POINT('Ctrl Pts',(-3.95579014116899,1.,0.140986665829937));
#48646=CARTESIAN_POINT('Ctrl Pts',(-3.96287658098896,-1.,0.143635947692791));
#48647=CARTESIAN_POINT('Ctrl Pts',(-3.96287658098896,1.,0.143635947692791));
#48648=CARTESIAN_POINT('Ctrl Pts',(-3.96995018565891,-1.,0.146330797814513));
#48649=CARTESIAN_POINT('Ctrl Pts',(-3.96995018565891,1.,0.146330797814513));
#48650=CARTESIAN_POINT('Ctrl Pts',(-3.97701581473643,-1.,0.149070594803543));
#48651=CARTESIAN_POINT('Ctrl Pts',(-3.97701581473643,1.,0.149070594803543));
#48652=CARTESIAN_POINT('Ctrl Pts',(-3.9840772985098,-1.,0.151854737441405));
#48653=CARTESIAN_POINT('Ctrl Pts',(-3.9840772985098,1.,0.151854737441405));
#48654=CARTESIAN_POINT('Ctrl Pts',(-3.99113582086059,-1.,0.154682618338563));
#48655=CARTESIAN_POINT('Ctrl Pts',(-3.99113582086059,1.,0.154682618338563));
#48656=CARTESIAN_POINT('Ctrl Pts',(-3.99819074631874,-1.,0.157553634383809));
#48657=CARTESIAN_POINT('Ctrl Pts',(-3.99819074631874,1.,0.157553634383809));
#48658=CARTESIAN_POINT('Ctrl Pts',(-4.00524031064509,-1.,0.160467194882219));
#48659=CARTESIAN_POINT('Ctrl Pts',(-4.00524031064509,1.,0.160467194882219));
#48660=CARTESIAN_POINT('Ctrl Pts',(-4.01228237022301,-1.,0.163422730287458));
#48661=CARTESIAN_POINT('Ctrl Pts',(-4.01228237022301,1.,0.163422730287458));
#48662=CARTESIAN_POINT('Ctrl Pts',(-4.01931510507143,-1.,0.166419700015847));
#48663=CARTESIAN_POINT('Ctrl Pts',(-4.01931510507143,1.,0.166419700015847));
#48664=CARTESIAN_POINT('Ctrl Pts',(-4.0263377970371,-1.,0.169457601001653));
#48665=CARTESIAN_POINT('Ctrl Pts',(-4.0263377970371,1.,0.169457601001653));
#48666=CARTESIAN_POINT('Ctrl Pts',(-4.03335057326093,-1.,0.172535962484466));
#48667=CARTESIAN_POINT('Ctrl Pts',(-4.03335057326093,1.,0.172535962484466));
#48668=CARTESIAN_POINT('Ctrl Pts',(-4.04035407891161,-1.,0.175654339673757));
#48669=CARTESIAN_POINT('Ctrl Pts',(-4.04035407891161,1.,0.175654339673757));
#48670=CARTESIAN_POINT('Ctrl Pts',(-4.04734916719722,-1.,0.178812307240715));
#48671=CARTESIAN_POINT('Ctrl Pts',(-4.04734916719722,1.,0.178812307240715));
#48672=CARTESIAN_POINT('Ctrl Pts',(-4.05433660358402,-1.,0.18200945304855));
#48673=CARTESIAN_POINT('Ctrl Pts',(-4.05433660358402,1.,0.18200945304855));
#48674=CARTESIAN_POINT('Ctrl Pts',(-4.06131670998589,-1.,0.185245370038948));
#48675=CARTESIAN_POINT('Ctrl Pts',(-4.06131670998589,1.,0.185245370038948));
#48676=CARTESIAN_POINT('Ctrl Pts',(-4.06828941192308,-1.,0.188519658060255));
#48677=CARTESIAN_POINT('Ctrl Pts',(-4.06828941192308,1.,0.188519658060255));
#48678=CARTESIAN_POINT('Ctrl Pts',(-4.07525439703137,-1.,0.191831928181081));
#48679=CARTESIAN_POINT('Ctrl Pts',(-4.07525439703137,1.,0.191831928181081));
#48680=CARTESIAN_POINT('Ctrl Pts',(-4.08221124060385,-1.,0.195181806054714));
#48681=CARTESIAN_POINT('Ctrl Pts',(-4.08221124060385,1.,0.195181806054714));
#48682=CARTESIAN_POINT('Ctrl Pts',(-4.08915953359753,-1.,0.19856893480081));
#48683=CARTESIAN_POINT('Ctrl Pts',(-4.08915953359753,1.,0.19856893480081));
#48684=CARTESIAN_POINT('Ctrl Pts',(-4.09609903751912,-1.,0.201992979049984));
#48685=CARTESIAN_POINT('Ctrl Pts',(-4.09609903751912,1.,0.201992979049984));
#48686=CARTESIAN_POINT('Ctrl Pts',(-4.10302969965374,-1.,0.205453622198233));
#48687=CARTESIAN_POINT('Ctrl Pts',(-4.10302969965374,1.,0.205453622198233));
#48688=CARTESIAN_POINT('Ctrl Pts',(-4.10995157639026,-1.,0.208950559400172));
#48689=CARTESIAN_POINT('Ctrl Pts',(-4.10995157639026,1.,0.208950559400172));
#48690=CARTESIAN_POINT('Ctrl Pts',(-4.11686478264545,-1.,0.212483491087068));
#48691=CARTESIAN_POINT('Ctrl Pts',(-4.11686478264545,1.,0.212483491087068));
#48692=CARTESIAN_POINT('Ctrl Pts',(-4.12376943492249,-1.,0.216052116898425));
#48693=CARTESIAN_POINT('Ctrl Pts',(-4.12376943492249,1.,0.216052116898425));
#48694=CARTESIAN_POINT('Ctrl Pts',(-4.13066558698156,-1.,0.219656126701851));
#48695=CARTESIAN_POINT('Ctrl Pts',(-4.13066558698156,1.,0.219656126701851));
#48696=CARTESIAN_POINT('Ctrl Pts',(-4.13755320553563,-1.,0.223295201038383));
#48697=CARTESIAN_POINT('Ctrl Pts',(-4.13755320553563,1.,0.223295201038383));
#48698=CARTESIAN_POINT('Ctrl Pts',(-4.14443220607733,-1.,0.226969025061243));
#48699=CARTESIAN_POINT('Ctrl Pts',(-4.14443220607733,1.,0.226969025061243));
#48700=CARTESIAN_POINT('Ctrl Pts',(-4.15130247435029,-1.,0.230677299028738));
#48701=CARTESIAN_POINT('Ctrl Pts',(-4.15130247435029,1.,0.230677299028738));
#48702=CARTESIAN_POINT('Ctrl Pts',(-4.1581638926525,-1.,0.234419749543143));
#48703=CARTESIAN_POINT('Ctrl Pts',(-4.1581638926525,1.,0.234419749543143));
#48704=CARTESIAN_POINT('Ctrl Pts',(-4.1650163665385,-1.,0.238196140933976));
#48705=CARTESIAN_POINT('Ctrl Pts',(-4.1650163665385,1.,0.238196140933976));
#48706=CARTESIAN_POINT('Ctrl Pts',(-4.17185984409533,-1.,0.242006283923911));
#48707=CARTESIAN_POINT('Ctrl Pts',(-4.17185984409533,1.,0.242006283923911));
#48708=CARTESIAN_POINT('Ctrl Pts',(-4.17869430192868,-1.,0.245850033418583));
#48709=CARTESIAN_POINT('Ctrl Pts',(-4.17869430192868,1.,0.245850033418583));
#48710=CARTESIAN_POINT('Ctrl Pts',(-4.18415464959491,-1.,0.248951836910963));
#48711=CARTESIAN_POINT('Ctrl Pts',(-4.18415464959491,1.,0.248951836910963));
#48712=CARTESIAN_POINT('Ctrl Pts',(-4.18824585244066,-1.,0.251293239837692));
#48713=CARTESIAN_POINT('Ctrl Pts',(-4.18824585244066,1.,0.251293239837692));
#48714=CARTESIAN_POINT('Ctrl Pts',(-4.19097151819241,-1.,0.252860861572565));
#48715=CARTESIAN_POINT('Ctrl Pts',(-4.19097151819241,1.,0.252860861572565));
#48716=CARTESIAN_POINT('Ctrl Pts',(-4.1923339003649,-1.,0.253646344052521));
#48717=CARTESIAN_POINT('Ctrl Pts',(-4.1923339003649,1.,0.253646344052521));
#48718=CARTESIAN_POINT('',(-3.74888939116255,1.,0.0912596999166825));
#48719=CARTESIAN_POINT('Ctrl Pts',(-3.74888939116255,-1.,0.091259699916682));
#48720=CARTESIAN_POINT('Ctrl Pts',(-3.74888939116255,-0.666666666666667,
0.091259699916682));
#48721=CARTESIAN_POINT('Ctrl Pts',(-3.74888939116255,-0.333333333333333,
0.091259699916682));
#48722=CARTESIAN_POINT('Ctrl Pts',(-3.74888939116255,0.333333333333333,
0.091259699916682));
#48723=CARTESIAN_POINT('Ctrl Pts',(-3.74888939116255,0.666666666666667,
0.0912596999166817));
#48724=CARTESIAN_POINT('Ctrl Pts',(-3.74888939116255,1.,0.0912596999166817));
#48725=CARTESIAN_POINT('',(-4.1923339003649,1.,0.253646344052521));
#48726=CARTESIAN_POINT('',(-4.1923339003649,0.,0.253646344052521));
#48727=CARTESIAN_POINT('Ctrl Pts',(-3.74888939116255,1.,0.0912596999166823));
#48728=CARTESIAN_POINT('Ctrl Pts',(-3.74892890040974,1.,0.0912308016421982));
#48729=CARTESIAN_POINT('Ctrl Pts',(-3.74911539914542,1.,0.0911666301812817));
#48730=CARTESIAN_POINT('Ctrl Pts',(-3.74976844886346,1.,0.0911090736805509));
#48731=CARTESIAN_POINT('Ctrl Pts',(-3.75145357872422,1.,0.0911323999574425));
#48732=CARTESIAN_POINT('Ctrl Pts',(-3.75495560118212,1.,0.0913419622736397));
#48733=CARTESIAN_POINT('Ctrl Pts',(-3.76024199359303,1.,0.0917773084998334));
#48734=CARTESIAN_POINT('Ctrl Pts',(-3.76678860031841,1.,0.092409058960269));
#48735=CARTESIAN_POINT('Ctrl Pts',(-3.77424159971059,1.,0.0932185546203178));
#48736=CARTESIAN_POINT('Ctrl Pts',(-3.782205218991,1.,0.0941840095090813));
#48737=CARTESIAN_POINT('Ctrl Pts',(-3.79030016353111,1.,0.09528298851008));
#48738=CARTESIAN_POINT('Ctrl Pts',(-3.79822128513845,1.,0.0964949352873131));
#48739=CARTESIAN_POINT('Ctrl Pts',(-3.80581088847809,1.,0.0978042222906642));
#48740=CARTESIAN_POINT('Ctrl Pts',(-3.81306649386461,1.,0.0992008728096513));
#48741=CARTESIAN_POINT('Ctrl Pts',(-3.82007889742625,1.,0.100678769650632));
#48742=CARTESIAN_POINT('Ctrl Pts',(-3.82698737143255,1.,0.102234506488456));
#48743=CARTESIAN_POINT('Ctrl Pts',(-3.83393171228002,1.,0.103866063811622));
#48744=CARTESIAN_POINT('Ctrl Pts',(-3.84099658324803,1.,0.105571360916569));
#48745=CARTESIAN_POINT('Ctrl Pts',(-3.84819233070317,1.,0.107347597812183));
#48746=CARTESIAN_POINT('Ctrl Pts',(-3.855485714969,1.,0.109191717634943));
#48747=CARTESIAN_POINT('Ctrl Pts',(-3.86281867282965,1.,0.11110059303626));
#48748=CARTESIAN_POINT('Ctrl Pts',(-3.87013043445014,1.,0.113071304914561));
#48749=CARTESIAN_POINT('Ctrl Pts',(-3.87738168405343,1.,0.11510142664947));
#48750=CARTESIAN_POINT('Ctrl Pts',(-3.88456590045767,1.,0.117189150373144));
#48751=CARTESIAN_POINT('Ctrl Pts',(-3.89169600105201,1.,0.119333088190417));
#48752=CARTESIAN_POINT('Ctrl Pts',(-3.89879639336952,1.,0.121532144765723));
#48753=CARTESIAN_POINT('Ctrl Pts',(-3.90589336320508,1.,0.123785368272377));
#48754=CARTESIAN_POINT('Ctrl Pts',(-3.91300501605392,1.,0.126091793324136));
#48755=CARTESIAN_POINT('Ctrl Pts',(-3.92013513251642,1.,0.128450341339528));
#48756=CARTESIAN_POINT('Ctrl Pts',(-3.9272787679596,1.,0.130859892027798));
#48757=CARTESIAN_POINT('Ctrl Pts',(-3.93442567551035,1.,0.133319322794189));
#48758=CARTESIAN_POINT('Ctrl Pts',(-3.94156445130744,1.,0.135827558661188));
#48759=CARTESIAN_POINT('Ctrl Pts',(-3.94868667844355,1.,0.138383621255159));
#48760=CARTESIAN_POINT('Ctrl Pts',(-3.95579014116899,1.,0.140986665829937));
#48761=CARTESIAN_POINT('Ctrl Pts',(-3.96287658098896,1.,0.143635947692791));
#48762=CARTESIAN_POINT('Ctrl Pts',(-3.96995018565891,1.,0.146330797814513));
#48763=CARTESIAN_POINT('Ctrl Pts',(-3.97701581473643,1.,0.149070594803543));
#48764=CARTESIAN_POINT('Ctrl Pts',(-3.9840772985098,1.,0.151854737441405));
#48765=CARTESIAN_POINT('Ctrl Pts',(-3.99113582086059,1.,0.154682618338563));
#48766=CARTESIAN_POINT('Ctrl Pts',(-3.99819074631874,1.,0.157553634383809));
#48767=CARTESIAN_POINT('Ctrl Pts',(-4.00524031064509,1.,0.160467194882219));
#48768=CARTESIAN_POINT('Ctrl Pts',(-4.01228237022301,1.,0.163422730287458));
#48769=CARTESIAN_POINT('Ctrl Pts',(-4.01931510507143,1.,0.166419700015847));
#48770=CARTESIAN_POINT('Ctrl Pts',(-4.0263377970371,1.,0.169457601001653));
#48771=CARTESIAN_POINT('Ctrl Pts',(-4.03335057326093,1.,0.172535962484466));
#48772=CARTESIAN_POINT('Ctrl Pts',(-4.04035407891161,1.,0.175654339673757));
#48773=CARTESIAN_POINT('Ctrl Pts',(-4.04734916719722,1.,0.178812307240715));
#48774=CARTESIAN_POINT('Ctrl Pts',(-4.05433660358402,1.,0.18200945304855));
#48775=CARTESIAN_POINT('Ctrl Pts',(-4.06131670998589,1.,0.185245370038948));
#48776=CARTESIAN_POINT('Ctrl Pts',(-4.06828941192308,1.,0.188519658060255));
#48777=CARTESIAN_POINT('Ctrl Pts',(-4.07525439703137,1.,0.191831928181081));
#48778=CARTESIAN_POINT('Ctrl Pts',(-4.08221124060385,1.,0.195181806054714));
#48779=CARTESIAN_POINT('Ctrl Pts',(-4.08915953359753,1.,0.19856893480081));
#48780=CARTESIAN_POINT('Ctrl Pts',(-4.09609903751912,1.,0.201992979049984));
#48781=CARTESIAN_POINT('Ctrl Pts',(-4.10302969965374,1.,0.205453622198233));
#48782=CARTESIAN_POINT('Ctrl Pts',(-4.10995157639026,1.,0.208950559400172));
#48783=CARTESIAN_POINT('Ctrl Pts',(-4.11686478264545,1.,0.212483491087068));
#48784=CARTESIAN_POINT('Ctrl Pts',(-4.12376943492249,1.,0.216052116898425));
#48785=CARTESIAN_POINT('Ctrl Pts',(-4.13066558698156,1.,0.219656126701851));
#48786=CARTESIAN_POINT('Ctrl Pts',(-4.13755320553563,1.,0.223295201038383));
#48787=CARTESIAN_POINT('Ctrl Pts',(-4.14443220607733,1.,0.226969025061243));
#48788=CARTESIAN_POINT('Ctrl Pts',(-4.15130247435029,1.,0.230677299028738));
#48789=CARTESIAN_POINT('Ctrl Pts',(-4.1581638926525,1.,0.234419749543143));
#48790=CARTESIAN_POINT('Ctrl Pts',(-4.1650163665385,1.,0.238196140933976));
#48791=CARTESIAN_POINT('Ctrl Pts',(-4.17185984409533,1.,0.242006283923911));
#48792=CARTESIAN_POINT('Ctrl Pts',(-4.17869430192868,1.,0.245850033418583));
#48793=CARTESIAN_POINT('Ctrl Pts',(-4.18415464959491,1.,0.248951836910963));
#48794=CARTESIAN_POINT('Ctrl Pts',(-4.18824585244066,1.,0.251293239837692));
#48795=CARTESIAN_POINT('Ctrl Pts',(-4.19097151819241,1.,0.252860861572565));
#48796=CARTESIAN_POINT('Ctrl Pts',(-4.1923339003649,1.,0.253646344052521));
#48797=CARTESIAN_POINT('Origin',(-4.1923339003649,0.,0.253646344052521));
#48798=CARTESIAN_POINT('',(-4.18039834341342,1.,0.405301974318349));
#48799=CARTESIAN_POINT('Origin',(0.,0.,0.));
#48800=CARTESIAN_POINT('',(-3.74888939116259,1.,-0.0912596999148852));
#48801=CARTESIAN_POINT('Origin',(0.,1.,0.));
#48802=CARTESIAN_POINT('Ctrl Pts',(-3.74888939116259,1.,-0.091259699914886));
#48803=CARTESIAN_POINT('Ctrl Pts',(-3.74888939116259,0.666666666666667,
-0.091259699914886));
#48804=CARTESIAN_POINT('Ctrl Pts',(-3.74888939116259,0.333333333333333,
-0.091259699914886));
#48805=CARTESIAN_POINT('Ctrl Pts',(-3.74888939116259,-0.333333333333333,
-0.091259699914886));
#48806=CARTESIAN_POINT('Ctrl Pts',(-3.74888939116259,-0.666666666666667,
-0.0912596999148857));
#48807=CARTESIAN_POINT('Ctrl Pts',(-3.74888939116259,-1.,-0.0912596999148857));
#48808=CARTESIAN_POINT('Ctrl Pts',(-4.1923339003649,-1.,-0.253646344052522));
#48809=CARTESIAN_POINT('Ctrl Pts',(-4.1923339003649,1.,-0.253646344052522));
#48810=CARTESIAN_POINT('Ctrl Pts',(-4.19097151819684,-1.,-0.25286086157284));
#48811=CARTESIAN_POINT('Ctrl Pts',(-4.19097151819684,1.,-0.25286086157284));
#48812=CARTESIAN_POINT('Ctrl Pts',(-4.18824585245272,-1.,-0.251293239838441));
#48813=CARTESIAN_POINT('Ctrl Pts',(-4.18824585245272,1.,-0.251293239838441));
#48814=CARTESIAN_POINT('Ctrl Pts',(-4.18415464961466,-1.,-0.248951836912189));
#48815=CARTESIAN_POINT('Ctrl Pts',(-4.18415464961466,1.,-0.248951836912189));
#48816=CARTESIAN_POINT('Ctrl Pts',(-4.1786943019518,-1.,-0.245850033420019));
#48817=CARTESIAN_POINT('Ctrl Pts',(-4.1786943019518,1.,-0.245850033420019));
#48818=CARTESIAN_POINT('Ctrl Pts',(-4.17185984411426,-1.,-0.242006283925088));
#48819=CARTESIAN_POINT('Ctrl Pts',(-4.17185984411426,1.,-0.242006283925088));
#48820=CARTESIAN_POINT('Ctrl Pts',(-4.16501636654877,-1.,-0.238196140934616));
#48821=CARTESIAN_POINT('Ctrl Pts',(-4.16501636654877,1.,-0.238196140934616));
#48822=CARTESIAN_POINT('Ctrl Pts',(-4.15816389265352,-1.,-0.234419749543208));
#48823=CARTESIAN_POINT('Ctrl Pts',(-4.15816389265352,1.,-0.234419749543208));
#48824=CARTESIAN_POINT('Ctrl Pts',(-4.15130247434459,-1.,-0.230677299028383));
#48825=CARTESIAN_POINT('Ctrl Pts',(-4.15130247434459,1.,-0.230677299028383));
#48826=CARTESIAN_POINT('Ctrl Pts',(-4.14443220606869,-1.,-0.226969025060705));
#48827=CARTESIAN_POINT('Ctrl Pts',(-4.14443220606869,1.,-0.226969025060705));
#48828=CARTESIAN_POINT('Ctrl Pts',(-4.13755320552764,-1.,-0.223295201037886));
#48829=CARTESIAN_POINT('Ctrl Pts',(-4.13755320552764,1.,-0.223295201037886));
#48830=CARTESIAN_POINT('Ctrl Pts',(-4.13066558697658,-1.,-0.219656126701541));
#48831=CARTESIAN_POINT('Ctrl Pts',(-4.13066558697658,1.,-0.219656126701541));
#48832=CARTESIAN_POINT('Ctrl Pts',(-4.12376943492132,-1.,-0.216052116898352));
#48833=CARTESIAN_POINT('Ctrl Pts',(-4.12376943492132,1.,-0.216052116898352));
#48834=CARTESIAN_POINT('Ctrl Pts',(-4.11686478264739,-1.,-0.21248349108719));
#48835=CARTESIAN_POINT('Ctrl Pts',(-4.11686478264739,1.,-0.21248349108719));
#48836=CARTESIAN_POINT('Ctrl Pts',(-4.10995157639377,-1.,-0.208950559400392));
#48837=CARTESIAN_POINT('Ctrl Pts',(-4.10995157639377,1.,-0.208950559400392));
#48838=CARTESIAN_POINT('Ctrl Pts',(-4.10302969965728,-1.,-0.205453622198455));
#48839=CARTESIAN_POINT('Ctrl Pts',(-4.10302969965728,1.,-0.205453622198455));
#48840=CARTESIAN_POINT('Ctrl Pts',(-4.09609903752152,-1.,-0.201992979050136));
#48841=CARTESIAN_POINT('Ctrl Pts',(-4.09609903752152,1.,-0.201992979050136));
#48842=CARTESIAN_POINT('Ctrl Pts',(-4.08915953359833,-1.,-0.198568934800862));
#48843=CARTESIAN_POINT('Ctrl Pts',(-4.08915953359833,1.,-0.198568934800862));
#48844=CARTESIAN_POINT('Ctrl Pts',(-4.08221124060322,-1.,-0.195181806054676));
#48845=CARTESIAN_POINT('Ctrl Pts',(-4.08221124060322,1.,-0.195181806054676));
#48846=CARTESIAN_POINT('Ctrl Pts',(-4.07525439702992,-1.,-0.191831928180991));
#48847=CARTESIAN_POINT('Ctrl Pts',(-4.07525439702992,1.,-0.191831928180991));
#48848=CARTESIAN_POINT('Ctrl Pts',(-4.06828941192148,-1.,-0.188519658060155));
#48849=CARTESIAN_POINT('Ctrl Pts',(-4.06828941192148,1.,-0.188519658060155));
#48850=CARTESIAN_POINT('Ctrl Pts',(-4.06131670998469,-1.,-0.185245370038874));
#48851=CARTESIAN_POINT('Ctrl Pts',(-4.06131670998469,1.,-0.185245370038874));
#48852=CARTESIAN_POINT('Ctrl Pts',(-4.05433660358353,-1.,-0.18200945304852));
#48853=CARTESIAN_POINT('Ctrl Pts',(-4.05433660358353,1.,-0.18200945304852));
#48854=CARTESIAN_POINT('Ctrl Pts',(-4.04734916719741,-1.,-0.178812307240728));
#48855=CARTESIAN_POINT('Ctrl Pts',(-4.04734916719741,1.,-0.178812307240728));
#48856=CARTESIAN_POINT('Ctrl Pts',(-4.04035407891222,-1.,-0.175654339673797));
#48857=CARTESIAN_POINT('Ctrl Pts',(-4.04035407891222,1.,-0.175654339673797));
#48858=CARTESIAN_POINT('Ctrl Pts',(-4.03335057326163,-1.,-0.172535962484514));
#48859=CARTESIAN_POINT('Ctrl Pts',(-4.03335057326163,1.,-0.172535962484514));
#48860=CARTESIAN_POINT('Ctrl Pts',(-4.02633779703764,-1.,-0.169457601001691));
#48861=CARTESIAN_POINT('Ctrl Pts',(-4.02633779703764,1.,-0.169457601001691));
#48862=CARTESIAN_POINT('Ctrl Pts',(-4.01931510507167,-1.,-0.166419700015866));
#48863=CARTESIAN_POINT('Ctrl Pts',(-4.01931510507167,1.,-0.166419700015866));
#48864=CARTESIAN_POINT('Ctrl Pts',(-4.01228237022296,-1.,-0.163422730287456));
#48865=CARTESIAN_POINT('Ctrl Pts',(-4.01228237022296,1.,-0.163422730287456));
#48866=CARTESIAN_POINT('Ctrl Pts',(-4.00524031064487,-1.,-0.160467194882203));
#48867=CARTESIAN_POINT('Ctrl Pts',(-4.00524031064487,1.,-0.160467194882203));
#48868=CARTESIAN_POINT('Ctrl Pts',(-3.9981907463185,-1.,-0.15755363438379));
#48869=CARTESIAN_POINT('Ctrl Pts',(-3.9981907463185,1.,-0.15755363438379));
#48870=CARTESIAN_POINT('Ctrl Pts',(-3.99113582086043,-1.,-0.154682618338547));
#48871=CARTESIAN_POINT('Ctrl Pts',(-3.99113582086043,1.,-0.154682618338547));
#48872=CARTESIAN_POINT('Ctrl Pts',(-3.98407729850975,-1.,-0.151854737441398));
#48873=CARTESIAN_POINT('Ctrl Pts',(-3.98407729850975,1.,-0.151854737441398));
#48874=CARTESIAN_POINT('Ctrl Pts',(-3.97701581473644,-1.,-0.149070594803545));
#48875=CARTESIAN_POINT('Ctrl Pts',(-3.97701581473644,1.,-0.149070594803545));
#48876=CARTESIAN_POINT('Ctrl Pts',(-3.96995018565893,-1.,-0.14633079781452));
#48877=CARTESIAN_POINT('Ctrl Pts',(-3.96995018565893,1.,-0.14633079781452));
#48878=CARTESIAN_POINT('Ctrl Pts',(-3.96287658098896,-1.,-0.143635947692799));
#48879=CARTESIAN_POINT('Ctrl Pts',(-3.96287658098896,1.,-0.143635947692799));
#48880=CARTESIAN_POINT('Ctrl Pts',(-3.95579014116894,-1.,-0.140986665829942));
#48881=CARTESIAN_POINT('Ctrl Pts',(-3.95579014116894,1.,-0.140986665829942));
#48882=CARTESIAN_POINT('Ctrl Pts',(-3.94868667844347,-1.,-0.138383621255161));
#48883=CARTESIAN_POINT('Ctrl Pts',(-3.94868667844347,1.,-0.138383621255161));
#48884=CARTESIAN_POINT('Ctrl Pts',(-3.94156445130741,-1.,-0.135827558661188));
#48885=CARTESIAN_POINT('Ctrl Pts',(-3.94156445130741,1.,-0.135827558661188));
#48886=CARTESIAN_POINT('Ctrl Pts',(-3.93442567551042,-1.,-0.133319322794191));
#48887=CARTESIAN_POINT('Ctrl Pts',(-3.93442567551042,1.,-0.133319322794191));
#48888=CARTESIAN_POINT('Ctrl Pts',(-3.92727876795977,-1.,-0.130859892027801));
#48889=CARTESIAN_POINT('Ctrl Pts',(-3.92727876795977,1.,-0.130859892027801));
#48890=CARTESIAN_POINT('Ctrl Pts',(-3.92013513251664,-1.,-0.128450341339532));
#48891=CARTESIAN_POINT('Ctrl Pts',(-3.92013513251664,1.,-0.128450341339532));
#48892=CARTESIAN_POINT('Ctrl Pts',(-3.91300501605411,-1.,-0.126091793324141));
#48893=CARTESIAN_POINT('Ctrl Pts',(-3.91300501605411,1.,-0.126091793324141));
#48894=CARTESIAN_POINT('Ctrl Pts',(-3.90589336320515,-1.,-0.12378536827238));
#48895=CARTESIAN_POINT('Ctrl Pts',(-3.90589336320515,1.,-0.12378536827238));
#48896=CARTESIAN_POINT('Ctrl Pts',(-3.89879639336939,-1.,-0.121532144765721));
#48897=CARTESIAN_POINT('Ctrl Pts',(-3.89879639336939,1.,-0.121532144765721));
#48898=CARTESIAN_POINT('Ctrl Pts',(-3.8916960010517,-1.,-0.11933308819041));
#48899=CARTESIAN_POINT('Ctrl Pts',(-3.8916960010517,1.,-0.11933308819041));
#48900=CARTESIAN_POINT('Ctrl Pts',(-3.88456590045726,-1.,-0.117189150373134));
#48901=CARTESIAN_POINT('Ctrl Pts',(-3.88456590045726,1.,-0.117189150373134));
#48902=CARTESIAN_POINT('Ctrl Pts',(-3.87738168405308,-1.,-0.115101426649461));
#48903=CARTESIAN_POINT('Ctrl Pts',(-3.87738168405308,1.,-0.115101426649461));
#48904=CARTESIAN_POINT('Ctrl Pts',(-3.87013043445001,-1.,-0.113071304914559));
#48905=CARTESIAN_POINT('Ctrl Pts',(-3.87013043445001,1.,-0.113071304914559));
#48906=CARTESIAN_POINT('Ctrl Pts',(-3.86281867282984,-1.,-0.111100593036267));
#48907=CARTESIAN_POINT('Ctrl Pts',(-3.86281867282984,1.,-0.111100593036267));
#48908=CARTESIAN_POINT('Ctrl Pts',(-3.85548571496953,-1.,-0.109191717634961));
#48909=CARTESIAN_POINT('Ctrl Pts',(-3.85548571496953,1.,-0.109191717634961));
#48910=CARTESIAN_POINT('Ctrl Pts',(-3.84819233070391,-1.,-0.107347597812208));
#48911=CARTESIAN_POINT('Ctrl Pts',(-3.84819233070391,1.,-0.107347597812208));
#48912=CARTESIAN_POINT('Ctrl Pts',(-3.84099658324873,-1.,-0.105571360916593));
#48913=CARTESIAN_POINT('Ctrl Pts',(-3.84099658324873,1.,-0.105571360916593));
#48914=CARTESIAN_POINT('Ctrl Pts',(-3.83393171228034,-1.,-0.103866063811634));
#48915=CARTESIAN_POINT('Ctrl Pts',(-3.83393171228034,1.,-0.103866063811634));
#48916=CARTESIAN_POINT('Ctrl Pts',(-3.8269873714322,-1.,-0.102234506488445));
#48917=CARTESIAN_POINT('Ctrl Pts',(-3.8269873714322,1.,-0.102234506488445));
#48918=CARTESIAN_POINT('Ctrl Pts',(-3.82007889742512,-1.,-0.100678769650594));
#48919=CARTESIAN_POINT('Ctrl Pts',(-3.82007889742512,1.,-0.100678769650594));
#48920=CARTESIAN_POINT('Ctrl Pts',(-3.81306649386293,-1.,-0.0992008728095943));
#48921=CARTESIAN_POINT('Ctrl Pts',(-3.81306649386293,1.,-0.0992008728095943));
#48922=CARTESIAN_POINT('Ctrl Pts',(-3.80581088847642,-1.,-0.0978042222906075));
#48923=CARTESIAN_POINT('Ctrl Pts',(-3.80581088847642,1.,-0.0978042222906075));
#48924=CARTESIAN_POINT('Ctrl Pts',(-3.7982212851376,-1.,-0.0964949352872844));
#48925=CARTESIAN_POINT('Ctrl Pts',(-3.7982212851376,1.,-0.0964949352872844));
#48926=CARTESIAN_POINT('Ctrl Pts',(-3.79030016353186,-1.,-0.0952829885101068));
#48927=CARTESIAN_POINT('Ctrl Pts',(-3.79030016353186,1.,-0.0952829885101068));
#48928=CARTESIAN_POINT('Ctrl Pts',(-3.78220521899366,-1.,-0.0941840095091744));
#48929=CARTESIAN_POINT('Ctrl Pts',(-3.78220521899366,1.,-0.0941840095091744));
#48930=CARTESIAN_POINT('Ctrl Pts',(-3.77424159971456,-1.,-0.0932185546204574));
#48931=CARTESIAN_POINT('Ctrl Pts',(-3.77424159971456,1.,-0.0932185546204574));
#48932=CARTESIAN_POINT('Ctrl Pts',(-3.76678860032228,-1.,-0.0924090589604056));
#48933=CARTESIAN_POINT('Ctrl Pts',(-3.76678860032228,1.,-0.0924090589604056));
#48934=CARTESIAN_POINT('Ctrl Pts',(-3.76024199359493,-1.,-0.0917773084999007));
#48935=CARTESIAN_POINT('Ctrl Pts',(-3.76024199359493,1.,-0.0917773084999007));
#48936=CARTESIAN_POINT('Ctrl Pts',(-3.75495560118053,-1.,-0.0913419622735852));
#48937=CARTESIAN_POINT('Ctrl Pts',(-3.75495560118053,1.,-0.0913419622735852));
#48938=CARTESIAN_POINT('Ctrl Pts',(-3.75116949194125,-1.,-0.0911154000996406));
#48939=CARTESIAN_POINT('Ctrl Pts',(-3.75116949194125,1.,-0.0911154000996406));
#48940=CARTESIAN_POINT('Ctrl Pts',(-3.74943097853257,-1.,-0.091105754750466));
#48941=CARTESIAN_POINT('Ctrl Pts',(-3.74943097853257,1.,-0.091105754750466));
#48942=CARTESIAN_POINT('Ctrl Pts',(-3.7488701717383,-1.,-0.0911958743733925));
#48943=CARTESIAN_POINT('Ctrl Pts',(-3.7488701717383,1.,-0.0911958743733925));
#48944=CARTESIAN_POINT('Ctrl Pts',(-3.74882632118923,-1.,-0.0912992005792091));
#48945=CARTESIAN_POINT('Ctrl Pts',(-3.74882632118923,1.,-0.0912992005792091));
#48946=CARTESIAN_POINT('Ctrl Pts',(-3.74888690736767,-1.,-0.0913616755937429));
#48947=CARTESIAN_POINT('Ctrl Pts',(-3.74888690736767,1.,-0.0913616755937429));
#48948=CARTESIAN_POINT('',(-4.1923339003649,1.,-0.253646344052522));
#48949=CARTESIAN_POINT('Ctrl Pts',(-4.1923339003649,1.,-0.253646344052522));
#48950=CARTESIAN_POINT('Ctrl Pts',(-4.19097151819684,1.,-0.25286086157284));
#48951=CARTESIAN_POINT('Ctrl Pts',(-4.18824585245272,1.,-0.251293239838441));
#48952=CARTESIAN_POINT('Ctrl Pts',(-4.18415464961466,1.,-0.248951836912189));
#48953=CARTESIAN_POINT('Ctrl Pts',(-4.1786943019518,1.,-0.245850033420019));
#48954=CARTESIAN_POINT('Ctrl Pts',(-4.17185984411426,1.,-0.242006283925088));
#48955=CARTESIAN_POINT('Ctrl Pts',(-4.16501636654877,1.,-0.238196140934616));
#48956=CARTESIAN_POINT('Ctrl Pts',(-4.15816389265352,1.,-0.234419749543208));
#48957=CARTESIAN_POINT('Ctrl Pts',(-4.15130247434459,1.,-0.230677299028383));
#48958=CARTESIAN_POINT('Ctrl Pts',(-4.14443220606869,1.,-0.226969025060705));
#48959=CARTESIAN_POINT('Ctrl Pts',(-4.13755320552764,1.,-0.223295201037886));
#48960=CARTESIAN_POINT('Ctrl Pts',(-4.13066558697658,1.,-0.219656126701541));
#48961=CARTESIAN_POINT('Ctrl Pts',(-4.12376943492132,1.,-0.216052116898352));
#48962=CARTESIAN_POINT('Ctrl Pts',(-4.11686478264739,1.,-0.21248349108719));
#48963=CARTESIAN_POINT('Ctrl Pts',(-4.10995157639377,1.,-0.208950559400392));
#48964=CARTESIAN_POINT('Ctrl Pts',(-4.10302969965728,1.,-0.205453622198455));
#48965=CARTESIAN_POINT('Ctrl Pts',(-4.09609903752152,1.,-0.201992979050136));
#48966=CARTESIAN_POINT('Ctrl Pts',(-4.08915953359833,1.,-0.198568934800862));
#48967=CARTESIAN_POINT('Ctrl Pts',(-4.08221124060322,1.,-0.195181806054676));
#48968=CARTESIAN_POINT('Ctrl Pts',(-4.07525439702992,1.,-0.191831928180991));
#48969=CARTESIAN_POINT('Ctrl Pts',(-4.06828941192148,1.,-0.188519658060155));
#48970=CARTESIAN_POINT('Ctrl Pts',(-4.06131670998469,1.,-0.185245370038874));
#48971=CARTESIAN_POINT('Ctrl Pts',(-4.05433660358353,1.,-0.18200945304852));
#48972=CARTESIAN_POINT('Ctrl Pts',(-4.04734916719741,1.,-0.178812307240728));
#48973=CARTESIAN_POINT('Ctrl Pts',(-4.04035407891222,1.,-0.175654339673797));
#48974=CARTESIAN_POINT('Ctrl Pts',(-4.03335057326163,1.,-0.172535962484514));
#48975=CARTESIAN_POINT('Ctrl Pts',(-4.02633779703764,1.,-0.169457601001691));
#48976=CARTESIAN_POINT('Ctrl Pts',(-4.01931510507167,1.,-0.166419700015866));
#48977=CARTESIAN_POINT('Ctrl Pts',(-4.01228237022296,1.,-0.163422730287456));
#48978=CARTESIAN_POINT('Ctrl Pts',(-4.00524031064487,1.,-0.160467194882203));
#48979=CARTESIAN_POINT('Ctrl Pts',(-3.9981907463185,1.,-0.15755363438379));
#48980=CARTESIAN_POINT('Ctrl Pts',(-3.99113582086043,1.,-0.154682618338547));
#48981=CARTESIAN_POINT('Ctrl Pts',(-3.98407729850975,1.,-0.151854737441398));
#48982=CARTESIAN_POINT('Ctrl Pts',(-3.97701581473644,1.,-0.149070594803545));
#48983=CARTESIAN_POINT('Ctrl Pts',(-3.96995018565893,1.,-0.14633079781452));
#48984=CARTESIAN_POINT('Ctrl Pts',(-3.96287658098896,1.,-0.143635947692799));
#48985=CARTESIAN_POINT('Ctrl Pts',(-3.95579014116894,1.,-0.140986665829942));
#48986=CARTESIAN_POINT('Ctrl Pts',(-3.94868667844347,1.,-0.138383621255161));
#48987=CARTESIAN_POINT('Ctrl Pts',(-3.94156445130741,1.,-0.135827558661188));
#48988=CARTESIAN_POINT('Ctrl Pts',(-3.93442567551042,1.,-0.133319322794191));
#48989=CARTESIAN_POINT('Ctrl Pts',(-3.92727876795977,1.,-0.130859892027801));
#48990=CARTESIAN_POINT('Ctrl Pts',(-3.92013513251664,1.,-0.128450341339532));
#48991=CARTESIAN_POINT('Ctrl Pts',(-3.91300501605411,1.,-0.126091793324141));
#48992=CARTESIAN_POINT('Ctrl Pts',(-3.90589336320515,1.,-0.12378536827238));
#48993=CARTESIAN_POINT('Ctrl Pts',(-3.89879639336939,1.,-0.121532144765721));
#48994=CARTESIAN_POINT('Ctrl Pts',(-3.8916960010517,1.,-0.11933308819041));
#48995=CARTESIAN_POINT('Ctrl Pts',(-3.88456590045726,1.,-0.117189150373134));
#48996=CARTESIAN_POINT('Ctrl Pts',(-3.87738168405308,1.,-0.115101426649461));
#48997=CARTESIAN_POINT('Ctrl Pts',(-3.87013043445001,1.,-0.113071304914559));
#48998=CARTESIAN_POINT('Ctrl Pts',(-3.86281867282984,1.,-0.111100593036267));
#48999=CARTESIAN_POINT('Ctrl Pts',(-3.85548571496953,1.,-0.109191717634961));
#49000=CARTESIAN_POINT('Ctrl Pts',(-3.84819233070391,1.,-0.107347597812208));
#49001=CARTESIAN_POINT('Ctrl Pts',(-3.84099658324873,1.,-0.105571360916593));
#49002=CARTESIAN_POINT('Ctrl Pts',(-3.83393171228034,1.,-0.103866063811634));
#49003=CARTESIAN_POINT('Ctrl Pts',(-3.8269873714322,1.,-0.102234506488445));
#49004=CARTESIAN_POINT('Ctrl Pts',(-3.82007889742512,1.,-0.100678769650594));
#49005=CARTESIAN_POINT('Ctrl Pts',(-3.81306649386293,1.,-0.0992008728095943));
#49006=CARTESIAN_POINT('Ctrl Pts',(-3.80581088847642,1.,-0.0978042222906075));
#49007=CARTESIAN_POINT('Ctrl Pts',(-3.7982212851376,1.,-0.0964949352872844));
#49008=CARTESIAN_POINT('Ctrl Pts',(-3.79030016353186,1.,-0.0952829885101068));
#49009=CARTESIAN_POINT('Ctrl Pts',(-3.78220521899366,1.,-0.0941840095091744));
#49010=CARTESIAN_POINT('Ctrl Pts',(-3.77424159971456,1.,-0.0932185546204574));
#49011=CARTESIAN_POINT('Ctrl Pts',(-3.76678860032228,1.,-0.0924090589604056));
#49012=CARTESIAN_POINT('Ctrl Pts',(-3.76024199359493,1.,-0.0917773084999007));
#49013=CARTESIAN_POINT('Ctrl Pts',(-3.75495560118053,1.,-0.0913419622735852));
#49014=CARTESIAN_POINT('Ctrl Pts',(-3.75145357872511,1.,-0.0911323999576144));
#49015=CARTESIAN_POINT('Ctrl Pts',(-3.74976844886495,1.,-0.0911090736804571));
#49016=CARTESIAN_POINT('Ctrl Pts',(-3.74911539914664,1.,-0.0911666301806425));
#49017=CARTESIAN_POINT('Ctrl Pts',(-3.74892890041021,1.,-0.0912308016409232));
#49018=CARTESIAN_POINT('Ctrl Pts',(-3.74888939116259,1.,-0.0912596999148857));
#49019=CARTESIAN_POINT('',(-4.1923339003649,0.,-0.253646344052522));
#49020=CARTESIAN_POINT('Ctrl Pts',(-3.71702400346349,-1.,-0.496218256089212));
#49021=CARTESIAN_POINT('Ctrl Pts',(-3.71702400346349,1.,-0.496218256089212));
#49022=CARTESIAN_POINT('Ctrl Pts',(-3.7169543899574,-1.,-0.496270484166409));
#49023=CARTESIAN_POINT('Ctrl Pts',(-3.7169543899574,1.,-0.496270484166409));
#49024=CARTESIAN_POINT('Ctrl Pts',(-3.71698153685602,-1.,-0.49637939799264));
#49025=CARTESIAN_POINT('Ctrl Pts',(-3.71698153685602,1.,-0.49637939799264));
#49026=CARTESIAN_POINT('Ctrl Pts',(-3.71752134137482,-1.,-0.496556137604532));
#49027=CARTESIAN_POINT('Ctrl Pts',(-3.71752134137482,1.,-0.496556137604532));
#49028=CARTESIAN_POINT('Ctrl Pts',(-3.71923995966302,-1.,-0.496818574420596));
#49029=CARTESIAN_POINT('Ctrl Pts',(-3.71923995966302,1.,-0.496818574420596));
#49030=CARTESIAN_POINT('Ctrl Pts',(-3.72301489774398,-1.,-0.497187079575988));
#49031=CARTESIAN_POINT('Ctrl Pts',(-3.72301489774398,1.,-0.497187079575988));
#49032=CARTESIAN_POINT('Ctrl Pts',(-3.72830430904606,-1.,-0.497584067153049));
#49033=CARTESIAN_POINT('Ctrl Pts',(-3.72830430904606,1.,-0.497584067153049));
#49034=CARTESIAN_POINT('Ctrl Pts',(-3.73486914372449,-1.,-0.497984209510024));
#49035=CARTESIAN_POINT('Ctrl Pts',(-3.73486914372449,1.,-0.497984209510024));
#49036=CARTESIAN_POINT('Ctrl Pts',(-3.74235701734714,-1.,-0.498350586057692));
#49037=CARTESIAN_POINT('Ctrl Pts',(-3.74235701734714,1.,-0.498350586057692));
#49038=CARTESIAN_POINT('Ctrl Pts',(-3.75037362167839,-1.,-0.498642802042606));
#49039=CARTESIAN_POINT('Ctrl Pts',(-3.75037362167839,1.,-0.498642802042606));
#49040=CARTESIAN_POINT('Ctrl Pts',(-3.75854082221053,-1.,-0.498823681615422));
#49041=CARTESIAN_POINT('Ctrl Pts',(-3.75854082221053,1.,-0.498823681615422));
#49042=CARTESIAN_POINT('Ctrl Pts',(-3.76655401191229,-1.,-0.49886579233529));
#49043=CARTESIAN_POINT('Ctrl Pts',(-3.76655401191229,1.,-0.49886579233529));
#49044=CARTESIAN_POINT('Ctrl Pts',(-3.77425499225255,-1.,-0.498759900365892));
#49045=CARTESIAN_POINT('Ctrl Pts',(-3.77425499225255,1.,-0.498759900365892));
#49046=CARTESIAN_POINT('Ctrl Pts',(-3.78163975337356,-1.,-0.498515471679585));
#49047=CARTESIAN_POINT('Ctrl Pts',(-3.78163975337356,1.,-0.498515471679585));
#49048=CARTESIAN_POINT('Ctrl Pts',(-3.78879701661264,-1.,-0.498152751800958));
#49049=CARTESIAN_POINT('Ctrl Pts',(-3.78879701661264,1.,-0.498152751800958));
#49050=CARTESIAN_POINT('Ctrl Pts',(-3.79586380669994,-1.,-0.497696892100625));
#49051=CARTESIAN_POINT('Ctrl Pts',(-3.79586380669994,1.,-0.497696892100625));
#49052=CARTESIAN_POINT('Ctrl Pts',(-3.80297788298514,-1.,-0.497171756201052));
#49053=CARTESIAN_POINT('Ctrl Pts',(-3.80297788298514,1.,-0.497171756201052));
#49054=CARTESIAN_POINT('Ctrl Pts',(-3.81022254090839,-1.,-0.496592643443704));
#49055=CARTESIAN_POINT('Ctrl Pts',(-3.81022254090839,1.,-0.496592643443704));
#49056=CARTESIAN_POINT('Ctrl Pts',(-3.81760756144025,-1.,-0.49596393787548));
#49057=CARTESIAN_POINT('Ctrl Pts',(-3.81760756144025,1.,-0.49596393787548));
#49058=CARTESIAN_POINT('Ctrl Pts',(-3.82509963594103,-1.,-0.495283458893837));
#49059=CARTESIAN_POINT('Ctrl Pts',(-3.82509963594103,1.,-0.495283458893837));
#49060=CARTESIAN_POINT('Ctrl Pts',(-3.83264092682431,-1.,-0.494545212256401));
#49061=CARTESIAN_POINT('Ctrl Pts',(-3.83264092682431,1.,-0.494545212256401));
#49062=CARTESIAN_POINT('Ctrl Pts',(-3.84017095578451,-1.,-0.493742574629134));
#49063=CARTESIAN_POINT('Ctrl Pts',(-3.84017095578451,1.,-0.493742574629134));
#49064=CARTESIAN_POINT('Ctrl Pts',(-3.84765051147999,-1.,-0.492871792414141));
#49065=CARTESIAN_POINT('Ctrl Pts',(-3.84765051147999,1.,-0.492871792414141));
#49066=CARTESIAN_POINT('Ctrl Pts',(-3.85507287020263,-1.,-0.491933631083813));
#49067=CARTESIAN_POINT('Ctrl Pts',(-3.85507287020263,1.,-0.491933631083813));
#49068=CARTESIAN_POINT('Ctrl Pts',(-3.86245057319246,-1.,-0.490931482170891));
#49069=CARTESIAN_POINT('Ctrl Pts',(-3.86245057319246,1.,-0.490931482170891));
#49070=CARTESIAN_POINT('Ctrl Pts',(-3.86980755613707,-1.,-0.489870245704918));
#49071=CARTESIAN_POINT('Ctrl Pts',(-3.86980755613707,1.,-0.489870245704918));
#49072=CARTESIAN_POINT('Ctrl Pts',(-3.87716963231109,-1.,-0.488754973798274));
#49073=CARTESIAN_POINT('Ctrl Pts',(-3.87716963231109,1.,-0.488754973798274));
#49074=CARTESIAN_POINT('Ctrl Pts',(-3.88455453328138,-1.,-0.487589452275154));
#49075=CARTESIAN_POINT('Ctrl Pts',(-3.88455453328138,1.,-0.487589452275154));
#49076=CARTESIAN_POINT('Ctrl Pts',(-3.89196582437552,-1.,-0.486375337854103));
#49077=CARTESIAN_POINT('Ctrl Pts',(-3.89196582437552,1.,-0.486375337854103));
#49078=CARTESIAN_POINT('Ctrl Pts',(-3.89939844658513,-1.,-0.485112963522222));
#49079=CARTESIAN_POINT('Ctrl Pts',(-3.89939844658513,1.,-0.485112963522222));
#49080=CARTESIAN_POINT('Ctrl Pts',(-3.90684210358056,-1.,-0.48380183508915));
#49081=CARTESIAN_POINT('Ctrl Pts',(-3.90684210358056,1.,-0.48380183508915));
#49082=CARTESIAN_POINT('Ctrl Pts',(-3.91428536373751,-1.,-0.482441230340713));
#49083=CARTESIAN_POINT('Ctrl Pts',(-3.91428536373751,1.,-0.482441230340713));
#49084=CARTESIAN_POINT('Ctrl Pts',(-3.92171976072341,-1.,-0.481030798910748));
#49085=CARTESIAN_POINT('Ctrl Pts',(-3.92171976072341,1.,-0.481030798910748));
#49086=CARTESIAN_POINT('Ctrl Pts',(-3.92914297392071,-1.,-0.479571028525579));
#49087=CARTESIAN_POINT('Ctrl Pts',(-3.92914297392071,1.,-0.479571028525579));
#49088=CARTESIAN_POINT('Ctrl Pts',(-3.93655660689819,-1.,-0.478062927140964));
#49089=CARTESIAN_POINT('Ctrl Pts',(-3.93655660689819,1.,-0.478062927140964));
#49090=CARTESIAN_POINT('Ctrl Pts',(-3.94396469119383,-1.,-0.476507810658537));
#49091=CARTESIAN_POINT('Ctrl Pts',(-3.94396469119383,1.,-0.476507810658537));
#49092=CARTESIAN_POINT('Ctrl Pts',(-3.95137192932897,-1.,-0.47490705302179));
#49093=CARTESIAN_POINT('Ctrl Pts',(-3.95137192932897,1.,-0.47490705302179));
#49094=CARTESIAN_POINT('Ctrl Pts',(-3.95878201038338,-1.,-0.473261847236297));
#49095=CARTESIAN_POINT('Ctrl Pts',(-3.95878201038338,1.,-0.473261847236297));
#49096=CARTESIAN_POINT('Ctrl Pts',(-3.96619600864643,-1.,-0.471572978413503));
#49097=CARTESIAN_POINT('Ctrl Pts',(-3.96619600864643,1.,-0.471572978413503));
#49098=CARTESIAN_POINT('Ctrl Pts',(-3.97361320212436,-1.,-0.469840942829895));
#49099=CARTESIAN_POINT('Ctrl Pts',(-3.97361320212436,1.,-0.469840942829895));
#49100=CARTESIAN_POINT('Ctrl Pts',(-3.98103175589371,-1.,-0.468066047920157));
#49101=CARTESIAN_POINT('Ctrl Pts',(-3.98103175589371,1.,-0.468066047920157));
#49102=CARTESIAN_POINT('Ctrl Pts',(-3.98844946363262,-1.,-0.46624852088304));
#49103=CARTESIAN_POINT('Ctrl Pts',(-3.98844946363262,1.,-0.46624852088304));
#49104=CARTESIAN_POINT('Ctrl Pts',(-3.9958644432011,-1.,-0.464388610938975));
#49105=CARTESIAN_POINT('Ctrl Pts',(-3.9958644432011,1.,-0.464388610938975));
#49106=CARTESIAN_POINT('Ctrl Pts',(-4.00327590659075,-1.,-0.462486702616205));
#49107=CARTESIAN_POINT('Ctrl Pts',(-4.00327590659075,1.,-0.462486702616205));
#49108=CARTESIAN_POINT('Ctrl Pts',(-4.01068390573399,-1.,-0.460543280768515));
#49109=CARTESIAN_POINT('Ctrl Pts',(-4.01068390573399,1.,-0.460543280768515));
#49110=CARTESIAN_POINT('Ctrl Pts',(-4.01808900827587,-1.,-0.458558885636945));
#49111=CARTESIAN_POINT('Ctrl Pts',(-4.01808900827587,1.,-0.458558885636945));
#49112=CARTESIAN_POINT('Ctrl Pts',(-4.02549199038394,-1.,-0.456534070784951));
#49113=CARTESIAN_POINT('Ctrl Pts',(-4.02549199038394,1.,-0.456534070784951));
#49114=CARTESIAN_POINT('Ctrl Pts',(-4.03289354362794,-1.,-0.454469363020542));
#49115=CARTESIAN_POINT('Ctrl Pts',(-4.03289354362794,1.,-0.454469363020542));
#49116=CARTESIAN_POINT('Ctrl Pts',(-4.04029392228049,-1.,-0.452365214748892));
#49117=CARTESIAN_POINT('Ctrl Pts',(-4.04029392228049,1.,-0.452365214748892));
#49118=CARTESIAN_POINT('Ctrl Pts',(-4.0476929901813,-1.,-0.450222009543926));
#49119=CARTESIAN_POINT('Ctrl Pts',(-4.0476929901813,1.,-0.450222009543926));
#49120=CARTESIAN_POINT('Ctrl Pts',(-4.0550903779696,-1.,-0.448040082684114));
#49121=CARTESIAN_POINT('Ctrl Pts',(-4.0550903779696,1.,-0.448040082684114));
#49122=CARTESIAN_POINT('Ctrl Pts',(-4.06248560760659,-1.,-0.445819737468538));
#49123=CARTESIAN_POINT('Ctrl Pts',(-4.06248560760659,1.,-0.445819737468538));
#49124=CARTESIAN_POINT('Ctrl Pts',(-4.0698782192569,-1.,-0.443561262395333));
#49125=CARTESIAN_POINT('Ctrl Pts',(-4.0698782192569,1.,-0.443561262395333));
#49126=CARTESIAN_POINT('Ctrl Pts',(-4.07726792490016,-1.,-0.44126495139636));
#49127=CARTESIAN_POINT('Ctrl Pts',(-4.07726792490016,1.,-0.44126495139636));
#49128=CARTESIAN_POINT('Ctrl Pts',(-4.08465462294273,-1.,-0.438931108931279));
#49129=CARTESIAN_POINT('Ctrl Pts',(-4.08465462294273,1.,-0.438931108931279));
#49130=CARTESIAN_POINT('Ctrl Pts',(-4.09203832139089,-1.,-0.436560044913482));
#49131=CARTESIAN_POINT('Ctrl Pts',(-4.09203832139089,1.,-0.436560044913482));
#49132=CARTESIAN_POINT('Ctrl Pts',(-4.09941908688373,-1.,-0.43415207320046));
#49133=CARTESIAN_POINT('Ctrl Pts',(-4.09941908688373,1.,-0.43415207320046));
#49134=CARTESIAN_POINT('Ctrl Pts',(-4.10679698750336,-1.,-0.431707508679884));
#49135=CARTESIAN_POINT('Ctrl Pts',(-4.10679698750336,1.,-0.431707508679884));
#49136=CARTESIAN_POINT('Ctrl Pts',(-4.11417202783267,-1.,-0.429226666075845));
#49137=CARTESIAN_POINT('Ctrl Pts',(-4.11417202783267,1.,-0.429226666075845));
#49138=CARTESIAN_POINT('Ctrl Pts',(-4.12154412502007,-1.,-0.426709855707));
#49139=CARTESIAN_POINT('Ctrl Pts',(-4.12154412502007,1.,-0.426709855707));
#49140=CARTESIAN_POINT('Ctrl Pts',(-4.12891314634572,-1.,-0.424157375323975));
#49141=CARTESIAN_POINT('Ctrl Pts',(-4.12891314634572,1.,-0.424157375323975));
#49142=CARTESIAN_POINT('Ctrl Pts',(-4.13627893207002,-1.,-0.421569503104513));
#49143=CARTESIAN_POINT('Ctrl Pts',(-4.13627893207002,1.,-0.421569503104513));
#49144=CARTESIAN_POINT('Ctrl Pts',(-4.14364132317121,-1.,-0.418946490667703));
#49145=CARTESIAN_POINT('Ctrl Pts',(-4.14364132317121,1.,-0.418946490667703));
#49146=CARTESIAN_POINT('Ctrl Pts',(-4.15100018949965,-1.,-0.416288556008012));
#49147=CARTESIAN_POINT('Ctrl Pts',(-4.15100018949965,1.,-0.416288556008012));
#49148=CARTESIAN_POINT('Ctrl Pts',(-4.15835545017202,-1.,-0.41359587795147));
#49149=CARTESIAN_POINT('Ctrl Pts',(-4.15835545017202,1.,-0.41359587795147));
#49150=CARTESIAN_POINT('Ctrl Pts',(-4.16570705938425,-1.,-0.410868596146414));
#49151=CARTESIAN_POINT('Ctrl Pts',(-4.16570705938425,1.,-0.410868596146414));
#49152=CARTESIAN_POINT('Ctrl Pts',(-4.17158541007977,-1.,-0.408659167568273));
#49153=CARTESIAN_POINT('Ctrl Pts',(-4.17158541007977,1.,-0.408659167568273));
#49154=CARTESIAN_POINT('Ctrl Pts',(-4.17599251954382,-1.,-0.406986596325455));
#49155=CARTESIAN_POINT('Ctrl Pts',(-4.17599251954382,1.,-0.406986596325455));
#49156=CARTESIAN_POINT('Ctrl Pts',(-4.17892985789466,-1.,-0.40586466267921));
#49157=CARTESIAN_POINT('Ctrl Pts',(-4.17892985789466,1.,-0.40586466267921));
#49158=CARTESIAN_POINT('Ctrl Pts',(-4.18039834341342,-1.,-0.40530197431835));
#49159=CARTESIAN_POINT('Ctrl Pts',(-4.18039834341342,1.,-0.40530197431835));
#49160=CARTESIAN_POINT('',(-3.71701050416825,1.,-0.496319364827592));
#49161=CARTESIAN_POINT('Ctrl Pts',(-3.71701050416825,-1.,-0.496319364827592));
#49162=CARTESIAN_POINT('Ctrl Pts',(-3.71701050416825,-0.666666666666667,
-0.496319364827592));
#49163=CARTESIAN_POINT('Ctrl Pts',(-3.71701050416825,-0.333333333333333,
-0.496319364827592));
#49164=CARTESIAN_POINT('Ctrl Pts',(-3.71701050416825,0.333333333333333,
-0.496319364827592));
#49165=CARTESIAN_POINT('Ctrl Pts',(-3.71701050416825,0.666666666666667,
-0.496319364827592));
#49166=CARTESIAN_POINT('Ctrl Pts',(-3.71701050416825,1.,-0.496319364827592));
#49167=CARTESIAN_POINT('',(-4.18039834341342,1.,-0.40530197431835));
#49168=CARTESIAN_POINT('',(-4.18039834341342,0.,-0.40530197431835));
#49169=CARTESIAN_POINT('Ctrl Pts',(-3.71701050416825,1.,-0.496319364827592));
#49170=CARTESIAN_POINT('Ctrl Pts',(-3.71704500630495,1.,-0.496354087924312));
#49171=CARTESIAN_POINT('Ctrl Pts',(-3.71721917030355,1.,-0.496446644158005));
#49172=CARTESIAN_POINT('Ctrl Pts',(-3.71785517607549,1.,-0.496605651525989));
#49173=CARTESIAN_POINT('Ctrl Pts',(-3.71952320822499,1.,-0.496846224822563));
#49174=CARTESIAN_POINT('Ctrl Pts',(-3.72301489774398,1.,-0.497187079575988));
#49175=CARTESIAN_POINT('Ctrl Pts',(-3.72830430904606,1.,-0.497584067153049));
#49176=CARTESIAN_POINT('Ctrl Pts',(-3.73486914372449,1.,-0.497984209510024));
#49177=CARTESIAN_POINT('Ctrl Pts',(-3.74235701734714,1.,-0.498350586057692));
#49178=CARTESIAN_POINT('Ctrl Pts',(-3.75037362167839,1.,-0.498642802042606));
#49179=CARTESIAN_POINT('Ctrl Pts',(-3.75854082221053,1.,-0.498823681615422));
#49180=CARTESIAN_POINT('Ctrl Pts',(-3.76655401191229,1.,-0.49886579233529));
#49181=CARTESIAN_POINT('Ctrl Pts',(-3.77425499225255,1.,-0.498759900365892));
#49182=CARTESIAN_POINT('Ctrl Pts',(-3.78163975337356,1.,-0.498515471679585));
#49183=CARTESIAN_POINT('Ctrl Pts',(-3.78879701661264,1.,-0.498152751800958));
#49184=CARTESIAN_POINT('Ctrl Pts',(-3.79586380669994,1.,-0.497696892100625));
#49185=CARTESIAN_POINT('Ctrl Pts',(-3.80297788298514,1.,-0.497171756201052));
#49186=CARTESIAN_POINT('Ctrl Pts',(-3.81022254090839,1.,-0.496592643443704));
#49187=CARTESIAN_POINT('Ctrl Pts',(-3.81760756144025,1.,-0.49596393787548));
#49188=CARTESIAN_POINT('Ctrl Pts',(-3.82509963594103,1.,-0.495283458893837));
#49189=CARTESIAN_POINT('Ctrl Pts',(-3.83264092682431,1.,-0.494545212256401));
#49190=CARTESIAN_POINT('Ctrl Pts',(-3.84017095578451,1.,-0.493742574629134));
#49191=CARTESIAN_POINT('Ctrl Pts',(-3.84765051147999,1.,-0.492871792414141));
#49192=CARTESIAN_POINT('Ctrl Pts',(-3.85507287020263,1.,-0.491933631083813));
#49193=CARTESIAN_POINT('Ctrl Pts',(-3.86245057319246,1.,-0.490931482170891));
#49194=CARTESIAN_POINT('Ctrl Pts',(-3.86980755613707,1.,-0.489870245704918));
#49195=CARTESIAN_POINT('Ctrl Pts',(-3.87716963231109,1.,-0.488754973798274));
#49196=CARTESIAN_POINT('Ctrl Pts',(-3.88455453328138,1.,-0.487589452275154));
#49197=CARTESIAN_POINT('Ctrl Pts',(-3.89196582437552,1.,-0.486375337854103));
#49198=CARTESIAN_POINT('Ctrl Pts',(-3.89939844658513,1.,-0.485112963522222));
#49199=CARTESIAN_POINT('Ctrl Pts',(-3.90684210358056,1.,-0.48380183508915));
#49200=CARTESIAN_POINT('Ctrl Pts',(-3.91428536373751,1.,-0.482441230340713));
#49201=CARTESIAN_POINT('Ctrl Pts',(-3.92171976072341,1.,-0.481030798910748));
#49202=CARTESIAN_POINT('Ctrl Pts',(-3.92914297392071,1.,-0.479571028525579));
#49203=CARTESIAN_POINT('Ctrl Pts',(-3.93655660689819,1.,-0.478062927140964));
#49204=CARTESIAN_POINT('Ctrl Pts',(-3.94396469119383,1.,-0.476507810658537));
#49205=CARTESIAN_POINT('Ctrl Pts',(-3.95137192932897,1.,-0.47490705302179));
#49206=CARTESIAN_POINT('Ctrl Pts',(-3.95878201038338,1.,-0.473261847236297));
#49207=CARTESIAN_POINT('Ctrl Pts',(-3.96619600864643,1.,-0.471572978413503));
#49208=CARTESIAN_POINT('Ctrl Pts',(-3.97361320212436,1.,-0.469840942829895));
#49209=CARTESIAN_POINT('Ctrl Pts',(-3.98103175589371,1.,-0.468066047920157));
#49210=CARTESIAN_POINT('Ctrl Pts',(-3.98844946363262,1.,-0.46624852088304));
#49211=CARTESIAN_POINT('Ctrl Pts',(-3.9958644432011,1.,-0.464388610938975));
#49212=CARTESIAN_POINT('Ctrl Pts',(-4.00327590659075,1.,-0.462486702616205));
#49213=CARTESIAN_POINT('Ctrl Pts',(-4.01068390573399,1.,-0.460543280768515));
#49214=CARTESIAN_POINT('Ctrl Pts',(-4.01808900827587,1.,-0.458558885636945));
#49215=CARTESIAN_POINT('Ctrl Pts',(-4.02549199038394,1.,-0.456534070784951));
#49216=CARTESIAN_POINT('Ctrl Pts',(-4.03289354362794,1.,-0.454469363020542));
#49217=CARTESIAN_POINT('Ctrl Pts',(-4.04029392228049,1.,-0.452365214748892));
#49218=CARTESIAN_POINT('Ctrl Pts',(-4.0476929901813,1.,-0.450222009543926));
#49219=CARTESIAN_POINT('Ctrl Pts',(-4.0550903779696,1.,-0.448040082684114));
#49220=CARTESIAN_POINT('Ctrl Pts',(-4.06248560760659,1.,-0.445819737468538));
#49221=CARTESIAN_POINT('Ctrl Pts',(-4.0698782192569,1.,-0.443561262395333));
#49222=CARTESIAN_POINT('Ctrl Pts',(-4.07726792490016,1.,-0.44126495139636));
#49223=CARTESIAN_POINT('Ctrl Pts',(-4.08465462294273,1.,-0.438931108931279));
#49224=CARTESIAN_POINT('Ctrl Pts',(-4.09203832139089,1.,-0.436560044913482));
#49225=CARTESIAN_POINT('Ctrl Pts',(-4.09941908688373,1.,-0.43415207320046));
#49226=CARTESIAN_POINT('Ctrl Pts',(-4.10679698750336,1.,-0.431707508679884));
#49227=CARTESIAN_POINT('Ctrl Pts',(-4.11417202783267,1.,-0.429226666075845));
#49228=CARTESIAN_POINT('Ctrl Pts',(-4.12154412502007,1.,-0.426709855707));
#49229=CARTESIAN_POINT('Ctrl Pts',(-4.12891314634572,1.,-0.424157375323975));
#49230=CARTESIAN_POINT('Ctrl Pts',(-4.13627893207002,1.,-0.421569503104513));
#49231=CARTESIAN_POINT('Ctrl Pts',(-4.14364132317121,1.,-0.418946490667703));
#49232=CARTESIAN_POINT('Ctrl Pts',(-4.15100018949965,1.,-0.416288556008012));
#49233=CARTESIAN_POINT('Ctrl Pts',(-4.15835545017202,1.,-0.41359587795147));
#49234=CARTESIAN_POINT('Ctrl Pts',(-4.16570705938425,1.,-0.410868596146414));
#49235=CARTESIAN_POINT('Ctrl Pts',(-4.17158541007977,1.,-0.408659167568273));
#49236=CARTESIAN_POINT('Ctrl Pts',(-4.17599251954382,1.,-0.406986596325455));
#49237=CARTESIAN_POINT('Ctrl Pts',(-4.17892985789466,1.,-0.40586466267921));
#49238=CARTESIAN_POINT('Ctrl Pts',(-4.18039834341342,1.,-0.40530197431835));
#49239=CARTESIAN_POINT('Origin',(-4.18039834341342,0.,-0.40530197431835));
#49240=CARTESIAN_POINT('',(-4.1923339003649,1.,-0.253646344052522));
#49241=CARTESIAN_POINT('Origin',(0.,0.,0.));
#49242=CARTESIAN_POINT('',(-3.68845817949618,1.,-0.67659164797366));
#49243=CARTESIAN_POINT('Origin',(0.,1.,0.));
#49244=CARTESIAN_POINT('Ctrl Pts',(-3.68845817949618,1.,-0.676591647973661));
#49245=CARTESIAN_POINT('Ctrl Pts',(-3.68845817949618,0.666666666666667,
-0.676591647973661));
#49246=CARTESIAN_POINT('Ctrl Pts',(-3.68845817949618,0.333333333333333,
-0.676591647973661));
#49247=CARTESIAN_POINT('Ctrl Pts',(-3.68845817949618,-0.333333333333333,
-0.676591647973661));
#49248=CARTESIAN_POINT('Ctrl Pts',(-3.68845817949618,-0.666666666666667,
-0.676591647973661));
#49249=CARTESIAN_POINT('Ctrl Pts',(-3.68845817949618,-1.,-0.676591647973661));
#49250=CARTESIAN_POINT('Ctrl Pts',(-4.10104028313088,-1.,-0.906349047628866));
#49251=CARTESIAN_POINT('Ctrl Pts',(-4.10104028313088,1.,-0.906349047628866));
#49252=CARTESIAN_POINT('Ctrl Pts',(-4.09981755067956,-1.,-0.905360112216302));
#49253=CARTESIAN_POINT('Ctrl Pts',(-4.09981755067956,1.,-0.905360112216302));
#49254=CARTESIAN_POINT('Ctrl Pts',(-4.09737067247114,-1.,-0.903385402444212));
#49255=CARTESIAN_POINT('Ctrl Pts',(-4.09737067247114,1.,-0.903385402444212));
#49256=CARTESIAN_POINT('Ctrl Pts',(-4.09369611524319,-1.,-0.900432820945975));
#49257=CARTESIAN_POINT('Ctrl Pts',(-4.09369611524319,1.,-0.900432820945975));
#49258=CARTESIAN_POINT('Ctrl Pts',(-4.08878822249095,-1.,-0.896515019236368));
#49259=CARTESIAN_POINT('Ctrl Pts',(-4.08878822249095,1.,-0.896515019236368));
#49260=CARTESIAN_POINT('Ctrl Pts',(-4.08263920306651,-1.,-0.891649447920401));
#49261=CARTESIAN_POINT('Ctrl Pts',(-4.08263920306651,1.,-0.891649447920401));
#49262=CARTESIAN_POINT('Ctrl Pts',(-4.07647601774639,-1.,-0.886815658360739));
#49263=CARTESIAN_POINT('Ctrl Pts',(-4.07647601774639,1.,-0.886815658360739));
#49264=CARTESIAN_POINT('Ctrl Pts',(-4.07029866694292,-1.,-0.882013797525916));
#49265=CARTESIAN_POINT('Ctrl Pts',(-4.07029866694292,1.,-0.882013797525916));
#49266=CARTESIAN_POINT('Ctrl Pts',(-4.06410717232347,-1.,-0.877244060484595));
#49267=CARTESIAN_POINT('Ctrl Pts',(-4.06410717232347,1.,-0.877244060484595));
#49268=CARTESIAN_POINT('Ctrl Pts',(-4.05790159030495,-1.,-0.872506694780563));
#49269=CARTESIAN_POINT('Ctrl Pts',(-4.05790159030495,1.,-0.872506694780563));
#49270=CARTESIAN_POINT('Ctrl Pts',(-4.05168199437128,-1.,-0.867801988858176));
#49271=CARTESIAN_POINT('Ctrl Pts',(-4.05168199437128,1.,-0.867801988858176));
#49272=CARTESIAN_POINT('Ctrl Pts',(-4.04544845048097,-1.,-0.863130256642173));
#49273=CARTESIAN_POINT('Ctrl Pts',(-4.04544845048097,1.,-0.863130256642173));
#49274=CARTESIAN_POINT('Ctrl Pts',(-4.03920099284658,-1.,-0.858491822322571));
#49275=CARTESIAN_POINT('Ctrl Pts',(-4.03920099284658,1.,-0.858491822322571));
#49276=CARTESIAN_POINT('Ctrl Pts',(-4.03293960436945,-1.,-0.853887006632178));
#49277=CARTESIAN_POINT('Ctrl Pts',(-4.03293960436945,1.,-0.853887006632178));
#49278=CARTESIAN_POINT('Ctrl Pts',(-4.02666418343508,-1.,-0.849316107475012));
#49279=CARTESIAN_POINT('Ctrl Pts',(-4.02666418343508,1.,-0.849316107475012));
#49280=CARTESIAN_POINT('Ctrl Pts',(-4.02037456798787,-1.,-0.844779403288517));
#49281=CARTESIAN_POINT('Ctrl Pts',(-4.02037456798787,1.,-0.844779403288517));
#49282=CARTESIAN_POINT('Ctrl Pts',(-4.01407059766338,-1.,-0.84027717197638));
#49283=CARTESIAN_POINT('Ctrl Pts',(-4.01407059766338,1.,-0.84027717197638));
#49284=CARTESIAN_POINT('Ctrl Pts',(-4.00775216907934,-1.,-0.835809705809821));
#49285=CARTESIAN_POINT('Ctrl Pts',(-4.00775216907934,1.,-0.835809705809821));
#49286=CARTESIAN_POINT('Ctrl Pts',(-4.00141928477447,-1.,-0.831377325741487));
#49287=CARTESIAN_POINT('Ctrl Pts',(-4.00141928477447,1.,-0.831377325741487));
#49288=CARTESIAN_POINT('Ctrl Pts',(-3.99507212784289,-1.,-0.826980400320473));
#49289=CARTESIAN_POINT('Ctrl Pts',(-3.99507212784289,1.,-0.826980400320473));
#49290=CARTESIAN_POINT('Ctrl Pts',(-3.98871104646328,-1.,-0.822619346021769));
#49291=CARTESIAN_POINT('Ctrl Pts',(-3.98871104646328,1.,-0.822619346021769));
#49292=CARTESIAN_POINT('Ctrl Pts',(-3.98233640155287,-1.,-0.818294599022033));
#49293=CARTESIAN_POINT('Ctrl Pts',(-3.98233640155287,1.,-0.818294599022033));
#49294=CARTESIAN_POINT('Ctrl Pts',(-3.97594844078763,-1.,-0.814006592328737));
#49295=CARTESIAN_POINT('Ctrl Pts',(-3.97594844078763,1.,-0.814006592328737));
#49296=CARTESIAN_POINT('Ctrl Pts',(-3.96954717513251,-1.,-0.809755732818134));
#49297=CARTESIAN_POINT('Ctrl Pts',(-3.96954717513251,1.,-0.809755732818134));
#49298=CARTESIAN_POINT('Ctrl Pts',(-3.96313222295874,-1.,-0.805542372178496));
#49299=CARTESIAN_POINT('Ctrl Pts',(-3.96313222295874,1.,-0.805542372178496));
#49300=CARTESIAN_POINT('Ctrl Pts',(-3.95670276375176,-1.,-0.801366797727206));
#49301=CARTESIAN_POINT('Ctrl Pts',(-3.95670276375176,1.,-0.801366797727206));
#49302=CARTESIAN_POINT('Ctrl Pts',(-3.95025788827189,-1.,-0.797229296085438));
#49303=CARTESIAN_POINT('Ctrl Pts',(-3.95025788827189,1.,-0.797229296085438));
#49304=CARTESIAN_POINT('Ctrl Pts',(-3.94379688971307,-1.,-0.793130205641017));
#49305=CARTESIAN_POINT('Ctrl Pts',(-3.94379688971307,1.,-0.793130205641017));
#49306=CARTESIAN_POINT('Ctrl Pts',(-3.93731956885671,-1.,-0.789069971469323));
#49307=CARTESIAN_POINT('Ctrl Pts',(-3.93731956885671,1.,-0.789069971469323));
#49308=CARTESIAN_POINT('Ctrl Pts',(-3.93082655631768,-1.,-0.785049202786458));
#49309=CARTESIAN_POINT('Ctrl Pts',(-3.93082655631768,1.,-0.785049202786458));
#49310=CARTESIAN_POINT('Ctrl Pts',(-3.92431956510418,-1.,-0.781068718228395));
#49311=CARTESIAN_POINT('Ctrl Pts',(-3.92431956510418,1.,-0.781068718228395));
#49312=CARTESIAN_POINT('Ctrl Pts',(-3.91780062334464,-1.,-0.777129415664915));
#49313=CARTESIAN_POINT('Ctrl Pts',(-3.91780062334464,1.,-0.777129415664915));
#49314=CARTESIAN_POINT('Ctrl Pts',(-3.91127138115238,-1.,-0.773232154506305));
#49315=CARTESIAN_POINT('Ctrl Pts',(-3.91127138115238,1.,-0.773232154506305));
#49316=CARTESIAN_POINT('Ctrl Pts',(-3.90473237182634,-1.,-0.769377629847876));
#49317=CARTESIAN_POINT('Ctrl Pts',(-3.90473237182634,1.,-0.769377629847876));
#49318=CARTESIAN_POINT('Ctrl Pts',(-3.89818233104381,-1.,-0.765566256401306));
#49319=CARTESIAN_POINT('Ctrl Pts',(-3.89818233104381,1.,-0.765566256401306));
#49320=CARTESIAN_POINT('Ctrl Pts',(-3.89161738162245,-1.,-0.761798028793978));
#49321=CARTESIAN_POINT('Ctrl Pts',(-3.89161738162245,1.,-0.761798028793978));
#49322=CARTESIAN_POINT('Ctrl Pts',(-3.88503262662684,-1.,-0.758072800564798));
#49323=CARTESIAN_POINT('Ctrl Pts',(-3.88503262662684,1.,-0.758072800564798));
#49324=CARTESIAN_POINT('Ctrl Pts',(-3.87842382520058,-1.,-0.754390577396846));
#49325=CARTESIAN_POINT('Ctrl Pts',(-3.87842382520058,1.,-0.754390577396846));
#49326=CARTESIAN_POINT('Ctrl Pts',(-3.87178914078372,-1.,-0.750751822383023));
#49327=CARTESIAN_POINT('Ctrl Pts',(-3.87178914078372,1.,-0.750751822383023));
#49328=CARTESIAN_POINT('Ctrl Pts',(-3.86513062969896,-1.,-0.747157716488884));
#49329=CARTESIAN_POINT('Ctrl Pts',(-3.86513062969896,1.,-0.747157716488884));
#49330=CARTESIAN_POINT('Ctrl Pts',(-3.85845645217611,-1.,-0.743610542737042));
#49331=CARTESIAN_POINT('Ctrl Pts',(-3.85845645217611,1.,-0.743610542737042));
#49332=CARTESIAN_POINT('Ctrl Pts',(-3.85177770351237,-1.,-0.740113146827176));
#49333=CARTESIAN_POINT('Ctrl Pts',(-3.85177770351237,1.,-0.740113146827176));
#49334=CARTESIAN_POINT('Ctrl Pts',(-3.84510432881231,-1.,-0.736668240497151));
#49335=CARTESIAN_POINT('Ctrl Pts',(-3.84510432881231,1.,-0.736668240497151));
#49336=CARTESIAN_POINT('Ctrl Pts',(-3.83844103658016,-1.,-0.73327770375609));
#49337=CARTESIAN_POINT('Ctrl Pts',(-3.83844103658016,1.,-0.73327770375609));
#49338=CARTESIAN_POINT('Ctrl Pts',(-3.8317839240337,-1.,-0.729942010490145));
#49339=CARTESIAN_POINT('Ctrl Pts',(-3.8317839240337,1.,-0.729942010490145));
#49340=CARTESIAN_POINT('Ctrl Pts',(-3.82511495756682,-1.,-0.726659281876608));
#49341=CARTESIAN_POINT('Ctrl Pts',(-3.82511495756682,1.,-0.726659281876608));
#49342=CARTESIAN_POINT('Ctrl Pts',(-3.81840802610795,-1.,-0.723426346019349));
#49343=CARTESIAN_POINT('Ctrl Pts',(-3.81840802610795,1.,-0.723426346019349));
#49344=CARTESIAN_POINT('Ctrl Pts',(-3.81163885127309,-1.,-0.720240466589172));
#49345=CARTESIAN_POINT('Ctrl Pts',(-3.81163885127309,1.,-0.720240466589172));
#49346=CARTESIAN_POINT('Ctrl Pts',(-3.80479445759296,-1.,-0.717100993669091));
#49347=CARTESIAN_POINT('Ctrl Pts',(-3.80479445759296,1.,-0.717100993669091));
#49348=CARTESIAN_POINT('Ctrl Pts',(-3.79788100314994,-1.,-0.714010733006677));
#49349=CARTESIAN_POINT('Ctrl Pts',(-3.79788100314994,1.,-0.714010733006677));
#49350=CARTESIAN_POINT('Ctrl Pts',(-3.79093694007146,-1.,-0.710978231689117));
#49351=CARTESIAN_POINT('Ctrl Pts',(-3.79093694007146,1.,-0.710978231689117));
#49352=CARTESIAN_POINT('Ctrl Pts',(-3.78402183336678,-1.,-0.7080158793756));
#49353=CARTESIAN_POINT('Ctrl Pts',(-3.78402183336678,1.,-0.7080158793756));
#49354=CARTESIAN_POINT('Ctrl Pts',(-3.77719254217197,-1.,-0.705135847999949));
#49355=CARTESIAN_POINT('Ctrl Pts',(-3.77719254217197,1.,-0.705135847999949));
#49356=CARTESIAN_POINT('Ctrl Pts',(-3.77048141872904,-1.,-0.702346356621613));
#49357=CARTESIAN_POINT('Ctrl Pts',(-3.77048141872904,1.,-0.702346356621613));
#49358=CARTESIAN_POINT('Ctrl Pts',(-3.76387780603725,-1.,-0.699648552230851));
#49359=CARTESIAN_POINT('Ctrl Pts',(-3.76387780603725,1.,-0.699648552230851));
#49360=CARTESIAN_POINT('Ctrl Pts',(-3.75729775766913,-1.,-0.69703124565953));
#49361=CARTESIAN_POINT('Ctrl Pts',(-3.75729775766913,1.,-0.69703124565953));
#49362=CARTESIAN_POINT('Ctrl Pts',(-3.7506028824329,-1.,-0.694474562581173));
#49363=CARTESIAN_POINT('Ctrl Pts',(-3.7506028824329,1.,-0.694474562581173));
#49364=CARTESIAN_POINT('Ctrl Pts',(-3.74365508986548,-1.,-0.691960080400503));
#49365=CARTESIAN_POINT('Ctrl Pts',(-3.74365508986548,1.,-0.691960080400503));
#49366=CARTESIAN_POINT('Ctrl Pts',(-3.73636374474993,-1.,-0.689479637354651));
#49367=CARTESIAN_POINT('Ctrl Pts',(-3.73636374474993,1.,-0.689479637354651));
#49368=CARTESIAN_POINT('Ctrl Pts',(-3.72872973554125,-1.,-0.687043475232499));
#49369=CARTESIAN_POINT('Ctrl Pts',(-3.72872973554125,1.,-0.687043475232499));
#49370=CARTESIAN_POINT('Ctrl Pts',(-3.7209063713952,-1.,-0.684691698168355));
#49371=CARTESIAN_POINT('Ctrl Pts',(-3.7209063713952,1.,-0.684691698168355));
#49372=CARTESIAN_POINT('Ctrl Pts',(-3.71319182790334,-1.,-0.682492345109689));
#49373=CARTESIAN_POINT('Ctrl Pts',(-3.71319182790334,1.,-0.682492345109689));
#49374=CARTESIAN_POINT('Ctrl Pts',(-3.70595722032165,-1.,-0.680526909711617));
#49375=CARTESIAN_POINT('Ctrl Pts',(-3.70595722032165,1.,-0.680526909711617));
#49376=CARTESIAN_POINT('Ctrl Pts',(-3.69959004073192,-1.,-0.678878822226389));
#49377=CARTESIAN_POINT('Ctrl Pts',(-3.69959004073192,1.,-0.678878822226389));
#49378=CARTESIAN_POINT('Ctrl Pts',(-3.69443683573443,-1.,-0.677621861865196));
#49379=CARTESIAN_POINT('Ctrl Pts',(-3.69443683573443,1.,-0.677621861865196));
#49380=CARTESIAN_POINT('Ctrl Pts',(-3.69073278191505,-1.,-0.67680581107414));
#49381=CARTESIAN_POINT('Ctrl Pts',(-3.69073278191505,1.,-0.67680581107414));
#49382=CARTESIAN_POINT('Ctrl Pts',(-3.68901718135636,-1.,-0.676524321060167));
#49383=CARTESIAN_POINT('Ctrl Pts',(-3.68901718135636,1.,-0.676524321060167));
#49384=CARTESIAN_POINT('Ctrl Pts',(-3.68844918120934,-1.,-0.676525601650139));
#49385=CARTESIAN_POINT('Ctrl Pts',(-3.68844918120934,1.,-0.676525601650139));
#49386=CARTESIAN_POINT('Ctrl Pts',(-3.68838970675356,-1.,-0.676620796001716));
#49387=CARTESIAN_POINT('Ctrl Pts',(-3.68838970675356,1.,-0.676620796001716));
#49388=CARTESIAN_POINT('Ctrl Pts',(-3.68843977377012,-1.,-0.676691979611562));
#49389=CARTESIAN_POINT('Ctrl Pts',(-3.68843977377012,1.,-0.676691979611562));
#49390=CARTESIAN_POINT('',(-4.10104028313088,1.,-0.906349047628866));
#49391=CARTESIAN_POINT('Ctrl Pts',(-4.10104028313088,1.,-0.906349047628866));
#49392=CARTESIAN_POINT('Ctrl Pts',(-4.09981755067956,1.,-0.905360112216302));
#49393=CARTESIAN_POINT('Ctrl Pts',(-4.09737067247114,1.,-0.903385402444212));
#49394=CARTESIAN_POINT('Ctrl Pts',(-4.09369611524319,1.,-0.900432820945975));
#49395=CARTESIAN_POINT('Ctrl Pts',(-4.08878822249095,1.,-0.896515019236368));
#49396=CARTESIAN_POINT('Ctrl Pts',(-4.08263920306651,1.,-0.891649447920401));
#49397=CARTESIAN_POINT('Ctrl Pts',(-4.07647601774639,1.,-0.886815658360739));
#49398=CARTESIAN_POINT('Ctrl Pts',(-4.07029866694292,1.,-0.882013797525916));
#49399=CARTESIAN_POINT('Ctrl Pts',(-4.06410717232347,1.,-0.877244060484595));
#49400=CARTESIAN_POINT('Ctrl Pts',(-4.05790159030495,1.,-0.872506694780563));
#49401=CARTESIAN_POINT('Ctrl Pts',(-4.05168199437128,1.,-0.867801988858176));
#49402=CARTESIAN_POINT('Ctrl Pts',(-4.04544845048097,1.,-0.863130256642173));
#49403=CARTESIAN_POINT('Ctrl Pts',(-4.03920099284658,1.,-0.858491822322571));
#49404=CARTESIAN_POINT('Ctrl Pts',(-4.03293960436945,1.,-0.853887006632178));
#49405=CARTESIAN_POINT('Ctrl Pts',(-4.02666418343508,1.,-0.849316107475012));
#49406=CARTESIAN_POINT('Ctrl Pts',(-4.02037456798787,1.,-0.844779403288517));
#49407=CARTESIAN_POINT('Ctrl Pts',(-4.01407059766338,1.,-0.84027717197638));
#49408=CARTESIAN_POINT('Ctrl Pts',(-4.00775216907934,1.,-0.835809705809821));
#49409=CARTESIAN_POINT('Ctrl Pts',(-4.00141928477447,1.,-0.831377325741487));
#49410=CARTESIAN_POINT('Ctrl Pts',(-3.99507212784289,1.,-0.826980400320473));
#49411=CARTESIAN_POINT('Ctrl Pts',(-3.98871104646328,1.,-0.822619346021769));
#49412=CARTESIAN_POINT('Ctrl Pts',(-3.98233640155287,1.,-0.818294599022033));
#49413=CARTESIAN_POINT('Ctrl Pts',(-3.97594844078763,1.,-0.814006592328737));
#49414=CARTESIAN_POINT('Ctrl Pts',(-3.96954717513251,1.,-0.809755732818134));
#49415=CARTESIAN_POINT('Ctrl Pts',(-3.96313222295874,1.,-0.805542372178496));
#49416=CARTESIAN_POINT('Ctrl Pts',(-3.95670276375176,1.,-0.801366797727206));
#49417=CARTESIAN_POINT('Ctrl Pts',(-3.95025788827189,1.,-0.797229296085438));
#49418=CARTESIAN_POINT('Ctrl Pts',(-3.94379688971307,1.,-0.793130205641017));
#49419=CARTESIAN_POINT('Ctrl Pts',(-3.93731956885671,1.,-0.789069971469323));
#49420=CARTESIAN_POINT('Ctrl Pts',(-3.93082655631768,1.,-0.785049202786458));
#49421=CARTESIAN_POINT('Ctrl Pts',(-3.92431956510418,1.,-0.781068718228395));
#49422=CARTESIAN_POINT('Ctrl Pts',(-3.91780062334464,1.,-0.777129415664915));
#49423=CARTESIAN_POINT('Ctrl Pts',(-3.91127138115238,1.,-0.773232154506305));
#49424=CARTESIAN_POINT('Ctrl Pts',(-3.90473237182634,1.,-0.769377629847876));
#49425=CARTESIAN_POINT('Ctrl Pts',(-3.89818233104381,1.,-0.765566256401306));
#49426=CARTESIAN_POINT('Ctrl Pts',(-3.89161738162245,1.,-0.761798028793978));
#49427=CARTESIAN_POINT('Ctrl Pts',(-3.88503262662684,1.,-0.758072800564798));
#49428=CARTESIAN_POINT('Ctrl Pts',(-3.87842382520058,1.,-0.754390577396846));
#49429=CARTESIAN_POINT('Ctrl Pts',(-3.87178914078372,1.,-0.750751822383023));
#49430=CARTESIAN_POINT('Ctrl Pts',(-3.86513062969896,1.,-0.747157716488884));
#49431=CARTESIAN_POINT('Ctrl Pts',(-3.85845645217611,1.,-0.743610542737042));
#49432=CARTESIAN_POINT('Ctrl Pts',(-3.85177770351237,1.,-0.740113146827176));
#49433=CARTESIAN_POINT('Ctrl Pts',(-3.84510432881231,1.,-0.736668240497151));
#49434=CARTESIAN_POINT('Ctrl Pts',(-3.83844103658016,1.,-0.73327770375609));
#49435=CARTESIAN_POINT('Ctrl Pts',(-3.8317839240337,1.,-0.729942010490145));
#49436=CARTESIAN_POINT('Ctrl Pts',(-3.82511495756682,1.,-0.726659281876608));
#49437=CARTESIAN_POINT('Ctrl Pts',(-3.81840802610795,1.,-0.723426346019349));
#49438=CARTESIAN_POINT('Ctrl Pts',(-3.81163885127309,1.,-0.720240466589172));
#49439=CARTESIAN_POINT('Ctrl Pts',(-3.80479445759296,1.,-0.717100993669091));
#49440=CARTESIAN_POINT('Ctrl Pts',(-3.79788100314994,1.,-0.714010733006677));
#49441=CARTESIAN_POINT('Ctrl Pts',(-3.79093694007146,1.,-0.710978231689117));
#49442=CARTESIAN_POINT('Ctrl Pts',(-3.78402183336678,1.,-0.7080158793756));
#49443=CARTESIAN_POINT('Ctrl Pts',(-3.77719254217197,1.,-0.705135847999949));
#49444=CARTESIAN_POINT('Ctrl Pts',(-3.77048141872904,1.,-0.702346356621613));
#49445=CARTESIAN_POINT('Ctrl Pts',(-3.76387780603725,1.,-0.699648552230851));
#49446=CARTESIAN_POINT('Ctrl Pts',(-3.75729775766913,1.,-0.69703124565953));
#49447=CARTESIAN_POINT('Ctrl Pts',(-3.7506028824329,1.,-0.694474562581173));
#49448=CARTESIAN_POINT('Ctrl Pts',(-3.74365508986548,1.,-0.691960080400503));
#49449=CARTESIAN_POINT('Ctrl Pts',(-3.73636374474993,1.,-0.689479637354651));
#49450=CARTESIAN_POINT('Ctrl Pts',(-3.72872973554125,1.,-0.687043475232499));
#49451=CARTESIAN_POINT('Ctrl Pts',(-3.7209063713952,1.,-0.684691698168355));
#49452=CARTESIAN_POINT('Ctrl Pts',(-3.71319182790334,1.,-0.682492345109689));
#49453=CARTESIAN_POINT('Ctrl Pts',(-3.70595722032165,1.,-0.680526909711617));
#49454=CARTESIAN_POINT('Ctrl Pts',(-3.69959004073192,1.,-0.678878822226389));
#49455=CARTESIAN_POINT('Ctrl Pts',(-3.69443683573443,1.,-0.677621861865196));
#49456=CARTESIAN_POINT('Ctrl Pts',(-3.6910107117555,1.,-0.676867042599711));
#49457=CARTESIAN_POINT('Ctrl Pts',(-3.68934997767391,1.,-0.676580391119535));
#49458=CARTESIAN_POINT('Ctrl Pts',(-3.68869596426099,1.,-0.676535079520365));
#49459=CARTESIAN_POINT('Ctrl Pts',(-3.68850172300543,1.,-0.67656928609342));
#49460=CARTESIAN_POINT('Ctrl Pts',(-3.68845817949618,1.,-0.676591647973661));
#49461=CARTESIAN_POINT('',(-4.10104028313088,0.,-0.906349047628866));
#49462=CARTESIAN_POINT('Ctrl Pts',(-3.59363563249864,-1.,-1.07157964745328));
#49463=CARTESIAN_POINT('Ctrl Pts',(-3.59363563249864,1.,-1.07157964745328));
#49464=CARTESIAN_POINT('Ctrl Pts',(-3.59355870577901,-1.,-1.07162034256459));
#49465=CARTESIAN_POINT('Ctrl Pts',(-3.59355870577901,1.,-1.07162034256459));
#49466=CARTESIAN_POINT('Ctrl Pts',(-3.59356848057812,-1.,-1.07173216219145));
#49467=CARTESIAN_POINT('Ctrl Pts',(-3.59356848057812,1.,-1.07173216219145));
#49468=CARTESIAN_POINT('Ctrl Pts',(-3.5940739910409,-1.,-1.07199116987656));
#49469=CARTESIAN_POINT('Ctrl Pts',(-3.5940739910409,1.,-1.07199116987656));
#49470=CARTESIAN_POINT('Ctrl Pts',(-3.59573039612316,-1.,-1.07251922679245));
#49471=CARTESIAN_POINT('Ctrl Pts',(-3.59573039612316,1.,-1.07251922679245));
#49472=CARTESIAN_POINT('Ctrl Pts',(-3.59940121154535,-1.,-1.07347372545714));
#49473=CARTESIAN_POINT('Ctrl Pts',(-3.59940121154535,1.,-1.07347372545714));
#49474=CARTESIAN_POINT('Ctrl Pts',(-3.60456339887778,-1.,-1.07469327168578));
#49475=CARTESIAN_POINT('Ctrl Pts',(-3.60456339887778,1.,-1.07469327168578));
#49476=CARTESIAN_POINT('Ctrl Pts',(-3.61098481349204,-1.,-1.07611545402734));
#49477=CARTESIAN_POINT('Ctrl Pts',(-3.61098481349204,1.,-1.07611545402734));
#49478=CARTESIAN_POINT('Ctrl Pts',(-3.61832318504574,-1.,-1.07764868137619));
#49479=CARTESIAN_POINT('Ctrl Pts',(-3.61832318504574,1.,-1.07764868137619));
#49480=CARTESIAN_POINT('Ctrl Pts',(-3.62619537902361,-1.,-1.07919137290742));
#49481=CARTESIAN_POINT('Ctrl Pts',(-3.62619537902361,1.,-1.07919137290742));
#49482=CARTESIAN_POINT('Ctrl Pts',(-3.63423373196529,-1.,-1.08064765719867));
#49483=CARTESIAN_POINT('Ctrl Pts',(-3.63423373196529,1.,-1.08064765719867));
#49484=CARTESIAN_POINT('Ctrl Pts',(-3.64214167843677,-1.,-1.08194278850996));
#49485=CARTESIAN_POINT('Ctrl Pts',(-3.64214167843677,1.,-1.08194278850996));
#49486=CARTESIAN_POINT('Ctrl Pts',(-3.64976441208358,-1.,-1.08304289898623));
#49487=CARTESIAN_POINT('Ctrl Pts',(-3.64976441208358,1.,-1.08304289898623));
#49488=CARTESIAN_POINT('Ctrl Pts',(-3.65709649161166,-1.,-1.08395671077807));
#49489=CARTESIAN_POINT('Ctrl Pts',(-3.65709649161166,1.,-1.08395671077807));
#49490=CARTESIAN_POINT('Ctrl Pts',(-3.66422237895365,-1.,-1.08471809922901));
#49491=CARTESIAN_POINT('Ctrl Pts',(-3.66422237895365,1.,-1.08471809922901));
#49492=CARTESIAN_POINT('Ctrl Pts',(-3.67127347729666,-1.,-1.0853733414449));
#49493=CARTESIAN_POINT('Ctrl Pts',(-3.67127347729666,1.,-1.0853733414449));
#49494=CARTESIAN_POINT('Ctrl Pts',(-3.67838211685117,-1.,-1.0859675575576));
#49495=CARTESIAN_POINT('Ctrl Pts',(-3.67838211685117,1.,-1.0859675575576));
#49496=CARTESIAN_POINT('Ctrl Pts',(-3.68562817420797,-1.,-1.0865288888259));
#49497=CARTESIAN_POINT('Ctrl Pts',(-3.68562817420797,1.,-1.0865288888259));
#49498=CARTESIAN_POINT('Ctrl Pts',(-3.69302062410157,-1.,-1.08706319540271));
#49499=CARTESIAN_POINT('Ctrl Pts',(-3.69302062410157,1.,-1.08706319540271));
#49500=CARTESIAN_POINT('Ctrl Pts',(-3.70052690909833,-1.,-1.08756311291309));
#49501=CARTESIAN_POINT('Ctrl Pts',(-3.70052690909833,1.,-1.08756311291309));
#49502=CARTESIAN_POINT('Ctrl Pts',(-3.70809084139457,-1.,-1.08801367312185));
#49503=CARTESIAN_POINT('Ctrl Pts',(-3.70809084139457,1.,-1.08801367312185));
#49504=CARTESIAN_POINT('Ctrl Pts',(-3.71565372339075,-1.,-1.0883988733478));
#49505=CARTESIAN_POINT('Ctrl Pts',(-3.71565372339075,1.,-1.0883988733478));
#49506=CARTESIAN_POINT('Ctrl Pts',(-3.72317741369398,-1.,-1.08870887220082));
#49507=CARTESIAN_POINT('Ctrl Pts',(-3.72317741369398,1.,-1.08870887220082));
#49508=CARTESIAN_POINT('Ctrl Pts',(-3.73065515162988,-1.,-1.08894337390937));
#49509=CARTESIAN_POINT('Ctrl Pts',(-3.73065515162988,1.,-1.08894337390937));
#49510=CARTESIAN_POINT('Ctrl Pts',(-3.73809879348239,-1.,-1.08910769013297));
#49511=CARTESIAN_POINT('Ctrl Pts',(-3.73809879348239,1.,-1.08910769013297));
#49512=CARTESIAN_POINT('Ctrl Pts',(-3.74553121371757,-1.,-1.08921040494017));
#49513=CARTESIAN_POINT('Ctrl Pts',(-3.74553121371757,1.,-1.08921040494017));
#49514=CARTESIAN_POINT('Ctrl Pts',(-3.75297711748132,-1.,-1.08926054632925));
#49515=CARTESIAN_POINT('Ctrl Pts',(-3.75297711748132,1.,-1.08926054632925));
#49516=CARTESIAN_POINT('Ctrl Pts',(-3.76045342580208,-1.,-1.08926462734281));
#49517=CARTESIAN_POINT('Ctrl Pts',(-3.76045342580208,1.,-1.08926462734281));
#49518=CARTESIAN_POINT('Ctrl Pts',(-3.76796340094448,-1.,-1.08922484204256));
#49519=CARTESIAN_POINT('Ctrl Pts',(-3.76796340094448,1.,-1.08922484204256));
#49520=CARTESIAN_POINT('Ctrl Pts',(-3.77550199409424,-1.,-1.0891407279127));
#49521=CARTESIAN_POINT('Ctrl Pts',(-3.77550199409424,1.,-1.0891407279127));
#49522=CARTESIAN_POINT('Ctrl Pts',(-3.78305911299504,-1.,-1.08901018614636));
#49523=CARTESIAN_POINT('Ctrl Pts',(-3.78305911299504,1.,-1.08901018614636));
#49524=CARTESIAN_POINT('Ctrl Pts',(-3.79062357974404,-1.,-1.08883071512098));
#49525=CARTESIAN_POINT('Ctrl Pts',(-3.79062357974404,1.,-1.08883071512098));
#49526=CARTESIAN_POINT('Ctrl Pts',(-3.79818708705259,-1.,-1.08860064435778));
#49527=CARTESIAN_POINT('Ctrl Pts',(-3.79818708705259,1.,-1.08860064435778));
#49528=CARTESIAN_POINT('Ctrl Pts',(-3.8057472665766,-1.,-1.0883200925538));
#49529=CARTESIAN_POINT('Ctrl Pts',(-3.8057472665766,1.,-1.0883200925538));
#49530=CARTESIAN_POINT('Ctrl Pts',(-3.81330554446323,-1.,-1.08799030610862));
#49531=CARTESIAN_POINT('Ctrl Pts',(-3.81330554446323,1.,-1.08799030610862));
#49532=CARTESIAN_POINT('Ctrl Pts',(-3.82086569676319,-1.,-1.08761321539442));
#49533=CARTESIAN_POINT('Ctrl Pts',(-3.82086569676319,1.,-1.08761321539442));
#49534=CARTESIAN_POINT('Ctrl Pts',(-3.82843215316984,-1.,-1.08719091307558));
#49535=CARTESIAN_POINT('Ctrl Pts',(-3.82843215316984,1.,-1.08719091307558));
#49536=CARTESIAN_POINT('Ctrl Pts',(-3.83600837071708,-1.,-1.08672515456902));
#49537=CARTESIAN_POINT('Ctrl Pts',(-3.83600837071708,1.,-1.08672515456902));
#49538=CARTESIAN_POINT('Ctrl Pts',(-3.8435952876495,-1.,-1.08621688337604));
#49539=CARTESIAN_POINT('Ctrl Pts',(-3.8435952876495,1.,-1.08621688337604));
#49540=CARTESIAN_POINT('Ctrl Pts',(-3.85119211322755,-1.,-1.08566647671844));
#49541=CARTESIAN_POINT('Ctrl Pts',(-3.85119211322755,1.,-1.08566647671844));
#49542=CARTESIAN_POINT('Ctrl Pts',(-3.85879698702532,-1.,-1.08507395120059));
#49543=CARTESIAN_POINT('Ctrl Pts',(-3.85879698702532,1.,-1.08507395120059));
#49544=CARTESIAN_POINT('Ctrl Pts',(-3.86640769434274,-1.,-1.08443918607927));
#49545=CARTESIAN_POINT('Ctrl Pts',(-3.86640769434274,1.,-1.08443918607927));
#49546=CARTESIAN_POINT('Ctrl Pts',(-3.8740223372254,-1.,-1.08376213307504));
#49547=CARTESIAN_POINT('Ctrl Pts',(-3.8740223372254,1.,-1.08376213307504));
#49548=CARTESIAN_POINT('Ctrl Pts',(-3.88164007721312,-1.,-1.08304304871028));
#49549=CARTESIAN_POINT('Ctrl Pts',(-3.88164007721312,1.,-1.08304304871028));
#49550=CARTESIAN_POINT('Ctrl Pts',(-3.88926088975114,-1.,-1.08228241999346));
#49551=CARTESIAN_POINT('Ctrl Pts',(-3.88926088975114,1.,-1.08228241999346));
#49552=CARTESIAN_POINT('Ctrl Pts',(-3.8968852509835,-1.,-1.08148086931358));
#49553=CARTESIAN_POINT('Ctrl Pts',(-3.8968852509835,1.,-1.08148086931358));
#49554=CARTESIAN_POINT('Ctrl Pts',(-3.90451384092545,-1.,-1.08063906483818));
#49555=CARTESIAN_POINT('Ctrl Pts',(-3.90451384092545,1.,-1.08063906483818));
#49556=CARTESIAN_POINT('Ctrl Pts',(-3.91214726022143,-1.,-1.07975763507473));
#49557=CARTESIAN_POINT('Ctrl Pts',(-3.91214726022143,1.,-1.07975763507473));
#49558=CARTESIAN_POINT('Ctrl Pts',(-3.91978568924178,-1.,-1.07883706663554));
#49559=CARTESIAN_POINT('Ctrl Pts',(-3.91978568924178,1.,-1.07883706663554));
#49560=CARTESIAN_POINT('Ctrl Pts',(-3.9274289334984,-1.,-1.07787771707195));
#49561=CARTESIAN_POINT('Ctrl Pts',(-3.9274289334984,1.,-1.07787771707195));
#49562=CARTESIAN_POINT('Ctrl Pts',(-3.93507657572883,-1.,-1.07687985975384));
#49563=CARTESIAN_POINT('Ctrl Pts',(-3.93507657572883,1.,-1.07687985975384));
#49564=CARTESIAN_POINT('Ctrl Pts',(-3.94272809633331,-1.,-1.07584371946443));
#49565=CARTESIAN_POINT('Ctrl Pts',(-3.94272809633331,1.,-1.07584371946443));
#49566=CARTESIAN_POINT('Ctrl Pts',(-3.95038299600676,-1.,-1.07476950921587));
#49567=CARTESIAN_POINT('Ctrl Pts',(-3.95038299600676,1.,-1.07476950921587));
#49568=CARTESIAN_POINT('Ctrl Pts',(-3.95804094429373,-1.,-1.07365747426491));
#49569=CARTESIAN_POINT('Ctrl Pts',(-3.95804094429373,1.,-1.07365747426491));
#49570=CARTESIAN_POINT('Ctrl Pts',(-3.96570179322338,-1.,-1.07250789943007));
#49571=CARTESIAN_POINT('Ctrl Pts',(-3.96570179322338,1.,-1.07250789943007));
#49572=CARTESIAN_POINT('Ctrl Pts',(-3.9733655022223,-1.,-1.07132109206164));
#49573=CARTESIAN_POINT('Ctrl Pts',(-3.9733655022223,1.,-1.07132109206164));
#49574=CARTESIAN_POINT('Ctrl Pts',(-3.98103208801101,-1.,-1.07009737257767));
#49575=CARTESIAN_POINT('Ctrl Pts',(-3.98103208801101,1.,-1.07009737257767));
#49576=CARTESIAN_POINT('Ctrl Pts',(-3.98870156857412,-1.,-1.06883706263941));
#49577=CARTESIAN_POINT('Ctrl Pts',(-3.98870156857412,1.,-1.06883706263941));
#49578=CARTESIAN_POINT('Ctrl Pts',(-3.99637389920441,-1.,-1.06754047381312));
#49579=CARTESIAN_POINT('Ctrl Pts',(-3.99637389920441,1.,-1.06754047381312));
#49580=CARTESIAN_POINT('Ctrl Pts',(-4.00404894952579,-1.,-1.06620789963606));
#49581=CARTESIAN_POINT('Ctrl Pts',(-4.00404894952579,1.,-1.06620789963606));
#49582=CARTESIAN_POINT('Ctrl Pts',(-4.01172654187398,-1.,-1.06483961343109));
#49583=CARTESIAN_POINT('Ctrl Pts',(-4.01172654187398,1.,-1.06483961343109));
#49584=CARTESIAN_POINT('Ctrl Pts',(-4.01940647495943,-1.,-1.06343586496236));
#49585=CARTESIAN_POINT('Ctrl Pts',(-4.01940647495943,1.,-1.06343586496236));
#49586=CARTESIAN_POINT('Ctrl Pts',(-4.02708855235633,-1.,-1.06199687787462));
#49587=CARTESIAN_POINT('Ctrl Pts',(-4.02708855235633,1.,-1.06199687787462));
#49588=CARTESIAN_POINT('Ctrl Pts',(-4.03477261141553,-1.,-1.06052284711857));
#49589=CARTESIAN_POINT('Ctrl Pts',(-4.03477261141553,1.,-1.06052284711857));
#49590=CARTESIAN_POINT('Ctrl Pts',(-4.04245854427496,-1.,-1.05901393666566));
#49591=CARTESIAN_POINT('Ctrl Pts',(-4.04245854427496,1.,-1.05901393666566));
#49592=CARTESIAN_POINT('Ctrl Pts',(-4.05014628384869,-1.,-1.05747027727959));
#49593=CARTESIAN_POINT('Ctrl Pts',(-4.05014628384869,1.,-1.05747027727959));
#49594=CARTESIAN_POINT('Ctrl Pts',(-4.05629789307025,-1.,-1.05620762707996));
#49595=CARTESIAN_POINT('Ctrl Pts',(-4.05629789307025,1.,-1.05620762707996));
#49596=CARTESIAN_POINT('Ctrl Pts',(-4.06091239149123,-1.,-1.05524507177599));
#49597=CARTESIAN_POINT('Ctrl Pts',(-4.06091239149123,1.,-1.05524507177599));
#49598=CARTESIAN_POINT('Ctrl Pts',(-4.06398907542249,-1.,-1.05459645194823));
#49599=CARTESIAN_POINT('Ctrl Pts',(-4.06398907542249,1.,-1.05459645194823));
#49600=CARTESIAN_POINT('Ctrl Pts',(-4.06552750530042,-1.,-1.05427041296137));
#49601=CARTESIAN_POINT('Ctrl Pts',(-4.06552750530042,1.,-1.05427041296137));
#49602=CARTESIAN_POINT('',(-3.59360648251073,1.,-1.07167739962028));
#49603=CARTESIAN_POINT('Ctrl Pts',(-3.59360648251073,-1.,-1.07167739962028));
#49604=CARTESIAN_POINT('Ctrl Pts',(-3.59360648251073,-0.666666666666667,
-1.07167739962028));
#49605=CARTESIAN_POINT('Ctrl Pts',(-3.59360648251073,-0.333333333333333,
-1.07167739962028));
#49606=CARTESIAN_POINT('Ctrl Pts',(-3.59360648251073,0.333333333333333,
-1.07167739962028));
#49607=CARTESIAN_POINT('Ctrl Pts',(-3.59360648251073,0.666666666666667,
-1.07167739962028));
#49608=CARTESIAN_POINT('Ctrl Pts',(-3.59360648251073,1.,-1.07167739962028));
#49609=CARTESIAN_POINT('',(-4.06552750530042,1.,-1.05427041296137));
#49610=CARTESIAN_POINT('',(-4.06552750530042,0.,-1.05427041296137));
#49611=CARTESIAN_POINT('Ctrl Pts',(-3.59360648251073,1.,-1.07167739962028));
#49612=CARTESIAN_POINT('Ctrl Pts',(-3.5936351279798,1.,-1.07171709254135));
#49613=CARTESIAN_POINT('Ctrl Pts',(-3.59379266874567,1.,-1.07183575450617));
#49614=CARTESIAN_POINT('Ctrl Pts',(-3.59439596999862,1.,-1.07209229745229));
#49615=CARTESIAN_POINT('Ctrl Pts',(-3.59600583194946,1.,-1.07259084660936));
#49616=CARTESIAN_POINT('Ctrl Pts',(-3.59940121154535,1.,-1.07347372545714));
#49617=CARTESIAN_POINT('Ctrl Pts',(-3.60456339887778,1.,-1.07469327168578));
#49618=CARTESIAN_POINT('Ctrl Pts',(-3.61098481349204,1.,-1.07611545402734));
#49619=CARTESIAN_POINT('Ctrl Pts',(-3.61832318504574,1.,-1.07764868137619));
#49620=CARTESIAN_POINT('Ctrl Pts',(-3.62619537902361,1.,-1.07919137290742));
#49621=CARTESIAN_POINT('Ctrl Pts',(-3.63423373196529,1.,-1.08064765719867));
#49622=CARTESIAN_POINT('Ctrl Pts',(-3.64214167843677,1.,-1.08194278850996));
#49623=CARTESIAN_POINT('Ctrl Pts',(-3.64976441208358,1.,-1.08304289898623));
#49624=CARTESIAN_POINT('Ctrl Pts',(-3.65709649161166,1.,-1.08395671077807));
#49625=CARTESIAN_POINT('Ctrl Pts',(-3.66422237895365,1.,-1.08471809922901));
#49626=CARTESIAN_POINT('Ctrl Pts',(-3.67127347729666,1.,-1.0853733414449));
#49627=CARTESIAN_POINT('Ctrl Pts',(-3.67838211685117,1.,-1.0859675575576));
#49628=CARTESIAN_POINT('Ctrl Pts',(-3.68562817420797,1.,-1.0865288888259));
#49629=CARTESIAN_POINT('Ctrl Pts',(-3.69302062410157,1.,-1.08706319540271));
#49630=CARTESIAN_POINT('Ctrl Pts',(-3.70052690909833,1.,-1.08756311291309));
#49631=CARTESIAN_POINT('Ctrl Pts',(-3.70809084139457,1.,-1.08801367312185));
#49632=CARTESIAN_POINT('Ctrl Pts',(-3.71565372339075,1.,-1.0883988733478));
#49633=CARTESIAN_POINT('Ctrl Pts',(-3.72317741369398,1.,-1.08870887220082));
#49634=CARTESIAN_POINT('Ctrl Pts',(-3.73065515162988,1.,-1.08894337390937));
#49635=CARTESIAN_POINT('Ctrl Pts',(-3.73809879348239,1.,-1.08910769013297));
#49636=CARTESIAN_POINT('Ctrl Pts',(-3.74553121371757,1.,-1.08921040494017));
#49637=CARTESIAN_POINT('Ctrl Pts',(-3.75297711748132,1.,-1.08926054632925));
#49638=CARTESIAN_POINT('Ctrl Pts',(-3.76045342580208,1.,-1.08926462734281));
#49639=CARTESIAN_POINT('Ctrl Pts',(-3.76796340094448,1.,-1.08922484204256));
#49640=CARTESIAN_POINT('Ctrl Pts',(-3.77550199409424,1.,-1.0891407279127));
#49641=CARTESIAN_POINT('Ctrl Pts',(-3.78305911299504,1.,-1.08901018614636));
#49642=CARTESIAN_POINT('Ctrl Pts',(-3.79062357974404,1.,-1.08883071512098));
#49643=CARTESIAN_POINT('Ctrl Pts',(-3.79818708705259,1.,-1.08860064435778));
#49644=CARTESIAN_POINT('Ctrl Pts',(-3.8057472665766,1.,-1.0883200925538));
#49645=CARTESIAN_POINT('Ctrl Pts',(-3.81330554446323,1.,-1.08799030610862));
#49646=CARTESIAN_POINT('Ctrl Pts',(-3.82086569676319,1.,-1.08761321539442));
#49647=CARTESIAN_POINT('Ctrl Pts',(-3.82843215316984,1.,-1.08719091307558));
#49648=CARTESIAN_POINT('Ctrl Pts',(-3.83600837071708,1.,-1.08672515456902));
#49649=CARTESIAN_POINT('Ctrl Pts',(-3.8435952876495,1.,-1.08621688337604));
#49650=CARTESIAN_POINT('Ctrl Pts',(-3.85119211322755,1.,-1.08566647671844));
#49651=CARTESIAN_POINT('Ctrl Pts',(-3.85879698702532,1.,-1.08507395120059));
#49652=CARTESIAN_POINT('Ctrl Pts',(-3.86640769434274,1.,-1.08443918607927));
#49653=CARTESIAN_POINT('Ctrl Pts',(-3.8740223372254,1.,-1.08376213307504));
#49654=CARTESIAN_POINT('Ctrl Pts',(-3.88164007721312,1.,-1.08304304871028));
#49655=CARTESIAN_POINT('Ctrl Pts',(-3.88926088975114,1.,-1.08228241999346));
#49656=CARTESIAN_POINT('Ctrl Pts',(-3.8968852509835,1.,-1.08148086931358));
#49657=CARTESIAN_POINT('Ctrl Pts',(-3.90451384092545,1.,-1.08063906483818));
#49658=CARTESIAN_POINT('Ctrl Pts',(-3.91214726022143,1.,-1.07975763507473));
#49659=CARTESIAN_POINT('Ctrl Pts',(-3.91978568924178,1.,-1.07883706663554));
#49660=CARTESIAN_POINT('Ctrl Pts',(-3.9274289334984,1.,-1.07787771707195));
#49661=CARTESIAN_POINT('Ctrl Pts',(-3.93507657572883,1.,-1.07687985975384));
#49662=CARTESIAN_POINT('Ctrl Pts',(-3.94272809633331,1.,-1.07584371946443));
#49663=CARTESIAN_POINT('Ctrl Pts',(-3.95038299600676,1.,-1.07476950921587));
#49664=CARTESIAN_POINT('Ctrl Pts',(-3.95804094429373,1.,-1.07365747426491));
#49665=CARTESIAN_POINT('Ctrl Pts',(-3.96570179322338,1.,-1.07250789943007));
#49666=CARTESIAN_POINT('Ctrl Pts',(-3.9733655022223,1.,-1.07132109206164));
#49667=CARTESIAN_POINT('Ctrl Pts',(-3.98103208801101,1.,-1.07009737257767));
#49668=CARTESIAN_POINT('Ctrl Pts',(-3.98870156857412,1.,-1.06883706263941));
#49669=CARTESIAN_POINT('Ctrl Pts',(-3.99637389920441,1.,-1.06754047381312));
#49670=CARTESIAN_POINT('Ctrl Pts',(-4.00404894952579,1.,-1.06620789963606));
#49671=CARTESIAN_POINT('Ctrl Pts',(-4.01172654187398,1.,-1.06483961343109));
#49672=CARTESIAN_POINT('Ctrl Pts',(-4.01940647495943,1.,-1.06343586496236));
#49673=CARTESIAN_POINT('Ctrl Pts',(-4.02708855235633,1.,-1.06199687787462));
#49674=CARTESIAN_POINT('Ctrl Pts',(-4.03477261141553,1.,-1.06052284711857));
#49675=CARTESIAN_POINT('Ctrl Pts',(-4.04245854427496,1.,-1.05901393666566));
#49676=CARTESIAN_POINT('Ctrl Pts',(-4.05014628384869,1.,-1.05747027727959));
#49677=CARTESIAN_POINT('Ctrl Pts',(-4.05629789307025,1.,-1.05620762707996));
#49678=CARTESIAN_POINT('Ctrl Pts',(-4.06091239149123,1.,-1.05524507177599));
#49679=CARTESIAN_POINT('Ctrl Pts',(-4.06398907542249,1.,-1.05459645194823));
#49680=CARTESIAN_POINT('Ctrl Pts',(-4.06552750530042,1.,-1.05427041296137));
#49681=CARTESIAN_POINT('Origin',(-4.06552750530042,0.,-1.05427041296137));
#49682=CARTESIAN_POINT('',(-4.10104028313088,1.,-0.906349047628866));
#49683=CARTESIAN_POINT('Origin',(0.,0.,0.));
#49684=CARTESIAN_POINT('',(-3.5372048861597,1.,-1.24526366418038));
#49685=CARTESIAN_POINT('Origin',(0.,1.,0.));
#49686=CARTESIAN_POINT('Ctrl Pts',(-3.5372048861597,1.,-1.24526366418038));
#49687=CARTESIAN_POINT('Ctrl Pts',(-3.5372048861597,0.666666666666667,-1.24526366418038));
#49688=CARTESIAN_POINT('Ctrl Pts',(-3.5372048861597,0.333333333333333,-1.24526366418038));
#49689=CARTESIAN_POINT('Ctrl Pts',(-3.5372048861597,-0.333333333333333,
-1.24526366418038));
#49690=CARTESIAN_POINT('Ctrl Pts',(-3.5372048861597,-0.666666666666667,
-1.24526366418038));
#49691=CARTESIAN_POINT('Ctrl Pts',(-3.5372048861597,-1.,-1.24526366418038));
#49692=CARTESIAN_POINT('Ctrl Pts',(-3.90876544355381,-1.,-1.53673442965256));
#49693=CARTESIAN_POINT('Ctrl Pts',(-3.90876544355381,1.,-1.53673442965256));
#49694=CARTESIAN_POINT('Ctrl Pts',(-3.90771246855019,-1.,-1.53556639217905));
#49695=CARTESIAN_POINT('Ctrl Pts',(-3.90771246855019,1.,-1.53556639217905));
#49696=CARTESIAN_POINT('Ctrl Pts',(-3.90560462813969,-1.,-1.53323321827755));
#49697=CARTESIAN_POINT('Ctrl Pts',(-3.90560462813969,1.,-1.53323321827755));
#49698=CARTESIAN_POINT('Ctrl Pts',(-3.90243719631596,-1.,-1.52974216056287));
#49699=CARTESIAN_POINT('Ctrl Pts',(-3.90243719631596,1.,-1.52974216056287));
#49700=CARTESIAN_POINT('Ctrl Pts',(-3.89820260708225,-1.,-1.52510482991635));
#49701=CARTESIAN_POINT('Ctrl Pts',(-3.89820260708225,1.,-1.52510482991635));
#49702=CARTESIAN_POINT('Ctrl Pts',(-3.89289043533657,-1.,-1.51933724329305));
#49703=CARTESIAN_POINT('Ctrl Pts',(-3.89289043533657,1.,-1.51933724329305));
#49704=CARTESIAN_POINT('Ctrl Pts',(-3.88755930033884,-1.,-1.51359883110559));
#49705=CARTESIAN_POINT('Ctrl Pts',(-3.88755930033884,1.,-1.51359883110559));
#49706=CARTESIAN_POINT('Ctrl Pts',(-3.88220917950538,-1.,-1.50788973857757));
#49707=CARTESIAN_POINT('Ctrl Pts',(-3.88220917950538,1.,-1.50788973857757));
#49708=CARTESIAN_POINT('Ctrl Pts',(-3.87684006372134,-1.,-1.50221016176556));
#49709=CARTESIAN_POINT('Ctrl Pts',(-3.87684006372134,1.,-1.50221016176556));
#49710=CARTESIAN_POINT('Ctrl Pts',(-3.87145196998465,-1.,-1.49656035399122));
#49711=CARTESIAN_POINT('Ctrl Pts',(-3.87145196998465,1.,-1.49656035399122));
#49712=CARTESIAN_POINT('Ctrl Pts',(-3.86604492575189,-1.,-1.4909406116431));
#49713=CARTESIAN_POINT('Ctrl Pts',(-3.86604492575189,1.,-1.4909406116431));
#49714=CARTESIAN_POINT('Ctrl Pts',(-3.86061894706087,-1.,-1.48535125509919));
#49715=CARTESIAN_POINT('Ctrl Pts',(-3.86061894706087,1.,-1.48535125509919));
#49716=CARTESIAN_POINT('Ctrl Pts',(-3.85517401698843,-1.,-1.4797926099102));
#49717=CARTESIAN_POINT('Ctrl Pts',(-3.85517401698843,1.,-1.4797926099102));
#49718=CARTESIAN_POINT('Ctrl Pts',(-3.84971006847277,-1.,-1.47426499018538));
#49719=CARTESIAN_POINT('Ctrl Pts',(-3.84971006847277,1.,-1.47426499018538));
#49720=CARTESIAN_POINT('Ctrl Pts',(-3.84422695454796,-1.,-1.46876867426504));
#49721=CARTESIAN_POINT('Ctrl Pts',(-3.84422695454796,1.,-1.46876867426504));
#49722=CARTESIAN_POINT('Ctrl Pts',(-3.83872447159639,-1.,-1.46330391180752));
#49723=CARTESIAN_POINT('Ctrl Pts',(-3.83872447159639,1.,-1.46330391180752));
#49724=CARTESIAN_POINT('Ctrl Pts',(-3.83320241775423,-1.,-1.45787095220852));
#49725=CARTESIAN_POINT('Ctrl Pts',(-3.83320241775423,1.,-1.45787095220852));
#49726=CARTESIAN_POINT('Ctrl Pts',(-3.82766064519074,-1.,-1.45247006796836));
#49727=CARTESIAN_POINT('Ctrl Pts',(-3.82766064519074,1.,-1.45247006796836));
#49728=CARTESIAN_POINT('Ctrl Pts',(-3.82209910620533,-1.,-1.44710157648539));
#49729=CARTESIAN_POINT('Ctrl Pts',(-3.82209910620533,1.,-1.44710157648539));
#49730=CARTESIAN_POINT('Ctrl Pts',(-3.81651792398414,-1.,-1.44176587041347));
#49731=CARTESIAN_POINT('Ctrl Pts',(-3.81651792398414,1.,-1.44176587041347));
#49732=CARTESIAN_POINT('Ctrl Pts',(-3.81091737726815,-1.,-1.43646341556724));
#49733=CARTESIAN_POINT('Ctrl Pts',(-3.81091737726815,1.,-1.43646341556724));
#49734=CARTESIAN_POINT('Ctrl Pts',(-3.80529775429805,-1.,-1.4311946992132));
#49735=CARTESIAN_POINT('Ctrl Pts',(-3.80529775429805,1.,-1.4311946992132));
#49736=CARTESIAN_POINT('Ctrl Pts',(-3.7996592319632,-1.,-1.42596018777283));
#49737=CARTESIAN_POINT('Ctrl Pts',(-3.7996592319632,1.,-1.42596018777283));
#49738=CARTESIAN_POINT('Ctrl Pts',(-3.79400175744408,-1.,-1.42076028482836));
#49739=CARTESIAN_POINT('Ctrl Pts',(-3.79400175744408,1.,-1.42076028482836));
#49740=CARTESIAN_POINT('Ctrl Pts',(-3.78832489879426,-1.,-1.4155952780383));
#49741=CARTESIAN_POINT('Ctrl Pts',(-3.78832489879426,1.,-1.4155952780383));
#49742=CARTESIAN_POINT('Ctrl Pts',(-3.78262780065471,-1.,-1.41046532282593));
#49743=CARTESIAN_POINT('Ctrl Pts',(-3.78262780065471,1.,-1.41046532282593));
#49744=CARTESIAN_POINT('Ctrl Pts',(-3.77690952014259,-1.,-1.40537056004722));
#49745=CARTESIAN_POINT('Ctrl Pts',(-3.77690952014259,1.,-1.40537056004722));
#49746=CARTESIAN_POINT('Ctrl Pts',(-3.77116930621827,-1.,-1.40031121335505));
#49747=CARTESIAN_POINT('Ctrl Pts',(-3.77116930621827,1.,-1.40031121335505));
#49748=CARTESIAN_POINT('Ctrl Pts',(-3.76540689249074,-1.,-1.39528769118052));
#49749=CARTESIAN_POINT('Ctrl Pts',(-3.76540689249074,1.,-1.39528769118052));
#49750=CARTESIAN_POINT('Ctrl Pts',(-3.75962280650855,-1.,-1.39030069388918));
#49751=CARTESIAN_POINT('Ctrl Pts',(-3.75962280650855,1.,-1.39030069388918));
#49752=CARTESIAN_POINT('Ctrl Pts',(-3.75381861212707,-1.,-1.38535129801176));
#49753=CARTESIAN_POINT('Ctrl Pts',(-3.75381861212707,1.,-1.38535129801176));
#49754=CARTESIAN_POINT('Ctrl Pts',(-3.74799617204729,-1.,-1.38044070763295));
#49755=CARTESIAN_POINT('Ctrl Pts',(-3.74799617204729,1.,-1.38044070763295));
#49756=CARTESIAN_POINT('Ctrl Pts',(-3.74215698162555,-1.,-1.37557002971687));
#49757=CARTESIAN_POINT('Ctrl Pts',(-3.74215698162555,1.,-1.37557002971687));
#49758=CARTESIAN_POINT('Ctrl Pts',(-3.7363014588581,-1.,-1.37074003422739));
#49759=CARTESIAN_POINT('Ctrl Pts',(-3.7363014588581,1.,-1.37074003422739));
#49760=CARTESIAN_POINT('Ctrl Pts',(-3.73042829011295,-1.,-1.36595093298676));
#49761=CARTESIAN_POINT('Ctrl Pts',(-3.73042829011295,1.,-1.36595093298676));
#49762=CARTESIAN_POINT('Ctrl Pts',(-3.72453364678279,-1.,-1.36120211416354));
#49763=CARTESIAN_POINT('Ctrl Pts',(-3.72453364678279,1.,-1.36120211416354));
#49764=CARTESIAN_POINT('Ctrl Pts',(-3.71861271513313,-1.,-1.35649266705037));
#49765=CARTESIAN_POINT('Ctrl Pts',(-3.71861271513313,1.,-1.35649266705037));
#49766=CARTESIAN_POINT('Ctrl Pts',(-3.71266130563054,-1.,-1.35182193384424));
#49767=CARTESIAN_POINT('Ctrl Pts',(-3.71266130563054,1.,-1.35182193384424));
#49768=CARTESIAN_POINT('Ctrl Pts',(-3.70667753188248,-1.,-1.34719008463534));
#49769=CARTESIAN_POINT('Ctrl Pts',(-3.70667753188248,1.,-1.34719008463534));
#49770=CARTESIAN_POINT('Ctrl Pts',(-3.70066324015119,-1.,-1.34259860752933));
#49771=CARTESIAN_POINT('Ctrl Pts',(-3.70066324015119,1.,-1.34259860752933));
#49772=CARTESIAN_POINT('Ctrl Pts',(-3.69462613305708,-1.,-1.33805103398219));
#49773=CARTESIAN_POINT('Ctrl Pts',(-3.69462613305708,1.,-1.33805103398219));
#49774=CARTESIAN_POINT('Ctrl Pts',(-3.68857672413033,-1.,-1.33355191034523));
#49775=CARTESIAN_POINT('Ctrl Pts',(-3.68857672413033,1.,-1.33355191034523));
#49776=CARTESIAN_POINT('Ctrl Pts',(-3.68252441182551,-1.,-1.3291054707274));
#49777=CARTESIAN_POINT('Ctrl Pts',(-3.68252441182551,1.,-1.3291054707274));
#49778=CARTESIAN_POINT('Ctrl Pts',(-3.67647355257912,-1.,-1.32471430856415));
#49779=CARTESIAN_POINT('Ctrl Pts',(-3.67647355257912,1.,-1.32471430856415));
#49780=CARTESIAN_POINT('Ctrl Pts',(-3.67042021752656,-1.,-1.32037828137766));
#49781=CARTESIAN_POINT('Ctrl Pts',(-3.67042021752656,1.,-1.32037828137766));
#49782=CARTESIAN_POINT('Ctrl Pts',(-3.66434688899793,-1.,-1.31609271239911));
#49783=CARTESIAN_POINT('Ctrl Pts',(-3.66434688899793,1.,-1.31609271239911));
#49784=CARTESIAN_POINT('Ctrl Pts',(-3.65822827358617,-1.,-1.31185038411218));
#49785=CARTESIAN_POINT('Ctrl Pts',(-3.65822827358617,1.,-1.31185038411218));
#49786=CARTESIAN_POINT('Ctrl Pts',(-3.65204081987068,-1.,-1.30764479590039));
#49787=CARTESIAN_POINT('Ctrl Pts',(-3.65204081987068,1.,-1.30764479590039));
#49788=CARTESIAN_POINT('Ctrl Pts',(-3.64577181380113,-1.,-1.30347327603774));
#49789=CARTESIAN_POINT('Ctrl Pts',(-3.64577181380113,1.,-1.30347327603774));
#49790=CARTESIAN_POINT('Ctrl Pts',(-3.63942689872808,-1.,-1.2993395590647));
#49791=CARTESIAN_POINT('Ctrl Pts',(-3.63942689872808,1.,-1.2993395590647));
#49792=CARTESIAN_POINT('Ctrl Pts',(-3.63304271631046,-1.,-1.29525810207762));
#49793=CARTESIAN_POINT('Ctrl Pts',(-3.63304271631046,1.,-1.29525810207762));
#49794=CARTESIAN_POINT('Ctrl Pts',(-3.62667616004369,-1.,-1.29125046021878));
#49795=CARTESIAN_POINT('Ctrl Pts',(-3.62667616004369,1.,-1.29125046021878));
#49796=CARTESIAN_POINT('Ctrl Pts',(-3.6203814849236,-1.,-1.28733755029384));
#49797=CARTESIAN_POINT('Ctrl Pts',(-3.6203814849236,1.,-1.28733755029384));
#49798=CARTESIAN_POINT('Ctrl Pts',(-3.61418935913823,-1.,-1.28353255117765));
#49799=CARTESIAN_POINT('Ctrl Pts',(-3.61418935913823,1.,-1.28353255117765));
#49800=CARTESIAN_POINT('Ctrl Pts',(-3.60808907746339,-1.,-1.27983492861691));
#49801=CARTESIAN_POINT('Ctrl Pts',(-3.60808907746339,1.,-1.27983492861691));
#49802=CARTESIAN_POINT('Ctrl Pts',(-3.60199947736298,-1.,-1.27622049908625));
#49803=CARTESIAN_POINT('Ctrl Pts',(-3.60199947736298,1.,-1.27622049908625));
#49804=CARTESIAN_POINT('Ctrl Pts',(-3.59578698050006,-1.,-1.27264798379307));
#49805=CARTESIAN_POINT('Ctrl Pts',(-3.59578698050006,1.,-1.27264798379307));
#49806=CARTESIAN_POINT('Ctrl Pts',(-3.58931807846313,-1.,-1.26907758484709));
#49807=CARTESIAN_POINT('Ctrl Pts',(-3.58931807846313,1.,-1.26907758484709));
#49808=CARTESIAN_POINT('Ctrl Pts',(-3.58250452868618,-1.,-1.26548706249862));
#49809=CARTESIAN_POINT('Ctrl Pts',(-3.58250452868618,1.,-1.26548706249862));
#49810=CARTESIAN_POINT('Ctrl Pts',(-3.5753456065171,-1.,-1.2618866714281));
#49811=CARTESIAN_POINT('Ctrl Pts',(-3.5753456065171,1.,-1.2618866714281));
#49812=CARTESIAN_POINT('Ctrl Pts',(-3.56798645995275,-1.,-1.25834000485716));
#49813=CARTESIAN_POINT('Ctrl Pts',(-3.56798645995275,1.,-1.25834000485716));
#49814=CARTESIAN_POINT('Ctrl Pts',(-3.56071094991199,-1.,-1.25496090900009));
#49815=CARTESIAN_POINT('Ctrl Pts',(-3.56071094991199,1.,-1.25496090900009));
#49816=CARTESIAN_POINT('Ctrl Pts',(-3.55387287418985,-1.,-1.2518879294064));
#49817=CARTESIAN_POINT('Ctrl Pts',(-3.55387287418985,1.,-1.2518879294064));
#49818=CARTESIAN_POINT('Ctrl Pts',(-3.54784190283068,-1.,-1.24926408628003));
#49819=CARTESIAN_POINT('Ctrl Pts',(-3.54784190283068,1.,-1.24926408628003));
#49820=CARTESIAN_POINT('Ctrl Pts',(-3.54294877425964,-1.,-1.24721646231966));
#49821=CARTESIAN_POINT('Ctrl Pts',(-3.54294877425964,1.,-1.24721646231966));
#49822=CARTESIAN_POINT('Ctrl Pts',(-3.53941798195825,-1.,-1.24583101679029));
#49823=CARTESIAN_POINT('Ctrl Pts',(-3.53941798195825,1.,-1.24583101679029));
#49824=CARTESIAN_POINT('Ctrl Pts',(-3.53776753802906,-1.,-1.24528461332987));
#49825=CARTESIAN_POINT('Ctrl Pts',(-3.53776753802906,1.,-1.24528461332987));
#49826=CARTESIAN_POINT('Ctrl Pts',(-3.53720633057798,-1.,-1.24519702335451));
#49827=CARTESIAN_POINT('Ctrl Pts',(-3.53720633057798,1.,-1.24519702335451));
#49828=CARTESIAN_POINT('Ctrl Pts',(-3.53713269667399,-1.,-1.24528174185098));
#49829=CARTESIAN_POINT('Ctrl Pts',(-3.53713269667399,1.,-1.24528174185098));
#49830=CARTESIAN_POINT('Ctrl Pts',(-3.53717101171257,-1.,-1.24535988127942));
#49831=CARTESIAN_POINT('Ctrl Pts',(-3.53717101171257,1.,-1.24535988127942));
#49832=CARTESIAN_POINT('',(-3.90876544355381,1.,-1.53673442965256));
#49833=CARTESIAN_POINT('Ctrl Pts',(-3.90876544355381,1.,-1.53673442965256));
#49834=CARTESIAN_POINT('Ctrl Pts',(-3.90771246855019,1.,-1.53556639217905));
#49835=CARTESIAN_POINT('Ctrl Pts',(-3.90560462813969,1.,-1.53323321827755));
#49836=CARTESIAN_POINT('Ctrl Pts',(-3.90243719631596,1.,-1.52974216056287));
#49837=CARTESIAN_POINT('Ctrl Pts',(-3.89820260708225,1.,-1.52510482991635));
#49838=CARTESIAN_POINT('Ctrl Pts',(-3.89289043533657,1.,-1.51933724329305));
#49839=CARTESIAN_POINT('Ctrl Pts',(-3.88755930033884,1.,-1.51359883110559));
#49840=CARTESIAN_POINT('Ctrl Pts',(-3.88220917950538,1.,-1.50788973857757));
#49841=CARTESIAN_POINT('Ctrl Pts',(-3.87684006372134,1.,-1.50221016176556));
#49842=CARTESIAN_POINT('Ctrl Pts',(-3.87145196998465,1.,-1.49656035399122));
#49843=CARTESIAN_POINT('Ctrl Pts',(-3.86604492575189,1.,-1.4909406116431));
#49844=CARTESIAN_POINT('Ctrl Pts',(-3.86061894706087,1.,-1.48535125509919));
#49845=CARTESIAN_POINT('Ctrl Pts',(-3.85517401698843,1.,-1.4797926099102));
#49846=CARTESIAN_POINT('Ctrl Pts',(-3.84971006847277,1.,-1.47426499018538));
#49847=CARTESIAN_POINT('Ctrl Pts',(-3.84422695454796,1.,-1.46876867426504));
#49848=CARTESIAN_POINT('Ctrl Pts',(-3.83872447159639,1.,-1.46330391180752));
#49849=CARTESIAN_POINT('Ctrl Pts',(-3.83320241775423,1.,-1.45787095220852));
#49850=CARTESIAN_POINT('Ctrl Pts',(-3.82766064519074,1.,-1.45247006796836));
#49851=CARTESIAN_POINT('Ctrl Pts',(-3.82209910620533,1.,-1.44710157648539));
#49852=CARTESIAN_POINT('Ctrl Pts',(-3.81651792398414,1.,-1.44176587041347));
#49853=CARTESIAN_POINT('Ctrl Pts',(-3.81091737726815,1.,-1.43646341556724));
#49854=CARTESIAN_POINT('Ctrl Pts',(-3.80529775429805,1.,-1.4311946992132));
#49855=CARTESIAN_POINT('Ctrl Pts',(-3.7996592319632,1.,-1.42596018777283));
#49856=CARTESIAN_POINT('Ctrl Pts',(-3.79400175744408,1.,-1.42076028482836));
#49857=CARTESIAN_POINT('Ctrl Pts',(-3.78832489879426,1.,-1.4155952780383));
#49858=CARTESIAN_POINT('Ctrl Pts',(-3.78262780065471,1.,-1.41046532282593));
#49859=CARTESIAN_POINT('Ctrl Pts',(-3.77690952014259,1.,-1.40537056004722));
#49860=CARTESIAN_POINT('Ctrl Pts',(-3.77116930621827,1.,-1.40031121335505));
#49861=CARTESIAN_POINT('Ctrl Pts',(-3.76540689249074,1.,-1.39528769118052));
#49862=CARTESIAN_POINT('Ctrl Pts',(-3.75962280650855,1.,-1.39030069388918));
#49863=CARTESIAN_POINT('Ctrl Pts',(-3.75381861212707,1.,-1.38535129801176));
#49864=CARTESIAN_POINT('Ctrl Pts',(-3.74799617204729,1.,-1.38044070763295));
#49865=CARTESIAN_POINT('Ctrl Pts',(-3.74215698162555,1.,-1.37557002971687));
#49866=CARTESIAN_POINT('Ctrl Pts',(-3.7363014588581,1.,-1.37074003422739));
#49867=CARTESIAN_POINT('Ctrl Pts',(-3.73042829011295,1.,-1.36595093298676));
#49868=CARTESIAN_POINT('Ctrl Pts',(-3.72453364678279,1.,-1.36120211416354));
#49869=CARTESIAN_POINT('Ctrl Pts',(-3.71861271513313,1.,-1.35649266705037));
#49870=CARTESIAN_POINT('Ctrl Pts',(-3.71266130563054,1.,-1.35182193384424));
#49871=CARTESIAN_POINT('Ctrl Pts',(-3.70667753188248,1.,-1.34719008463534));
#49872=CARTESIAN_POINT('Ctrl Pts',(-3.70066324015119,1.,-1.34259860752933));
#49873=CARTESIAN_POINT('Ctrl Pts',(-3.69462613305708,1.,-1.33805103398219));
#49874=CARTESIAN_POINT('Ctrl Pts',(-3.68857672413033,1.,-1.33355191034523));
#49875=CARTESIAN_POINT('Ctrl Pts',(-3.68252441182551,1.,-1.3291054707274));
#49876=CARTESIAN_POINT('Ctrl Pts',(-3.67647355257912,1.,-1.32471430856415));
#49877=CARTESIAN_POINT('Ctrl Pts',(-3.67042021752656,1.,-1.32037828137766));
#49878=CARTESIAN_POINT('Ctrl Pts',(-3.66434688899793,1.,-1.31609271239911));
#49879=CARTESIAN_POINT('Ctrl Pts',(-3.65822827358617,1.,-1.31185038411218));
#49880=CARTESIAN_POINT('Ctrl Pts',(-3.65204081987068,1.,-1.30764479590039));
#49881=CARTESIAN_POINT('Ctrl Pts',(-3.64577181380113,1.,-1.30347327603774));
#49882=CARTESIAN_POINT('Ctrl Pts',(-3.63942689872808,1.,-1.2993395590647));
#49883=CARTESIAN_POINT('Ctrl Pts',(-3.63304271631046,1.,-1.29525810207762));
#49884=CARTESIAN_POINT('Ctrl Pts',(-3.62667616004369,1.,-1.29125046021878));
#49885=CARTESIAN_POINT('Ctrl Pts',(-3.6203814849236,1.,-1.28733755029384));
#49886=CARTESIAN_POINT('Ctrl Pts',(-3.61418935913823,1.,-1.28353255117765));
#49887=CARTESIAN_POINT('Ctrl Pts',(-3.60808907746339,1.,-1.27983492861691));
#49888=CARTESIAN_POINT('Ctrl Pts',(-3.60199947736298,1.,-1.27622049908625));
#49889=CARTESIAN_POINT('Ctrl Pts',(-3.59578698050006,1.,-1.27264798379307));
#49890=CARTESIAN_POINT('Ctrl Pts',(-3.58931807846313,1.,-1.26907758484709));
#49891=CARTESIAN_POINT('Ctrl Pts',(-3.58250452868618,1.,-1.26548706249862));
#49892=CARTESIAN_POINT('Ctrl Pts',(-3.5753456065171,1.,-1.2618866714281));
#49893=CARTESIAN_POINT('Ctrl Pts',(-3.56798645995275,1.,-1.25834000485716));
#49894=CARTESIAN_POINT('Ctrl Pts',(-3.56071094991199,1.,-1.25496090900009));
#49895=CARTESIAN_POINT('Ctrl Pts',(-3.55387287418985,1.,-1.2518879294064));
#49896=CARTESIAN_POINT('Ctrl Pts',(-3.54784190283068,1.,-1.24926408628003));
#49897=CARTESIAN_POINT('Ctrl Pts',(-3.54294877425964,1.,-1.24721646231966));
#49898=CARTESIAN_POINT('Ctrl Pts',(-3.53968291130022,1.,-1.24593497226008));
#49899=CARTESIAN_POINT('Ctrl Pts',(-3.53808746578196,1.,-1.24539205388767));
#49900=CARTESIAN_POINT('Ctrl Pts',(-3.5374485926552,1.,-1.2452449899111));
#49901=CARTESIAN_POINT('Ctrl Pts',(-3.53725139174486,1.,-1.24524838931757));
#49902=CARTESIAN_POINT('Ctrl Pts',(-3.5372048861597,1.,-1.24526366418038));
#49903=CARTESIAN_POINT('',(-3.90876544355381,0.,-1.53673442965256));
#49904=CARTESIAN_POINT('Ctrl Pts',(-3.38176002566879,-1.,-1.62055519152809));
#49905=CARTESIAN_POINT('Ctrl Pts',(-3.38176002566879,1.,-1.62055519152809));
#49906=CARTESIAN_POINT('Ctrl Pts',(-3.38167767992676,-1.,-1.62058335162482));
#49907=CARTESIAN_POINT('Ctrl Pts',(-3.38167767992676,1.,-1.62058335162482));
#49908=CARTESIAN_POINT('Ctrl Pts',(-3.38166984193836,-1.,-1.62069532368199));
#49909=CARTESIAN_POINT('Ctrl Pts',(-3.38166984193836,1.,-1.62069532368199));
#49910=CARTESIAN_POINT('Ctrl Pts',(-3.38212861099984,-1.,-1.62103022181151));
#49911=CARTESIAN_POINT('Ctrl Pts',(-3.38212861099984,1.,-1.62103022181151));
#49912=CARTESIAN_POINT('Ctrl Pts',(-3.38368201668574,-1.,-1.62181089631344));
#49913=CARTESIAN_POINT('Ctrl Pts',(-3.38368201668574,1.,-1.62181089631344));
#49914=CARTESIAN_POINT('Ctrl Pts',(-3.38715832179072,-1.,-1.6233278855625));
#49915=CARTESIAN_POINT('Ctrl Pts',(-3.38715832179072,1.,-1.6233278855625));
#49916=CARTESIAN_POINT('Ctrl Pts',(-3.39206617496906,-1.,-1.62533996116713));
#49917=CARTESIAN_POINT('Ctrl Pts',(-3.39206617496906,1.,-1.62533996116713));
#49918=CARTESIAN_POINT('Ctrl Pts',(-3.39818605297991,-1.,-1.62774916464408));
#49919=CARTESIAN_POINT('Ctrl Pts',(-3.39818605297991,1.,-1.62774916464408));
#49920=CARTESIAN_POINT('Ctrl Pts',(-3.40519422740235,-1.,-1.63041148964828));
#49921=CARTESIAN_POINT('Ctrl Pts',(-3.40519422740235,1.,-1.63041148964828));
#49922=CARTESIAN_POINT('Ctrl Pts',(-3.41272817148478,-1.,-1.63316667054044));
#49923=CARTESIAN_POINT('Ctrl Pts',(-3.41272817148478,1.,-1.63316667054044));
#49924=CARTESIAN_POINT('Ctrl Pts',(-3.42043974590882,-1.,-1.63586250099773));
#49925=CARTESIAN_POINT('Ctrl Pts',(-3.42043974590882,1.,-1.63586250099773));
#49926=CARTESIAN_POINT('Ctrl Pts',(-3.42804772926291,-1.,-1.63837876246926));
#49927=CARTESIAN_POINT('Ctrl Pts',(-3.42804772926291,1.,-1.63837876246926));
#49928=CARTESIAN_POINT('Ctrl Pts',(-3.43540451921548,-1.,-1.64065778702023));
#49929=CARTESIAN_POINT('Ctrl Pts',(-3.43540451921548,1.,-1.64065778702023));
#49930=CARTESIAN_POINT('Ctrl Pts',(-3.44250337701888,-1.,-1.64270733821113));
#49931=CARTESIAN_POINT('Ctrl Pts',(-3.44250337701888,1.,-1.64270733821113));
#49932=CARTESIAN_POINT('Ctrl Pts',(-3.44942242546795,-1.,-1.64457408708107));
#49933=CARTESIAN_POINT('Ctrl Pts',(-3.44942242546795,1.,-1.64457408708107));
#49934=CARTESIAN_POINT('Ctrl Pts',(-3.45628421062422,-1.,-1.64632429697521));
#49935=CARTESIAN_POINT('Ctrl Pts',(-3.45628421062422,1.,-1.64632429697521));
#49936=CARTESIAN_POINT('Ctrl Pts',(-3.46321237515,-1.,-1.64802323352738));
#49937=CARTESIAN_POINT('Ctrl Pts',(-3.46321237515,1.,-1.64802323352738));
#49938=CARTESIAN_POINT('Ctrl Pts',(-3.47028140995992,-1.,-1.64971118698256));
#49939=CARTESIAN_POINT('Ctrl Pts',(-3.47028140995992,1.,-1.64971118698256));
#49940=CARTESIAN_POINT('Ctrl Pts',(-3.47749926256476,-1.,-1.65139534930322));
#49941=CARTESIAN_POINT('Ctrl Pts',(-3.47749926256476,1.,-1.65139534930322));
#49942=CARTESIAN_POINT('Ctrl Pts',(-3.48483492840894,-1.,-1.65306335367739));
#49943=CARTESIAN_POINT('Ctrl Pts',(-3.48483492840894,1.,-1.65306335367739));
#49944=CARTESIAN_POINT('Ctrl Pts',(-3.49223525300176,-1.,-1.65469162644468));
#49945=CARTESIAN_POINT('Ctrl Pts',(-3.49223525300176,1.,-1.65469162644468));
#49946=CARTESIAN_POINT('Ctrl Pts',(-3.4996447647794,-1.,-1.65625517961588));
#49947=CARTESIAN_POINT('Ctrl Pts',(-3.4996447647794,1.,-1.65625517961588));
#49948=CARTESIAN_POINT('Ctrl Pts',(-3.50702733146542,-1.,-1.65773832633632));
#49949=CARTESIAN_POINT('Ctrl Pts',(-3.50702733146542,1.,-1.65773832633632));
#49950=CARTESIAN_POINT('Ctrl Pts',(-3.5143763218894,-1.,-1.65913971687342));
#49951=CARTESIAN_POINT('Ctrl Pts',(-3.5143763218894,1.,-1.65913971687342));
#49952=CARTESIAN_POINT('Ctrl Pts',(-3.52170261543815,-1.,-1.66046645222279));
#49953=CARTESIAN_POINT('Ctrl Pts',(-3.52170261543815,1.,-1.66046645222279));
#49954=CARTESIAN_POINT('Ctrl Pts',(-3.52902746211093,-1.,-1.66173058912371));
#49955=CARTESIAN_POINT('Ctrl Pts',(-3.52902746211093,1.,-1.66173058912371));
#49956=CARTESIAN_POINT('Ctrl Pts',(-3.5363738506022,-1.,-1.66294490916111));
#49957=CARTESIAN_POINT('Ctrl Pts',(-3.5363738506022,1.,-1.66294490916111));
#49958=CARTESIAN_POINT('Ctrl Pts',(-3.54375747475014,-1.,-1.66411849222326));
#49959=CARTESIAN_POINT('Ctrl Pts',(-3.54375747475014,1.,-1.66411849222326));
#49960=CARTESIAN_POINT('Ctrl Pts',(-3.55118121342861,-1.,-1.66525401568994));
#49961=CARTESIAN_POINT('Ctrl Pts',(-3.55118121342861,1.,-1.66525401568994));
#49962=CARTESIAN_POINT('Ctrl Pts',(-3.55864015233602,-1.,-1.66635023293114));
#49963=CARTESIAN_POINT('Ctrl Pts',(-3.55864015233602,1.,-1.66635023293114));
#49964=CARTESIAN_POINT('Ctrl Pts',(-3.56612465179422,-1.,-1.66740349220305));
#49965=CARTESIAN_POINT('Ctrl Pts',(-3.56612465179422,1.,-1.66740349220305));
#49966=CARTESIAN_POINT('Ctrl Pts',(-3.57362406285887,-1.,-1.668409574073));
#49967=CARTESIAN_POINT('Ctrl Pts',(-3.57362406285887,1.,-1.668409574073));
#49968=CARTESIAN_POINT('Ctrl Pts',(-3.58113044183829,-1.,-1.66936552908232));
#49969=CARTESIAN_POINT('Ctrl Pts',(-3.58113044183829,1.,-1.66936552908232));
#49970=CARTESIAN_POINT('Ctrl Pts',(-3.58864143097834,-1.,-1.67027110397604));
#49971=CARTESIAN_POINT('Ctrl Pts',(-3.58864143097834,1.,-1.67027110397604));
#49972=CARTESIAN_POINT('Ctrl Pts',(-3.59615824388807,-1.,-1.67112775290707));
#49973=CARTESIAN_POINT('Ctrl Pts',(-3.59615824388807,1.,-1.67112775290707));
#49974=CARTESIAN_POINT('Ctrl Pts',(-3.603684308152,-1.,-1.67193797318597));
#49975=CARTESIAN_POINT('Ctrl Pts',(-3.603684308152,1.,-1.67193797318597));
#49976=CARTESIAN_POINT('Ctrl Pts',(-3.61122367156181,-1.,-1.67270452466968));
#49977=CARTESIAN_POINT('Ctrl Pts',(-3.61122367156181,1.,-1.67270452466968));
#49978=CARTESIAN_POINT('Ctrl Pts',(-3.61877947398184,-1.,-1.67342968196224));
#49979=CARTESIAN_POINT('Ctrl Pts',(-3.61877947398184,1.,-1.67342968196224));
#49980=CARTESIAN_POINT('Ctrl Pts',(-3.62635249450923,-1.,-1.67411452372271));
#49981=CARTESIAN_POINT('Ctrl Pts',(-3.62635249450923,1.,-1.67411452372271));
#49982=CARTESIAN_POINT('Ctrl Pts',(-3.63394189312924,-1.,-1.67475929882971));
#49983=CARTESIAN_POINT('Ctrl Pts',(-3.63394189312924,1.,-1.67475929882971));
#49984=CARTESIAN_POINT('Ctrl Pts',(-3.6415458297234,-1.,-1.67536373264848));
#49985=CARTESIAN_POINT('Ctrl Pts',(-3.6415458297234,1.,-1.67536373264848));
#49986=CARTESIAN_POINT('Ctrl Pts',(-3.64916213574667,-1.,-1.67592735946692));
#49987=CARTESIAN_POINT('Ctrl Pts',(-3.64916213574667,1.,-1.67592735946692));
#49988=CARTESIAN_POINT('Ctrl Pts',(-3.6567889441642,-1.,-1.67644983469449));
#49989=CARTESIAN_POINT('Ctrl Pts',(-3.6567889441642,1.,-1.67644983469449));
#49990=CARTESIAN_POINT('Ctrl Pts',(-3.66442538670968,-1.,-1.67693128053132));
#49991=CARTESIAN_POINT('Ctrl Pts',(-3.66442538670968,1.,-1.67693128053132));
#49992=CARTESIAN_POINT('Ctrl Pts',(-3.67207136294575,-1.,-1.67737217414874));
#49993=CARTESIAN_POINT('Ctrl Pts',(-3.67207136294575,1.,-1.67737217414874));
#49994=CARTESIAN_POINT('Ctrl Pts',(-3.67972724579124,-1.,-1.67777320475848));
#49995=CARTESIAN_POINT('Ctrl Pts',(-3.67972724579124,1.,-1.67777320475848));
#49996=CARTESIAN_POINT('Ctrl Pts',(-3.68739360236487,-1.,-1.67813513867965));
#49997=CARTESIAN_POINT('Ctrl Pts',(-3.68739360236487,1.,-1.67813513867965));
#49998=CARTESIAN_POINT('Ctrl Pts',(-3.6950709275959,-1.,-1.67845869064323));
#49999=CARTESIAN_POINT('Ctrl Pts',(-3.6950709275959,1.,-1.67845869064323));
#50000=CARTESIAN_POINT('Ctrl Pts',(-3.70275932351108,-1.,-1.67874436948667));
#50001=CARTESIAN_POINT('Ctrl Pts',(-3.70275932351108,1.,-1.67874436948667));
#50002=CARTESIAN_POINT('Ctrl Pts',(-3.71045854208343,-1.,-1.67899249793462));
#50003=CARTESIAN_POINT('Ctrl Pts',(-3.71045854208343,1.,-1.67899249793462));
#50004=CARTESIAN_POINT('Ctrl Pts',(-3.71816812842322,-1.,-1.67920328071708));
#50005=CARTESIAN_POINT('Ctrl Pts',(-3.71816812842322,1.,-1.67920328071708));
#50006=CARTESIAN_POINT('Ctrl Pts',(-3.72588753416396,-1.,-1.67937685856652));
#50007=CARTESIAN_POINT('Ctrl Pts',(-3.72588753416396,1.,-1.67937685856652));
#50008=CARTESIAN_POINT('Ctrl Pts',(-3.73361623282543,-1.,-1.67951336376402));
#50009=CARTESIAN_POINT('Ctrl Pts',(-3.73361623282543,1.,-1.67951336376402));
#50010=CARTESIAN_POINT('Ctrl Pts',(-3.74135385965401,-1.,-1.6796129868522));
#50011=CARTESIAN_POINT('Ctrl Pts',(-3.74135385965401,1.,-1.6796129868522));
#50012=CARTESIAN_POINT('Ctrl Pts',(-3.7491002239452,-1.,-1.67967598599525));
#50013=CARTESIAN_POINT('Ctrl Pts',(-3.7491002239452,1.,-1.67967598599525));
#50014=CARTESIAN_POINT('Ctrl Pts',(-3.75685523754493,-1.,-1.67970265841239));
#50015=CARTESIAN_POINT('Ctrl Pts',(-3.75685523754493,1.,-1.67970265841239));
#50016=CARTESIAN_POINT('Ctrl Pts',(-3.76461886684344,-1.,-1.67969332319245));
#50017=CARTESIAN_POINT('Ctrl Pts',(-3.76461886684344,1.,-1.67969332319245));
#50018=CARTESIAN_POINT('Ctrl Pts',(-3.77239107928502,-1.,-1.67964830084993));
#50019=CARTESIAN_POINT('Ctrl Pts',(-3.77239107928502,1.,-1.67964830084993));
#50020=CARTESIAN_POINT('Ctrl Pts',(-3.78017178197317,-1.,-1.67956789212141));
#50021=CARTESIAN_POINT('Ctrl Pts',(-3.78017178197317,1.,-1.67956789212141));
#50022=CARTESIAN_POINT('Ctrl Pts',(-3.7879608002176,-1.,-1.67945236653493));
#50023=CARTESIAN_POINT('Ctrl Pts',(-3.7879608002176,1.,-1.67945236653493));
#50024=CARTESIAN_POINT('Ctrl Pts',(-3.79575791578424,-1.,-1.67930196625548));
#50025=CARTESIAN_POINT('Ctrl Pts',(-3.79575791578424,1.,-1.67930196625548));
#50026=CARTESIAN_POINT('Ctrl Pts',(-3.80356289079005,-1.,-1.67911690648355));
#50027=CARTESIAN_POINT('Ctrl Pts',(-3.80356289079005,1.,-1.67911690648355));
#50028=CARTESIAN_POINT('Ctrl Pts',(-3.81137549624178,-1.,-1.6788973773827));
#50029=CARTESIAN_POINT('Ctrl Pts',(-3.81137549624178,1.,-1.6788973773827));
#50030=CARTESIAN_POINT('Ctrl Pts',(-3.81919554099578,-1.,-1.67864354605954));
#50031=CARTESIAN_POINT('Ctrl Pts',(-3.81919554099578,1.,-1.67864354605954));
#50032=CARTESIAN_POINT('Ctrl Pts',(-3.82702289286713,-1.,-1.6783555575934));
#50033=CARTESIAN_POINT('Ctrl Pts',(-3.82702289286713,1.,-1.6783555575934));
#50034=CARTESIAN_POINT('Ctrl Pts',(-3.83485746513989,-1.,-1.67803353064351));
#50035=CARTESIAN_POINT('Ctrl Pts',(-3.83485746513989,1.,-1.67803353064351));
#50036=CARTESIAN_POINT('Ctrl Pts',(-3.84113085985244,-1.,-1.67774874946079));
#50037=CARTESIAN_POINT('Ctrl Pts',(-3.84113085985244,1.,-1.67774874946079));
#50038=CARTESIAN_POINT('Ctrl Pts',(-3.84583912296459,-1.,-1.6775199114018));
#50039=CARTESIAN_POINT('Ctrl Pts',(-3.84583912296459,1.,-1.6775199114018));
#50040=CARTESIAN_POINT('Ctrl Pts',(-3.84897939430696,-1.,-1.67736057656533));
#50041=CARTESIAN_POINT('Ctrl Pts',(-3.84897939430696,1.,-1.67736057656533));
#50042=CARTESIAN_POINT('Ctrl Pts',(-3.85054988729471,-1.,-1.67727921511438));
#50043=CARTESIAN_POINT('Ctrl Pts',(-3.85054988729471,1.,-1.67727921511438));
#50044=CARTESIAN_POINT('',(-3.38171594275765,1.,-1.62064718014094));
#50045=CARTESIAN_POINT('Ctrl Pts',(-3.38171594275765,-1.,-1.62064718014094));
#50046=CARTESIAN_POINT('Ctrl Pts',(-3.38171594275765,-0.666666666666667,
-1.62064718014094));
#50047=CARTESIAN_POINT('Ctrl Pts',(-3.38171594275765,-0.333333333333333,
-1.62064718014094));
#50048=CARTESIAN_POINT('Ctrl Pts',(-3.38171594275765,0.333333333333333,
-1.62064718014094));
#50049=CARTESIAN_POINT('Ctrl Pts',(-3.38171594275765,0.666666666666667,
-1.62064718014094));
#50050=CARTESIAN_POINT('Ctrl Pts',(-3.38171594275765,1.,-1.62064718014094));
#50051=CARTESIAN_POINT('',(-3.85054988729471,1.,-1.67727921511438));
#50052=CARTESIAN_POINT('',(-3.85054988729471,0.,-1.67727921511438));
#50053=CARTESIAN_POINT('Ctrl Pts',(-3.38171594275765,1.,-1.62064718014094));
#50054=CARTESIAN_POINT('Ctrl Pts',(-3.38173802621259,1.,-1.62069086551492));
#50055=CARTESIAN_POINT('Ctrl Pts',(-3.38187506456922,1.,-1.62083271135947));
#50056=CARTESIAN_POINT('Ctrl Pts',(-3.38243080602409,1.,-1.62118047294498));
#50057=CARTESIAN_POINT('Ctrl Pts',(-3.38394285763222,1.,-1.62192472202769));
#50058=CARTESIAN_POINT('Ctrl Pts',(-3.38715832179072,1.,-1.6233278855625));
#50059=CARTESIAN_POINT('Ctrl Pts',(-3.39206617496906,1.,-1.62533996116713));
#50060=CARTESIAN_POINT('Ctrl Pts',(-3.39818605297991,1.,-1.62774916464408));
#50061=CARTESIAN_POINT('Ctrl Pts',(-3.40519422740235,1.,-1.63041148964828));
#50062=CARTESIAN_POINT('Ctrl Pts',(-3.41272817148478,1.,-1.63316667054044));
#50063=CARTESIAN_POINT('Ctrl Pts',(-3.42043974590882,1.,-1.63586250099773));
#50064=CARTESIAN_POINT('Ctrl Pts',(-3.42804772926291,1.,-1.63837876246926));
#50065=CARTESIAN_POINT('Ctrl Pts',(-3.43540451921548,1.,-1.64065778702023));
#50066=CARTESIAN_POINT('Ctrl Pts',(-3.44250337701888,1.,-1.64270733821113));
#50067=CARTESIAN_POINT('Ctrl Pts',(-3.44942242546795,1.,-1.64457408708107));
#50068=CARTESIAN_POINT('Ctrl Pts',(-3.45628421062422,1.,-1.64632429697521));
#50069=CARTESIAN_POINT('Ctrl Pts',(-3.46321237515,1.,-1.64802323352738));
#50070=CARTESIAN_POINT('Ctrl Pts',(-3.47028140995992,1.,-1.64971118698256));
#50071=CARTESIAN_POINT('Ctrl Pts',(-3.47749926256476,1.,-1.65139534930322));
#50072=CARTESIAN_POINT('Ctrl Pts',(-3.48483492840894,1.,-1.65306335367739));
#50073=CARTESIAN_POINT('Ctrl Pts',(-3.49223525300176,1.,-1.65469162644468));
#50074=CARTESIAN_POINT('Ctrl Pts',(-3.4996447647794,1.,-1.65625517961588));
#50075=CARTESIAN_POINT('Ctrl Pts',(-3.50702733146542,1.,-1.65773832633632));
#50076=CARTESIAN_POINT('Ctrl Pts',(-3.5143763218894,1.,-1.65913971687342));
#50077=CARTESIAN_POINT('Ctrl Pts',(-3.52170261543815,1.,-1.66046645222279));
#50078=CARTESIAN_POINT('Ctrl Pts',(-3.52902746211093,1.,-1.66173058912371));
#50079=CARTESIAN_POINT('Ctrl Pts',(-3.5363738506022,1.,-1.66294490916111));
#50080=CARTESIAN_POINT('Ctrl Pts',(-3.54375747475014,1.,-1.66411849222326));
#50081=CARTESIAN_POINT('Ctrl Pts',(-3.55118121342861,1.,-1.66525401568994));
#50082=CARTESIAN_POINT('Ctrl Pts',(-3.55864015233602,1.,-1.66635023293114));
#50083=CARTESIAN_POINT('Ctrl Pts',(-3.56612465179422,1.,-1.66740349220305));
#50084=CARTESIAN_POINT('Ctrl Pts',(-3.57362406285887,1.,-1.668409574073));
#50085=CARTESIAN_POINT('Ctrl Pts',(-3.58113044183829,1.,-1.66936552908232));
#50086=CARTESIAN_POINT('Ctrl Pts',(-3.58864143097834,1.,-1.67027110397604));
#50087=CARTESIAN_POINT('Ctrl Pts',(-3.59615824388807,1.,-1.67112775290707));
#50088=CARTESIAN_POINT('Ctrl Pts',(-3.603684308152,1.,-1.67193797318597));
#50089=CARTESIAN_POINT('Ctrl Pts',(-3.61122367156181,1.,-1.67270452466968));
#50090=CARTESIAN_POINT('Ctrl Pts',(-3.61877947398184,1.,-1.67342968196224));
#50091=CARTESIAN_POINT('Ctrl Pts',(-3.62635249450923,1.,-1.67411452372271));
#50092=CARTESIAN_POINT('Ctrl Pts',(-3.63394189312924,1.,-1.67475929882971));
#50093=CARTESIAN_POINT('Ctrl Pts',(-3.6415458297234,1.,-1.67536373264848));
#50094=CARTESIAN_POINT('Ctrl Pts',(-3.64916213574667,1.,-1.67592735946692));
#50095=CARTESIAN_POINT('Ctrl Pts',(-3.6567889441642,1.,-1.67644983469449));
#50096=CARTESIAN_POINT('Ctrl Pts',(-3.66442538670968,1.,-1.67693128053132));
#50097=CARTESIAN_POINT('Ctrl Pts',(-3.67207136294575,1.,-1.67737217414874));
#50098=CARTESIAN_POINT('Ctrl Pts',(-3.67972724579124,1.,-1.67777320475848));
#50099=CARTESIAN_POINT('Ctrl Pts',(-3.68739360236487,1.,-1.67813513867965));
#50100=CARTESIAN_POINT('Ctrl Pts',(-3.6950709275959,1.,-1.67845869064323));
#50101=CARTESIAN_POINT('Ctrl Pts',(-3.70275932351108,1.,-1.67874436948667));
#50102=CARTESIAN_POINT('Ctrl Pts',(-3.71045854208343,1.,-1.67899249793462));
#50103=CARTESIAN_POINT('Ctrl Pts',(-3.71816812842322,1.,-1.67920328071708));
#50104=CARTESIAN_POINT('Ctrl Pts',(-3.72588753416396,1.,-1.67937685856652));
#50105=CARTESIAN_POINT('Ctrl Pts',(-3.73361623282543,1.,-1.67951336376402));
#50106=CARTESIAN_POINT('Ctrl Pts',(-3.74135385965401,1.,-1.6796129868522));
#50107=CARTESIAN_POINT('Ctrl Pts',(-3.7491002239452,1.,-1.67967598599525));
#50108=CARTESIAN_POINT('Ctrl Pts',(-3.75685523754493,1.,-1.67970265841239));
#50109=CARTESIAN_POINT('Ctrl Pts',(-3.76461886684344,1.,-1.67969332319245));
#50110=CARTESIAN_POINT('Ctrl Pts',(-3.77239107928502,1.,-1.67964830084993));
#50111=CARTESIAN_POINT('Ctrl Pts',(-3.78017178197317,1.,-1.67956789212141));
#50112=CARTESIAN_POINT('Ctrl Pts',(-3.7879608002176,1.,-1.67945236653493));
#50113=CARTESIAN_POINT('Ctrl Pts',(-3.79575791578424,1.,-1.67930196625548));
#50114=CARTESIAN_POINT('Ctrl Pts',(-3.80356289079005,1.,-1.67911690648355));
#50115=CARTESIAN_POINT('Ctrl Pts',(-3.81137549624178,1.,-1.6788973773827));
#50116=CARTESIAN_POINT('Ctrl Pts',(-3.81919554099578,1.,-1.67864354605954));
#50117=CARTESIAN_POINT('Ctrl Pts',(-3.82702289286713,1.,-1.6783555575934));
#50118=CARTESIAN_POINT('Ctrl Pts',(-3.83485746513989,1.,-1.67803353064351));
#50119=CARTESIAN_POINT('Ctrl Pts',(-3.84113085985244,1.,-1.67774874946079));
#50120=CARTESIAN_POINT('Ctrl Pts',(-3.84583912296459,1.,-1.6775199114018));
#50121=CARTESIAN_POINT('Ctrl Pts',(-3.84897939430696,1.,-1.67736057656533));
#50122=CARTESIAN_POINT('Ctrl Pts',(-3.85054988729471,1.,-1.67727921511438));
#50123=CARTESIAN_POINT('Origin',(-3.85054988729471,0.,-1.67727921511438));
#50124=CARTESIAN_POINT('',(-3.90876544355381,1.,-1.53673442965256));
#50125=CARTESIAN_POINT('Origin',(0.,0.,0.));
#50126=CARTESIAN_POINT('',(-3.29885386921599,1.,-1.78327315618183));
#50127=CARTESIAN_POINT('Origin',(0.,1.,0.));
#50128=CARTESIAN_POINT('Ctrl Pts',(-3.29885386921599,1.,-1.78327315618183));
#50129=CARTESIAN_POINT('Ctrl Pts',(-3.29885386921599,0.666666666666667,
-1.78327315618183));
#50130=CARTESIAN_POINT('Ctrl Pts',(-3.29885386921599,0.333333333333333,
-1.78327315618183));
#50131=CARTESIAN_POINT('Ctrl Pts',(-3.29885386921599,-0.333333333333333,
-1.78327315618183));
#50132=CARTESIAN_POINT('Ctrl Pts',(-3.29885386921599,-0.666666666666667,
-1.78327315618183));
#50133=CARTESIAN_POINT('Ctrl Pts',(-3.29885386921599,-1.,-1.78327315618183));
#50134=CARTESIAN_POINT('Ctrl Pts',(-3.62024382630768,-1.,-2.12928030988903));
#50135=CARTESIAN_POINT('Ctrl Pts',(-3.62024382630768,1.,-2.12928030988903));
#50136=CARTESIAN_POINT('Ctrl Pts',(-3.61938653649098,-1.,-2.12796193131368));
#50137=CARTESIAN_POINT('Ctrl Pts',(-3.61938653649098,1.,-2.12796193131368));
#50138=CARTESIAN_POINT('Ctrl Pts',(-3.61766963590482,-1.,-2.12532774376758));
#50139=CARTESIAN_POINT('Ctrl Pts',(-3.61766963590482,1.,-2.12532774376758));
#50140=CARTESIAN_POINT('Ctrl Pts',(-3.61508732216891,-1.,-2.12138417126355));
#50141=CARTESIAN_POINT('Ctrl Pts',(-3.61508732216891,1.,-2.12138417126355));
#50142=CARTESIAN_POINT('Ctrl Pts',(-3.61163030609447,-1.,-2.11614149815106));
#50143=CARTESIAN_POINT('Ctrl Pts',(-3.61163030609447,1.,-2.11614149815106));
#50144=CARTESIAN_POINT('Ctrl Pts',(-3.60728578532601,-1.,-2.10961391334462));
#50145=CARTESIAN_POINT('Ctrl Pts',(-3.60728578532601,1.,-2.10961391334462));
#50146=CARTESIAN_POINT('Ctrl Pts',(-3.60291797088734,-1.,-2.1031121772821));
#50147=CARTESIAN_POINT('Ctrl Pts',(-3.60291797088734,1.,-2.1031121772821));
#50148=CARTESIAN_POINT('Ctrl Pts',(-3.59852681775485,-1.,-2.09663642986631));
#50149=CARTESIAN_POINT('Ctrl Pts',(-3.59852681775485,1.,-2.09663642986631));
#50150=CARTESIAN_POINT('Ctrl Pts',(-3.59411228625588,-1.,-2.09018686331416));
#50151=CARTESIAN_POINT('Ctrl Pts',(-3.59411228625588,1.,-2.09018686331416));
#50152=CARTESIAN_POINT('Ctrl Pts',(-3.58967435355088,-1.,-2.08376373048756));
#50153=CARTESIAN_POINT('Ctrl Pts',(-3.58967435355088,1.,-2.08376373048756));
#50154=CARTESIAN_POINT('Ctrl Pts',(-3.58521300039299,-1.,-2.07736732842117));
#50155=CARTESIAN_POINT('Ctrl Pts',(-3.58521300039299,1.,-2.07736732842117));
#50156=CARTESIAN_POINT('Ctrl Pts',(-3.58072819250442,-1.,-2.07099797605747));
#50157=CARTESIAN_POINT('Ctrl Pts',(-3.58072819250442,1.,-2.07099797605747));
#50158=CARTESIAN_POINT('Ctrl Pts',(-3.576219862243,-1.,-2.06465599229174));
#50159=CARTESIAN_POINT('Ctrl Pts',(-3.576219862243,1.,-2.06465599229174));
#50160=CARTESIAN_POINT('Ctrl Pts',(-3.57168789423507,-1.,-2.05834167687523));
#50161=CARTESIAN_POINT('Ctrl Pts',(-3.57168789423507,1.,-2.05834167687523));
#50162=CARTESIAN_POINT('Ctrl Pts',(-3.56713209978207,-1.,-2.0520552817309));
#50163=CARTESIAN_POINT('Ctrl Pts',(-3.56713209978207,1.,-2.0520552817309));
#50164=CARTESIAN_POINT('Ctrl Pts',(-3.5625522387181,-1.,-2.04579702159056));
#50165=CARTESIAN_POINT('Ctrl Pts',(-3.5625522387181,1.,-2.04579702159056));
#50166=CARTESIAN_POINT('Ctrl Pts',(-3.55794807265052,-1.,-2.03956711120099));
#50167=CARTESIAN_POINT('Ctrl Pts',(-3.55794807265052,1.,-2.03956711120099));
#50168=CARTESIAN_POINT('Ctrl Pts',(-3.55331941294018,-1.,-2.03336579658174));
#50169=CARTESIAN_POINT('Ctrl Pts',(-3.55331941294018,1.,-2.03336579658174));
#50170=CARTESIAN_POINT('Ctrl Pts',(-3.54866616282173,-1.,-2.02719338376144));
#50171=CARTESIAN_POINT('Ctrl Pts',(-3.54866616282173,1.,-2.02719338376144));
#50172=CARTESIAN_POINT('Ctrl Pts',(-3.54398838254011,-1.,-2.0210502798303));
#50173=CARTESIAN_POINT('Ctrl Pts',(-3.54398838254011,1.,-2.0210502798303));
#50174=CARTESIAN_POINT('Ctrl Pts',(-3.53928627453503,-1.,-2.0149369884727));
#50175=CARTESIAN_POINT('Ctrl Pts',(-3.53928627453503,1.,-2.0149369884727));
#50176=CARTESIAN_POINT('Ctrl Pts',(-3.53456004727321,-1.,-2.00885403604685));
#50177=CARTESIAN_POINT('Ctrl Pts',(-3.53456004727321,1.,-2.00885403604685));
#50178=CARTESIAN_POINT('Ctrl Pts',(-3.52980980250181,-1.,-2.00280191090341));
#50179=CARTESIAN_POINT('Ctrl Pts',(-3.52980980250181,1.,-2.00280191090341));
#50180=CARTESIAN_POINT('Ctrl Pts',(-3.52503542491745,-1.,-1.99678100339305));
#50181=CARTESIAN_POINT('Ctrl Pts',(-3.52503542491745,1.,-1.99678100339305));
#50182=CARTESIAN_POINT('Ctrl Pts',(-3.52023644289195,-1.,-1.99079153006143));
#50183=CARTESIAN_POINT('Ctrl Pts',(-3.52023644289195,1.,-1.99079153006143));
#50184=CARTESIAN_POINT('Ctrl Pts',(-3.51541198728362,-1.,-1.98483351061066));
#50185=CARTESIAN_POINT('Ctrl Pts',(-3.51541198728362,1.,-1.98483351061066));
#50186=CARTESIAN_POINT('Ctrl Pts',(-3.51056110478334,-1.,-1.97890693666316));
#50187=CARTESIAN_POINT('Ctrl Pts',(-3.51056110478334,1.,-1.97890693666316));
#50188=CARTESIAN_POINT('Ctrl Pts',(-3.505683018611,-1.,-1.9730119116298));
#50189=CARTESIAN_POINT('Ctrl Pts',(-3.505683018611,1.,-1.9730119116298));
#50190=CARTESIAN_POINT('Ctrl Pts',(-3.50077740176262,-1.,-1.9671487972405));
#50191=CARTESIAN_POINT('Ctrl Pts',(-3.50077740176262,1.,-1.9671487972405));
#50192=CARTESIAN_POINT('Ctrl Pts',(-3.49584466573045,-1.,-1.96131836776489));
#50193=CARTESIAN_POINT('Ctrl Pts',(-3.49584466573045,1.,-1.96131836776489));
#50194=CARTESIAN_POINT('Ctrl Pts',(-3.49088618670967,-1.,-1.95552193112071));
#50195=CARTESIAN_POINT('Ctrl Pts',(-3.49088618670967,1.,-1.95552193112071));
#50196=CARTESIAN_POINT('Ctrl Pts',(-3.485903616108,-1.,-1.94976096795902));
#50197=CARTESIAN_POINT('Ctrl Pts',(-3.485903616108,1.,-1.94976096795902));
#50198=CARTESIAN_POINT('Ctrl Pts',(-3.48089825770411,-1.,-1.94403680554062));
#50199=CARTESIAN_POINT('Ctrl Pts',(-3.48089825770411,1.,-1.94403680554062));
#50200=CARTESIAN_POINT('Ctrl Pts',(-3.47587040389916,-1.,-1.93835026973888));
#50201=CARTESIAN_POINT('Ctrl Pts',(-3.47587040389916,1.,-1.93835026973888));
#50202=CARTESIAN_POINT('Ctrl Pts',(-3.47081872409783,-1.,-1.93270136427083));
#50203=CARTESIAN_POINT('Ctrl Pts',(-3.47081872409783,1.,-1.93270136427083));
#50204=CARTESIAN_POINT('Ctrl Pts',(-3.46573953254084,-1.,-1.92708888591159));
#50205=CARTESIAN_POINT('Ctrl Pts',(-3.46573953254084,1.,-1.92708888591159));
#50206=CARTESIAN_POINT('Ctrl Pts',(-3.4606282172248,-1.,-1.9215111821321));
#50207=CARTESIAN_POINT('Ctrl Pts',(-3.4606282172248,1.,-1.9215111821321));
#50208=CARTESIAN_POINT('Ctrl Pts',(-3.45548074309943,-1.,-1.9159669478406));
#50209=CARTESIAN_POINT('Ctrl Pts',(-3.45548074309943,1.,-1.9159669478406));
#50210=CARTESIAN_POINT('Ctrl Pts',(-3.45029522038885,-1.,-1.91045605593638));
#50211=CARTESIAN_POINT('Ctrl Pts',(-3.45029522038885,1.,-1.91045605593638));
#50212=CARTESIAN_POINT('Ctrl Pts',(-3.44507323983374,-1.,-1.90498026502308));
#50213=CARTESIAN_POINT('Ctrl Pts',(-3.44507323983374,1.,-1.90498026502308));
#50214=CARTESIAN_POINT('Ctrl Pts',(-3.43982185678105,-1.,-1.89954426803392));
#50215=CARTESIAN_POINT('Ctrl Pts',(-3.43982185678105,1.,-1.89954426803392));
#50216=CARTESIAN_POINT('Ctrl Pts',(-3.43455074411591,-1.,-1.89415420002553));
#50217=CARTESIAN_POINT('Ctrl Pts',(-3.43455074411591,1.,-1.89415420002553));
#50218=CARTESIAN_POINT('Ctrl Pts',(-3.42926852222174,-1.,-1.88881571322018));
#50219=CARTESIAN_POINT('Ctrl Pts',(-3.42926852222174,1.,-1.88881571322018));
#50220=CARTESIAN_POINT('Ctrl Pts',(-3.42397908819741,-1.,-1.88353205062063));
#50221=CARTESIAN_POINT('Ctrl Pts',(-3.42397908819741,1.,-1.88353205062063));
#50222=CARTESIAN_POINT('Ctrl Pts',(-3.4186785838376,-1.,-1.87830245689338));
#50223=CARTESIAN_POINT('Ctrl Pts',(-3.4186785838376,1.,-1.87830245689338));
#50224=CARTESIAN_POINT('Ctrl Pts',(-3.41335043875182,-1.,-1.87311957248106));
#50225=CARTESIAN_POINT('Ctrl Pts',(-3.41335043875182,1.,-1.87311957248106));
#50226=CARTESIAN_POINT('Ctrl Pts',(-3.40797080000513,-1.,-1.86797231196635));
#50227=CARTESIAN_POINT('Ctrl Pts',(-3.40797080000513,1.,-1.86797231196635));
#50228=CARTESIAN_POINT('Ctrl Pts',(-3.40251742305445,-1.,-1.86285057051228));
#50229=CARTESIAN_POINT('Ctrl Pts',(-3.40251742305445,1.,-1.86285057051228));
#50230=CARTESIAN_POINT('Ctrl Pts',(-3.39697816833056,-1.,-1.85774972037055));
#50231=CARTESIAN_POINT('Ctrl Pts',(-3.39697816833056,1.,-1.85774972037055));
#50232=CARTESIAN_POINT('Ctrl Pts',(-3.39135802549415,-1.,-1.85267433291778));
#50233=CARTESIAN_POINT('Ctrl Pts',(-3.39135802549415,1.,-1.85267433291778));
#50234=CARTESIAN_POINT('Ctrl Pts',(-3.38569092349639,-1.,-1.84764441927778));
#50235=CARTESIAN_POINT('Ctrl Pts',(-3.38569092349639,1.,-1.84764441927778));
#50236=CARTESIAN_POINT('Ctrl Pts',(-3.38002968341222,-1.,-1.84269016931679));
#50237=CARTESIAN_POINT('Ctrl Pts',(-3.38002968341222,1.,-1.84269016931679));
#50238=CARTESIAN_POINT('Ctrl Pts',(-3.37442462015914,-1.,-1.83784072967111));
#50239=CARTESIAN_POINT('Ctrl Pts',(-3.37442462015914,1.,-1.83784072967111));
#50240=CARTESIAN_POINT('Ctrl Pts',(-3.36890396271864,-1.,-1.83311391452338));
#50241=CARTESIAN_POINT('Ctrl Pts',(-3.36890396271864,1.,-1.83311391452338));
#50242=CARTESIAN_POINT('Ctrl Pts',(-3.36345722124127,-1.,-1.82850752153182));
#50243=CARTESIAN_POINT('Ctrl Pts',(-3.36345722124127,1.,-1.82850752153182));
#50244=CARTESIAN_POINT('Ctrl Pts',(-3.35800801557326,-1.,-1.82398496829247));
#50245=CARTESIAN_POINT('Ctrl Pts',(-3.35800801557326,1.,-1.82398496829247));
#50246=CARTESIAN_POINT('Ctrl Pts',(-3.35243086937451,-1.,-1.81948458796748));
#50247=CARTESIAN_POINT('Ctrl Pts',(-3.35243086937451,1.,-1.81948458796748));
#50248=CARTESIAN_POINT('Ctrl Pts',(-3.34660014370527,-1.,-1.81494618732772));
#50249=CARTESIAN_POINT('Ctrl Pts',(-3.34660014370527,1.,-1.81494618732772));
#50250=CARTESIAN_POINT('Ctrl Pts',(-3.34043216147532,-1.,-1.81033399625311));
#50251=CARTESIAN_POINT('Ctrl Pts',(-3.34043216147532,1.,-1.81033399625311));
#50252=CARTESIAN_POINT('Ctrl Pts',(-3.33392460276874,-1.,-1.80565802981138));
#50253=CARTESIAN_POINT('Ctrl Pts',(-3.33392460276874,1.,-1.80565802981138));
#50254=CARTESIAN_POINT('Ctrl Pts',(-3.3272108803981,-1.,-1.80100380443535));
#50255=CARTESIAN_POINT('Ctrl Pts',(-3.3272108803981,1.,-1.80100380443535));
#50256=CARTESIAN_POINT('Ctrl Pts',(-3.32055355101168,-1.,-1.79652817033444));
#50257=CARTESIAN_POINT('Ctrl Pts',(-3.32055355101168,1.,-1.79652817033444));
#50258=CARTESIAN_POINT('Ctrl Pts',(-3.31428038326763,-1.,-1.79242331350137));
#50259=CARTESIAN_POINT('Ctrl Pts',(-3.31428038326763,1.,-1.79242331350137));
#50260=CARTESIAN_POINT('Ctrl Pts',(-3.30873412266954,-1.,-1.78888832245965));
#50261=CARTESIAN_POINT('Ctrl Pts',(-3.30873412266954,1.,-1.78888832245965));
#50262=CARTESIAN_POINT('Ctrl Pts',(-3.30422155558973,-1.,-1.78610045419769));
#50263=CARTESIAN_POINT('Ctrl Pts',(-3.30422155558973,1.,-1.78610045419769));
#50264=CARTESIAN_POINT('Ctrl Pts',(-3.30095096463082,-1.,-1.78417972819696));
#50265=CARTESIAN_POINT('Ctrl Pts',(-3.30095096463082,1.,-1.78417972819696));
#50266=CARTESIAN_POINT('Ctrl Pts',(-3.29940631673818,-1.,-1.78338186555671));
#50267=CARTESIAN_POINT('Ctrl Pts',(-3.29940631673818,1.,-1.78338186555671));
#50268=CARTESIAN_POINT('Ctrl Pts',(-3.29886572077303,-1.,-1.78320756177191));
#50269=CARTESIAN_POINT('Ctrl Pts',(-3.29886572077303,1.,-1.78320756177191));
#50270=CARTESIAN_POINT('Ctrl Pts',(-3.29877974053191,-1.,-1.78327971836272));
#50271=CARTESIAN_POINT('Ctrl Pts',(-3.29877974053191,1.,-1.78327971836272));
#50272=CARTESIAN_POINT('Ctrl Pts',(-3.2988053601491,-1.,-1.7833628895577));
#50273=CARTESIAN_POINT('Ctrl Pts',(-3.2988053601491,1.,-1.7833628895577));
#50274=CARTESIAN_POINT('',(-3.62024382630768,1.,-2.12928030988903));
#50275=CARTESIAN_POINT('Ctrl Pts',(-3.62024382630768,1.,-2.12928030988903));
#50276=CARTESIAN_POINT('Ctrl Pts',(-3.61938653649098,1.,-2.12796193131368));
#50277=CARTESIAN_POINT('Ctrl Pts',(-3.61766963590482,1.,-2.12532774376758));
#50278=CARTESIAN_POINT('Ctrl Pts',(-3.61508732216891,1.,-2.12138417126355));
#50279=CARTESIAN_POINT('Ctrl Pts',(-3.61163030609447,1.,-2.11614149815106));
#50280=CARTESIAN_POINT('Ctrl Pts',(-3.60728578532601,1.,-2.10961391334462));
#50281=CARTESIAN_POINT('Ctrl Pts',(-3.60291797088734,1.,-2.1031121772821));
#50282=CARTESIAN_POINT('Ctrl Pts',(-3.59852681775485,1.,-2.09663642986631));
#50283=CARTESIAN_POINT('Ctrl Pts',(-3.59411228625588,1.,-2.09018686331416));
#50284=CARTESIAN_POINT('Ctrl Pts',(-3.58967435355088,1.,-2.08376373048756));
#50285=CARTESIAN_POINT('Ctrl Pts',(-3.58521300039299,1.,-2.07736732842117));
#50286=CARTESIAN_POINT('Ctrl Pts',(-3.58072819250442,1.,-2.07099797605747));
#50287=CARTESIAN_POINT('Ctrl Pts',(-3.576219862243,1.,-2.06465599229174));
#50288=CARTESIAN_POINT('Ctrl Pts',(-3.57168789423507,1.,-2.05834167687523));
#50289=CARTESIAN_POINT('Ctrl Pts',(-3.56713209978207,1.,-2.0520552817309));
#50290=CARTESIAN_POINT('Ctrl Pts',(-3.5625522387181,1.,-2.04579702159056));
#50291=CARTESIAN_POINT('Ctrl Pts',(-3.55794807265052,1.,-2.03956711120099));
#50292=CARTESIAN_POINT('Ctrl Pts',(-3.55331941294018,1.,-2.03336579658174));
#50293=CARTESIAN_POINT('Ctrl Pts',(-3.54866616282173,1.,-2.02719338376144));
#50294=CARTESIAN_POINT('Ctrl Pts',(-3.54398838254011,1.,-2.0210502798303));
#50295=CARTESIAN_POINT('Ctrl Pts',(-3.53928627453503,1.,-2.0149369884727));
#50296=CARTESIAN_POINT('Ctrl Pts',(-3.53456004727321,1.,-2.00885403604685));
#50297=CARTESIAN_POINT('Ctrl Pts',(-3.52980980250181,1.,-2.00280191090341));
#50298=CARTESIAN_POINT('Ctrl Pts',(-3.52503542491745,1.,-1.99678100339305));
#50299=CARTESIAN_POINT('Ctrl Pts',(-3.52023644289195,1.,-1.99079153006143));
#50300=CARTESIAN_POINT('Ctrl Pts',(-3.51541198728362,1.,-1.98483351061066));
#50301=CARTESIAN_POINT('Ctrl Pts',(-3.51056110478334,1.,-1.97890693666316));
#50302=CARTESIAN_POINT('Ctrl Pts',(-3.505683018611,1.,-1.9730119116298));
#50303=CARTESIAN_POINT('Ctrl Pts',(-3.50077740176262,1.,-1.9671487972405));
#50304=CARTESIAN_POINT('Ctrl Pts',(-3.49584466573045,1.,-1.96131836776489));
#50305=CARTESIAN_POINT('Ctrl Pts',(-3.49088618670967,1.,-1.95552193112071));
#50306=CARTESIAN_POINT('Ctrl Pts',(-3.485903616108,1.,-1.94976096795902));
#50307=CARTESIAN_POINT('Ctrl Pts',(-3.48089825770411,1.,-1.94403680554062));
#50308=CARTESIAN_POINT('Ctrl Pts',(-3.47587040389916,1.,-1.93835026973888));
#50309=CARTESIAN_POINT('Ctrl Pts',(-3.47081872409783,1.,-1.93270136427083));
#50310=CARTESIAN_POINT('Ctrl Pts',(-3.46573953254084,1.,-1.92708888591159));
#50311=CARTESIAN_POINT('Ctrl Pts',(-3.4606282172248,1.,-1.9215111821321));
#50312=CARTESIAN_POINT('Ctrl Pts',(-3.45548074309943,1.,-1.9159669478406));
#50313=CARTESIAN_POINT('Ctrl Pts',(-3.45029522038885,1.,-1.91045605593638));
#50314=CARTESIAN_POINT('Ctrl Pts',(-3.44507323983374,1.,-1.90498026502308));
#50315=CARTESIAN_POINT('Ctrl Pts',(-3.43982185678105,1.,-1.89954426803392));
#50316=CARTESIAN_POINT('Ctrl Pts',(-3.43455074411591,1.,-1.89415420002553));
#50317=CARTESIAN_POINT('Ctrl Pts',(-3.42926852222174,1.,-1.88881571322018));
#50318=CARTESIAN_POINT('Ctrl Pts',(-3.42397908819741,1.,-1.88353205062063));
#50319=CARTESIAN_POINT('Ctrl Pts',(-3.4186785838376,1.,-1.87830245689338));
#50320=CARTESIAN_POINT('Ctrl Pts',(-3.41335043875182,1.,-1.87311957248106));
#50321=CARTESIAN_POINT('Ctrl Pts',(-3.40797080000513,1.,-1.86797231196635));
#50322=CARTESIAN_POINT('Ctrl Pts',(-3.40251742305445,1.,-1.86285057051228));
#50323=CARTESIAN_POINT('Ctrl Pts',(-3.39697816833056,1.,-1.85774972037055));
#50324=CARTESIAN_POINT('Ctrl Pts',(-3.39135802549415,1.,-1.85267433291778));
#50325=CARTESIAN_POINT('Ctrl Pts',(-3.38569092349639,1.,-1.84764441927778));
#50326=CARTESIAN_POINT('Ctrl Pts',(-3.38002968341222,1.,-1.84269016931679));
#50327=CARTESIAN_POINT('Ctrl Pts',(-3.37442462015914,1.,-1.83784072967111));
#50328=CARTESIAN_POINT('Ctrl Pts',(-3.36890396271864,1.,-1.83311391452338));
#50329=CARTESIAN_POINT('Ctrl Pts',(-3.36345722124127,1.,-1.82850752153182));
#50330=CARTESIAN_POINT('Ctrl Pts',(-3.35800801557326,1.,-1.82398496829247));
#50331=CARTESIAN_POINT('Ctrl Pts',(-3.35243086937451,1.,-1.81948458796748));
#50332=CARTESIAN_POINT('Ctrl Pts',(-3.34660014370527,1.,-1.81494618732772));
#50333=CARTESIAN_POINT('Ctrl Pts',(-3.34043216147532,1.,-1.81033399625311));
#50334=CARTESIAN_POINT('Ctrl Pts',(-3.33392460276874,1.,-1.80565802981138));
#50335=CARTESIAN_POINT('Ctrl Pts',(-3.3272108803981,1.,-1.80100380443535));
#50336=CARTESIAN_POINT('Ctrl Pts',(-3.32055355101168,1.,-1.79652817033444));
#50337=CARTESIAN_POINT('Ctrl Pts',(-3.31428038326763,1.,-1.79242331350137));
#50338=CARTESIAN_POINT('Ctrl Pts',(-3.30873412266954,1.,-1.78888832245965));
#50339=CARTESIAN_POINT('Ctrl Pts',(-3.30422155558973,1.,-1.78610045419769));
#50340=CARTESIAN_POINT('Ctrl Pts',(-3.30119637003466,1.,-1.7843238478823));
#50341=CARTESIAN_POINT('Ctrl Pts',(-3.29970549824336,1.,-1.78353803106983));
#50342=CARTESIAN_POINT('Ctrl Pts',(-3.29909749657945,1.,-1.78329283591903));
#50343=CARTESIAN_POINT('Ctrl Pts',(-3.29890219175522,1.,-1.78326534445426));
#50344=CARTESIAN_POINT('Ctrl Pts',(-3.29885386921599,1.,-1.78327315618183));
#50345=CARTESIAN_POINT('',(-3.62024382630768,0.,-2.12928030988903));
#50346=CARTESIAN_POINT('Ctrl Pts',(-3.08661426358891,-1.,-2.12962728847315));
#50347=CARTESIAN_POINT('Ctrl Pts',(-3.08661426358891,1.,-2.12962728847315));
#50348=CARTESIAN_POINT('Ctrl Pts',(-3.08652852644995,-1.,-2.12964222016025));
#50349=CARTESIAN_POINT('Ctrl Pts',(-3.08652852644995,1.,-2.12964222016025));
#50350=CARTESIAN_POINT('Ctrl Pts',(-3.08650326867133,-1.,-2.12975158752407));
#50351=CARTESIAN_POINT('Ctrl Pts',(-3.08650326867133,1.,-2.12975158752407));
#50352=CARTESIAN_POINT('Ctrl Pts',(-3.08690399991463,-1.,-2.1301541297946));
#50353=CARTESIAN_POINT('Ctrl Pts',(-3.08690399991463,1.,-2.1301541297946));
#50354=CARTESIAN_POINT('Ctrl Pts',(-3.08831615620074,-1.,-2.13116819908542));
#50355=CARTESIAN_POINT('Ctrl Pts',(-3.08831615620074,1.,-2.13116819908542));
#50356=CARTESIAN_POINT('Ctrl Pts',(-3.09151235281963,-1.,-2.13321032560893));
#50357=CARTESIAN_POINT('Ctrl Pts',(-3.09151235281963,1.,-2.13321032560893));
#50358=CARTESIAN_POINT('Ctrl Pts',(-3.0960450242104,-1.,-2.13596538661048));
#50359=CARTESIAN_POINT('Ctrl Pts',(-3.0960450242104,1.,-2.13596538661048));
#50360=CARTESIAN_POINT('Ctrl Pts',(-3.10171267391049,-1.,-2.13930228863751));
#50361=CARTESIAN_POINT('Ctrl Pts',(-3.10171267391049,1.,-2.13930228863751));
#50362=CARTESIAN_POINT('Ctrl Pts',(-3.10821808668859,-1.,-2.14302815601973));
#50363=CARTESIAN_POINT('Ctrl Pts',(-3.10821808668859,1.,-2.14302815601973));
#50364=CARTESIAN_POINT('Ctrl Pts',(-3.11522827016855,-1.,-2.14692798457532));
#50365=CARTESIAN_POINT('Ctrl Pts',(-3.11522827016855,1.,-2.14692798457532));
#50366=CARTESIAN_POINT('Ctrl Pts',(-3.12242318151938,-1.,-2.15079698090585));
#50367=CARTESIAN_POINT('Ctrl Pts',(-3.12242318151938,1.,-2.15079698090585));
#50368=CARTESIAN_POINT('Ctrl Pts',(-3.12954386795646,-1.,-2.1544724138292));
#50369=CARTESIAN_POINT('Ctrl Pts',(-3.12954386795646,1.,-2.1544724138292));
#50370=CARTESIAN_POINT('Ctrl Pts',(-3.13645356563038,-1.,-2.15787423530676));
#50371=CARTESIAN_POINT('Ctrl Pts',(-3.13645356563038,1.,-2.15787423530676));
#50372=CARTESIAN_POINT('Ctrl Pts',(-3.14314440427022,-1.,-2.16100905914435));
#50373=CARTESIAN_POINT('Ctrl Pts',(-3.14314440427022,1.,-2.16100905914435));
#50374=CARTESIAN_POINT('Ctrl Pts',(-3.14968624389054,-1.,-2.16393520288072));
#50375=CARTESIAN_POINT('Ctrl Pts',(-3.14968624389054,1.,-2.16393520288072));
#50376=CARTESIAN_POINT('Ctrl Pts',(-3.15618975593656,-1.,-2.1667372844769));
#50377=CARTESIAN_POINT('Ctrl Pts',(-3.15618975593656,1.,-2.1667372844769));
#50378=CARTESIAN_POINT('Ctrl Pts',(-3.16276685102972,-1.,-2.16949910801219));
#50379=CARTESIAN_POINT('Ctrl Pts',(-3.16276685102972,1.,-2.16949910801219));
#50380=CARTESIAN_POINT('Ctrl Pts',(-3.16948480019497,-1.,-2.17227212063817));
#50381=CARTESIAN_POINT('Ctrl Pts',(-3.16948480019497,1.,-2.17227212063817));
#50382=CARTESIAN_POINT('Ctrl Pts',(-3.17635032802523,-1.,-2.17506466903694));
#50383=CARTESIAN_POINT('Ctrl Pts',(-3.17635032802523,1.,-2.17506466903694));
#50384=CARTESIAN_POINT('Ctrl Pts',(-3.18333474627807,-1.,-2.17785968847142));
#50385=CARTESIAN_POINT('Ctrl Pts',(-3.18333474627807,1.,-2.17785968847142));
#50386=CARTESIAN_POINT('Ctrl Pts',(-3.19038924261573,-1.,-2.18062558031778));
#50387=CARTESIAN_POINT('Ctrl Pts',(-3.19038924261573,1.,-2.18062558031778));
#50388=CARTESIAN_POINT('Ctrl Pts',(-3.19746293740411,-1.,-2.18332898656602));
#50389=CARTESIAN_POINT('Ctrl Pts',(-3.19746293740411,1.,-2.18332898656602));
#50390=CARTESIAN_POINT('Ctrl Pts',(-3.20452259717976,-1.,-2.18594876115934));
#50391=CARTESIAN_POINT('Ctrl Pts',(-3.20452259717976,1.,-2.18594876115934));
#50392=CARTESIAN_POINT('Ctrl Pts',(-3.21156188355769,-1.,-2.18848253363901));
#50393=CARTESIAN_POINT('Ctrl Pts',(-3.21156188355769,1.,-2.18848253363901));
#50394=CARTESIAN_POINT('Ctrl Pts',(-3.21859043114095,-1.,-2.19093901948667));
#50395=CARTESIAN_POINT('Ctrl Pts',(-3.21859043114095,1.,-2.19093901948667));
#50396=CARTESIAN_POINT('Ctrl Pts',(-3.22562734221646,-1.,-2.19333345123538));
#50397=CARTESIAN_POINT('Ctrl Pts',(-3.22562734221646,1.,-2.19333345123538));
#50398=CARTESIAN_POINT('Ctrl Pts',(-3.23269332296933,-1.,-2.19568204933168));
#50399=CARTESIAN_POINT('Ctrl Pts',(-3.23269332296933,1.,-2.19568204933168));
#50400=CARTESIAN_POINT('Ctrl Pts',(-3.23980245361308,-1.,-2.19799623693253));
#50401=CARTESIAN_POINT('Ctrl Pts',(-3.23980245361308,1.,-2.19799623693253));
#50402=CARTESIAN_POINT('Ctrl Pts',(-3.24695715874338,-1.,-2.20027910880981));
#50403=CARTESIAN_POINT('Ctrl Pts',(-3.24695715874338,1.,-2.20027910880981));
#50404=CARTESIAN_POINT('Ctrl Pts',(-3.25415277957775,-1.,-2.20252866491545));
#50405=CARTESIAN_POINT('Ctrl Pts',(-3.25415277957775,1.,-2.20252866491545));
#50406=CARTESIAN_POINT('Ctrl Pts',(-3.26138036637705,-1.,-2.20473979048678));
#50407=CARTESIAN_POINT('Ctrl Pts',(-3.26138036637705,1.,-2.20473979048678));
#50408=CARTESIAN_POINT('Ctrl Pts',(-3.26863006136782,-1.,-2.20690665217743));
#50409=CARTESIAN_POINT('Ctrl Pts',(-3.26863006136782,1.,-2.20690665217743));
#50410=CARTESIAN_POINT('Ctrl Pts',(-3.2758944800554,-1.,-2.2090250941743));
#50411=CARTESIAN_POINT('Ctrl Pts',(-3.2758944800554,1.,-2.2090250941743));
#50412=CARTESIAN_POINT('Ctrl Pts',(-3.28317133333131,-1.,-2.21109449750641));
#50413=CARTESIAN_POINT('Ctrl Pts',(-3.28317133333131,1.,-2.21109449750641));
#50414=CARTESIAN_POINT('Ctrl Pts',(-3.29046159238343,-1.,-2.21311648827391));
#50415=CARTESIAN_POINT('Ctrl Pts',(-3.29046159238343,1.,-2.21311648827391));
#50416=CARTESIAN_POINT('Ctrl Pts',(-3.29776825193159,-1.,-2.21509406923368));
#50417=CARTESIAN_POINT('Ctrl Pts',(-3.29776825193159,1.,-2.21509406923368));
#50418=CARTESIAN_POINT('Ctrl Pts',(-3.30509487819569,-1.,-2.21703059947836));
#50419=CARTESIAN_POINT('Ctrl Pts',(-3.30509487819569,1.,-2.21703059947836));
#50420=CARTESIAN_POINT('Ctrl Pts',(-3.31244421655666,-1.,-2.21892881679086));
#50421=CARTESIAN_POINT('Ctrl Pts',(-3.31244421655666,1.,-2.21892881679086));
#50422=CARTESIAN_POINT('Ctrl Pts',(-3.31981686778022,-1.,-2.22078990842776));
#50423=CARTESIAN_POINT('Ctrl Pts',(-3.31981686778022,1.,-2.22078990842776));
#50424=CARTESIAN_POINT('Ctrl Pts',(-3.3272119632604,-1.,-2.22261398879635));
#50425=CARTESIAN_POINT('Ctrl Pts',(-3.3272119632604,1.,-2.22261398879635));
#50426=CARTESIAN_POINT('Ctrl Pts',(-3.33462772849598,-1.,-2.22440049878511));
#50427=CARTESIAN_POINT('Ctrl Pts',(-3.33462772849598,1.,-2.22440049878511));
#50428=CARTESIAN_POINT('Ctrl Pts',(-3.34206209449375,-1.,-2.22614863918047));
#50429=CARTESIAN_POINT('Ctrl Pts',(-3.34206209449375,1.,-2.22614863918047));
#50430=CARTESIAN_POINT('Ctrl Pts',(-3.34951327111096,-1.,-2.22785777756576));
#50431=CARTESIAN_POINT('Ctrl Pts',(-3.34951327111096,1.,-2.22785777756576));
#50432=CARTESIAN_POINT('Ctrl Pts',(-3.35698038165483,-1.,-2.22952789880982));
#50433=CARTESIAN_POINT('Ctrl Pts',(-3.35698038165483,1.,-2.22952789880982));
#50434=CARTESIAN_POINT('Ctrl Pts',(-3.36446325227848,-1.,-2.23115945849739));
#50435=CARTESIAN_POINT('Ctrl Pts',(-3.36446325227848,1.,-2.23115945849739));
#50436=CARTESIAN_POINT('Ctrl Pts',(-3.37196214349304,-1.,-2.23275319569221));
#50437=CARTESIAN_POINT('Ctrl Pts',(-3.37196214349304,1.,-2.23275319569221));
#50438=CARTESIAN_POINT('Ctrl Pts',(-3.37947749555632,-1.,-2.23430995599561));
#50439=CARTESIAN_POINT('Ctrl Pts',(-3.37947749555632,1.,-2.23430995599561));
#50440=CARTESIAN_POINT('Ctrl Pts',(-3.38700968549563,-1.,-2.23583052276308));
#50441=CARTESIAN_POINT('Ctrl Pts',(-3.38700968549563,1.,-2.23583052276308));
#50442=CARTESIAN_POINT('Ctrl Pts',(-3.39455873448189,-1.,-2.23731541452791));
#50443=CARTESIAN_POINT('Ctrl Pts',(-3.39455873448189,1.,-2.23731541452791));
#50444=CARTESIAN_POINT('Ctrl Pts',(-3.40212434705647,-1.,-2.2387649112415));
#50445=CARTESIAN_POINT('Ctrl Pts',(-3.40212434705647,1.,-2.2387649112415));
#50446=CARTESIAN_POINT('Ctrl Pts',(-3.40970604190328,-1.,-2.24017914395289));
#50447=CARTESIAN_POINT('Ctrl Pts',(-3.40970604190328,1.,-2.24017914395289));
#50448=CARTESIAN_POINT('Ctrl Pts',(-3.41730325539172,-1.,-2.24155816587844));
#50449=CARTESIAN_POINT('Ctrl Pts',(-3.41730325539172,1.,-2.24155816587844));
#50450=CARTESIAN_POINT('Ctrl Pts',(-3.42491544683008,-1.,-2.24290202531101));
#50451=CARTESIAN_POINT('Ctrl Pts',(-3.42491544683008,1.,-2.24290202531101));
#50452=CARTESIAN_POINT('Ctrl Pts',(-3.43254222614803,-1.,-2.24421085338727));
#50453=CARTESIAN_POINT('Ctrl Pts',(-3.43254222614803,1.,-2.24421085338727));
#50454=CARTESIAN_POINT('Ctrl Pts',(-3.4401833646032,-1.,-2.24548487526022));
#50455=CARTESIAN_POINT('Ctrl Pts',(-3.4401833646032,1.,-2.24548487526022));
#50456=CARTESIAN_POINT('Ctrl Pts',(-3.44783872863151,-1.,-2.2467243706995));
#50457=CARTESIAN_POINT('Ctrl Pts',(-3.44783872863151,1.,-2.2467243706995));
#50458=CARTESIAN_POINT('Ctrl Pts',(-3.45550823512049,-1.,-2.2479296496077));
#50459=CARTESIAN_POINT('Ctrl Pts',(-3.45550823512049,1.,-2.2479296496077));
#50460=CARTESIAN_POINT('Ctrl Pts',(-3.46319180177573,-1.,-2.2491010234604));
#50461=CARTESIAN_POINT('Ctrl Pts',(-3.46319180177573,1.,-2.2491010234604));
#50462=CARTESIAN_POINT('Ctrl Pts',(-3.47088928979888,-1.,-2.25023877475942));
#50463=CARTESIAN_POINT('Ctrl Pts',(-3.47088928979888,1.,-2.25023877475942));
#50464=CARTESIAN_POINT('Ctrl Pts',(-3.47860048448691,-1.,-2.25134314238687));
#50465=CARTESIAN_POINT('Ctrl Pts',(-3.47860048448691,1.,-2.25134314238687));
#50466=CARTESIAN_POINT('Ctrl Pts',(-3.48632513240961,-1.,-2.25241433138695));
#50467=CARTESIAN_POINT('Ctrl Pts',(-3.48632513240961,1.,-2.25241433138695));
#50468=CARTESIAN_POINT('Ctrl Pts',(-3.49406296494791,-1.,-2.2534525170976));
#50469=CARTESIAN_POINT('Ctrl Pts',(-3.49406296494791,1.,-2.2534525170976));
#50470=CARTESIAN_POINT('Ctrl Pts',(-3.50181372617971,-1.,-2.25445785151868));
#50471=CARTESIAN_POINT('Ctrl Pts',(-3.50181372617971,1.,-2.25445785151868));
#50472=CARTESIAN_POINT('Ctrl Pts',(-3.50957720117341,-1.,-2.25543046979799));
#50473=CARTESIAN_POINT('Ctrl Pts',(-3.50957720117341,1.,-2.25543046979799));
#50474=CARTESIAN_POINT('Ctrl Pts',(-3.51735323667612,-1.,-2.25637049455044));
#50475=CARTESIAN_POINT('Ctrl Pts',(-3.51735323667612,1.,-2.25637049455044));
#50476=CARTESIAN_POINT('Ctrl Pts',(-3.52514172847711,-1.,-2.25727802940898));
#50477=CARTESIAN_POINT('Ctrl Pts',(-3.52514172847711,1.,-2.25727802940898));
#50478=CARTESIAN_POINT('Ctrl Pts',(-3.53138243688262,-1.,-2.25797812950104));
#50479=CARTESIAN_POINT('Ctrl Pts',(-3.53138243688262,1.,-2.25797812950104));
#50480=CARTESIAN_POINT('Ctrl Pts',(-3.53606853162228,-1.,-2.25848864343951));
#50481=CARTESIAN_POINT('Ctrl Pts',(-3.53606853162228,1.,-2.25848864343951));
#50482=CARTESIAN_POINT('Ctrl Pts',(-3.53919506647335,-1.,-2.2588225169468));
#50483=CARTESIAN_POINT('Ctrl Pts',(-3.53919506647335,1.,-2.2588225169468));
#50484=CARTESIAN_POINT('Ctrl Pts',(-3.54075895182139,-1.,-2.25898783642071));
#50485=CARTESIAN_POINT('Ctrl Pts',(-3.54075895182139,1.,-2.25898783642071));
#50486=CARTESIAN_POINT('',(-3.08655633322212,1.,-2.1297112484669));
#50487=CARTESIAN_POINT('Ctrl Pts',(-3.08655633322212,-1.,-2.1297112484669));
#50488=CARTESIAN_POINT('Ctrl Pts',(-3.08655633322212,-0.666666666666667,
-2.1297112484669));
#50489=CARTESIAN_POINT('Ctrl Pts',(-3.08655633322212,-0.333333333333333,
-2.1297112484669));
#50490=CARTESIAN_POINT('Ctrl Pts',(-3.08655633322212,0.333333333333333,
-2.1297112484669));
#50491=CARTESIAN_POINT('Ctrl Pts',(-3.08655633322212,0.666666666666667,
-2.1297112484669));
#50492=CARTESIAN_POINT('Ctrl Pts',(-3.08655633322212,1.,-2.1297112484669));
#50493=CARTESIAN_POINT('',(-3.54075895182139,1.,-2.25898783642071));
#50494=CARTESIAN_POINT('',(-3.54075895182139,0.,-2.25898783642071));
#50495=CARTESIAN_POINT('Ctrl Pts',(-3.08655633322211,1.,-2.1297112484669));
#50496=CARTESIAN_POINT('Ctrl Pts',(-3.08657131089497,1.,-2.1297578506149));
#50497=CARTESIAN_POINT('Ctrl Pts',(-3.08668447250322,1.,-2.12991938762374));
#50498=CARTESIAN_POINT('Ctrl Pts',(-3.08717896996098,1.,-2.13034980480424));
#50499=CARTESIAN_POINT('Ctrl Pts',(-3.08855597949761,1.,-2.13132142793017));
#50500=CARTESIAN_POINT('Ctrl Pts',(-3.09151235281963,1.,-2.13321032560893));
#50501=CARTESIAN_POINT('Ctrl Pts',(-3.0960450242104,1.,-2.13596538661048));
#50502=CARTESIAN_POINT('Ctrl Pts',(-3.10171267391049,1.,-2.13930228863751));
#50503=CARTESIAN_POINT('Ctrl Pts',(-3.10821808668859,1.,-2.14302815601973));
#50504=CARTESIAN_POINT('Ctrl Pts',(-3.11522827016855,1.,-2.14692798457532));
#50505=CARTESIAN_POINT('Ctrl Pts',(-3.12242318151938,1.,-2.15079698090585));
#50506=CARTESIAN_POINT('Ctrl Pts',(-3.12954386795646,1.,-2.1544724138292));
#50507=CARTESIAN_POINT('Ctrl Pts',(-3.13645356563038,1.,-2.15787423530676));
#50508=CARTESIAN_POINT('Ctrl Pts',(-3.14314440427022,1.,-2.16100905914435));
#50509=CARTESIAN_POINT('Ctrl Pts',(-3.14968624389054,1.,-2.16393520288072));
#50510=CARTESIAN_POINT('Ctrl Pts',(-3.15618975593656,1.,-2.1667372844769));
#50511=CARTESIAN_POINT('Ctrl Pts',(-3.16276685102972,1.,-2.16949910801219));
#50512=CARTESIAN_POINT('Ctrl Pts',(-3.16948480019497,1.,-2.17227212063817));
#50513=CARTESIAN_POINT('Ctrl Pts',(-3.17635032802523,1.,-2.17506466903694));
#50514=CARTESIAN_POINT('Ctrl Pts',(-3.18333474627807,1.,-2.17785968847142));
#50515=CARTESIAN_POINT('Ctrl Pts',(-3.19038924261573,1.,-2.18062558031778));
#50516=CARTESIAN_POINT('Ctrl Pts',(-3.19746293740411,1.,-2.18332898656602));
#50517=CARTESIAN_POINT('Ctrl Pts',(-3.20452259717976,1.,-2.18594876115934));
#50518=CARTESIAN_POINT('Ctrl Pts',(-3.21156188355769,1.,-2.18848253363901));
#50519=CARTESIAN_POINT('Ctrl Pts',(-3.21859043114095,1.,-2.19093901948667));
#50520=CARTESIAN_POINT('Ctrl Pts',(-3.22562734221646,1.,-2.19333345123538));
#50521=CARTESIAN_POINT('Ctrl Pts',(-3.23269332296933,1.,-2.19568204933168));
#50522=CARTESIAN_POINT('Ctrl Pts',(-3.23980245361308,1.,-2.19799623693253));
#50523=CARTESIAN_POINT('Ctrl Pts',(-3.24695715874338,1.,-2.20027910880981));
#50524=CARTESIAN_POINT('Ctrl Pts',(-3.25415277957775,1.,-2.20252866491545));
#50525=CARTESIAN_POINT('Ctrl Pts',(-3.26138036637705,1.,-2.20473979048678));
#50526=CARTESIAN_POINT('Ctrl Pts',(-3.26863006136782,1.,-2.20690665217743));
#50527=CARTESIAN_POINT('Ctrl Pts',(-3.2758944800554,1.,-2.2090250941743));
#50528=CARTESIAN_POINT('Ctrl Pts',(-3.28317133333131,1.,-2.21109449750641));
#50529=CARTESIAN_POINT('Ctrl Pts',(-3.29046159238343,1.,-2.21311648827391));
#50530=CARTESIAN_POINT('Ctrl Pts',(-3.29776825193159,1.,-2.21509406923368));
#50531=CARTESIAN_POINT('Ctrl Pts',(-3.30509487819569,1.,-2.21703059947836));
#50532=CARTESIAN_POINT('Ctrl Pts',(-3.31244421655666,1.,-2.21892881679086));
#50533=CARTESIAN_POINT('Ctrl Pts',(-3.31981686778022,1.,-2.22078990842776));
#50534=CARTESIAN_POINT('Ctrl Pts',(-3.3272119632604,1.,-2.22261398879635));
#50535=CARTESIAN_POINT('Ctrl Pts',(-3.33462772849598,1.,-2.22440049878511));
#50536=CARTESIAN_POINT('Ctrl Pts',(-3.34206209449375,1.,-2.22614863918047));
#50537=CARTESIAN_POINT('Ctrl Pts',(-3.34951327111096,1.,-2.22785777756576));
#50538=CARTESIAN_POINT('Ctrl Pts',(-3.35698038165483,1.,-2.22952789880982));
#50539=CARTESIAN_POINT('Ctrl Pts',(-3.36446325227848,1.,-2.23115945849739));
#50540=CARTESIAN_POINT('Ctrl Pts',(-3.37196214349304,1.,-2.23275319569221));
#50541=CARTESIAN_POINT('Ctrl Pts',(-3.37947749555632,1.,-2.23430995599561));
#50542=CARTESIAN_POINT('Ctrl Pts',(-3.38700968549563,1.,-2.23583052276308));
#50543=CARTESIAN_POINT('Ctrl Pts',(-3.39455873448189,1.,-2.23731541452791));
#50544=CARTESIAN_POINT('Ctrl Pts',(-3.40212434705647,1.,-2.2387649112415));
#50545=CARTESIAN_POINT('Ctrl Pts',(-3.40970604190328,1.,-2.24017914395289));
#50546=CARTESIAN_POINT('Ctrl Pts',(-3.41730325539172,1.,-2.24155816587844));
#50547=CARTESIAN_POINT('Ctrl Pts',(-3.42491544683008,1.,-2.24290202531101));
#50548=CARTESIAN_POINT('Ctrl Pts',(-3.43254222614803,1.,-2.24421085338727));
#50549=CARTESIAN_POINT('Ctrl Pts',(-3.4401833646032,1.,-2.24548487526022));
#50550=CARTESIAN_POINT('Ctrl Pts',(-3.44783872863151,1.,-2.2467243706995));
#50551=CARTESIAN_POINT('Ctrl Pts',(-3.45550823512049,1.,-2.2479296496077));
#50552=CARTESIAN_POINT('Ctrl Pts',(-3.46319180177573,1.,-2.2491010234604));
#50553=CARTESIAN_POINT('Ctrl Pts',(-3.47088928979888,1.,-2.25023877475942));
#50554=CARTESIAN_POINT('Ctrl Pts',(-3.47860048448691,1.,-2.25134314238687));
#50555=CARTESIAN_POINT('Ctrl Pts',(-3.48632513240961,1.,-2.25241433138695));
#50556=CARTESIAN_POINT('Ctrl Pts',(-3.49406296494791,1.,-2.2534525170976));
#50557=CARTESIAN_POINT('Ctrl Pts',(-3.50181372617971,1.,-2.25445785151868));
#50558=CARTESIAN_POINT('Ctrl Pts',(-3.50957720117341,1.,-2.25543046979799));
#50559=CARTESIAN_POINT('Ctrl Pts',(-3.51735323667612,1.,-2.25637049455044));
#50560=CARTESIAN_POINT('Ctrl Pts',(-3.52514172847711,1.,-2.25727802940898));
#50561=CARTESIAN_POINT('Ctrl Pts',(-3.53138243688262,1.,-2.25797812950104));
#50562=CARTESIAN_POINT('Ctrl Pts',(-3.53606853162228,1.,-2.25848864343951));
#50563=CARTESIAN_POINT('Ctrl Pts',(-3.53919506647335,1.,-2.2588225169468));
#50564=CARTESIAN_POINT('Ctrl Pts',(-3.54075895182139,1.,-2.25898783642071));
#50565=CARTESIAN_POINT('Origin',(-3.54075895182139,0.,-2.25898783642071));
#50566=CARTESIAN_POINT('',(-3.62024382630768,1.,-2.12928030988903));
#50567=CARTESIAN_POINT('Origin',(0.,0.,0.));
#50568=CARTESIAN_POINT('',(-2.97927412174388,1.,-2.27737254473378));
#50569=CARTESIAN_POINT('Origin',(0.,1.,0.));
#50570=CARTESIAN_POINT('Ctrl Pts',(-2.97927412174388,1.,-2.27737254473378));
#50571=CARTESIAN_POINT('Ctrl Pts',(-2.97927412174388,0.666666666666667,
-2.27737254473378));
#50572=CARTESIAN_POINT('Ctrl Pts',(-2.97927412174388,0.333333333333333,
-2.27737254473378));
#50573=CARTESIAN_POINT('Ctrl Pts',(-2.97927412174388,-0.333333333333333,
-2.27737254473378));
#50574=CARTESIAN_POINT('Ctrl Pts',(-2.97927412174388,-0.666666666666667,
-2.27737254473378));
#50575=CARTESIAN_POINT('Ctrl Pts',(-2.97927412174388,-1.,-2.27737254473378));
#50576=CARTESIAN_POINT('Ctrl Pts',(-3.24257979115744,-1.,-2.66939624221984));
#50577=CARTESIAN_POINT('Ctrl Pts',(-3.24257979115744,1.,-2.66939624221984));
#50578=CARTESIAN_POINT('Ctrl Pts',(-3.24193929584813,-1.,-2.66795998539861));
#50579=CARTESIAN_POINT('Ctrl Pts',(-3.24193929584813,1.,-2.66795998539861));
#50580=CARTESIAN_POINT('Ctrl Pts',(-3.24065561087681,-1.,-2.66508964664767));
#50581=CARTESIAN_POINT('Ctrl Pts',(-3.24065561087681,1.,-2.66508964664767));
#50582=CARTESIAN_POINT('Ctrl Pts',(-3.23872200036311,-1.,-2.6607906631973));
#50583=CARTESIAN_POINT('Ctrl Pts',(-3.23872200036311,1.,-2.6607906631973));
#50584=CARTESIAN_POINT('Ctrl Pts',(-3.23612768065687,-1.,-2.6550717396303));
#50585=CARTESIAN_POINT('Ctrl Pts',(-3.23612768065687,1.,-2.6550717396303));
#50586=CARTESIAN_POINT('Ctrl Pts',(-3.23285778738558,-1.,-2.64794488744246));
#50587=CARTESIAN_POINT('Ctrl Pts',(-3.23285778738558,1.,-2.64794488744246));
#50588=CARTESIAN_POINT('Ctrl Pts',(-3.2295608435934,-1.,-2.64083992182478));
#50589=CARTESIAN_POINT('Ctrl Pts',(-3.2295608435934,1.,-2.64083992182478));
#50590=CARTESIAN_POINT('Ctrl Pts',(-3.22623678292539,-1.,-2.63375697391438));
#50591=CARTESIAN_POINT('Ctrl Pts',(-3.22623678292539,1.,-2.63375697391438));
#50592=CARTESIAN_POINT('Ctrl Pts',(-3.222885536128,-1.,-2.62669622735548));
#50593=CARTESIAN_POINT('Ctrl Pts',(-3.222885536128,1.,-2.62669622735548));
#50594=CARTESIAN_POINT('Ctrl Pts',(-3.21950704108654,-1.,-2.61965792832396));
#50595=CARTESIAN_POINT('Ctrl Pts',(-3.21950704108654,1.,-2.61965792832396));
#50596=CARTESIAN_POINT('Ctrl Pts',(-3.21610123232465,-1.,-2.61264236718662));
#50597=CARTESIAN_POINT('Ctrl Pts',(-3.21610123232465,1.,-2.61264236718662));
#50598=CARTESIAN_POINT('Ctrl Pts',(-3.21266802609297,-1.,-2.60564985359699));
#50599=CARTESIAN_POINT('Ctrl Pts',(-3.21266802609297,1.,-2.60564985359699));
#50600=CARTESIAN_POINT('Ctrl Pts',(-3.2092073056959,-1.,-2.59868069194267));
#50601=CARTESIAN_POINT('Ctrl Pts',(-3.2092073056959,1.,-2.59868069194267));
#50602=CARTESIAN_POINT('Ctrl Pts',(-3.20571891028879,-1.,-2.59173516023605));
#50603=CARTESIAN_POINT('Ctrl Pts',(-3.20571891028879,1.,-2.59173516023605));
#50604=CARTESIAN_POINT('Ctrl Pts',(-3.20220261408685,-1.,-2.58481347777953));
#50605=CARTESIAN_POINT('Ctrl Pts',(-3.20220261408685,1.,-2.58481347777953));
#50606=CARTESIAN_POINT('Ctrl Pts',(-3.19865814628955,-1.,-2.577915819091));
#50607=CARTESIAN_POINT('Ctrl Pts',(-3.19865814628955,1.,-2.577915819091));
#50608=CARTESIAN_POINT('Ctrl Pts',(-3.19508523784548,-1.,-2.57104235898053));
#50609=CARTESIAN_POINT('Ctrl Pts',(-3.19508523784548,1.,-2.57104235898053));
#50610=CARTESIAN_POINT('Ctrl Pts',(-3.19148366395201,-1.,-2.56419331092909));
#50611=CARTESIAN_POINT('Ctrl Pts',(-3.19148366395201,1.,-2.56419331092909));
#50612=CARTESIAN_POINT('Ctrl Pts',(-3.1878532811617,-1.,-2.55736896206016));
#50613=CARTESIAN_POINT('Ctrl Pts',(-3.1878532811617,1.,-2.55736896206016));
#50614=CARTESIAN_POINT('Ctrl Pts',(-3.18419408529482,-1.,-2.55056972387638));
#50615=CARTESIAN_POINT('Ctrl Pts',(-3.18419408529482,1.,-2.55056972387638));
#50616=CARTESIAN_POINT('Ctrl Pts',(-3.18050619750515,-1.,-2.54379612552948));
#50617=CARTESIAN_POINT('Ctrl Pts',(-3.18050619750515,1.,-2.54379612552948));
#50618=CARTESIAN_POINT('Ctrl Pts',(-3.17678974135225,-1.,-2.53704871950871));
#50619=CARTESIAN_POINT('Ctrl Pts',(-3.17678974135225,1.,-2.53704871950871));
#50620=CARTESIAN_POINT('Ctrl Pts',(-3.17304474093574,-1.,-2.5303280040691));
#50621=CARTESIAN_POINT('Ctrl Pts',(-3.17304474093574,1.,-2.5303280040691));
#50622=CARTESIAN_POINT('Ctrl Pts',(-3.16927102130751,-1.,-2.523634346718));
#50623=CARTESIAN_POINT('Ctrl Pts',(-3.16927102130751,1.,-2.523634346718));
#50624=CARTESIAN_POINT('Ctrl Pts',(-3.16546808277069,-1.,-2.51696788755615));
#50625=CARTESIAN_POINT('Ctrl Pts',(-3.16546808277069,1.,-2.51696788755615));
#50626=CARTESIAN_POINT('Ctrl Pts',(-3.16163506380211,-1.,-2.51032851007939));
#50627=CARTESIAN_POINT('Ctrl Pts',(-3.16163506380211,1.,-2.51032851007939));
#50628=CARTESIAN_POINT('Ctrl Pts',(-3.15777102413998,-1.,-2.50371605688287));
#50629=CARTESIAN_POINT('Ctrl Pts',(-3.15777102413998,1.,-2.50371605688287));
#50630=CARTESIAN_POINT('Ctrl Pts',(-3.15387518039064,-1.,-2.49713050858911));
#50631=CARTESIAN_POINT('Ctrl Pts',(-3.15387518039064,1.,-2.49713050858911));
#50632=CARTESIAN_POINT('Ctrl Pts',(-3.14994715298903,-1.,-2.49057217131985));
#50633=CARTESIAN_POINT('Ctrl Pts',(-3.14994715298903,1.,-2.49057217131985));
#50634=CARTESIAN_POINT('Ctrl Pts',(-3.1459872272388,-1.,-2.48404187418376));
#50635=CARTESIAN_POINT('Ctrl Pts',(-3.1459872272388,1.,-2.48404187418376));
#50636=CARTESIAN_POINT('Ctrl Pts',(-3.14199655778845,-1.,-2.47754112428027));
#50637=CARTESIAN_POINT('Ctrl Pts',(-3.14199655778845,1.,-2.47754112428027));
#50638=CARTESIAN_POINT('Ctrl Pts',(-3.13797654408931,-1.,-2.47107164236827));
#50639=CARTESIAN_POINT('Ctrl Pts',(-3.13797654408931,1.,-2.47107164236827));
#50640=CARTESIAN_POINT('Ctrl Pts',(-3.13392826623902,-1.,-2.4646349433237));
#50641=CARTESIAN_POINT('Ctrl Pts',(-3.13392826623902,1.,-2.4646349433237));
#50642=CARTESIAN_POINT('Ctrl Pts',(-3.12985188384372,-1.,-2.45823188859366));
#50643=CARTESIAN_POINT('Ctrl Pts',(-3.12985188384372,1.,-2.45823188859366));
#50644=CARTESIAN_POINT('Ctrl Pts',(-3.12574608210849,-1.,-2.45186227369848));
#50645=CARTESIAN_POINT('Ctrl Pts',(-3.12574608210849,1.,-2.45186227369848));
#50646=CARTESIAN_POINT('Ctrl Pts',(-3.12160740887768,-1.,-2.44552433364716));
#50647=CARTESIAN_POINT('Ctrl Pts',(-3.12160740887768,1.,-2.44552433364716));
#50648=CARTESIAN_POINT('Ctrl Pts',(-3.11743156744182,-1.,-2.43921571477975));
#50649=CARTESIAN_POINT('Ctrl Pts',(-3.11743156744182,1.,-2.43921571477975));
#50650=CARTESIAN_POINT('Ctrl Pts',(-3.11321477659012,-1.,-2.4329344968514));
#50651=CARTESIAN_POINT('Ctrl Pts',(-3.11321477659012,1.,-2.4329344968514));
#50652=CARTESIAN_POINT('Ctrl Pts',(-3.10895518969592,-1.,-2.42668025870013));
#50653=CARTESIAN_POINT('Ctrl Pts',(-3.10895518969592,1.,-2.42668025870013));
#50654=CARTESIAN_POINT('Ctrl Pts',(-3.10465410280902,-1.,-2.42045498612494));
#50655=CARTESIAN_POINT('Ctrl Pts',(-3.10465410280902,1.,-2.42045498612494));
#50656=CARTESIAN_POINT('Ctrl Pts',(-3.10031775027683,-1.,-2.41426441798067));
#50657=CARTESIAN_POINT('Ctrl Pts',(-3.10031775027683,1.,-2.41426441798067));
#50658=CARTESIAN_POINT('Ctrl Pts',(-3.09595472616093,-1.,-2.40811612696382));
#50659=CARTESIAN_POINT('Ctrl Pts',(-3.09595472616093,1.,-2.40811612696382));
#50660=CARTESIAN_POINT('Ctrl Pts',(-3.09157266051115,-1.,-2.40201704423352));
#50661=CARTESIAN_POINT('Ctrl Pts',(-3.09157266051115,1.,-2.40201704423352));
#50662=CARTESIAN_POINT('Ctrl Pts',(-3.08717489512919,-1.,-2.39597098250635));
#50663=CARTESIAN_POINT('Ctrl Pts',(-3.08717489512919,1.,-2.39597098250635));
#50664=CARTESIAN_POINT('Ctrl Pts',(-3.08275773747083,-1.,-2.38997659219192));
#50665=CARTESIAN_POINT('Ctrl Pts',(-3.08275773747083,1.,-2.38997659219192));
#50666=CARTESIAN_POINT('Ctrl Pts',(-3.07830597244301,-1.,-2.38402401216107));
#50667=CARTESIAN_POINT('Ctrl Pts',(-3.07830597244301,1.,-2.38402401216107));
#50668=CARTESIAN_POINT('Ctrl Pts',(-3.07379777492133,-1.,-2.37809856205524));
#50669=CARTESIAN_POINT('Ctrl Pts',(-3.07379777492133,1.,-2.37809856205524));
#50670=CARTESIAN_POINT('Ctrl Pts',(-3.06921275497472,-1.,-2.37218678163157));
#50671=CARTESIAN_POINT('Ctrl Pts',(-3.06921275497472,1.,-2.37218678163157));
#50672=CARTESIAN_POINT('Ctrl Pts',(-3.06453964643152,-1.,-2.36628220107001));
#50673=CARTESIAN_POINT('Ctrl Pts',(-3.06453964643152,1.,-2.36628220107001));
#50674=CARTESIAN_POINT('Ctrl Pts',(-3.05978266240056,-1.,-2.36039011602084));
#50675=CARTESIAN_POINT('Ctrl Pts',(-3.05978266240056,1.,-2.36039011602084));
#50676=CARTESIAN_POINT('Ctrl Pts',(-3.05497218368188,-1.,-2.35453559889506));
#50677=CARTESIAN_POINT('Ctrl Pts',(-3.05497218368188,1.,-2.35453559889506));
#50678=CARTESIAN_POINT('Ctrl Pts',(-3.05015565829976,-1.,-2.34875673090816));
#50679=CARTESIAN_POINT('Ctrl Pts',(-3.05015565829976,1.,-2.34875673090816));
#50680=CARTESIAN_POINT('Ctrl Pts',(-3.04537822217311,-1.,-2.3430901708402));
#50681=CARTESIAN_POINT('Ctrl Pts',(-3.04537822217311,1.,-2.3430901708402));
#50682=CARTESIAN_POINT('Ctrl Pts',(-3.04066496998569,-1.,-2.33755792953726));
#50683=CARTESIAN_POINT('Ctrl Pts',(-3.04066496998569,1.,-2.33755792953726));
#50684=CARTESIAN_POINT('Ctrl Pts',(-3.03600588555765,-1.,-2.33215619079807));
#50685=CARTESIAN_POINT('Ctrl Pts',(-3.03600588555765,1.,-2.33215619079807));
#50686=CARTESIAN_POINT('Ctrl Pts',(-3.03133125185047,-1.,-2.32683687412027));
#50687=CARTESIAN_POINT('Ctrl Pts',(-3.03133125185047,1.,-2.32683687412027));
#50688=CARTESIAN_POINT('Ctrl Pts',(-3.02652678416478,-1.,-2.32151944306299));
#50689=CARTESIAN_POINT('Ctrl Pts',(-3.02652678416478,1.,-2.32151944306299));
#50690=CARTESIAN_POINT('Ctrl Pts',(-3.02147780668029,-1.,-2.31612479121528));
#50691=CARTESIAN_POINT('Ctrl Pts',(-3.02147780668029,1.,-2.31612479121528));
#50692=CARTESIAN_POINT('Ctrl Pts',(-3.01610726819019,-1.,-2.31060449886577));
#50693=CARTESIAN_POINT('Ctrl Pts',(-3.01610726819019,1.,-2.31060449886577));
#50694=CARTESIAN_POINT('Ctrl Pts',(-3.01041131063882,-1.,-2.30496809486528));
#50695=CARTESIAN_POINT('Ctrl Pts',(-3.01041131063882,1.,-2.30496809486528));
#50696=CARTESIAN_POINT('Ctrl Pts',(-3.00450832658822,-1.,-2.29932091315939));
#50697=CARTESIAN_POINT('Ctrl Pts',(-3.00450832658822,1.,-2.29932091315939));
#50698=CARTESIAN_POINT('Ctrl Pts',(-2.99863310340004,-1.,-2.29385894577999));
#50699=CARTESIAN_POINT('Ctrl Pts',(-2.99863310340004,1.,-2.29385894577999));
#50700=CARTESIAN_POINT('Ctrl Pts',(-2.9930793098434,-1.,-2.28882328690601));
#50701=CARTESIAN_POINT('Ctrl Pts',(-2.9930793098434,1.,-2.28882328690601));
#50702=CARTESIAN_POINT('Ctrl Pts',(-2.98815432734929,-1.,-2.28446419116036));
#50703=CARTESIAN_POINT('Ctrl Pts',(-2.98815432734929,1.,-2.28446419116036));
#50704=CARTESIAN_POINT('Ctrl Pts',(-2.98413343613858,-1.,-2.28100472516582));
#50705=CARTESIAN_POINT('Ctrl Pts',(-2.98413343613858,1.,-2.28100472516582));
#50706=CARTESIAN_POINT('Ctrl Pts',(-2.98120357932601,-1.,-2.2785960133424));
#50707=CARTESIAN_POINT('Ctrl Pts',(-2.98120357932601,1.,-2.2785960133424));
#50708=CARTESIAN_POINT('Ctrl Pts',(-2.97980276182744,-1.,-2.27756633754846));
#50709=CARTESIAN_POINT('Ctrl Pts',(-2.97980276182744,1.,-2.27756633754846));
#50710=CARTESIAN_POINT('Ctrl Pts',(-2.97929608861502,-1.,-2.27730961189188));
#50711=CARTESIAN_POINT('Ctrl Pts',(-2.97929608861502,1.,-2.27730961189188));
#50712=CARTESIAN_POINT('Ctrl Pts',(-2.97919987915565,-1.,-2.2773674298423));
#50713=CARTESIAN_POINT('Ctrl Pts',(-2.97919987915565,1.,-2.2773674298423));
#50714=CARTESIAN_POINT('Ctrl Pts',(-2.97921217251145,-1.,-2.27745358485296));
#50715=CARTESIAN_POINT('Ctrl Pts',(-2.97921217251145,1.,-2.27745358485296));
#50716=CARTESIAN_POINT('',(-3.24257979115744,1.,-2.66939624221984));
#50717=CARTESIAN_POINT('Ctrl Pts',(-3.24257979115744,1.,-2.66939624221984));
#50718=CARTESIAN_POINT('Ctrl Pts',(-3.24193929584813,1.,-2.66795998539861));
#50719=CARTESIAN_POINT('Ctrl Pts',(-3.24065561087681,1.,-2.66508964664767));
#50720=CARTESIAN_POINT('Ctrl Pts',(-3.23872200036311,1.,-2.6607906631973));
#50721=CARTESIAN_POINT('Ctrl Pts',(-3.23612768065687,1.,-2.6550717396303));
#50722=CARTESIAN_POINT('Ctrl Pts',(-3.23285778738558,1.,-2.64794488744246));
#50723=CARTESIAN_POINT('Ctrl Pts',(-3.2295608435934,1.,-2.64083992182478));
#50724=CARTESIAN_POINT('Ctrl Pts',(-3.22623678292539,1.,-2.63375697391438));
#50725=CARTESIAN_POINT('Ctrl Pts',(-3.222885536128,1.,-2.62669622735548));
#50726=CARTESIAN_POINT('Ctrl Pts',(-3.21950704108654,1.,-2.61965792832396));
#50727=CARTESIAN_POINT('Ctrl Pts',(-3.21610123232465,1.,-2.61264236718662));
#50728=CARTESIAN_POINT('Ctrl Pts',(-3.21266802609297,1.,-2.60564985359699));
#50729=CARTESIAN_POINT('Ctrl Pts',(-3.2092073056959,1.,-2.59868069194267));
#50730=CARTESIAN_POINT('Ctrl Pts',(-3.20571891028879,1.,-2.59173516023605));
#50731=CARTESIAN_POINT('Ctrl Pts',(-3.20220261408685,1.,-2.58481347777953));
#50732=CARTESIAN_POINT('Ctrl Pts',(-3.19865814628955,1.,-2.577915819091));
#50733=CARTESIAN_POINT('Ctrl Pts',(-3.19508523784548,1.,-2.57104235898053));
#50734=CARTESIAN_POINT('Ctrl Pts',(-3.19148366395201,1.,-2.56419331092909));
#50735=CARTESIAN_POINT('Ctrl Pts',(-3.1878532811617,1.,-2.55736896206016));
#50736=CARTESIAN_POINT('Ctrl Pts',(-3.18419408529482,1.,-2.55056972387638));
#50737=CARTESIAN_POINT('Ctrl Pts',(-3.18050619750515,1.,-2.54379612552948));
#50738=CARTESIAN_POINT('Ctrl Pts',(-3.17678974135225,1.,-2.53704871950871));
#50739=CARTESIAN_POINT('Ctrl Pts',(-3.17304474093574,1.,-2.5303280040691));
#50740=CARTESIAN_POINT('Ctrl Pts',(-3.16927102130751,1.,-2.523634346718));
#50741=CARTESIAN_POINT('Ctrl Pts',(-3.16546808277069,1.,-2.51696788755615));
#50742=CARTESIAN_POINT('Ctrl Pts',(-3.16163506380211,1.,-2.51032851007939));
#50743=CARTESIAN_POINT('Ctrl Pts',(-3.15777102413998,1.,-2.50371605688287));
#50744=CARTESIAN_POINT('Ctrl Pts',(-3.15387518039064,1.,-2.49713050858911));
#50745=CARTESIAN_POINT('Ctrl Pts',(-3.14994715298903,1.,-2.49057217131985));
#50746=CARTESIAN_POINT('Ctrl Pts',(-3.1459872272388,1.,-2.48404187418376));
#50747=CARTESIAN_POINT('Ctrl Pts',(-3.14199655778845,1.,-2.47754112428027));
#50748=CARTESIAN_POINT('Ctrl Pts',(-3.13797654408931,1.,-2.47107164236827));
#50749=CARTESIAN_POINT('Ctrl Pts',(-3.13392826623902,1.,-2.4646349433237));
#50750=CARTESIAN_POINT('Ctrl Pts',(-3.12985188384372,1.,-2.45823188859366));
#50751=CARTESIAN_POINT('Ctrl Pts',(-3.12574608210849,1.,-2.45186227369848));
#50752=CARTESIAN_POINT('Ctrl Pts',(-3.12160740887768,1.,-2.44552433364716));
#50753=CARTESIAN_POINT('Ctrl Pts',(-3.11743156744182,1.,-2.43921571477975));
#50754=CARTESIAN_POINT('Ctrl Pts',(-3.11321477659012,1.,-2.4329344968514));
#50755=CARTESIAN_POINT('Ctrl Pts',(-3.10895518969592,1.,-2.42668025870013));
#50756=CARTESIAN_POINT('Ctrl Pts',(-3.10465410280902,1.,-2.42045498612494));
#50757=CARTESIAN_POINT('Ctrl Pts',(-3.10031775027683,1.,-2.41426441798067));
#50758=CARTESIAN_POINT('Ctrl Pts',(-3.09595472616093,1.,-2.40811612696382));
#50759=CARTESIAN_POINT('Ctrl Pts',(-3.09157266051115,1.,-2.40201704423352));
#50760=CARTESIAN_POINT('Ctrl Pts',(-3.08717489512919,1.,-2.39597098250635));
#50761=CARTESIAN_POINT('Ctrl Pts',(-3.08275773747083,1.,-2.38997659219192));
#50762=CARTESIAN_POINT('Ctrl Pts',(-3.07830597244301,1.,-2.38402401216107));
#50763=CARTESIAN_POINT('Ctrl Pts',(-3.07379777492133,1.,-2.37809856205524));
#50764=CARTESIAN_POINT('Ctrl Pts',(-3.06921275497472,1.,-2.37218678163157));
#50765=CARTESIAN_POINT('Ctrl Pts',(-3.06453964643152,1.,-2.36628220107001));
#50766=CARTESIAN_POINT('Ctrl Pts',(-3.05978266240056,1.,-2.36039011602084));
#50767=CARTESIAN_POINT('Ctrl Pts',(-3.05497218368188,1.,-2.35453559889506));
#50768=CARTESIAN_POINT('Ctrl Pts',(-3.05015565829976,1.,-2.34875673090816));
#50769=CARTESIAN_POINT('Ctrl Pts',(-3.04537822217311,1.,-2.3430901708402));
#50770=CARTESIAN_POINT('Ctrl Pts',(-3.04066496998569,1.,-2.33755792953726));
#50771=CARTESIAN_POINT('Ctrl Pts',(-3.03600588555765,1.,-2.33215619079807));
#50772=CARTESIAN_POINT('Ctrl Pts',(-3.03133125185047,1.,-2.32683687412027));
#50773=CARTESIAN_POINT('Ctrl Pts',(-3.02652678416478,1.,-2.32151944306299));
#50774=CARTESIAN_POINT('Ctrl Pts',(-3.02147780668029,1.,-2.31612479121528));
#50775=CARTESIAN_POINT('Ctrl Pts',(-3.01610726819019,1.,-2.31060449886577));
#50776=CARTESIAN_POINT('Ctrl Pts',(-3.01041131063882,1.,-2.30496809486528));
#50777=CARTESIAN_POINT('Ctrl Pts',(-3.00450832658822,1.,-2.29932091315939));
#50778=CARTESIAN_POINT('Ctrl Pts',(-2.99863310340004,1.,-2.29385894577999));
#50779=CARTESIAN_POINT('Ctrl Pts',(-2.9930793098434,1.,-2.28882328690601));
#50780=CARTESIAN_POINT('Ctrl Pts',(-2.98815432734929,1.,-2.28446419116036));
#50781=CARTESIAN_POINT('Ctrl Pts',(-2.98413343613858,1.,-2.28100472516582));
#50782=CARTESIAN_POINT('Ctrl Pts',(-2.98142341809623,1.,-2.27877674853833));
#50783=CARTESIAN_POINT('Ctrl Pts',(-2.98007383024333,1.,-2.27776738270369));
#50784=CARTESIAN_POINT('Ctrl Pts',(-2.97951167106106,1.,-2.27743009389704));
#50785=CARTESIAN_POINT('Ctrl Pts',(-2.97932307137589,1.,-2.27737238849212));
#50786=CARTESIAN_POINT('Ctrl Pts',(-2.97927412174388,1.,-2.27737254473378));
#50787=CARTESIAN_POINT('',(-3.24257979115744,0.,-2.66939624221984));
#50788=CARTESIAN_POINT('Ctrl Pts',(-2.71546581445404,-1.,-2.58626089374824));
#50789=CARTESIAN_POINT('Ctrl Pts',(-2.71546581445404,1.,-2.58626089374824));
#50790=CARTESIAN_POINT('Ctrl Pts',(-2.71537879705104,-1.,-2.58626222935803));
#50791=CARTESIAN_POINT('Ctrl Pts',(-2.71537879705104,1.,-2.58626222935803));
#50792=CARTESIAN_POINT('Ctrl Pts',(-2.71533674141254,-1.,-2.58636629904103));
#50793=CARTESIAN_POINT('Ctrl Pts',(-2.71533674141254,1.,-2.58636629904103));
#50794=CARTESIAN_POINT('Ctrl Pts',(-2.71566956750452,-1.,-2.5868265735259));
#50795=CARTESIAN_POINT('Ctrl Pts',(-2.71566956750452,1.,-2.5868265735259));
#50796=CARTESIAN_POINT('Ctrl Pts',(-2.71690570241638,-1.,-2.58804906785417));
#50797=CARTESIAN_POINT('Ctrl Pts',(-2.71690570241638,1.,-2.58804906785417));
#50798=CARTESIAN_POINT('Ctrl Pts',(-2.71974308958086,-1.,-2.59056604771971));
#50799=CARTESIAN_POINT('Ctrl Pts',(-2.71974308958086,1.,-2.59056604771971));
#50800=CARTESIAN_POINT('Ctrl Pts',(-2.72378896977134,-1.,-2.59399625537278));
#50801=CARTESIAN_POINT('Ctrl Pts',(-2.72378896977134,1.,-2.59399625537278));
#50802=CARTESIAN_POINT('Ctrl Pts',(-2.7288648348152,-1.,-2.59817869034746));
#50803=CARTESIAN_POINT('Ctrl Pts',(-2.7288648348152,1.,-2.59817869034746));
#50804=CARTESIAN_POINT('Ctrl Pts',(-2.73470730109615,-1.,-2.60287635688728));
#50805=CARTESIAN_POINT('Ctrl Pts',(-2.73470730109615,1.,-2.60287635688728));
#50806=CARTESIAN_POINT('Ctrl Pts',(-2.7410211099909,-1.,-2.60782480638448));
#50807=CARTESIAN_POINT('Ctrl Pts',(-2.7410211099909,1.,-2.60782480638448));
#50808=CARTESIAN_POINT('Ctrl Pts',(-2.74752219567252,-1.,-2.61277170105813));
#50809=CARTESIAN_POINT('Ctrl Pts',(-2.74752219567252,1.,-2.61277170105813));
#50810=CARTESIAN_POINT('Ctrl Pts',(-2.7539802502603,-1.,-2.61751580407667));
#50811=CARTESIAN_POINT('Ctrl Pts',(-2.7539802502603,1.,-2.61751580407667));
#50812=CARTESIAN_POINT('Ctrl Pts',(-2.76027271596686,-1.,-2.62195665834605));
#50813=CARTESIAN_POINT('Ctrl Pts',(-2.76027271596686,1.,-2.62195665834605));
#50814=CARTESIAN_POINT('Ctrl Pts',(-2.76639078479021,-1.,-2.62609956506355));
#50815=CARTESIAN_POINT('Ctrl Pts',(-2.76639078479021,1.,-2.62609956506355));
#50816=CARTESIAN_POINT('Ctrl Pts',(-2.77239433377921,-1.,-2.63001305229625));
#50817=CARTESIAN_POINT('Ctrl Pts',(-2.77239433377921,1.,-2.63001305229625));
#50818=CARTESIAN_POINT('Ctrl Pts',(-2.77837943466449,-1.,-2.63379800904599));
#50819=CARTESIAN_POINT('Ctrl Pts',(-2.77837943466449,1.,-2.63379800904599));
#50820=CARTESIAN_POINT('Ctrl Pts',(-2.78444351041571,-1.,-2.637554714303));
#50821=CARTESIAN_POINT('Ctrl Pts',(-2.78444351041571,1.,-2.637554714303));
#50822=CARTESIAN_POINT('Ctrl Pts',(-2.79064495573224,-1.,-2.64134450532584));
#50823=CARTESIAN_POINT('Ctrl Pts',(-2.79064495573224,1.,-2.64134450532584));
#50824=CARTESIAN_POINT('Ctrl Pts',(-2.79698910670736,-1.,-2.64517667799319));
#50825=CARTESIAN_POINT('Ctrl Pts',(-2.79698910670736,1.,-2.64517667799319));
#50826=CARTESIAN_POINT('Ctrl Pts',(-2.80345029781152,-1.,-2.64902988983337));
#50827=CARTESIAN_POINT('Ctrl Pts',(-2.80345029781152,1.,-2.64902988983337));
#50828=CARTESIAN_POINT('Ctrl Pts',(-2.80998526078165,-1.,-2.65286529532208));
#50829=CARTESIAN_POINT('Ctrl Pts',(-2.80998526078165,1.,-2.65286529532208));
#50830=CARTESIAN_POINT('Ctrl Pts',(-2.81654896073883,-1.,-2.65664198781344));
#50831=CARTESIAN_POINT('Ctrl Pts',(-2.81654896073883,1.,-2.65664198781344));
#50832=CARTESIAN_POINT('Ctrl Pts',(-2.82311188135078,-1.,-2.66033388273461));
#50833=CARTESIAN_POINT('Ctrl Pts',(-2.82311188135078,1.,-2.66033388273461));
#50834=CARTESIAN_POINT('Ctrl Pts',(-2.82966813308998,-1.,-2.6639376472693));
#50835=CARTESIAN_POINT('Ctrl Pts',(-2.82966813308998,1.,-2.6639376472693));
#50836=CARTESIAN_POINT('Ctrl Pts',(-2.83622586853982,-1.,-2.66746339678107));
#50837=CARTESIAN_POINT('Ctrl Pts',(-2.83622586853982,1.,-2.66746339678107));
#50838=CARTESIAN_POINT('Ctrl Pts',(-2.84280157191323,-1.,-2.67092916452125));
#50839=CARTESIAN_POINT('Ctrl Pts',(-2.84280157191323,1.,-2.67092916452125));
#50840=CARTESIAN_POINT('Ctrl Pts',(-2.84941315703092,-1.,-2.67435421039677));
#50841=CARTESIAN_POINT('Ctrl Pts',(-2.84941315703092,1.,-2.67435421039677));
#50842=CARTESIAN_POINT('Ctrl Pts',(-2.85607274378018,-1.,-2.67775201955724));
#50843=CARTESIAN_POINT('Ctrl Pts',(-2.85607274378018,1.,-2.67775201955724));
#50844=CARTESIAN_POINT('Ctrl Pts',(-2.86278224277689,-1.,-2.68112602796308));
#50845=CARTESIAN_POINT('Ctrl Pts',(-2.86278224277689,1.,-2.68112602796308));
#50846=CARTESIAN_POINT('Ctrl Pts',(-2.86953736547238,-1.,-2.68447353139599));
#50847=CARTESIAN_POINT('Ctrl Pts',(-2.86953736547238,1.,-2.68447353139599));
#50848=CARTESIAN_POINT('Ctrl Pts',(-2.8763300724388,-1.,-2.68778807801686));
#50849=CARTESIAN_POINT('Ctrl Pts',(-2.8763300724388,1.,-2.68778807801686));
#50850=CARTESIAN_POINT('Ctrl Pts',(-2.88315153980466,-1.,-2.69106236420198));
#50851=CARTESIAN_POINT('Ctrl Pts',(-2.88315153980466,1.,-2.69106236420198));
#50852=CARTESIAN_POINT('Ctrl Pts',(-2.88999512410309,-1.,-2.69429113011374));
#50853=CARTESIAN_POINT('Ctrl Pts',(-2.88999512410309,1.,-2.69429113011374));
#50854=CARTESIAN_POINT('Ctrl Pts',(-2.89685866123671,-1.,-2.69747340630625));
#50855=CARTESIAN_POINT('Ctrl Pts',(-2.89685866123671,1.,-2.69747340630625));
#50856=CARTESIAN_POINT('Ctrl Pts',(-2.90374285605838,-1.,-2.70061095078692));
#50857=CARTESIAN_POINT('Ctrl Pts',(-2.90374285605838,1.,-2.70061095078692));
#50858=CARTESIAN_POINT('Ctrl Pts',(-2.91065019668329,-1.,-2.70370719782113));
#50859=CARTESIAN_POINT('Ctrl Pts',(-2.91065019668329,1.,-2.70370719782113));
#50860=CARTESIAN_POINT('Ctrl Pts',(-2.91758367994737,-1.,-2.70676602302518));
#50861=CARTESIAN_POINT('Ctrl Pts',(-2.91758367994737,1.,-2.70676602302518));
#50862=CARTESIAN_POINT('Ctrl Pts',(-2.92454558914778,-1.,-2.70979055994754));
#50863=CARTESIAN_POINT('Ctrl Pts',(-2.92454558914778,1.,-2.70979055994754));
#50864=CARTESIAN_POINT('Ctrl Pts',(-2.93153633192595,-1.,-2.71278207520817));
#50865=CARTESIAN_POINT('Ctrl Pts',(-2.93153633192595,1.,-2.71278207520817));
#50866=CARTESIAN_POINT('Ctrl Pts',(-2.93855503247266,-1.,-2.7157405459259));
#50867=CARTESIAN_POINT('Ctrl Pts',(-2.93855503247266,1.,-2.7157405459259));
#50868=CARTESIAN_POINT('Ctrl Pts',(-2.94560002559806,-1.,-2.71866514227965));
#50869=CARTESIAN_POINT('Ctrl Pts',(-2.94560002559806,1.,-2.71866514227965));
#50870=CARTESIAN_POINT('Ctrl Pts',(-2.95266939280621,-1.,-2.72155475123364));
#50871=CARTESIAN_POINT('Ctrl Pts',(-2.95266939280621,1.,-2.72155475123364));
#50872=CARTESIAN_POINT('Ctrl Pts',(-2.95976146492576,-1.,-2.72440846811729));
#50873=CARTESIAN_POINT('Ctrl Pts',(-2.95976146492576,1.,-2.72440846811729));
#50874=CARTESIAN_POINT('Ctrl Pts',(-2.96687537842451,-1.,-2.72722614084076));
#50875=CARTESIAN_POINT('Ctrl Pts',(-2.96687537842451,1.,-2.72722614084076));
#50876=CARTESIAN_POINT('Ctrl Pts',(-2.97401089032677,-1.,-2.73000819218414));
#50877=CARTESIAN_POINT('Ctrl Pts',(-2.97401089032677,1.,-2.73000819218414));
#50878=CARTESIAN_POINT('Ctrl Pts',(-2.98116814232129,-1.,-2.73275539286497));
#50879=CARTESIAN_POINT('Ctrl Pts',(-2.98116814232129,1.,-2.73275539286497));
#50880=CARTESIAN_POINT('Ctrl Pts',(-2.9883474369644,-1.,-2.73546864694536));
#50881=CARTESIAN_POINT('Ctrl Pts',(-2.9883474369644,1.,-2.73546864694536));
#50882=CARTESIAN_POINT('Ctrl Pts',(-2.99554902409778,-1.,-2.73814878711641));
#50883=CARTESIAN_POINT('Ctrl Pts',(-2.99554902409778,1.,-2.73814878711641));
#50884=CARTESIAN_POINT('Ctrl Pts',(-3.00277284351521,-1.,-2.74079632883931));
#50885=CARTESIAN_POINT('Ctrl Pts',(-3.00277284351521,1.,-2.74079632883931));
#50886=CARTESIAN_POINT('Ctrl Pts',(-3.01001855960162,-1.,-2.74341150239887));
#50887=CARTESIAN_POINT('Ctrl Pts',(-3.01001855960162,1.,-2.74341150239887));
#50888=CARTESIAN_POINT('Ctrl Pts',(-3.01728567646611,-1.,-2.74599436193625));
#50889=CARTESIAN_POINT('Ctrl Pts',(-3.01728567646611,1.,-2.74599436193625));
#50890=CARTESIAN_POINT('Ctrl Pts',(-3.02457362909245,-1.,-2.7485448718414));
#50891=CARTESIAN_POINT('Ctrl Pts',(-3.02457362909245,1.,-2.7485448718414));
#50892=CARTESIAN_POINT('Ctrl Pts',(-3.03188187589107,-1.,-2.75106299522979));
#50893=CARTESIAN_POINT('Ctrl Pts',(-3.03188187589107,1.,-2.75106299522979));
#50894=CARTESIAN_POINT('Ctrl Pts',(-3.03921001107977,-1.,-2.75354880060314));
#50895=CARTESIAN_POINT('Ctrl Pts',(-3.03921001107977,1.,-2.75354880060314));
#50896=CARTESIAN_POINT('Ctrl Pts',(-3.04655777351067,-1.,-2.75600247455925));
#50897=CARTESIAN_POINT('Ctrl Pts',(-3.04655777351067,1.,-2.75600247455925));
#50898=CARTESIAN_POINT('Ctrl Pts',(-3.05392498749847,-1.,-2.75842427252931));
#50899=CARTESIAN_POINT('Ctrl Pts',(-3.05392498749847,1.,-2.75842427252931));
#50900=CARTESIAN_POINT('Ctrl Pts',(-3.06131152247454,-1.,-2.76081448759882));
#50901=CARTESIAN_POINT('Ctrl Pts',(-3.06131152247454,1.,-2.76081448759882));
#50902=CARTESIAN_POINT('Ctrl Pts',(-3.0687172484321,-1.,-2.76317341453493));
#50903=CARTESIAN_POINT('Ctrl Pts',(-3.0687172484321,1.,-2.76317341453493));
#50904=CARTESIAN_POINT('Ctrl Pts',(-3.07614198408862,-1.,-2.76550131064852));
#50905=CARTESIAN_POINT('Ctrl Pts',(-3.07614198408862,1.,-2.76550131064852));
#50906=CARTESIAN_POINT('Ctrl Pts',(-3.08358548001504,-1.,-2.76779837829373));
#50907=CARTESIAN_POINT('Ctrl Pts',(-3.08358548001504,1.,-2.76779837829373));
#50908=CARTESIAN_POINT('Ctrl Pts',(-3.09104745382531,-1.,-2.7700647803451));
#50909=CARTESIAN_POINT('Ctrl Pts',(-3.09104745382531,1.,-2.7700647803451));
#50910=CARTESIAN_POINT('Ctrl Pts',(-3.0985276127786,-1.,-2.77230064796057));
#50911=CARTESIAN_POINT('Ctrl Pts',(-3.0985276127786,1.,-2.77230064796057));
#50912=CARTESIAN_POINT('Ctrl Pts',(-3.10602568032564,-1.,-2.77450609123362));
#50913=CARTESIAN_POINT('Ctrl Pts',(-3.10602568032564,1.,-2.77450609123362));
#50914=CARTESIAN_POINT('Ctrl Pts',(-3.11354142303921,-1.,-2.77668121002545));
#50915=CARTESIAN_POINT('Ctrl Pts',(-3.11354142303921,1.,-2.77668121002545));
#50916=CARTESIAN_POINT('Ctrl Pts',(-3.12107467037201,-1.,-2.77882610146731));
#50917=CARTESIAN_POINT('Ctrl Pts',(-3.12107467037201,1.,-2.77882610146731));
#50918=CARTESIAN_POINT('Ctrl Pts',(-3.12862530318457,-1.,-2.78094085161413));
#50919=CARTESIAN_POINT('Ctrl Pts',(-3.12862530318457,1.,-2.78094085161413));
#50920=CARTESIAN_POINT('Ctrl Pts',(-3.13467965833037,-1.,-2.78260859419319));
#50921=CARTESIAN_POINT('Ctrl Pts',(-3.13467965833037,1.,-2.78260859419319));
#50922=CARTESIAN_POINT('Ctrl Pts',(-3.13922819749279,-1.,-2.78384588958165));
#50923=CARTESIAN_POINT('Ctrl Pts',(-3.13922819749279,1.,-2.78384588958165));
#50924=CARTESIAN_POINT('Ctrl Pts',(-3.14226401018816,-1.,-2.7846647503589));
#50925=CARTESIAN_POINT('Ctrl Pts',(-3.14226401018816,1.,-2.7846647503589));
#50926=CARTESIAN_POINT('Ctrl Pts',(-3.14378277984898,-1.,-2.78507268004356));
#50927=CARTESIAN_POINT('Ctrl Pts',(-3.14378277984898,1.,-2.78507268004356));
#50928=CARTESIAN_POINT('',(-2.71539546306948,1.,-2.58633475774921));
#50929=CARTESIAN_POINT('Ctrl Pts',(-2.71539546306948,-1.,-2.58633475774921));
#50930=CARTESIAN_POINT('Ctrl Pts',(-2.71539546306948,-0.666666666666667,
-2.58633475774921));
#50931=CARTESIAN_POINT('Ctrl Pts',(-2.71539546306948,-0.333333333333333,
-2.58633475774921));
#50932=CARTESIAN_POINT('Ctrl Pts',(-2.71539546306948,0.333333333333333,
-2.58633475774921));
#50933=CARTESIAN_POINT('Ctrl Pts',(-2.71539546306948,0.666666666666667,
-2.58633475774921));
#50934=CARTESIAN_POINT('Ctrl Pts',(-2.71539546306948,1.,-2.58633475774921));
#50935=CARTESIAN_POINT('',(-3.14378277984898,1.,-2.78507268004356));
#50936=CARTESIAN_POINT('',(-3.14378277984898,0.,-2.78507268004356));
#50937=CARTESIAN_POINT('Ctrl Pts',(-2.71539546306948,1.,-2.58633475774921));
#50938=CARTESIAN_POINT('Ctrl Pts',(-2.71540296616024,1.,-2.58638312917167));
#50939=CARTESIAN_POINT('Ctrl Pts',(-2.71548946460575,1.,-2.58656037976753));
#50940=CARTESIAN_POINT('Ctrl Pts',(-2.71591054189786,1.,-2.58706285424357));
#50941=CARTESIAN_POINT('Ctrl Pts',(-2.71711860281815,1.,-2.58823792682672));
#50942=CARTESIAN_POINT('Ctrl Pts',(-2.71974308958086,1.,-2.59056604771971));
#50943=CARTESIAN_POINT('Ctrl Pts',(-2.72378896977134,1.,-2.59399625537278));
#50944=CARTESIAN_POINT('Ctrl Pts',(-2.7288648348152,1.,-2.59817869034746));
#50945=CARTESIAN_POINT('Ctrl Pts',(-2.73470730109615,1.,-2.60287635688728));
#50946=CARTESIAN_POINT('Ctrl Pts',(-2.7410211099909,1.,-2.60782480638448));
#50947=CARTESIAN_POINT('Ctrl Pts',(-2.74752219567252,1.,-2.61277170105813));
#50948=CARTESIAN_POINT('Ctrl Pts',(-2.7539802502603,1.,-2.61751580407667));
#50949=CARTESIAN_POINT('Ctrl Pts',(-2.76027271596686,1.,-2.62195665834605));
#50950=CARTESIAN_POINT('Ctrl Pts',(-2.76639078479021,1.,-2.62609956506355));
#50951=CARTESIAN_POINT('Ctrl Pts',(-2.77239433377921,1.,-2.63001305229625));
#50952=CARTESIAN_POINT('Ctrl Pts',(-2.77837943466449,1.,-2.63379800904599));
#50953=CARTESIAN_POINT('Ctrl Pts',(-2.78444351041571,1.,-2.637554714303));
#50954=CARTESIAN_POINT('Ctrl Pts',(-2.79064495573224,1.,-2.64134450532584));
#50955=CARTESIAN_POINT('Ctrl Pts',(-2.79698910670736,1.,-2.64517667799319));
#50956=CARTESIAN_POINT('Ctrl Pts',(-2.80345029781152,1.,-2.64902988983337));
#50957=CARTESIAN_POINT('Ctrl Pts',(-2.80998526078165,1.,-2.65286529532208));
#50958=CARTESIAN_POINT('Ctrl Pts',(-2.81654896073883,1.,-2.65664198781344));
#50959=CARTESIAN_POINT('Ctrl Pts',(-2.82311188135078,1.,-2.66033388273461));
#50960=CARTESIAN_POINT('Ctrl Pts',(-2.82966813308998,1.,-2.6639376472693));
#50961=CARTESIAN_POINT('Ctrl Pts',(-2.83622586853982,1.,-2.66746339678107));
#50962=CARTESIAN_POINT('Ctrl Pts',(-2.84280157191323,1.,-2.67092916452125));
#50963=CARTESIAN_POINT('Ctrl Pts',(-2.84941315703092,1.,-2.67435421039677));
#50964=CARTESIAN_POINT('Ctrl Pts',(-2.85607274378018,1.,-2.67775201955724));
#50965=CARTESIAN_POINT('Ctrl Pts',(-2.86278224277689,1.,-2.68112602796308));
#50966=CARTESIAN_POINT('Ctrl Pts',(-2.86953736547238,1.,-2.68447353139599));
#50967=CARTESIAN_POINT('Ctrl Pts',(-2.8763300724388,1.,-2.68778807801686));
#50968=CARTESIAN_POINT('Ctrl Pts',(-2.88315153980466,1.,-2.69106236420198));
#50969=CARTESIAN_POINT('Ctrl Pts',(-2.88999512410309,1.,-2.69429113011374));
#50970=CARTESIAN_POINT('Ctrl Pts',(-2.89685866123671,1.,-2.69747340630625));
#50971=CARTESIAN_POINT('Ctrl Pts',(-2.90374285605838,1.,-2.70061095078692));
#50972=CARTESIAN_POINT('Ctrl Pts',(-2.91065019668329,1.,-2.70370719782113));
#50973=CARTESIAN_POINT('Ctrl Pts',(-2.91758367994737,1.,-2.70676602302518));
#50974=CARTESIAN_POINT('Ctrl Pts',(-2.92454558914778,1.,-2.70979055994754));
#50975=CARTESIAN_POINT('Ctrl Pts',(-2.93153633192595,1.,-2.71278207520817));
#50976=CARTESIAN_POINT('Ctrl Pts',(-2.93855503247266,1.,-2.7157405459259));
#50977=CARTESIAN_POINT('Ctrl Pts',(-2.94560002559806,1.,-2.71866514227965));
#50978=CARTESIAN_POINT('Ctrl Pts',(-2.95266939280621,1.,-2.72155475123364));
#50979=CARTESIAN_POINT('Ctrl Pts',(-2.95976146492576,1.,-2.72440846811729));
#50980=CARTESIAN_POINT('Ctrl Pts',(-2.96687537842451,1.,-2.72722614084076));
#50981=CARTESIAN_POINT('Ctrl Pts',(-2.97401089032677,1.,-2.73000819218414));
#50982=CARTESIAN_POINT('Ctrl Pts',(-2.98116814232129,1.,-2.73275539286497));
#50983=CARTESIAN_POINT('Ctrl Pts',(-2.9883474369644,1.,-2.73546864694536));
#50984=CARTESIAN_POINT('Ctrl Pts',(-2.99554902409778,1.,-2.73814878711641));
#50985=CARTESIAN_POINT('Ctrl Pts',(-3.00277284351521,1.,-2.74079632883931));
#50986=CARTESIAN_POINT('Ctrl Pts',(-3.01001855960162,1.,-2.74341150239887));
#50987=CARTESIAN_POINT('Ctrl Pts',(-3.01728567646611,1.,-2.74599436193625));
#50988=CARTESIAN_POINT('Ctrl Pts',(-3.02457362909245,1.,-2.7485448718414));
#50989=CARTESIAN_POINT('Ctrl Pts',(-3.03188187589107,1.,-2.75106299522979));
#50990=CARTESIAN_POINT('Ctrl Pts',(-3.03921001107977,1.,-2.75354880060314));
#50991=CARTESIAN_POINT('Ctrl Pts',(-3.04655777351067,1.,-2.75600247455925));
#50992=CARTESIAN_POINT('Ctrl Pts',(-3.05392498749847,1.,-2.75842427252931));
#50993=CARTESIAN_POINT('Ctrl Pts',(-3.06131152247454,1.,-2.76081448759882));
#50994=CARTESIAN_POINT('Ctrl Pts',(-3.0687172484321,1.,-2.76317341453493));
#50995=CARTESIAN_POINT('Ctrl Pts',(-3.07614198408862,1.,-2.76550131064852));
#50996=CARTESIAN_POINT('Ctrl Pts',(-3.08358548001504,1.,-2.76779837829373));
#50997=CARTESIAN_POINT('Ctrl Pts',(-3.09104745382531,1.,-2.7700647803451));
#50998=CARTESIAN_POINT('Ctrl Pts',(-3.0985276127786,1.,-2.77230064796057));
#50999=CARTESIAN_POINT('Ctrl Pts',(-3.10602568032564,1.,-2.77450609123362));
#51000=CARTESIAN_POINT('Ctrl Pts',(-3.11354142303921,1.,-2.77668121002545));
#51001=CARTESIAN_POINT('Ctrl Pts',(-3.12107467037201,1.,-2.77882610146731));
#51002=CARTESIAN_POINT('Ctrl Pts',(-3.12862530318457,1.,-2.78094085161413));
#51003=CARTESIAN_POINT('Ctrl Pts',(-3.13467965833037,1.,-2.78260859419319));
#51004=CARTESIAN_POINT('Ctrl Pts',(-3.13922819749279,1.,-2.78384588958165));
#51005=CARTESIAN_POINT('Ctrl Pts',(-3.14226401018816,1.,-2.7846647503589));
#51006=CARTESIAN_POINT('Ctrl Pts',(-3.14378277984898,1.,-2.78507268004356));
#51007=CARTESIAN_POINT('Origin',(-3.14378277984898,0.,-2.78507268004356));
#51008=CARTESIAN_POINT('',(-3.24257979115744,1.,-2.66939624221984));
#51009=CARTESIAN_POINT('Origin',(0.,0.,0.));
#51010=CARTESIAN_POINT('',(-2.58633475775051,1.,-2.71539546306824));
#51011=CARTESIAN_POINT('Origin',(0.,1.,0.));
#51012=CARTESIAN_POINT('Ctrl Pts',(-2.58633475775051,1.,-2.71539546306824));
#51013=CARTESIAN_POINT('Ctrl Pts',(-2.58633475775051,0.666666666666667,
-2.71539546306824));
#51014=CARTESIAN_POINT('Ctrl Pts',(-2.58633475775051,0.333333333333333,
-2.71539546306824));
#51015=CARTESIAN_POINT('Ctrl Pts',(-2.58633475775051,-0.333333333333333,
-2.71539546306824));
#51016=CARTESIAN_POINT('Ctrl Pts',(-2.58633475775051,-0.666666666666667,
-2.71539546306824));
#51017=CARTESIAN_POINT('Ctrl Pts',(-2.58633475775051,-1.,-2.71539546306824));
#51018=CARTESIAN_POINT('Ctrl Pts',(-2.78507268004356,-1.,-3.14378277984898));
#51019=CARTESIAN_POINT('Ctrl Pts',(-2.78507268004356,1.,-3.14378277984898));
#51020=CARTESIAN_POINT('Ctrl Pts',(-2.78466475036183,-1.,-3.14226401019149));
#51021=CARTESIAN_POINT('Ctrl Pts',(-2.78466475036183,1.,-3.14226401019149));
#51022=CARTESIAN_POINT('Ctrl Pts',(-2.78384588958965,-1.,-3.13922819750185));
#51023=CARTESIAN_POINT('Ctrl Pts',(-2.78384588958965,1.,-3.13922819750185));
#51024=CARTESIAN_POINT('Ctrl Pts',(-2.78260859420629,-1.,-3.1346796583452));
#51025=CARTESIAN_POINT('Ctrl Pts',(-2.78260859420629,1.,-3.1346796583452));
#51026=CARTESIAN_POINT('Ctrl Pts',(-2.78094085162947,-1.,-3.12862530320194));
#51027=CARTESIAN_POINT('Ctrl Pts',(-2.78094085162947,1.,-3.12862530320194));
#51028=CARTESIAN_POINT('Ctrl Pts',(-2.77882610147986,-1.,-3.12107467038623));
#51029=CARTESIAN_POINT('Ctrl Pts',(-2.77882610147986,1.,-3.12107467038623));
#51030=CARTESIAN_POINT('Ctrl Pts',(-2.77668121003225,-1.,-3.11354142304692));
#51031=CARTESIAN_POINT('Ctrl Pts',(-2.77668121003225,1.,-3.11354142304692));
#51032=CARTESIAN_POINT('Ctrl Pts',(-2.7745060912343,-1.,-3.10602568032641));
#51033=CARTESIAN_POINT('Ctrl Pts',(-2.7745060912343,1.,-3.10602568032641));
#51034=CARTESIAN_POINT('Ctrl Pts',(-2.77230064795679,-1.,-3.09852761277432));
#51035=CARTESIAN_POINT('Ctrl Pts',(-2.77230064795679,1.,-3.09852761277432));
#51036=CARTESIAN_POINT('Ctrl Pts',(-2.77006478033937,-1.,-3.09104745381882));
#51037=CARTESIAN_POINT('Ctrl Pts',(-2.77006478033937,1.,-3.09104745381882));
#51038=CARTESIAN_POINT('Ctrl Pts',(-2.76779837828843,-1.,-3.08358548000904));
#51039=CARTESIAN_POINT('Ctrl Pts',(-2.76779837828843,1.,-3.08358548000904));
#51040=CARTESIAN_POINT('Ctrl Pts',(-2.76550131064522,-1.,-3.07614198408488));
#51041=CARTESIAN_POINT('Ctrl Pts',(-2.76550131064522,1.,-3.07614198408488));
#51042=CARTESIAN_POINT('Ctrl Pts',(-2.76317341453415,-1.,-3.06871724843121));
#51043=CARTESIAN_POINT('Ctrl Pts',(-2.76317341453415,1.,-3.06871724843121));
#51044=CARTESIAN_POINT('Ctrl Pts',(-2.76081448760011,-1.,-3.06131152247599));
#51045=CARTESIAN_POINT('Ctrl Pts',(-2.76081448760011,1.,-3.06131152247599));
#51046=CARTESIAN_POINT('Ctrl Pts',(-2.75842427253164,-1.,-3.05392498750112));
#51047=CARTESIAN_POINT('Ctrl Pts',(-2.75842427253164,1.,-3.05392498750112));
#51048=CARTESIAN_POINT('Ctrl Pts',(-2.7560024745616,-1.,-3.04655777351333));
#51049=CARTESIAN_POINT('Ctrl Pts',(-2.7560024745616,1.,-3.04655777351333));
#51050=CARTESIAN_POINT('Ctrl Pts',(-2.75354880060473,-1.,-3.03921001108158));
#51051=CARTESIAN_POINT('Ctrl Pts',(-2.75354880060473,1.,-3.03921001108158));
#51052=CARTESIAN_POINT('Ctrl Pts',(-2.75106299523032,-1.,-3.03188187589168));
#51053=CARTESIAN_POINT('Ctrl Pts',(-2.75106299523032,1.,-3.03188187589168));
#51054=CARTESIAN_POINT('Ctrl Pts',(-2.74854487184099,-1.,-3.02457362909199));
#51055=CARTESIAN_POINT('Ctrl Pts',(-2.74854487184099,1.,-3.02457362909199));
#51056=CARTESIAN_POINT('Ctrl Pts',(-2.74599436193528,-1.,-3.01728567646502));
#51057=CARTESIAN_POINT('Ctrl Pts',(-2.74599436193528,1.,-3.01728567646502));
#51058=CARTESIAN_POINT('Ctrl Pts',(-2.7434115023978,-1.,-3.01001855960041));
#51059=CARTESIAN_POINT('Ctrl Pts',(-2.7434115023978,1.,-3.01001855960041));
#51060=CARTESIAN_POINT('Ctrl Pts',(-2.74079632883852,-1.,-3.00277284351431));
#51061=CARTESIAN_POINT('Ctrl Pts',(-2.74079632883852,1.,-3.00277284351431));
#51062=CARTESIAN_POINT('Ctrl Pts',(-2.73814878711609,-1.,-2.99554902409741));
#51063=CARTESIAN_POINT('Ctrl Pts',(-2.73814878711609,1.,-2.99554902409741));
#51064=CARTESIAN_POINT('Ctrl Pts',(-2.73546864694548,-1.,-2.98834743696455));
#51065=CARTESIAN_POINT('Ctrl Pts',(-2.73546864694548,1.,-2.98834743696455));
#51066=CARTESIAN_POINT('Ctrl Pts',(-2.73275539286537,-1.,-2.98116814232175));
#51067=CARTESIAN_POINT('Ctrl Pts',(-2.73275539286537,1.,-2.98116814232175));
#51068=CARTESIAN_POINT('Ctrl Pts',(-2.7300081921846,-1.,-2.97401089032729));
#51069=CARTESIAN_POINT('Ctrl Pts',(-2.7300081921846,1.,-2.97401089032729));
#51070=CARTESIAN_POINT('Ctrl Pts',(-2.72722614084112,-1.,-2.96687537842492));
#51071=CARTESIAN_POINT('Ctrl Pts',(-2.72722614084112,1.,-2.96687537842492));
#51072=CARTESIAN_POINT('Ctrl Pts',(-2.72440846811745,-1.,-2.95976146492595));
#51073=CARTESIAN_POINT('Ctrl Pts',(-2.72440846811745,1.,-2.95976146492595));
#51074=CARTESIAN_POINT('Ctrl Pts',(-2.72155475123361,-1.,-2.95266939280617));
#51075=CARTESIAN_POINT('Ctrl Pts',(-2.72155475123361,1.,-2.95266939280617));
#51076=CARTESIAN_POINT('Ctrl Pts',(-2.71866514227952,-1.,-2.94560002559789));
#51077=CARTESIAN_POINT('Ctrl Pts',(-2.71866514227952,1.,-2.94560002559789));
#51078=CARTESIAN_POINT('Ctrl Pts',(-2.71574054592575,-1.,-2.93855503247248));
#51079=CARTESIAN_POINT('Ctrl Pts',(-2.71574054592575,1.,-2.93855503247248));
#51080=CARTESIAN_POINT('Ctrl Pts',(-2.71278207520807,-1.,-2.93153633192583));
#51081=CARTESIAN_POINT('Ctrl Pts',(-2.71278207520807,1.,-2.93153633192583));
#51082=CARTESIAN_POINT('Ctrl Pts',(-2.70979055994751,-1.,-2.92454558914774));
#51083=CARTESIAN_POINT('Ctrl Pts',(-2.70979055994751,1.,-2.92454558914774));
#51084=CARTESIAN_POINT('Ctrl Pts',(-2.70676602302518,-1.,-2.91758367994738));
#51085=CARTESIAN_POINT('Ctrl Pts',(-2.70676602302518,1.,-2.91758367994738));
#51086=CARTESIAN_POINT('Ctrl Pts',(-2.70370719782114,-1.,-2.91065019668331));
#51087=CARTESIAN_POINT('Ctrl Pts',(-2.70370719782114,1.,-2.91065019668331));
#51088=CARTESIAN_POINT('Ctrl Pts',(-2.70061095078692,-1.,-2.90374285605839));
#51089=CARTESIAN_POINT('Ctrl Pts',(-2.70061095078692,1.,-2.90374285605839));
#51090=CARTESIAN_POINT('Ctrl Pts',(-2.69747340630621,-1.,-2.89685866123668));
#51091=CARTESIAN_POINT('Ctrl Pts',(-2.69747340630621,1.,-2.89685866123668));
#51092=CARTESIAN_POINT('Ctrl Pts',(-2.69429113011369,-1.,-2.88999512410304));
#51093=CARTESIAN_POINT('Ctrl Pts',(-2.69429113011369,1.,-2.88999512410304));
#51094=CARTESIAN_POINT('Ctrl Pts',(-2.69106236420197,-1.,-2.88315153980464));
#51095=CARTESIAN_POINT('Ctrl Pts',(-2.69106236420197,1.,-2.88315153980464));
#51096=CARTESIAN_POINT('Ctrl Pts',(-2.68778807801691,-1.,-2.87633007243885));
#51097=CARTESIAN_POINT('Ctrl Pts',(-2.68778807801691,1.,-2.87633007243885));
#51098=CARTESIAN_POINT('Ctrl Pts',(-2.68447353139611,-1.,-2.8695373654725));
#51099=CARTESIAN_POINT('Ctrl Pts',(-2.68447353139611,1.,-2.8695373654725));
#51100=CARTESIAN_POINT('Ctrl Pts',(-2.68112602796323,-1.,-2.86278224277705));
#51101=CARTESIAN_POINT('Ctrl Pts',(-2.68112602796323,1.,-2.86278224277705));
#51102=CARTESIAN_POINT('Ctrl Pts',(-2.67775201955736,-1.,-2.85607274378031));
#51103=CARTESIAN_POINT('Ctrl Pts',(-2.67775201955736,1.,-2.85607274378031));
#51104=CARTESIAN_POINT('Ctrl Pts',(-2.67435421039682,-1.,-2.84941315703096));
#51105=CARTESIAN_POINT('Ctrl Pts',(-2.67435421039682,1.,-2.84941315703096));
#51106=CARTESIAN_POINT('Ctrl Pts',(-2.67092916452117,-1.,-2.84280157191314));
#51107=CARTESIAN_POINT('Ctrl Pts',(-2.67092916452117,1.,-2.84280157191314));
#51108=CARTESIAN_POINT('Ctrl Pts',(-2.66746339678085,-1.,-2.8362258685396));
#51109=CARTESIAN_POINT('Ctrl Pts',(-2.66746339678085,1.,-2.8362258685396));
#51110=CARTESIAN_POINT('Ctrl Pts',(-2.66393764726902,-1.,-2.82966813308969));
#51111=CARTESIAN_POINT('Ctrl Pts',(-2.66393764726902,1.,-2.82966813308969));
#51112=CARTESIAN_POINT('Ctrl Pts',(-2.66033388273437,-1.,-2.82311188135053));
#51113=CARTESIAN_POINT('Ctrl Pts',(-2.66033388273437,1.,-2.82311188135053));
#51114=CARTESIAN_POINT('Ctrl Pts',(-2.65664198781335,-1.,-2.81654896073874));
#51115=CARTESIAN_POINT('Ctrl Pts',(-2.65664198781335,1.,-2.81654896073874));
#51116=CARTESIAN_POINT('Ctrl Pts',(-2.65286529532221,-1.,-2.80998526078179));
#51117=CARTESIAN_POINT('Ctrl Pts',(-2.65286529532221,1.,-2.80998526078179));
#51118=CARTESIAN_POINT('Ctrl Pts',(-2.64902988983373,-1.,-2.80345029781191));
#51119=CARTESIAN_POINT('Ctrl Pts',(-2.64902988983373,1.,-2.80345029781191));
#51120=CARTESIAN_POINT('Ctrl Pts',(-2.6451766779937,-1.,-2.7969891067079));
#51121=CARTESIAN_POINT('Ctrl Pts',(-2.6451766779937,1.,-2.7969891067079));
#51122=CARTESIAN_POINT('Ctrl Pts',(-2.64134450532632,-1.,-2.79064495573275));
#51123=CARTESIAN_POINT('Ctrl Pts',(-2.64134450532632,1.,-2.79064495573275));
#51124=CARTESIAN_POINT('Ctrl Pts',(-2.63755471430322,-1.,-2.78444351041594));
#51125=CARTESIAN_POINT('Ctrl Pts',(-2.63755471430322,1.,-2.78444351041594));
#51126=CARTESIAN_POINT('Ctrl Pts',(-2.63379800904575,-1.,-2.77837943466423));
#51127=CARTESIAN_POINT('Ctrl Pts',(-2.63379800904575,1.,-2.77837943466423));
#51128=CARTESIAN_POINT('Ctrl Pts',(-2.63001305229548,-1.,-2.77239433377839));
#51129=CARTESIAN_POINT('Ctrl Pts',(-2.63001305229548,1.,-2.77239433377839));
#51130=CARTESIAN_POINT('Ctrl Pts',(-2.6260995650624,-1.,-2.76639078478898));
#51131=CARTESIAN_POINT('Ctrl Pts',(-2.6260995650624,1.,-2.76639078478898));
#51132=CARTESIAN_POINT('Ctrl Pts',(-2.62195665834491,-1.,-2.76027271596564));
#51133=CARTESIAN_POINT('Ctrl Pts',(-2.62195665834491,1.,-2.76027271596564));
#51134=CARTESIAN_POINT('Ctrl Pts',(-2.61751580407608,-1.,-2.75398025025967));
#51135=CARTESIAN_POINT('Ctrl Pts',(-2.61751580407608,1.,-2.75398025025967));
#51136=CARTESIAN_POINT('Ctrl Pts',(-2.61277170105864,-1.,-2.74752219567307));
#51137=CARTESIAN_POINT('Ctrl Pts',(-2.61277170105864,1.,-2.74752219567307));
#51138=CARTESIAN_POINT('Ctrl Pts',(-2.60782480638629,-1.,-2.74102110999284));
#51139=CARTESIAN_POINT('Ctrl Pts',(-2.60782480638629,1.,-2.74102110999284));
#51140=CARTESIAN_POINT('Ctrl Pts',(-2.60287635689,-1.,-2.73470730109906));
#51141=CARTESIAN_POINT('Ctrl Pts',(-2.60287635689,1.,-2.73470730109906));
#51142=CARTESIAN_POINT('Ctrl Pts',(-2.5981786903501,-1.,-2.72886483481804));
#51143=CARTESIAN_POINT('Ctrl Pts',(-2.5981786903501,1.,-2.72886483481804));
#51144=CARTESIAN_POINT('Ctrl Pts',(-2.59399625537407,-1.,-2.72378896977273));
#51145=CARTESIAN_POINT('Ctrl Pts',(-2.59399625537407,1.,-2.72378896977273));
#51146=CARTESIAN_POINT('Ctrl Pts',(-2.59056604771863,-1.,-2.7197430895797));
#51147=CARTESIAN_POINT('Ctrl Pts',(-2.59056604771863,1.,-2.7197430895797));
#51148=CARTESIAN_POINT('Ctrl Pts',(-2.58804906785078,-1.,-2.71690570241274));
#51149=CARTESIAN_POINT('Ctrl Pts',(-2.58804906785078,1.,-2.71690570241274));
#51150=CARTESIAN_POINT('Ctrl Pts',(-2.58682657352212,-1.,-2.71566956750046));
#51151=CARTESIAN_POINT('Ctrl Pts',(-2.58682657352212,1.,-2.71566956750046));
#51152=CARTESIAN_POINT('Ctrl Pts',(-2.58636629903847,-1.,-2.71533674140979));
#51153=CARTESIAN_POINT('Ctrl Pts',(-2.58636629903847,1.,-2.71533674140979));
#51154=CARTESIAN_POINT('Ctrl Pts',(-2.58626222935706,-1.,-2.71537879705));
#51155=CARTESIAN_POINT('Ctrl Pts',(-2.58626222935706,1.,-2.71537879705));
#51156=CARTESIAN_POINT('Ctrl Pts',(-2.58626089374824,-1.,-2.71546581445404));
#51157=CARTESIAN_POINT('Ctrl Pts',(-2.58626089374824,1.,-2.71546581445404));
#51158=CARTESIAN_POINT('',(-2.78507268004356,1.,-3.14378277984898));
#51159=CARTESIAN_POINT('Ctrl Pts',(-2.78507268004356,1.,-3.14378277984898));
#51160=CARTESIAN_POINT('Ctrl Pts',(-2.78466475036183,1.,-3.14226401019149));
#51161=CARTESIAN_POINT('Ctrl Pts',(-2.78384588958965,1.,-3.13922819750185));
#51162=CARTESIAN_POINT('Ctrl Pts',(-2.78260859420629,1.,-3.1346796583452));
#51163=CARTESIAN_POINT('Ctrl Pts',(-2.78094085162947,1.,-3.12862530320194));
#51164=CARTESIAN_POINT('Ctrl Pts',(-2.77882610147986,1.,-3.12107467038623));
#51165=CARTESIAN_POINT('Ctrl Pts',(-2.77668121003225,1.,-3.11354142304692));
#51166=CARTESIAN_POINT('Ctrl Pts',(-2.7745060912343,1.,-3.10602568032641));
#51167=CARTESIAN_POINT('Ctrl Pts',(-2.77230064795679,1.,-3.09852761277432));
#51168=CARTESIAN_POINT('Ctrl Pts',(-2.77006478033937,1.,-3.09104745381882));
#51169=CARTESIAN_POINT('Ctrl Pts',(-2.76779837828843,1.,-3.08358548000904));
#51170=CARTESIAN_POINT('Ctrl Pts',(-2.76550131064522,1.,-3.07614198408488));
#51171=CARTESIAN_POINT('Ctrl Pts',(-2.76317341453415,1.,-3.06871724843121));
#51172=CARTESIAN_POINT('Ctrl Pts',(-2.76081448760011,1.,-3.06131152247599));
#51173=CARTESIAN_POINT('Ctrl Pts',(-2.75842427253164,1.,-3.05392498750112));
#51174=CARTESIAN_POINT('Ctrl Pts',(-2.7560024745616,1.,-3.04655777351333));
#51175=CARTESIAN_POINT('Ctrl Pts',(-2.75354880060473,1.,-3.03921001108158));
#51176=CARTESIAN_POINT('Ctrl Pts',(-2.75106299523032,1.,-3.03188187589168));
#51177=CARTESIAN_POINT('Ctrl Pts',(-2.74854487184099,1.,-3.02457362909199));
#51178=CARTESIAN_POINT('Ctrl Pts',(-2.74599436193528,1.,-3.01728567646502));
#51179=CARTESIAN_POINT('Ctrl Pts',(-2.7434115023978,1.,-3.01001855960041));
#51180=CARTESIAN_POINT('Ctrl Pts',(-2.74079632883852,1.,-3.00277284351431));
#51181=CARTESIAN_POINT('Ctrl Pts',(-2.73814878711609,1.,-2.99554902409741));
#51182=CARTESIAN_POINT('Ctrl Pts',(-2.73546864694548,1.,-2.98834743696455));
#51183=CARTESIAN_POINT('Ctrl Pts',(-2.73275539286537,1.,-2.98116814232175));
#51184=CARTESIAN_POINT('Ctrl Pts',(-2.7300081921846,1.,-2.97401089032729));
#51185=CARTESIAN_POINT('Ctrl Pts',(-2.72722614084112,1.,-2.96687537842492));
#51186=CARTESIAN_POINT('Ctrl Pts',(-2.72440846811745,1.,-2.95976146492595));
#51187=CARTESIAN_POINT('Ctrl Pts',(-2.72155475123361,1.,-2.95266939280617));
#51188=CARTESIAN_POINT('Ctrl Pts',(-2.71866514227952,1.,-2.94560002559789));
#51189=CARTESIAN_POINT('Ctrl Pts',(-2.71574054592575,1.,-2.93855503247248));
#51190=CARTESIAN_POINT('Ctrl Pts',(-2.71278207520807,1.,-2.93153633192583));
#51191=CARTESIAN_POINT('Ctrl Pts',(-2.70979055994751,1.,-2.92454558914774));
#51192=CARTESIAN_POINT('Ctrl Pts',(-2.70676602302518,1.,-2.91758367994738));
#51193=CARTESIAN_POINT('Ctrl Pts',(-2.70370719782114,1.,-2.91065019668331));
#51194=CARTESIAN_POINT('Ctrl Pts',(-2.70061095078692,1.,-2.90374285605839));
#51195=CARTESIAN_POINT('Ctrl Pts',(-2.69747340630621,1.,-2.89685866123668));
#51196=CARTESIAN_POINT('Ctrl Pts',(-2.69429113011369,1.,-2.88999512410304));
#51197=CARTESIAN_POINT('Ctrl Pts',(-2.69106236420197,1.,-2.88315153980464));
#51198=CARTESIAN_POINT('Ctrl Pts',(-2.68778807801691,1.,-2.87633007243885));
#51199=CARTESIAN_POINT('Ctrl Pts',(-2.68447353139611,1.,-2.8695373654725));
#51200=CARTESIAN_POINT('Ctrl Pts',(-2.68112602796323,1.,-2.86278224277705));
#51201=CARTESIAN_POINT('Ctrl Pts',(-2.67775201955736,1.,-2.85607274378031));
#51202=CARTESIAN_POINT('Ctrl Pts',(-2.67435421039682,1.,-2.84941315703096));
#51203=CARTESIAN_POINT('Ctrl Pts',(-2.67092916452117,1.,-2.84280157191314));
#51204=CARTESIAN_POINT('Ctrl Pts',(-2.66746339678085,1.,-2.8362258685396));
#51205=CARTESIAN_POINT('Ctrl Pts',(-2.66393764726902,1.,-2.82966813308969));
#51206=CARTESIAN_POINT('Ctrl Pts',(-2.66033388273437,1.,-2.82311188135053));
#51207=CARTESIAN_POINT('Ctrl Pts',(-2.65664198781335,1.,-2.81654896073874));
#51208=CARTESIAN_POINT('Ctrl Pts',(-2.65286529532221,1.,-2.80998526078179));
#51209=CARTESIAN_POINT('Ctrl Pts',(-2.64902988983373,1.,-2.80345029781191));
#51210=CARTESIAN_POINT('Ctrl Pts',(-2.6451766779937,1.,-2.7969891067079));
#51211=CARTESIAN_POINT('Ctrl Pts',(-2.64134450532632,1.,-2.79064495573275));
#51212=CARTESIAN_POINT('Ctrl Pts',(-2.63755471430322,1.,-2.78444351041594));
#51213=CARTESIAN_POINT('Ctrl Pts',(-2.63379800904575,1.,-2.77837943466423));
#51214=CARTESIAN_POINT('Ctrl Pts',(-2.63001305229548,1.,-2.77239433377839));
#51215=CARTESIAN_POINT('Ctrl Pts',(-2.6260995650624,1.,-2.76639078478898));
#51216=CARTESIAN_POINT('Ctrl Pts',(-2.62195665834491,1.,-2.76027271596564));
#51217=CARTESIAN_POINT('Ctrl Pts',(-2.61751580407608,1.,-2.75398025025967));
#51218=CARTESIAN_POINT('Ctrl Pts',(-2.61277170105864,1.,-2.74752219567307));
#51219=CARTESIAN_POINT('Ctrl Pts',(-2.60782480638629,1.,-2.74102110999284));
#51220=CARTESIAN_POINT('Ctrl Pts',(-2.60287635689,1.,-2.73470730109906));
#51221=CARTESIAN_POINT('Ctrl Pts',(-2.5981786903501,1.,-2.72886483481804));
#51222=CARTESIAN_POINT('Ctrl Pts',(-2.59399625537407,1.,-2.72378896977273));
#51223=CARTESIAN_POINT('Ctrl Pts',(-2.59056604771863,1.,-2.7197430895797));
#51224=CARTESIAN_POINT('Ctrl Pts',(-2.58823792682724,1.,-2.7171186028189));
#51225=CARTESIAN_POINT('Ctrl Pts',(-2.58706285424469,1.,-2.71591054189884));
#51226=CARTESIAN_POINT('Ctrl Pts',(-2.58656037976884,1.,-2.71548946460616));
#51227=CARTESIAN_POINT('Ctrl Pts',(-2.58638312917291,1.,-2.71540296615967));
#51228=CARTESIAN_POINT('Ctrl Pts',(-2.58633475775051,1.,-2.71539546306824));
#51229=CARTESIAN_POINT('',(-2.78507268004356,0.,-3.14378277984898));
#51230=CARTESIAN_POINT('Ctrl Pts',(-2.27745358485296,-1.,-2.97921217251145));
#51231=CARTESIAN_POINT('Ctrl Pts',(-2.27745358485296,1.,-2.97921217251145));
#51232=CARTESIAN_POINT('Ctrl Pts',(-2.27736742984319,-1.,-2.97919987915679));
#51233=CARTESIAN_POINT('Ctrl Pts',(-2.27736742984319,1.,-2.97919987915679));
#51234=CARTESIAN_POINT('Ctrl Pts',(-2.2773096118942,-1.,-2.97929608861798));
#51235=CARTESIAN_POINT('Ctrl Pts',(-2.2773096118942,1.,-2.97929608861798));
#51236=CARTESIAN_POINT('Ctrl Pts',(-2.27756633755188,-1.,-2.97980276183181));
#51237=CARTESIAN_POINT('Ctrl Pts',(-2.27756633755188,1.,-2.97980276183181));
#51238=CARTESIAN_POINT('Ctrl Pts',(-2.27859601334547,-1.,-2.98120357932994));
#51239=CARTESIAN_POINT('Ctrl Pts',(-2.27859601334547,1.,-2.98120357932994));
#51240=CARTESIAN_POINT('Ctrl Pts',(-2.28100472516679,-1.,-2.98413343613983));
#51241=CARTESIAN_POINT('Ctrl Pts',(-2.28100472516679,1.,-2.98413343613983));
#51242=CARTESIAN_POINT('Ctrl Pts',(-2.28446419115919,-1.,-2.9881543273478));
#51243=CARTESIAN_POINT('Ctrl Pts',(-2.28446419115919,1.,-2.9881543273478));
#51244=CARTESIAN_POINT('Ctrl Pts',(-2.28882328690362,-1.,-2.99307930984034));
#51245=CARTESIAN_POINT('Ctrl Pts',(-2.28882328690362,1.,-2.99307930984034));
#51246=CARTESIAN_POINT('Ctrl Pts',(-2.29385894577754,-1.,-2.99863310339691));
#51247=CARTESIAN_POINT('Ctrl Pts',(-2.29385894577754,1.,-2.99863310339691));
#51248=CARTESIAN_POINT('Ctrl Pts',(-2.29932091315775,-1.,-3.00450832658613));
#51249=CARTESIAN_POINT('Ctrl Pts',(-2.29932091315775,1.,-3.00450832658613));
#51250=CARTESIAN_POINT('Ctrl Pts',(-2.30496809486482,-1.,-3.01041131063823));
#51251=CARTESIAN_POINT('Ctrl Pts',(-2.30496809486482,1.,-3.01041131063823));
#51252=CARTESIAN_POINT('Ctrl Pts',(-2.31060449886629,-1.,-3.01610726819086));
#51253=CARTESIAN_POINT('Ctrl Pts',(-2.31060449886629,1.,-3.01610726819086));
#51254=CARTESIAN_POINT('Ctrl Pts',(-2.31612479121631,-1.,-3.02147780668161));
#51255=CARTESIAN_POINT('Ctrl Pts',(-2.31612479121631,1.,-3.02147780668161));
#51256=CARTESIAN_POINT('Ctrl Pts',(-2.32151944306402,-1.,-3.02652678416611));
#51257=CARTESIAN_POINT('Ctrl Pts',(-2.32151944306402,1.,-3.02652678416611));
#51258=CARTESIAN_POINT('Ctrl Pts',(-2.32683687412097,-1.,-3.03133125185136));
#51259=CARTESIAN_POINT('Ctrl Pts',(-2.32683687412097,1.,-3.03133125185136));
#51260=CARTESIAN_POINT('Ctrl Pts',(-2.33215619079829,-1.,-3.03600588555793));
#51261=CARTESIAN_POINT('Ctrl Pts',(-2.33215619079829,1.,-3.03600588555793));
#51262=CARTESIAN_POINT('Ctrl Pts',(-2.33755792953706,-1.,-3.04066496998544));
#51263=CARTESIAN_POINT('Ctrl Pts',(-2.33755792953706,1.,-3.04066496998544));
#51264=CARTESIAN_POINT('Ctrl Pts',(-2.34309017083977,-1.,-3.04537822217256));
#51265=CARTESIAN_POINT('Ctrl Pts',(-2.34309017083977,1.,-3.04537822217256));
#51266=CARTESIAN_POINT('Ctrl Pts',(-2.34875673090771,-1.,-3.05015565829918));
#51267=CARTESIAN_POINT('Ctrl Pts',(-2.34875673090771,1.,-3.05015565829918));
#51268=CARTESIAN_POINT('Ctrl Pts',(-2.35453559889474,-1.,-3.05497218368146));
#51269=CARTESIAN_POINT('Ctrl Pts',(-2.35453559889474,1.,-3.05497218368146));
#51270=CARTESIAN_POINT('Ctrl Pts',(-2.36039011602072,-1.,-3.0597826624004));
#51271=CARTESIAN_POINT('Ctrl Pts',(-2.36039011602072,1.,-3.0597826624004));
#51272=CARTESIAN_POINT('Ctrl Pts',(-2.36628220107009,-1.,-3.06453964643162));
#51273=CARTESIAN_POINT('Ctrl Pts',(-2.36628220107009,1.,-3.06453964643162));
#51274=CARTESIAN_POINT('Ctrl Pts',(-2.37218678163178,-1.,-3.069212754975));
#51275=CARTESIAN_POINT('Ctrl Pts',(-2.37218678163178,1.,-3.069212754975));
#51276=CARTESIAN_POINT('Ctrl Pts',(-2.37809856205548,-1.,-3.07379777492165));
#51277=CARTESIAN_POINT('Ctrl Pts',(-2.37809856205548,1.,-3.07379777492165));
#51278=CARTESIAN_POINT('Ctrl Pts',(-2.38402401216126,-1.,-3.07830597244326));
#51279=CARTESIAN_POINT('Ctrl Pts',(-2.38402401216126,1.,-3.07830597244326));
#51280=CARTESIAN_POINT('Ctrl Pts',(-2.38997659219199,-1.,-3.08275773747093));
#51281=CARTESIAN_POINT('Ctrl Pts',(-2.38997659219199,1.,-3.08275773747093));
#51282=CARTESIAN_POINT('Ctrl Pts',(-2.39597098250631,-1.,-3.08717489512914));
#51283=CARTESIAN_POINT('Ctrl Pts',(-2.39597098250631,1.,-3.08717489512914));
#51284=CARTESIAN_POINT('Ctrl Pts',(-2.40201704423341,-1.,-3.091572660511));
#51285=CARTESIAN_POINT('Ctrl Pts',(-2.40201704423341,1.,-3.091572660511));
#51286=CARTESIAN_POINT('Ctrl Pts',(-2.40811612696369,-1.,-3.09595472616076));
#51287=CARTESIAN_POINT('Ctrl Pts',(-2.40811612696369,1.,-3.09595472616076));
#51288=CARTESIAN_POINT('Ctrl Pts',(-2.41426441798057,-1.,-3.1003177502767));
#51289=CARTESIAN_POINT('Ctrl Pts',(-2.41426441798057,1.,-3.1003177502767));
#51290=CARTESIAN_POINT('Ctrl Pts',(-2.42045498612489,-1.,-3.10465410280896));
#51291=CARTESIAN_POINT('Ctrl Pts',(-2.42045498612489,1.,-3.10465410280896));
#51292=CARTESIAN_POINT('Ctrl Pts',(-2.42668025870015,-1.,-3.10895518969595));
#51293=CARTESIAN_POINT('Ctrl Pts',(-2.42668025870015,1.,-3.10895518969595));
#51294=CARTESIAN_POINT('Ctrl Pts',(-2.43293449685144,-1.,-3.11321477659018));
#51295=CARTESIAN_POINT('Ctrl Pts',(-2.43293449685144,1.,-3.11321477659018));
#51296=CARTESIAN_POINT('Ctrl Pts',(-2.43921571477977,-1.,-3.11743156744186));
#51297=CARTESIAN_POINT('Ctrl Pts',(-2.43921571477977,1.,-3.11743156744186));
#51298=CARTESIAN_POINT('Ctrl Pts',(-2.44552433364715,-1.,-3.12160740887768));
#51299=CARTESIAN_POINT('Ctrl Pts',(-2.44552433364715,1.,-3.12160740887768));
#51300=CARTESIAN_POINT('Ctrl Pts',(-2.45186227369846,-1.,-3.12574608210847));
#51301=CARTESIAN_POINT('Ctrl Pts',(-2.45186227369846,1.,-3.12574608210847));
#51302=CARTESIAN_POINT('Ctrl Pts',(-2.45823188859366,-1.,-3.12985188384371));
#51303=CARTESIAN_POINT('Ctrl Pts',(-2.45823188859366,1.,-3.12985188384371));
#51304=CARTESIAN_POINT('Ctrl Pts',(-2.46463494332374,-1.,-3.13392826623906));
#51305=CARTESIAN_POINT('Ctrl Pts',(-2.46463494332374,1.,-3.13392826623906));
#51306=CARTESIAN_POINT('Ctrl Pts',(-2.47107164236838,-1.,-3.13797654408943));
#51307=CARTESIAN_POINT('Ctrl Pts',(-2.47107164236838,1.,-3.13797654408943));
#51308=CARTESIAN_POINT('Ctrl Pts',(-2.47754112428043,-1.,-3.14199655778863));
#51309=CARTESIAN_POINT('Ctrl Pts',(-2.47754112428043,1.,-3.14199655778863));
#51310=CARTESIAN_POINT('Ctrl Pts',(-2.4840418741839,-1.,-3.14598722723896));
#51311=CARTESIAN_POINT('Ctrl Pts',(-2.4840418741839,1.,-3.14598722723896));
#51312=CARTESIAN_POINT('Ctrl Pts',(-2.49057217131988,-1.,-3.14994715298907));
#51313=CARTESIAN_POINT('Ctrl Pts',(-2.49057217131988,1.,-3.14994715298907));
#51314=CARTESIAN_POINT('Ctrl Pts',(-2.49713050858896,-1.,-3.15387518039046));
#51315=CARTESIAN_POINT('Ctrl Pts',(-2.49713050858896,1.,-3.15387518039046));
#51316=CARTESIAN_POINT('Ctrl Pts',(-2.50371605688252,-1.,-3.15777102413957));
#51317=CARTESIAN_POINT('Ctrl Pts',(-2.50371605688252,1.,-3.15777102413957));
#51318=CARTESIAN_POINT('Ctrl Pts',(-2.51032851007894,-1.,-3.16163506380157));
#51319=CARTESIAN_POINT('Ctrl Pts',(-2.51032851007894,1.,-3.16163506380157));
#51320=CARTESIAN_POINT('Ctrl Pts',(-2.51696788755577,-1.,-3.16546808277023));
#51321=CARTESIAN_POINT('Ctrl Pts',(-2.51696788755577,1.,-3.16546808277023));
#51322=CARTESIAN_POINT('Ctrl Pts',(-2.52363434671788,-1.,-3.16927102130736));
#51323=CARTESIAN_POINT('Ctrl Pts',(-2.52363434671788,1.,-3.16927102130736));
#51324=CARTESIAN_POINT('Ctrl Pts',(-2.53032800406941,-1.,-3.17304474093612));
#51325=CARTESIAN_POINT('Ctrl Pts',(-2.53032800406941,1.,-3.17304474093612));
#51326=CARTESIAN_POINT('Ctrl Pts',(-2.53704871950948,-1.,-3.17678974135318));
#51327=CARTESIAN_POINT('Ctrl Pts',(-2.53704871950948,1.,-3.17678974135318));
#51328=CARTESIAN_POINT('Ctrl Pts',(-2.54379612553051,-1.,-3.1805061975064));
#51329=CARTESIAN_POINT('Ctrl Pts',(-2.54379612553051,1.,-3.1805061975064));
#51330=CARTESIAN_POINT('Ctrl Pts',(-2.55056972387731,-1.,-3.18419408529594));
#51331=CARTESIAN_POINT('Ctrl Pts',(-2.55056972387731,1.,-3.18419408529594));
#51332=CARTESIAN_POINT('Ctrl Pts',(-2.55736896206056,-1.,-3.18785328116218));
#51333=CARTESIAN_POINT('Ctrl Pts',(-2.55736896206056,1.,-3.18785328116218));
#51334=CARTESIAN_POINT('Ctrl Pts',(-2.56419331092858,-1.,-3.19148366395139));
#51335=CARTESIAN_POINT('Ctrl Pts',(-2.56419331092858,1.,-3.19148366395139));
#51336=CARTESIAN_POINT('Ctrl Pts',(-2.57104235897899,-1.,-3.19508523784363));
#51337=CARTESIAN_POINT('Ctrl Pts',(-2.57104235897899,1.,-3.19508523784363));
#51338=CARTESIAN_POINT('Ctrl Pts',(-2.57791581908875,-1.,-3.19865814628682));
#51339=CARTESIAN_POINT('Ctrl Pts',(-2.57791581908875,1.,-3.19865814628682));
#51340=CARTESIAN_POINT('Ctrl Pts',(-2.58481347777729,-1.,-3.20220261408414));
#51341=CARTESIAN_POINT('Ctrl Pts',(-2.58481347777729,1.,-3.20220261408414));
#51342=CARTESIAN_POINT('Ctrl Pts',(-2.59173516023481,-1.,-3.2057189102873));
#51343=CARTESIAN_POINT('Ctrl Pts',(-2.59173516023481,1.,-3.2057189102873));
#51344=CARTESIAN_POINT('Ctrl Pts',(-2.59868069194342,-1.,-3.20920730569681));
#51345=CARTESIAN_POINT('Ctrl Pts',(-2.59868069194342,1.,-3.20920730569681));
#51346=CARTESIAN_POINT('Ctrl Pts',(-2.60564985360017,-1.,-3.21266802609682));
#51347=CARTESIAN_POINT('Ctrl Pts',(-2.60564985360017,1.,-3.21266802609682));
#51348=CARTESIAN_POINT('Ctrl Pts',(-2.61264236719171,-1.,-3.21610123233082));
#51349=CARTESIAN_POINT('Ctrl Pts',(-2.61264236719171,1.,-3.21610123233082));
#51350=CARTESIAN_POINT('Ctrl Pts',(-2.61965792832947,-1.,-3.21950704109321));
#51351=CARTESIAN_POINT('Ctrl Pts',(-2.61965792832947,1.,-3.21950704109321));
#51352=CARTESIAN_POINT('Ctrl Pts',(-2.62669622735912,-1.,-3.2228855361324));
#51353=CARTESIAN_POINT('Ctrl Pts',(-2.62669622735912,1.,-3.2228855361324));
#51354=CARTESIAN_POINT('Ctrl Pts',(-2.63375697391372,-1.,-3.2262367829246));
#51355=CARTESIAN_POINT('Ctrl Pts',(-2.63375697391372,1.,-3.2262367829246));
#51356=CARTESIAN_POINT('Ctrl Pts',(-2.64083992181823,-1.,-3.22956084358547));
#51357=CARTESIAN_POINT('Ctrl Pts',(-2.64083992181823,1.,-3.22956084358547));
#51358=CARTESIAN_POINT('Ctrl Pts',(-2.64794488743038,-1.,-3.23285778737096));
#51359=CARTESIAN_POINT('Ctrl Pts',(-2.64794488743038,1.,-3.23285778737096));
#51360=CARTESIAN_POINT('Ctrl Pts',(-2.65507173961555,-1.,-3.236127680639));
#51361=CARTESIAN_POINT('Ctrl Pts',(-2.65507173961555,1.,-3.236127680639));
#51362=CARTESIAN_POINT('Ctrl Pts',(-2.6607906631847,-1.,-3.23872200034785));
#51363=CARTESIAN_POINT('Ctrl Pts',(-2.6607906631847,1.,-3.23872200034785));
#51364=CARTESIAN_POINT('Ctrl Pts',(-2.66508964663997,-1.,-3.24065561086749));
#51365=CARTESIAN_POINT('Ctrl Pts',(-2.66508964663997,1.,-3.24065561086749));
#51366=CARTESIAN_POINT('Ctrl Pts',(-2.66795998539579,-1.,-3.24193929584471));
#51367=CARTESIAN_POINT('Ctrl Pts',(-2.66795998539579,1.,-3.24193929584471));
#51368=CARTESIAN_POINT('Ctrl Pts',(-2.66939624221984,-1.,-3.24257979115744));
#51369=CARTESIAN_POINT('Ctrl Pts',(-2.66939624221984,1.,-3.24257979115744));
#51370=CARTESIAN_POINT('',(-2.27737254473521,1.,-2.97927412174279));
#51371=CARTESIAN_POINT('Ctrl Pts',(-2.27737254473521,-1.,-2.97927412174279));
#51372=CARTESIAN_POINT('Ctrl Pts',(-2.27737254473521,-0.666666666666667,
-2.97927412174279));
#51373=CARTESIAN_POINT('Ctrl Pts',(-2.27737254473521,-0.333333333333333,
-2.97927412174279));
#51374=CARTESIAN_POINT('Ctrl Pts',(-2.27737254473521,0.333333333333333,
-2.97927412174279));
#51375=CARTESIAN_POINT('Ctrl Pts',(-2.27737254473521,0.666666666666667,
-2.97927412174279));
#51376=CARTESIAN_POINT('Ctrl Pts',(-2.27737254473521,1.,-2.97927412174279));
#51377=CARTESIAN_POINT('',(-2.66939624221984,1.,-3.24257979115744));
#51378=CARTESIAN_POINT('',(-2.66939624221984,0.,-3.24257979115744));
#51379=CARTESIAN_POINT('Ctrl Pts',(-2.27737254473521,1.,-2.97927412174279));
#51380=CARTESIAN_POINT('Ctrl Pts',(-2.27737238849288,1.,-2.97932307137477));
#51381=CARTESIAN_POINT('Ctrl Pts',(-2.27743009389684,1.,-2.9795116710597));
#51382=CARTESIAN_POINT('Ctrl Pts',(-2.27776738270289,1.,-2.98007383024208));
#51383=CARTESIAN_POINT('Ctrl Pts',(-2.27877674853766,1.,-2.9814234180956));
#51384=CARTESIAN_POINT('Ctrl Pts',(-2.28100472516679,1.,-2.98413343613983));
#51385=CARTESIAN_POINT('Ctrl Pts',(-2.28446419115919,1.,-2.9881543273478));
#51386=CARTESIAN_POINT('Ctrl Pts',(-2.28882328690362,1.,-2.99307930984034));
#51387=CARTESIAN_POINT('Ctrl Pts',(-2.29385894577754,1.,-2.99863310339691));
#51388=CARTESIAN_POINT('Ctrl Pts',(-2.29932091315775,1.,-3.00450832658613));
#51389=CARTESIAN_POINT('Ctrl Pts',(-2.30496809486482,1.,-3.01041131063823));
#51390=CARTESIAN_POINT('Ctrl Pts',(-2.31060449886629,1.,-3.01610726819086));
#51391=CARTESIAN_POINT('Ctrl Pts',(-2.31612479121631,1.,-3.02147780668161));
#51392=CARTESIAN_POINT('Ctrl Pts',(-2.32151944306402,1.,-3.02652678416611));
#51393=CARTESIAN_POINT('Ctrl Pts',(-2.32683687412097,1.,-3.03133125185136));
#51394=CARTESIAN_POINT('Ctrl Pts',(-2.33215619079829,1.,-3.03600588555793));
#51395=CARTESIAN_POINT('Ctrl Pts',(-2.33755792953706,1.,-3.04066496998544));
#51396=CARTESIAN_POINT('Ctrl Pts',(-2.34309017083977,1.,-3.04537822217256));
#51397=CARTESIAN_POINT('Ctrl Pts',(-2.34875673090771,1.,-3.05015565829918));
#51398=CARTESIAN_POINT('Ctrl Pts',(-2.35453559889474,1.,-3.05497218368146));
#51399=CARTESIAN_POINT('Ctrl Pts',(-2.36039011602072,1.,-3.0597826624004));
#51400=CARTESIAN_POINT('Ctrl Pts',(-2.36628220107009,1.,-3.06453964643162));
#51401=CARTESIAN_POINT('Ctrl Pts',(-2.37218678163178,1.,-3.069212754975));
#51402=CARTESIAN_POINT('Ctrl Pts',(-2.37809856205548,1.,-3.07379777492165));
#51403=CARTESIAN_POINT('Ctrl Pts',(-2.38402401216126,1.,-3.07830597244326));
#51404=CARTESIAN_POINT('Ctrl Pts',(-2.38997659219199,1.,-3.08275773747093));
#51405=CARTESIAN_POINT('Ctrl Pts',(-2.39597098250631,1.,-3.08717489512914));
#51406=CARTESIAN_POINT('Ctrl Pts',(-2.40201704423341,1.,-3.091572660511));
#51407=CARTESIAN_POINT('Ctrl Pts',(-2.40811612696369,1.,-3.09595472616076));
#51408=CARTESIAN_POINT('Ctrl Pts',(-2.41426441798057,1.,-3.1003177502767));
#51409=CARTESIAN_POINT('Ctrl Pts',(-2.42045498612489,1.,-3.10465410280896));
#51410=CARTESIAN_POINT('Ctrl Pts',(-2.42668025870015,1.,-3.10895518969595));
#51411=CARTESIAN_POINT('Ctrl Pts',(-2.43293449685144,1.,-3.11321477659018));
#51412=CARTESIAN_POINT('Ctrl Pts',(-2.43921571477977,1.,-3.11743156744186));
#51413=CARTESIAN_POINT('Ctrl Pts',(-2.44552433364715,1.,-3.12160740887768));
#51414=CARTESIAN_POINT('Ctrl Pts',(-2.45186227369846,1.,-3.12574608210847));
#51415=CARTESIAN_POINT('Ctrl Pts',(-2.45823188859366,1.,-3.12985188384371));
#51416=CARTESIAN_POINT('Ctrl Pts',(-2.46463494332374,1.,-3.13392826623906));
#51417=CARTESIAN_POINT('Ctrl Pts',(-2.47107164236838,1.,-3.13797654408943));
#51418=CARTESIAN_POINT('Ctrl Pts',(-2.47754112428043,1.,-3.14199655778863));
#51419=CARTESIAN_POINT('Ctrl Pts',(-2.4840418741839,1.,-3.14598722723896));
#51420=CARTESIAN_POINT('Ctrl Pts',(-2.49057217131988,1.,-3.14994715298907));
#51421=CARTESIAN_POINT('Ctrl Pts',(-2.49713050858896,1.,-3.15387518039046));
#51422=CARTESIAN_POINT('Ctrl Pts',(-2.50371605688252,1.,-3.15777102413957));
#51423=CARTESIAN_POINT('Ctrl Pts',(-2.51032851007894,1.,-3.16163506380157));
#51424=CARTESIAN_POINT('Ctrl Pts',(-2.51696788755577,1.,-3.16546808277023));
#51425=CARTESIAN_POINT('Ctrl Pts',(-2.52363434671788,1.,-3.16927102130736));
#51426=CARTESIAN_POINT('Ctrl Pts',(-2.53032800406941,1.,-3.17304474093612));
#51427=CARTESIAN_POINT('Ctrl Pts',(-2.53704871950948,1.,-3.17678974135318));
#51428=CARTESIAN_POINT('Ctrl Pts',(-2.54379612553051,1.,-3.1805061975064));
#51429=CARTESIAN_POINT('Ctrl Pts',(-2.55056972387731,1.,-3.18419408529594));
#51430=CARTESIAN_POINT('Ctrl Pts',(-2.55736896206056,1.,-3.18785328116218));
#51431=CARTESIAN_POINT('Ctrl Pts',(-2.56419331092858,1.,-3.19148366395139));
#51432=CARTESIAN_POINT('Ctrl Pts',(-2.57104235897899,1.,-3.19508523784363));
#51433=CARTESIAN_POINT('Ctrl Pts',(-2.57791581908875,1.,-3.19865814628682));
#51434=CARTESIAN_POINT('Ctrl Pts',(-2.58481347777729,1.,-3.20220261408414));
#51435=CARTESIAN_POINT('Ctrl Pts',(-2.59173516023481,1.,-3.2057189102873));
#51436=CARTESIAN_POINT('Ctrl Pts',(-2.59868069194342,1.,-3.20920730569681));
#51437=CARTESIAN_POINT('Ctrl Pts',(-2.60564985360017,1.,-3.21266802609682));
#51438=CARTESIAN_POINT('Ctrl Pts',(-2.61264236719171,1.,-3.21610123233082));
#51439=CARTESIAN_POINT('Ctrl Pts',(-2.61965792832947,1.,-3.21950704109321));
#51440=CARTESIAN_POINT('Ctrl Pts',(-2.62669622735912,1.,-3.2228855361324));
#51441=CARTESIAN_POINT('Ctrl Pts',(-2.63375697391372,1.,-3.2262367829246));
#51442=CARTESIAN_POINT('Ctrl Pts',(-2.64083992181823,1.,-3.22956084358547));
#51443=CARTESIAN_POINT('Ctrl Pts',(-2.64794488743038,1.,-3.23285778737096));
#51444=CARTESIAN_POINT('Ctrl Pts',(-2.65507173961555,1.,-3.236127680639));
#51445=CARTESIAN_POINT('Ctrl Pts',(-2.6607906631847,1.,-3.23872200034785));
#51446=CARTESIAN_POINT('Ctrl Pts',(-2.66508964663997,1.,-3.24065561086749));
#51447=CARTESIAN_POINT('Ctrl Pts',(-2.66795998539579,1.,-3.24193929584471));
#51448=CARTESIAN_POINT('Ctrl Pts',(-2.66939624221984,1.,-3.24257979115744));
#51449=CARTESIAN_POINT('Origin',(-2.66939624221984,0.,-3.24257979115744));
#51450=CARTESIAN_POINT('',(-2.78507268004356,1.,-3.14378277984898));
#51451=CARTESIAN_POINT('Origin',(0.,0.,0.));
#51452=CARTESIAN_POINT('',(-2.12971124846838,1.,-3.08655633322109));
#51453=CARTESIAN_POINT('Origin',(0.,1.,0.));
#51454=CARTESIAN_POINT('Ctrl Pts',(-2.12971124846838,1.,-3.08655633322109));
#51455=CARTESIAN_POINT('Ctrl Pts',(-2.12971124846838,0.666666666666667,
-3.08655633322109));
#51456=CARTESIAN_POINT('Ctrl Pts',(-2.12971124846838,0.333333333333333,
-3.08655633322109));
#51457=CARTESIAN_POINT('Ctrl Pts',(-2.12971124846838,-0.333333333333333,
-3.08655633322109));
#51458=CARTESIAN_POINT('Ctrl Pts',(-2.12971124846838,-0.666666666666667,
-3.08655633322109));
#51459=CARTESIAN_POINT('Ctrl Pts',(-2.12971124846838,-1.,-3.08655633322109));
#51460=CARTESIAN_POINT('Ctrl Pts',(-2.25898783642071,-1.,-3.54075895182139));
#51461=CARTESIAN_POINT('Ctrl Pts',(-2.25898783642071,1.,-3.54075895182139));
#51462=CARTESIAN_POINT('Ctrl Pts',(-2.25882251694918,-1.,-3.5391950664771));
#51463=CARTESIAN_POINT('Ctrl Pts',(-2.25882251694918,1.,-3.5391950664771));
#51464=CARTESIAN_POINT('Ctrl Pts',(-2.25848864344599,-1.,-3.53606853163247));
#51465=CARTESIAN_POINT('Ctrl Pts',(-2.25848864344599,1.,-3.53606853163247));
#51466=CARTESIAN_POINT('Ctrl Pts',(-2.25797812951166,-1.,-3.53138243689932));
#51467=CARTESIAN_POINT('Ctrl Pts',(-2.25797812951166,1.,-3.53138243689932));
#51468=CARTESIAN_POINT('Ctrl Pts',(-2.25727802942141,-1.,-3.52514172849666));
#51469=CARTESIAN_POINT('Ctrl Pts',(-2.25727802942141,1.,-3.52514172849666));
#51470=CARTESIAN_POINT('Ctrl Pts',(-2.25637049456061,-1.,-3.51735323669213));
#51471=CARTESIAN_POINT('Ctrl Pts',(-2.25637049456061,1.,-3.51735323669213));
#51472=CARTESIAN_POINT('Ctrl Pts',(-2.25543046980351,-1.,-3.50957720118209));
#51473=CARTESIAN_POINT('Ctrl Pts',(-2.25543046980351,1.,-3.50957720118209));
#51474=CARTESIAN_POINT('Ctrl Pts',(-2.25445785151923,-1.,-3.50181372618058));
#51475=CARTESIAN_POINT('Ctrl Pts',(-2.25445785151923,1.,-3.50181372618058));
#51476=CARTESIAN_POINT('Ctrl Pts',(-2.25345251709453,-1.,-3.49406296494309));
#51477=CARTESIAN_POINT('Ctrl Pts',(-2.25345251709453,1.,-3.49406296494309));
#51478=CARTESIAN_POINT('Ctrl Pts',(-2.25241433138231,-1.,-3.48632513240231));
#51479=CARTESIAN_POINT('Ctrl Pts',(-2.25241433138231,1.,-3.48632513240231));
#51480=CARTESIAN_POINT('Ctrl Pts',(-2.25134314238258,-1.,-3.47860048448015));
#51481=CARTESIAN_POINT('Ctrl Pts',(-2.25134314238258,1.,-3.47860048448015));
#51482=CARTESIAN_POINT('Ctrl Pts',(-2.25023877475674,-1.,-3.47088928979467));
#51483=CARTESIAN_POINT('Ctrl Pts',(-2.25023877475674,1.,-3.47088928979467));
#51484=CARTESIAN_POINT('Ctrl Pts',(-2.24910102345977,-1.,-3.46319180177474));
#51485=CARTESIAN_POINT('Ctrl Pts',(-2.24910102345977,1.,-3.46319180177474));
#51486=CARTESIAN_POINT('Ctrl Pts',(-2.24792964960874,-1.,-3.45550823512213));
#51487=CARTESIAN_POINT('Ctrl Pts',(-2.24792964960874,1.,-3.45550823512213));
#51488=CARTESIAN_POINT('Ctrl Pts',(-2.24672437070139,-1.,-3.44783872863448));
#51489=CARTESIAN_POINT('Ctrl Pts',(-2.24672437070139,1.,-3.44783872863448));
#51490=CARTESIAN_POINT('Ctrl Pts',(-2.24548487526212,-1.,-3.44018336460619));
#51491=CARTESIAN_POINT('Ctrl Pts',(-2.24548487526212,1.,-3.44018336460619));
#51492=CARTESIAN_POINT('Ctrl Pts',(-2.24421085338856,-1.,-3.43254222615007));
#51493=CARTESIAN_POINT('Ctrl Pts',(-2.24421085338856,1.,-3.43254222615007));
#51494=CARTESIAN_POINT('Ctrl Pts',(-2.24290202531144,-1.,-3.42491544683075));
#51495=CARTESIAN_POINT('Ctrl Pts',(-2.24290202531144,1.,-3.42491544683075));
#51496=CARTESIAN_POINT('Ctrl Pts',(-2.24155816587811,-1.,-3.41730325539119));
#51497=CARTESIAN_POINT('Ctrl Pts',(-2.24155816587811,1.,-3.41730325539119));
#51498=CARTESIAN_POINT('Ctrl Pts',(-2.24017914395211,-1.,-3.40970604190205));
#51499=CARTESIAN_POINT('Ctrl Pts',(-2.24017914395211,1.,-3.40970604190205));
#51500=CARTESIAN_POINT('Ctrl Pts',(-2.23876491124064,-1.,-3.40212434705511));
#51501=CARTESIAN_POINT('Ctrl Pts',(-2.23876491124064,1.,-3.40212434705511));
#51502=CARTESIAN_POINT('Ctrl Pts',(-2.23731541452727,-1.,-3.39455873448088));
#51503=CARTESIAN_POINT('Ctrl Pts',(-2.23731541452727,1.,-3.39455873448088));
#51504=CARTESIAN_POINT('Ctrl Pts',(-2.23583052276281,-1.,-3.38700968549522));
#51505=CARTESIAN_POINT('Ctrl Pts',(-2.23583052276281,1.,-3.38700968549522));
#51506=CARTESIAN_POINT('Ctrl Pts',(-2.23430995599572,-1.,-3.37947749555649));
#51507=CARTESIAN_POINT('Ctrl Pts',(-2.23430995599572,1.,-3.37947749555649));
#51508=CARTESIAN_POINT('Ctrl Pts',(-2.23275319569253,-1.,-3.37196214349356));
#51509=CARTESIAN_POINT('Ctrl Pts',(-2.23275319569253,1.,-3.37196214349356));
#51510=CARTESIAN_POINT('Ctrl Pts',(-2.23115945849777,-1.,-3.36446325227908));
#51511=CARTESIAN_POINT('Ctrl Pts',(-2.23115945849777,1.,-3.36446325227908));
#51512=CARTESIAN_POINT('Ctrl Pts',(-2.22952789881011,-1.,-3.35698038165529));
#51513=CARTESIAN_POINT('Ctrl Pts',(-2.22952789881011,1.,-3.35698038165529));
#51514=CARTESIAN_POINT('Ctrl Pts',(-2.22785777756588,-1.,-3.34951327111117));
#51515=CARTESIAN_POINT('Ctrl Pts',(-2.22785777756588,1.,-3.34951327111117));
#51516=CARTESIAN_POINT('Ctrl Pts',(-2.22614863918044,-1.,-3.34206209449371));
#51517=CARTESIAN_POINT('Ctrl Pts',(-2.22614863918044,1.,-3.34206209449371));
#51518=CARTESIAN_POINT('Ctrl Pts',(-2.224400498785,-1.,-3.3346277284958));
#51519=CARTESIAN_POINT('Ctrl Pts',(-2.224400498785,1.,-3.3346277284958));
#51520=CARTESIAN_POINT('Ctrl Pts',(-2.22261398879623,-1.,-3.32721196326019));
#51521=CARTESIAN_POINT('Ctrl Pts',(-2.22261398879623,1.,-3.32721196326019));
#51522=CARTESIAN_POINT('Ctrl Pts',(-2.22078990842768,-1.,-3.31981686778008));
#51523=CARTESIAN_POINT('Ctrl Pts',(-2.22078990842768,1.,-3.31981686778008));
#51524=CARTESIAN_POINT('Ctrl Pts',(-2.21892881679083,-1.,-3.31244421655662));
#51525=CARTESIAN_POINT('Ctrl Pts',(-2.21892881679083,1.,-3.31244421655662));
#51526=CARTESIAN_POINT('Ctrl Pts',(-2.21703059947837,-1.,-3.3050948781957));
#51527=CARTESIAN_POINT('Ctrl Pts',(-2.21703059947837,1.,-3.3050948781957));
#51528=CARTESIAN_POINT('Ctrl Pts',(-2.2150940692337,-1.,-3.29776825193162));
#51529=CARTESIAN_POINT('Ctrl Pts',(-2.2150940692337,1.,-3.29776825193162));
#51530=CARTESIAN_POINT('Ctrl Pts',(-2.21311648827391,-1.,-3.29046159238344));
#51531=CARTESIAN_POINT('Ctrl Pts',(-2.21311648827391,1.,-3.29046159238344));
#51532=CARTESIAN_POINT('Ctrl Pts',(-2.21109449750638,-1.,-3.28317133333127));
#51533=CARTESIAN_POINT('Ctrl Pts',(-2.21109449750638,1.,-3.28317133333127));
#51534=CARTESIAN_POINT('Ctrl Pts',(-2.20902509417425,-1.,-3.27589448005534));
#51535=CARTESIAN_POINT('Ctrl Pts',(-2.20902509417425,1.,-3.27589448005534));
#51536=CARTESIAN_POINT('Ctrl Pts',(-2.20690665217741,-1.,-3.2686300613678));
#51537=CARTESIAN_POINT('Ctrl Pts',(-2.20690665217741,1.,-3.2686300613678));
#51538=CARTESIAN_POINT('Ctrl Pts',(-2.20473979048682,-1.,-3.26138036637711));
#51539=CARTESIAN_POINT('Ctrl Pts',(-2.20473979048682,1.,-3.26138036637711));
#51540=CARTESIAN_POINT('Ctrl Pts',(-2.20252866491554,-1.,-3.25415277957789));
#51541=CARTESIAN_POINT('Ctrl Pts',(-2.20252866491554,1.,-3.25415277957789));
#51542=CARTESIAN_POINT('Ctrl Pts',(-2.20027910880993,-1.,-3.24695715874356));
#51543=CARTESIAN_POINT('Ctrl Pts',(-2.20027910880993,1.,-3.24695715874356));
#51544=CARTESIAN_POINT('Ctrl Pts',(-2.19799623693263,-1.,-3.23980245361323));
#51545=CARTESIAN_POINT('Ctrl Pts',(-2.19799623693263,1.,-3.23980245361323));
#51546=CARTESIAN_POINT('Ctrl Pts',(-2.19568204933172,-1.,-3.23269332296938));
#51547=CARTESIAN_POINT('Ctrl Pts',(-2.19568204933172,1.,-3.23269332296938));
#51548=CARTESIAN_POINT('Ctrl Pts',(-2.19333345123531,-1.,-3.22562734221636));
#51549=CARTESIAN_POINT('Ctrl Pts',(-2.19333345123531,1.,-3.22562734221636));
#51550=CARTESIAN_POINT('Ctrl Pts',(-2.1909390194865,-1.,-3.21859043114069));
#51551=CARTESIAN_POINT('Ctrl Pts',(-2.1909390194865,1.,-3.21859043114069));
#51552=CARTESIAN_POINT('Ctrl Pts',(-2.18848253363878,-1.,-3.21156188355736));
#51553=CARTESIAN_POINT('Ctrl Pts',(-2.18848253363878,1.,-3.21156188355736));
#51554=CARTESIAN_POINT('Ctrl Pts',(-2.18594876115914,-1.,-3.20452259717947));
#51555=CARTESIAN_POINT('Ctrl Pts',(-2.18594876115914,1.,-3.20452259717947));
#51556=CARTESIAN_POINT('Ctrl Pts',(-2.18332898656595,-1.,-3.197462937404));
#51557=CARTESIAN_POINT('Ctrl Pts',(-2.18332898656595,1.,-3.197462937404));
#51558=CARTESIAN_POINT('Ctrl Pts',(-2.18062558031789,-1.,-3.19038924261589));
#51559=CARTESIAN_POINT('Ctrl Pts',(-2.18062558031789,1.,-3.19038924261589));
#51560=CARTESIAN_POINT('Ctrl Pts',(-2.17785968847172,-1.,-3.18333474627851));
#51561=CARTESIAN_POINT('Ctrl Pts',(-2.17785968847172,1.,-3.18333474627851));
#51562=CARTESIAN_POINT('Ctrl Pts',(-2.17506466903736,-1.,-3.17635032802584));
#51563=CARTESIAN_POINT('Ctrl Pts',(-2.17506466903736,1.,-3.17635032802584));
#51564=CARTESIAN_POINT('Ctrl Pts',(-2.17227212063857,-1.,-3.16948480019555));
#51565=CARTESIAN_POINT('Ctrl Pts',(-2.17227212063857,1.,-3.16948480019555));
#51566=CARTESIAN_POINT('Ctrl Pts',(-2.16949910801237,-1.,-3.16276685102999));
#51567=CARTESIAN_POINT('Ctrl Pts',(-2.16949910801237,1.,-3.16276685102999));
#51568=CARTESIAN_POINT('Ctrl Pts',(-2.1667372844767,-1.,-3.15618975593627));
#51569=CARTESIAN_POINT('Ctrl Pts',(-2.1667372844767,1.,-3.15618975593627));
#51570=CARTESIAN_POINT('Ctrl Pts',(-2.16393520288009,-1.,-3.14968624388961));
#51571=CARTESIAN_POINT('Ctrl Pts',(-2.16393520288009,1.,-3.14968624388961));
#51572=CARTESIAN_POINT('Ctrl Pts',(-2.16100905914341,-1.,-3.14314440426882));
#51573=CARTESIAN_POINT('Ctrl Pts',(-2.16100905914341,1.,-3.14314440426882));
#51574=CARTESIAN_POINT('Ctrl Pts',(-2.15787423530583,-1.,-3.136453565629));
#51575=CARTESIAN_POINT('Ctrl Pts',(-2.15787423530583,1.,-3.136453565629));
#51576=CARTESIAN_POINT('Ctrl Pts',(-2.15447241382872,-1.,-3.12954386795575));
#51577=CARTESIAN_POINT('Ctrl Pts',(-2.15447241382872,1.,-3.12954386795575));
#51578=CARTESIAN_POINT('Ctrl Pts',(-2.15079698090627,-1.,-3.12242318152001));
#51579=CARTESIAN_POINT('Ctrl Pts',(-2.15079698090627,1.,-3.12242318152001));
#51580=CARTESIAN_POINT('Ctrl Pts',(-2.1469279845768,-1.,-3.11522827017075));
#51581=CARTESIAN_POINT('Ctrl Pts',(-2.1469279845768,1.,-3.11522827017075));
#51582=CARTESIAN_POINT('Ctrl Pts',(-2.14302815602195,-1.,-3.10821808669189));
#51583=CARTESIAN_POINT('Ctrl Pts',(-2.14302815602195,1.,-3.10821808669189));
#51584=CARTESIAN_POINT('Ctrl Pts',(-2.13930228863968,-1.,-3.1017126739137));
#51585=CARTESIAN_POINT('Ctrl Pts',(-2.13930228863968,1.,-3.1017126739137));
#51586=CARTESIAN_POINT('Ctrl Pts',(-2.13596538661154,-1.,-3.09604502421197));
#51587=CARTESIAN_POINT('Ctrl Pts',(-2.13596538661154,1.,-3.09604502421197));
#51588=CARTESIAN_POINT('Ctrl Pts',(-2.13321032560805,-1.,-3.09151235281832));
#51589=CARTESIAN_POINT('Ctrl Pts',(-2.13321032560805,1.,-3.09151235281832));
#51590=CARTESIAN_POINT('Ctrl Pts',(-2.13116819908264,-1.,-3.08831615619661));
#51591=CARTESIAN_POINT('Ctrl Pts',(-2.13116819908264,1.,-3.08831615619661));
#51592=CARTESIAN_POINT('Ctrl Pts',(-2.1301541297915,-1.,-3.08690399991003));
#51593=CARTESIAN_POINT('Ctrl Pts',(-2.1301541297915,1.,-3.08690399991003));
#51594=CARTESIAN_POINT('Ctrl Pts',(-2.12975158752197,-1.,-3.08650326866821));
#51595=CARTESIAN_POINT('Ctrl Pts',(-2.12975158752197,1.,-3.08650326866821));
#51596=CARTESIAN_POINT('Ctrl Pts',(-2.12964222015945,-1.,-3.08652852644876));
#51597=CARTESIAN_POINT('Ctrl Pts',(-2.12964222015945,1.,-3.08652852644876));
#51598=CARTESIAN_POINT('Ctrl Pts',(-2.12962728847314,-1.,-3.08661426358891));
#51599=CARTESIAN_POINT('Ctrl Pts',(-2.12962728847314,1.,-3.08661426358891));
#51600=CARTESIAN_POINT('',(-2.25898783642071,1.,-3.54075895182139));
#51601=CARTESIAN_POINT('Ctrl Pts',(-2.25898783642071,1.,-3.54075895182139));
#51602=CARTESIAN_POINT('Ctrl Pts',(-2.25882251694918,1.,-3.5391950664771));
#51603=CARTESIAN_POINT('Ctrl Pts',(-2.25848864344599,1.,-3.53606853163247));
#51604=CARTESIAN_POINT('Ctrl Pts',(-2.25797812951166,1.,-3.53138243689932));
#51605=CARTESIAN_POINT('Ctrl Pts',(-2.25727802942141,1.,-3.52514172849666));
#51606=CARTESIAN_POINT('Ctrl Pts',(-2.25637049456061,1.,-3.51735323669213));
#51607=CARTESIAN_POINT('Ctrl Pts',(-2.25543046980351,1.,-3.50957720118209));
#51608=CARTESIAN_POINT('Ctrl Pts',(-2.25445785151923,1.,-3.50181372618058));
#51609=CARTESIAN_POINT('Ctrl Pts',(-2.25345251709453,1.,-3.49406296494309));
#51610=CARTESIAN_POINT('Ctrl Pts',(-2.25241433138231,1.,-3.48632513240231));
#51611=CARTESIAN_POINT('Ctrl Pts',(-2.25134314238258,1.,-3.47860048448015));
#51612=CARTESIAN_POINT('Ctrl Pts',(-2.25023877475674,1.,-3.47088928979467));
#51613=CARTESIAN_POINT('Ctrl Pts',(-2.24910102345977,1.,-3.46319180177474));
#51614=CARTESIAN_POINT('Ctrl Pts',(-2.24792964960874,1.,-3.45550823512213));
#51615=CARTESIAN_POINT('Ctrl Pts',(-2.24672437070139,1.,-3.44783872863448));
#51616=CARTESIAN_POINT('Ctrl Pts',(-2.24548487526212,1.,-3.44018336460619));
#51617=CARTESIAN_POINT('Ctrl Pts',(-2.24421085338856,1.,-3.43254222615007));
#51618=CARTESIAN_POINT('Ctrl Pts',(-2.24290202531144,1.,-3.42491544683075));
#51619=CARTESIAN_POINT('Ctrl Pts',(-2.24155816587811,1.,-3.41730325539119));
#51620=CARTESIAN_POINT('Ctrl Pts',(-2.24017914395211,1.,-3.40970604190205));
#51621=CARTESIAN_POINT('Ctrl Pts',(-2.23876491124064,1.,-3.40212434705511));
#51622=CARTESIAN_POINT('Ctrl Pts',(-2.23731541452727,1.,-3.39455873448088));
#51623=CARTESIAN_POINT('Ctrl Pts',(-2.23583052276281,1.,-3.38700968549522));
#51624=CARTESIAN_POINT('Ctrl Pts',(-2.23430995599572,1.,-3.37947749555649));
#51625=CARTESIAN_POINT('Ctrl Pts',(-2.23275319569253,1.,-3.37196214349356));
#51626=CARTESIAN_POINT('Ctrl Pts',(-2.23115945849777,1.,-3.36446325227908));
#51627=CARTESIAN_POINT('Ctrl Pts',(-2.22952789881011,1.,-3.35698038165529));
#51628=CARTESIAN_POINT('Ctrl Pts',(-2.22785777756588,1.,-3.34951327111117));
#51629=CARTESIAN_POINT('Ctrl Pts',(-2.22614863918044,1.,-3.34206209449371));
#51630=CARTESIAN_POINT('Ctrl Pts',(-2.224400498785,1.,-3.3346277284958));
#51631=CARTESIAN_POINT('Ctrl Pts',(-2.22261398879623,1.,-3.32721196326019));
#51632=CARTESIAN_POINT('Ctrl Pts',(-2.22078990842768,1.,-3.31981686778008));
#51633=CARTESIAN_POINT('Ctrl Pts',(-2.21892881679083,1.,-3.31244421655662));
#51634=CARTESIAN_POINT('Ctrl Pts',(-2.21703059947837,1.,-3.3050948781957));
#51635=CARTESIAN_POINT('Ctrl Pts',(-2.2150940692337,1.,-3.29776825193162));
#51636=CARTESIAN_POINT('Ctrl Pts',(-2.21311648827391,1.,-3.29046159238344));
#51637=CARTESIAN_POINT('Ctrl Pts',(-2.21109449750638,1.,-3.28317133333127));
#51638=CARTESIAN_POINT('Ctrl Pts',(-2.20902509417425,1.,-3.27589448005534));
#51639=CARTESIAN_POINT('Ctrl Pts',(-2.20690665217741,1.,-3.2686300613678));
#51640=CARTESIAN_POINT('Ctrl Pts',(-2.20473979048682,1.,-3.26138036637711));
#51641=CARTESIAN_POINT('Ctrl Pts',(-2.20252866491554,1.,-3.25415277957789));
#51642=CARTESIAN_POINT('Ctrl Pts',(-2.20027910880993,1.,-3.24695715874356));
#51643=CARTESIAN_POINT('Ctrl Pts',(-2.19799623693263,1.,-3.23980245361323));
#51644=CARTESIAN_POINT('Ctrl Pts',(-2.19568204933172,1.,-3.23269332296938));
#51645=CARTESIAN_POINT('Ctrl Pts',(-2.19333345123531,1.,-3.22562734221636));
#51646=CARTESIAN_POINT('Ctrl Pts',(-2.1909390194865,1.,-3.21859043114069));
#51647=CARTESIAN_POINT('Ctrl Pts',(-2.18848253363878,1.,-3.21156188355736));
#51648=CARTESIAN_POINT('Ctrl Pts',(-2.18594876115914,1.,-3.20452259717947));
#51649=CARTESIAN_POINT('Ctrl Pts',(-2.18332898656595,1.,-3.197462937404));
#51650=CARTESIAN_POINT('Ctrl Pts',(-2.18062558031789,1.,-3.19038924261589));
#51651=CARTESIAN_POINT('Ctrl Pts',(-2.17785968847172,1.,-3.18333474627851));
#51652=CARTESIAN_POINT('Ctrl Pts',(-2.17506466903736,1.,-3.17635032802584));
#51653=CARTESIAN_POINT('Ctrl Pts',(-2.17227212063857,1.,-3.16948480019555));
#51654=CARTESIAN_POINT('Ctrl Pts',(-2.16949910801237,1.,-3.16276685102999));
#51655=CARTESIAN_POINT('Ctrl Pts',(-2.1667372844767,1.,-3.15618975593627));
#51656=CARTESIAN_POINT('Ctrl Pts',(-2.16393520288009,1.,-3.14968624388961));
#51657=CARTESIAN_POINT('Ctrl Pts',(-2.16100905914341,1.,-3.14314440426882));
#51658=CARTESIAN_POINT('Ctrl Pts',(-2.15787423530583,1.,-3.136453565629));
#51659=CARTESIAN_POINT('Ctrl Pts',(-2.15447241382872,1.,-3.12954386795575));
#51660=CARTESIAN_POINT('Ctrl Pts',(-2.15079698090627,1.,-3.12242318152001));
#51661=CARTESIAN_POINT('Ctrl Pts',(-2.1469279845768,1.,-3.11522827017075));
#51662=CARTESIAN_POINT('Ctrl Pts',(-2.14302815602195,1.,-3.10821808669189));
#51663=CARTESIAN_POINT('Ctrl Pts',(-2.13930228863968,1.,-3.1017126739137));
#51664=CARTESIAN_POINT('Ctrl Pts',(-2.13596538661154,1.,-3.09604502421197));
#51665=CARTESIAN_POINT('Ctrl Pts',(-2.13321032560805,1.,-3.09151235281832));
#51666=CARTESIAN_POINT('Ctrl Pts',(-2.13132142793056,1.,-3.08855597949844));
#51667=CARTESIAN_POINT('Ctrl Pts',(-2.13034980480519,1.,-3.08717896996213));
#51668=CARTESIAN_POINT('Ctrl Pts',(-2.12991938762497,1.,-3.08668447250383));
#51669=CARTESIAN_POINT('Ctrl Pts',(-2.1297578506162,1.,-3.0865713108946));
#51670=CARTESIAN_POINT('Ctrl Pts',(-2.12971124846838,1.,-3.0865563332211));
#51671=CARTESIAN_POINT('',(-2.25898783642071,0.,-3.54075895182139));
#51672=CARTESIAN_POINT('Ctrl Pts',(-1.7833628895577,-1.,-3.2988053601491));
#51673=CARTESIAN_POINT('Ctrl Pts',(-1.7833628895577,1.,-3.2988053601491));
#51674=CARTESIAN_POINT('Ctrl Pts',(-1.78327971836342,-1.,-3.29877974053316));
#51675=CARTESIAN_POINT('Ctrl Pts',(-1.78327971836342,1.,-3.29877974053316));
#51676=CARTESIAN_POINT('Ctrl Pts',(-1.78320756177373,-1.,-3.29886572077632));
#51677=CARTESIAN_POINT('Ctrl Pts',(-1.78320756177373,1.,-3.29886572077632));
#51678=CARTESIAN_POINT('Ctrl Pts',(-1.7833818655594,-1.,-3.29940631674303));
#51679=CARTESIAN_POINT('Ctrl Pts',(-1.7833818655594,1.,-3.29940631674303));
#51680=CARTESIAN_POINT('Ctrl Pts',(-1.78417972819938,-1.,-3.30095096463517));
#51681=CARTESIAN_POINT('Ctrl Pts',(-1.78417972819938,1.,-3.30095096463517));
#51682=CARTESIAN_POINT('Ctrl Pts',(-1.78610045419846,-1.,-3.30422155559112));
#51683=CARTESIAN_POINT('Ctrl Pts',(-1.78610045419846,1.,-3.30422155559112));
#51684=CARTESIAN_POINT('Ctrl Pts',(-1.78888832245873,-1.,-3.30873412266788));
#51685=CARTESIAN_POINT('Ctrl Pts',(-1.78888832245873,1.,-3.30873412266788));
#51686=CARTESIAN_POINT('Ctrl Pts',(-1.79242331349949,-1.,-3.31428038326424));
#51687=CARTESIAN_POINT('Ctrl Pts',(-1.79242331349949,1.,-3.31428038326424));
#51688=CARTESIAN_POINT('Ctrl Pts',(-1.79652817033251,-1.,-3.3205535510082));
#51689=CARTESIAN_POINT('Ctrl Pts',(-1.79652817033251,1.,-3.3205535510082));
#51690=CARTESIAN_POINT('Ctrl Pts',(-1.80100380443406,-1.,-3.32721088039578));
#51691=CARTESIAN_POINT('Ctrl Pts',(-1.80100380443406,1.,-3.32721088039578));
#51692=CARTESIAN_POINT('Ctrl Pts',(-1.80565802981102,-1.,-3.33392460276808));
#51693=CARTESIAN_POINT('Ctrl Pts',(-1.80565802981102,1.,-3.33392460276808));
#51694=CARTESIAN_POINT('Ctrl Pts',(-1.81033399625352,-1.,-3.34043216147606));
#51695=CARTESIAN_POINT('Ctrl Pts',(-1.81033399625352,1.,-3.34043216147606));
#51696=CARTESIAN_POINT('Ctrl Pts',(-1.81494618732853,-1.,-3.34660014370673));
#51697=CARTESIAN_POINT('Ctrl Pts',(-1.81494618732853,1.,-3.34660014370673));
#51698=CARTESIAN_POINT('Ctrl Pts',(-1.81948458796829,-1.,-3.35243086937598));
#51699=CARTESIAN_POINT('Ctrl Pts',(-1.81948458796829,1.,-3.35243086937598));
#51700=CARTESIAN_POINT('Ctrl Pts',(-1.82398496829301,-1.,-3.35800801557424));
#51701=CARTESIAN_POINT('Ctrl Pts',(-1.82398496829301,1.,-3.35800801557424));
#51702=CARTESIAN_POINT('Ctrl Pts',(-1.82850752153199,-1.,-3.36345722124158));
#51703=CARTESIAN_POINT('Ctrl Pts',(-1.82850752153199,1.,-3.36345722124158));
#51704=CARTESIAN_POINT('Ctrl Pts',(-1.83311391452322,-1.,-3.36890396271836));
#51705=CARTESIAN_POINT('Ctrl Pts',(-1.83311391452322,1.,-3.36890396271836));
#51706=CARTESIAN_POINT('Ctrl Pts',(-1.83784072967077,-1.,-3.37442462015853));
#51707=CARTESIAN_POINT('Ctrl Pts',(-1.83784072967077,1.,-3.37442462015853));
#51708=CARTESIAN_POINT('Ctrl Pts',(-1.84269016931643,-1.,-3.38002968341157));
#51709=CARTESIAN_POINT('Ctrl Pts',(-1.84269016931643,1.,-3.38002968341157));
#51710=CARTESIAN_POINT('Ctrl Pts',(-1.84764441927753,-1.,-3.38569092349592));
#51711=CARTESIAN_POINT('Ctrl Pts',(-1.84764441927753,1.,-3.38569092349592));
#51712=CARTESIAN_POINT('Ctrl Pts',(-1.85267433291769,-1.,-3.39135802549398));
#51713=CARTESIAN_POINT('Ctrl Pts',(-1.85267433291769,1.,-3.39135802549398));
#51714=CARTESIAN_POINT('Ctrl Pts',(-1.85774972037062,-1.,-3.39697816833067));
#51715=CARTESIAN_POINT('Ctrl Pts',(-1.85774972037062,1.,-3.39697816833067));
#51716=CARTESIAN_POINT('Ctrl Pts',(-1.86285057051245,-1.,-3.40251742305476));
#51717=CARTESIAN_POINT('Ctrl Pts',(-1.86285057051245,1.,-3.40251742305476));
#51718=CARTESIAN_POINT('Ctrl Pts',(-1.86797231196654,-1.,-3.40797080000549));
#51719=CARTESIAN_POINT('Ctrl Pts',(-1.86797231196654,1.,-3.40797080000549));
#51720=CARTESIAN_POINT('Ctrl Pts',(-1.87311957248121,-1.,-3.41335043875209));
#51721=CARTESIAN_POINT('Ctrl Pts',(-1.87311957248121,1.,-3.41335043875209));
#51722=CARTESIAN_POINT('Ctrl Pts',(-1.87830245689344,-1.,-3.41867858383771));
#51723=CARTESIAN_POINT('Ctrl Pts',(-1.87830245689344,1.,-3.41867858383771));
#51724=CARTESIAN_POINT('Ctrl Pts',(-1.8835320506206,-1.,-3.42397908819736));
#51725=CARTESIAN_POINT('Ctrl Pts',(-1.8835320506206,1.,-3.42397908819736));
#51726=CARTESIAN_POINT('Ctrl Pts',(-1.88881571322009,-1.,-3.42926852222158));
#51727=CARTESIAN_POINT('Ctrl Pts',(-1.88881571322009,1.,-3.42926852222158));
#51728=CARTESIAN_POINT('Ctrl Pts',(-1.89415420002542,-1.,-3.43455074411571));
#51729=CARTESIAN_POINT('Ctrl Pts',(-1.89415420002542,1.,-3.43455074411571));
#51730=CARTESIAN_POINT('Ctrl Pts',(-1.89954426803384,-1.,-3.4398218567809));
#51731=CARTESIAN_POINT('Ctrl Pts',(-1.89954426803384,1.,-3.4398218567809));
#51732=CARTESIAN_POINT('Ctrl Pts',(-1.90498026502305,-1.,-3.44507323983367));
#51733=CARTESIAN_POINT('Ctrl Pts',(-1.90498026502305,1.,-3.44507323983367));
#51734=CARTESIAN_POINT('Ctrl Pts',(-1.91045605593639,-1.,-3.45029522038888));
#51735=CARTESIAN_POINT('Ctrl Pts',(-1.91045605593639,1.,-3.45029522038888));
#51736=CARTESIAN_POINT('Ctrl Pts',(-1.91596694784064,-1.,-3.4554807430995));
#51737=CARTESIAN_POINT('Ctrl Pts',(-1.91596694784064,1.,-3.4554807430995));
#51738=CARTESIAN_POINT('Ctrl Pts',(-1.92151118213212,-1.,-3.46062821722485));
#51739=CARTESIAN_POINT('Ctrl Pts',(-1.92151118213212,1.,-3.46062821722485));
#51740=CARTESIAN_POINT('Ctrl Pts',(-1.92708888591158,-1.,-3.46573953254084));
#51741=CARTESIAN_POINT('Ctrl Pts',(-1.92708888591158,1.,-3.46573953254084));
#51742=CARTESIAN_POINT('Ctrl Pts',(-1.93270136427081,-1.,-3.47081872409781));
#51743=CARTESIAN_POINT('Ctrl Pts',(-1.93270136427081,1.,-3.47081872409781));
#51744=CARTESIAN_POINT('Ctrl Pts',(-1.93835026973887,-1.,-3.47587040389915));
#51745=CARTESIAN_POINT('Ctrl Pts',(-1.93835026973887,1.,-3.47587040389915));
#51746=CARTESIAN_POINT('Ctrl Pts',(-1.94403680554065,-1.,-3.48089825770416));
#51747=CARTESIAN_POINT('Ctrl Pts',(-1.94403680554065,1.,-3.48089825770416));
#51748=CARTESIAN_POINT('Ctrl Pts',(-1.94976096795911,-1.,-3.48590361610814));
#51749=CARTESIAN_POINT('Ctrl Pts',(-1.94976096795911,1.,-3.48590361610814));
#51750=CARTESIAN_POINT('Ctrl Pts',(-1.95552193112084,-1.,-3.49088618670987));
#51751=CARTESIAN_POINT('Ctrl Pts',(-1.95552193112084,1.,-3.49088618670987));
#51752=CARTESIAN_POINT('Ctrl Pts',(-1.961318367765,-1.,-3.49584466573064));
#51753=CARTESIAN_POINT('Ctrl Pts',(-1.961318367765,1.,-3.49584466573064));
#51754=CARTESIAN_POINT('Ctrl Pts',(-1.96714879724052,-1.,-3.50077740176267));
#51755=CARTESIAN_POINT('Ctrl Pts',(-1.96714879724052,1.,-3.50077740176267));
#51756=CARTESIAN_POINT('Ctrl Pts',(-1.97301191162968,-1.,-3.5056830186108));
#51757=CARTESIAN_POINT('Ctrl Pts',(-1.97301191162968,1.,-3.5056830186108));
#51758=CARTESIAN_POINT('Ctrl Pts',(-1.97890693666288,-1.,-3.51056110478287));
#51759=CARTESIAN_POINT('Ctrl Pts',(-1.97890693666288,1.,-3.51056110478287));
#51760=CARTESIAN_POINT('Ctrl Pts',(-1.9848335106103,-1.,-3.51541198728301));
#51761=CARTESIAN_POINT('Ctrl Pts',(-1.9848335106103,1.,-3.51541198728301));
#51762=CARTESIAN_POINT('Ctrl Pts',(-1.99079153006112,-1.,-3.52023644289142));
#51763=CARTESIAN_POINT('Ctrl Pts',(-1.99079153006112,1.,-3.52023644289142));
#51764=CARTESIAN_POINT('Ctrl Pts',(-1.99678100339296,-1.,-3.52503542491728));
#51765=CARTESIAN_POINT('Ctrl Pts',(-1.99678100339296,1.,-3.52503542491728));
#51766=CARTESIAN_POINT('Ctrl Pts',(-2.00280191090366,-1.,-3.52980980250224));
#51767=CARTESIAN_POINT('Ctrl Pts',(-2.00280191090366,1.,-3.52980980250224));
#51768=CARTESIAN_POINT('Ctrl Pts',(-2.00885403604746,-1.,-3.53456004727424));
#51769=CARTESIAN_POINT('Ctrl Pts',(-2.00885403604746,1.,-3.53456004727424));
#51770=CARTESIAN_POINT('Ctrl Pts',(-2.01493698847351,-1.,-3.53928627453642));
#51771=CARTESIAN_POINT('Ctrl Pts',(-2.01493698847351,1.,-3.53928627453642));
#51772=CARTESIAN_POINT('Ctrl Pts',(-2.02105027983104,-1.,-3.54398838254136));
#51773=CARTESIAN_POINT('Ctrl Pts',(-2.02105027983104,1.,-3.54398838254136));
#51774=CARTESIAN_POINT('Ctrl Pts',(-2.02719338376175,-1.,-3.54866616282227));
#51775=CARTESIAN_POINT('Ctrl Pts',(-2.02719338376175,1.,-3.54866616282227));
#51776=CARTESIAN_POINT('Ctrl Pts',(-2.03336579658133,-1.,-3.55331941293949));
#51777=CARTESIAN_POINT('Ctrl Pts',(-2.03336579658133,1.,-3.55331941293949));
#51778=CARTESIAN_POINT('Ctrl Pts',(-2.03956711119976,-1.,-3.55794807264844));
#51779=CARTESIAN_POINT('Ctrl Pts',(-2.03956711119976,1.,-3.55794807264844));
#51780=CARTESIAN_POINT('Ctrl Pts',(-2.04579702158876,-1.,-3.56255223871505));
#51781=CARTESIAN_POINT('Ctrl Pts',(-2.04579702158876,1.,-3.56255223871505));
#51782=CARTESIAN_POINT('Ctrl Pts',(-2.05205528172911,-1.,-3.56713209977904));
#51783=CARTESIAN_POINT('Ctrl Pts',(-2.05205528172911,1.,-3.56713209977904));
#51784=CARTESIAN_POINT('Ctrl Pts',(-2.05834167687425,-1.,-3.5716878942334));
#51785=CARTESIAN_POINT('Ctrl Pts',(-2.05834167687425,1.,-3.5716878942334));
#51786=CARTESIAN_POINT('Ctrl Pts',(-2.06465599229234,-1.,-3.57621986224402));
#51787=CARTESIAN_POINT('Ctrl Pts',(-2.06465599229234,1.,-3.57621986224402));
#51788=CARTESIAN_POINT('Ctrl Pts',(-2.07099797606,-1.,-3.58072819250872));
#51789=CARTESIAN_POINT('Ctrl Pts',(-2.07099797606,1.,-3.58072819250872));
#51790=CARTESIAN_POINT('Ctrl Pts',(-2.07736732842524,-1.,-3.58521300039988));
#51791=CARTESIAN_POINT('Ctrl Pts',(-2.07736732842524,1.,-3.58521300039988));
#51792=CARTESIAN_POINT('Ctrl Pts',(-2.08376373049196,-1.,-3.58967435355834));
#51793=CARTESIAN_POINT('Ctrl Pts',(-2.08376373049196,1.,-3.58967435355834));
#51794=CARTESIAN_POINT('Ctrl Pts',(-2.09018686331706,-1.,-3.5941122862608));
#51795=CARTESIAN_POINT('Ctrl Pts',(-2.09018686331706,1.,-3.5941122862608));
#51796=CARTESIAN_POINT('Ctrl Pts',(-2.09663642986579,-1.,-3.59852681775396));
#51797=CARTESIAN_POINT('Ctrl Pts',(-2.09663642986579,1.,-3.59852681775396));
#51798=CARTESIAN_POINT('Ctrl Pts',(-2.10311217727687,-1.,-3.60291797087849));
#51799=CARTESIAN_POINT('Ctrl Pts',(-2.10311217727687,1.,-3.60291797087849));
#51800=CARTESIAN_POINT('Ctrl Pts',(-2.10961391333497,-1.,-3.60728578530968));
#51801=CARTESIAN_POINT('Ctrl Pts',(-2.10961391333497,1.,-3.60728578530968));
#51802=CARTESIAN_POINT('Ctrl Pts',(-2.11614149813928,-1.,-3.61163030607452));
#51803=CARTESIAN_POINT('Ctrl Pts',(-2.11614149813928,1.,-3.61163030607452));
#51804=CARTESIAN_POINT('Ctrl Pts',(-2.12138417125349,-1.,-3.61508732215187));
#51805=CARTESIAN_POINT('Ctrl Pts',(-2.12138417125349,1.,-3.61508732215187));
#51806=CARTESIAN_POINT('Ctrl Pts',(-2.12532774376144,-1.,-3.61766963589442));
#51807=CARTESIAN_POINT('Ctrl Pts',(-2.12532774376144,1.,-3.61766963589442));
#51808=CARTESIAN_POINT('Ctrl Pts',(-2.12796193131142,-1.,-3.61938653648716));
#51809=CARTESIAN_POINT('Ctrl Pts',(-2.12796193131142,1.,-3.61938653648716));
#51810=CARTESIAN_POINT('Ctrl Pts',(-2.12928030988903,-1.,-3.62024382630768));
#51811=CARTESIAN_POINT('Ctrl Pts',(-2.12928030988903,1.,-3.62024382630768));
#51812=CARTESIAN_POINT('',(-1.78327315618341,1.,-3.29885386921514));
#51813=CARTESIAN_POINT('Ctrl Pts',(-1.78327315618341,-1.,-3.29885386921513));
#51814=CARTESIAN_POINT('Ctrl Pts',(-1.78327315618341,-0.666666666666667,
-3.29885386921513));
#51815=CARTESIAN_POINT('Ctrl Pts',(-1.78327315618341,-0.333333333333333,
-3.29885386921513));
#51816=CARTESIAN_POINT('Ctrl Pts',(-1.78327315618341,0.333333333333333,
-3.29885386921513));
#51817=CARTESIAN_POINT('Ctrl Pts',(-1.78327315618341,0.666666666666667,
-3.29885386921513));
#51818=CARTESIAN_POINT('Ctrl Pts',(-1.78327315618341,1.,-3.29885386921513));
#51819=CARTESIAN_POINT('',(-2.12928030988903,1.,-3.62024382630768));
#51820=CARTESIAN_POINT('',(-2.12928030988903,0.,-3.62024382630768));
#51821=CARTESIAN_POINT('Ctrl Pts',(-1.78327315618341,1.,-3.29885386921514));
#51822=CARTESIAN_POINT('Ctrl Pts',(-1.78326534445518,1.,-3.29890219175423));
#51823=CARTESIAN_POINT('Ctrl Pts',(-1.78329283591905,1.,-3.29909749657808));
#51824=CARTESIAN_POINT('Ctrl Pts',(-1.78353803106924,1.,-3.299705498242));
#51825=CARTESIAN_POINT('Ctrl Pts',(-1.78432384788174,1.,-3.30119637003394));
#51826=CARTESIAN_POINT('Ctrl Pts',(-1.78610045419846,1.,-3.30422155559112));
#51827=CARTESIAN_POINT('Ctrl Pts',(-1.78888832245873,1.,-3.30873412266788));
#51828=CARTESIAN_POINT('Ctrl Pts',(-1.79242331349949,1.,-3.31428038326424));
#51829=CARTESIAN_POINT('Ctrl Pts',(-1.79652817033251,1.,-3.3205535510082));
#51830=CARTESIAN_POINT('Ctrl Pts',(-1.80100380443406,1.,-3.32721088039578));
#51831=CARTESIAN_POINT('Ctrl Pts',(-1.80565802981102,1.,-3.33392460276808));
#51832=CARTESIAN_POINT('Ctrl Pts',(-1.81033399625352,1.,-3.34043216147606));
#51833=CARTESIAN_POINT('Ctrl Pts',(-1.81494618732853,1.,-3.34660014370673));
#51834=CARTESIAN_POINT('Ctrl Pts',(-1.81948458796829,1.,-3.35243086937598));
#51835=CARTESIAN_POINT('Ctrl Pts',(-1.82398496829301,1.,-3.35800801557424));
#51836=CARTESIAN_POINT('Ctrl Pts',(-1.82850752153199,1.,-3.36345722124158));
#51837=CARTESIAN_POINT('Ctrl Pts',(-1.83311391452322,1.,-3.36890396271836));
#51838=CARTESIAN_POINT('Ctrl Pts',(-1.83784072967077,1.,-3.37442462015853));
#51839=CARTESIAN_POINT('Ctrl Pts',(-1.84269016931643,1.,-3.38002968341157));
#51840=CARTESIAN_POINT('Ctrl Pts',(-1.84764441927753,1.,-3.38569092349592));
#51841=CARTESIAN_POINT('Ctrl Pts',(-1.85267433291769,1.,-3.39135802549398));
#51842=CARTESIAN_POINT('Ctrl Pts',(-1.85774972037062,1.,-3.39697816833067));
#51843=CARTESIAN_POINT('Ctrl Pts',(-1.86285057051245,1.,-3.40251742305476));
#51844=CARTESIAN_POINT('Ctrl Pts',(-1.86797231196654,1.,-3.40797080000549));
#51845=CARTESIAN_POINT('Ctrl Pts',(-1.87311957248121,1.,-3.41335043875209));
#51846=CARTESIAN_POINT('Ctrl Pts',(-1.87830245689344,1.,-3.41867858383771));
#51847=CARTESIAN_POINT('Ctrl Pts',(-1.8835320506206,1.,-3.42397908819736));
#51848=CARTESIAN_POINT('Ctrl Pts',(-1.88881571322009,1.,-3.42926852222158));
#51849=CARTESIAN_POINT('Ctrl Pts',(-1.89415420002542,1.,-3.43455074411571));
#51850=CARTESIAN_POINT('Ctrl Pts',(-1.89954426803384,1.,-3.4398218567809));
#51851=CARTESIAN_POINT('Ctrl Pts',(-1.90498026502305,1.,-3.44507323983367));
#51852=CARTESIAN_POINT('Ctrl Pts',(-1.91045605593639,1.,-3.45029522038888));
#51853=CARTESIAN_POINT('Ctrl Pts',(-1.91596694784064,1.,-3.4554807430995));
#51854=CARTESIAN_POINT('Ctrl Pts',(-1.92151118213212,1.,-3.46062821722485));
#51855=CARTESIAN_POINT('Ctrl Pts',(-1.92708888591158,1.,-3.46573953254084));
#51856=CARTESIAN_POINT('Ctrl Pts',(-1.93270136427081,1.,-3.47081872409781));
#51857=CARTESIAN_POINT('Ctrl Pts',(-1.93835026973887,1.,-3.47587040389915));
#51858=CARTESIAN_POINT('Ctrl Pts',(-1.94403680554065,1.,-3.48089825770416));
#51859=CARTESIAN_POINT('Ctrl Pts',(-1.94976096795911,1.,-3.48590361610814));
#51860=CARTESIAN_POINT('Ctrl Pts',(-1.95552193112084,1.,-3.49088618670987));
#51861=CARTESIAN_POINT('Ctrl Pts',(-1.961318367765,1.,-3.49584466573064));
#51862=CARTESIAN_POINT('Ctrl Pts',(-1.96714879724052,1.,-3.50077740176267));
#51863=CARTESIAN_POINT('Ctrl Pts',(-1.97301191162968,1.,-3.5056830186108));
#51864=CARTESIAN_POINT('Ctrl Pts',(-1.97890693666288,1.,-3.51056110478287));
#51865=CARTESIAN_POINT('Ctrl Pts',(-1.9848335106103,1.,-3.51541198728301));
#51866=CARTESIAN_POINT('Ctrl Pts',(-1.99079153006112,1.,-3.52023644289142));
#51867=CARTESIAN_POINT('Ctrl Pts',(-1.99678100339296,1.,-3.52503542491728));
#51868=CARTESIAN_POINT('Ctrl Pts',(-2.00280191090366,1.,-3.52980980250224));
#51869=CARTESIAN_POINT('Ctrl Pts',(-2.00885403604746,1.,-3.53456004727424));
#51870=CARTESIAN_POINT('Ctrl Pts',(-2.01493698847351,1.,-3.53928627453642));
#51871=CARTESIAN_POINT('Ctrl Pts',(-2.02105027983104,1.,-3.54398838254136));
#51872=CARTESIAN_POINT('Ctrl Pts',(-2.02719338376175,1.,-3.54866616282227));
#51873=CARTESIAN_POINT('Ctrl Pts',(-2.03336579658133,1.,-3.55331941293949));
#51874=CARTESIAN_POINT('Ctrl Pts',(-2.03956711119976,1.,-3.55794807264844));
#51875=CARTESIAN_POINT('Ctrl Pts',(-2.04579702158876,1.,-3.56255223871505));
#51876=CARTESIAN_POINT('Ctrl Pts',(-2.05205528172911,1.,-3.56713209977904));
#51877=CARTESIAN_POINT('Ctrl Pts',(-2.05834167687425,1.,-3.5716878942334));
#51878=CARTESIAN_POINT('Ctrl Pts',(-2.06465599229234,1.,-3.57621986224402));
#51879=CARTESIAN_POINT('Ctrl Pts',(-2.07099797606,1.,-3.58072819250872));
#51880=CARTESIAN_POINT('Ctrl Pts',(-2.07736732842524,1.,-3.58521300039988));
#51881=CARTESIAN_POINT('Ctrl Pts',(-2.08376373049196,1.,-3.58967435355834));
#51882=CARTESIAN_POINT('Ctrl Pts',(-2.09018686331706,1.,-3.5941122862608));
#51883=CARTESIAN_POINT('Ctrl Pts',(-2.09663642986579,1.,-3.59852681775396));
#51884=CARTESIAN_POINT('Ctrl Pts',(-2.10311217727687,1.,-3.60291797087849));
#51885=CARTESIAN_POINT('Ctrl Pts',(-2.10961391333497,1.,-3.60728578530968));
#51886=CARTESIAN_POINT('Ctrl Pts',(-2.11614149813928,1.,-3.61163030607452));
#51887=CARTESIAN_POINT('Ctrl Pts',(-2.12138417125349,1.,-3.61508732215187));
#51888=CARTESIAN_POINT('Ctrl Pts',(-2.12532774376144,1.,-3.61766963589442));
#51889=CARTESIAN_POINT('Ctrl Pts',(-2.12796193131142,1.,-3.61938653648716));
#51890=CARTESIAN_POINT('Ctrl Pts',(-2.12928030988903,1.,-3.62024382630768));
#51891=CARTESIAN_POINT('Origin',(-2.12928030988903,0.,-3.62024382630768));
#51892=CARTESIAN_POINT('',(-2.25898783642071,1.,-3.54075895182139));
#51893=CARTESIAN_POINT('Origin',(0.,0.,0.));
#51894=CARTESIAN_POINT('',(-1.62064718014256,1.,-3.38171594275687));
#51895=CARTESIAN_POINT('Origin',(0.,1.,0.));
#51896=CARTESIAN_POINT('Ctrl Pts',(-1.62064718014256,1.,-3.38171594275687));
#51897=CARTESIAN_POINT('Ctrl Pts',(-1.62064718014256,0.666666666666667,
-3.38171594275687));
#51898=CARTESIAN_POINT('Ctrl Pts',(-1.62064718014256,0.333333333333333,
-3.38171594275687));
#51899=CARTESIAN_POINT('Ctrl Pts',(-1.62064718014256,-0.333333333333333,
-3.38171594275687));
#51900=CARTESIAN_POINT('Ctrl Pts',(-1.62064718014256,-0.666666666666667,
-3.38171594275687));
#51901=CARTESIAN_POINT('Ctrl Pts',(-1.62064718014256,-1.,-3.38171594275687));
#51902=CARTESIAN_POINT('Ctrl Pts',(-1.67727921511438,-1.,-3.85054988729471));
#51903=CARTESIAN_POINT('Ctrl Pts',(-1.67727921511438,1.,-3.85054988729471));
#51904=CARTESIAN_POINT('Ctrl Pts',(-1.6773605765671,-1.,-3.84897939431104));
#51905=CARTESIAN_POINT('Ctrl Pts',(-1.6773605765671,1.,-3.84897939431104));
#51906=CARTESIAN_POINT('Ctrl Pts',(-1.67751991140661,-1.,-3.84583912297567));
#51907=CARTESIAN_POINT('Ctrl Pts',(-1.67751991140661,1.,-3.84583912297567));
#51908=CARTESIAN_POINT('Ctrl Pts',(-1.67774874946867,-1.,-3.8411308598706));
#51909=CARTESIAN_POINT('Ctrl Pts',(-1.67774874946867,1.,-3.8411308598706));
#51910=CARTESIAN_POINT('Ctrl Pts',(-1.67803353065273,-1.,-3.83485746516115));
#51911=CARTESIAN_POINT('Ctrl Pts',(-1.67803353065273,1.,-3.83485746516115));
#51912=CARTESIAN_POINT('Ctrl Pts',(-1.67835555760094,-1.,-3.82702289288453));
#51913=CARTESIAN_POINT('Ctrl Pts',(-1.67835555760094,1.,-3.82702289288453));
#51914=CARTESIAN_POINT('Ctrl Pts',(-1.67864354606363,-1.,-3.81919554100522));
#51915=CARTESIAN_POINT('Ctrl Pts',(-1.67864354606363,1.,-3.81919554100522));
#51916=CARTESIAN_POINT('Ctrl Pts',(-1.67889737738311,-1.,-3.81137549624273));
#51917=CARTESIAN_POINT('Ctrl Pts',(-1.67889737738311,1.,-3.81137549624273));
#51918=CARTESIAN_POINT('Ctrl Pts',(-1.67911690648128,-1.,-3.80356289078481));
#51919=CARTESIAN_POINT('Ctrl Pts',(-1.67911690648128,1.,-3.80356289078481));
#51920=CARTESIAN_POINT('Ctrl Pts',(-1.67930196625203,-1.,-3.7957579157763));
#51921=CARTESIAN_POINT('Ctrl Pts',(-1.67930196625203,1.,-3.7957579157763));
#51922=CARTESIAN_POINT('Ctrl Pts',(-1.67945236653175,-1.,-3.78796080021026));
#51923=CARTESIAN_POINT('Ctrl Pts',(-1.67945236653175,1.,-3.78796080021026));
#51924=CARTESIAN_POINT('Ctrl Pts',(-1.67956789211943,-1.,-3.78017178196859));
#51925=CARTESIAN_POINT('Ctrl Pts',(-1.67956789211943,1.,-3.78017178196859));
#51926=CARTESIAN_POINT('Ctrl Pts',(-1.67964830084946,-1.,-3.77239107928394));
#51927=CARTESIAN_POINT('Ctrl Pts',(-1.67964830084946,1.,-3.77239107928394));
#51928=CARTESIAN_POINT('Ctrl Pts',(-1.67969332319322,-1.,-3.76461886684523));
#51929=CARTESIAN_POINT('Ctrl Pts',(-1.67969332319322,1.,-3.76461886684523));
#51930=CARTESIAN_POINT('Ctrl Pts',(-1.67970265841379,-1.,-3.75685523754816));
#51931=CARTESIAN_POINT('Ctrl Pts',(-1.67970265841379,1.,-3.75685523754816));
#51932=CARTESIAN_POINT('Ctrl Pts',(-1.67967598599665,-1.,-3.74910022394845));
#51933=CARTESIAN_POINT('Ctrl Pts',(-1.67967598599665,1.,-3.74910022394845));
#51934=CARTESIAN_POINT('Ctrl Pts',(-1.67961298685316,-1.,-3.74135385965622));
#51935=CARTESIAN_POINT('Ctrl Pts',(-1.67961298685316,1.,-3.74135385965622));
#51936=CARTESIAN_POINT('Ctrl Pts',(-1.67951336376434,-1.,-3.73361623282617));
#51937=CARTESIAN_POINT('Ctrl Pts',(-1.67951336376434,1.,-3.73361623282617));
#51938=CARTESIAN_POINT('Ctrl Pts',(-1.67937685856627,-1.,-3.72588753416339));
#51939=CARTESIAN_POINT('Ctrl Pts',(-1.67937685856627,1.,-3.72588753416339));
#51940=CARTESIAN_POINT('Ctrl Pts',(-1.6792032807165,-1.,-3.71816812842188));
#51941=CARTESIAN_POINT('Ctrl Pts',(-1.6792032807165,1.,-3.71816812842188));
#51942=CARTESIAN_POINT('Ctrl Pts',(-1.67899249793398,-1.,-3.71045854208195));
#51943=CARTESIAN_POINT('Ctrl Pts',(-1.67899249793398,1.,-3.71045854208195));
#51944=CARTESIAN_POINT('Ctrl Pts',(-1.6787443694862,-1.,-3.70275932350998));
#51945=CARTESIAN_POINT('Ctrl Pts',(-1.6787443694862,1.,-3.70275932350998));
#51946=CARTESIAN_POINT('Ctrl Pts',(-1.67845869064304,-1.,-3.69507092759545));
#51947=CARTESIAN_POINT('Ctrl Pts',(-1.67845869064304,1.,-3.69507092759545));
#51948=CARTESIAN_POINT('Ctrl Pts',(-1.67813513867973,-1.,-3.68739360236505));
#51949=CARTESIAN_POINT('Ctrl Pts',(-1.67813513867973,1.,-3.68739360236505));
#51950=CARTESIAN_POINT('Ctrl Pts',(-1.67777320475872,-1.,-3.6797272457918));
#51951=CARTESIAN_POINT('Ctrl Pts',(-1.67777320475872,1.,-3.6797272457918));
#51952=CARTESIAN_POINT('Ctrl Pts',(-1.67737217414901,-1.,-3.67207136294639));
#51953=CARTESIAN_POINT('Ctrl Pts',(-1.67737217414901,1.,-3.67207136294639));
#51954=CARTESIAN_POINT('Ctrl Pts',(-1.67693128053153,-1.,-3.66442538671018));
#51955=CARTESIAN_POINT('Ctrl Pts',(-1.67693128053153,1.,-3.66442538671018));
#51956=CARTESIAN_POINT('Ctrl Pts',(-1.67644983469459,-1.,-3.65678894416442));
#51957=CARTESIAN_POINT('Ctrl Pts',(-1.67644983469459,1.,-3.65678894416442));
#51958=CARTESIAN_POINT('Ctrl Pts',(-1.6759273594669,-1.,-3.64916213574663));
#51959=CARTESIAN_POINT('Ctrl Pts',(-1.6759273594669,1.,-3.64916213574663));
#51960=CARTESIAN_POINT('Ctrl Pts',(-1.67536373264839,-1.,-3.6415458297232));
#51961=CARTESIAN_POINT('Ctrl Pts',(-1.67536373264839,1.,-3.6415458297232));
#51962=CARTESIAN_POINT('Ctrl Pts',(-1.67475929882962,-1.,-3.63394189312902));
#51963=CARTESIAN_POINT('Ctrl Pts',(-1.67475929882962,1.,-3.63394189312902));
#51964=CARTESIAN_POINT('Ctrl Pts',(-1.67411452372265,-1.,-3.62635249450908));
#51965=CARTESIAN_POINT('Ctrl Pts',(-1.67411452372265,1.,-3.62635249450908));
#51966=CARTESIAN_POINT('Ctrl Pts',(-1.67342968196223,-1.,-3.61877947398179));
#51967=CARTESIAN_POINT('Ctrl Pts',(-1.67342968196223,1.,-3.61877947398179));
#51968=CARTESIAN_POINT('Ctrl Pts',(-1.67270452466968,-1.,-3.61122367156182));
#51969=CARTESIAN_POINT('Ctrl Pts',(-1.67270452466968,1.,-3.61122367156182));
#51970=CARTESIAN_POINT('Ctrl Pts',(-1.67193797318598,-1.,-3.60368430815203));
#51971=CARTESIAN_POINT('Ctrl Pts',(-1.67193797318598,1.,-3.60368430815203));
#51972=CARTESIAN_POINT('Ctrl Pts',(-1.67112775290706,-1.,-3.59615824388808));
#51973=CARTESIAN_POINT('Ctrl Pts',(-1.67112775290706,1.,-3.59615824388808));
#51974=CARTESIAN_POINT('Ctrl Pts',(-1.67027110397601,-1.,-3.5886414309783));
#51975=CARTESIAN_POINT('Ctrl Pts',(-1.67027110397601,1.,-3.5886414309783));
#51976=CARTESIAN_POINT('Ctrl Pts',(-1.66936552908228,-1.,-3.58113044183823));
#51977=CARTESIAN_POINT('Ctrl Pts',(-1.66936552908228,1.,-3.58113044183823));
#51978=CARTESIAN_POINT('Ctrl Pts',(-1.66840957407299,-1.,-3.57362406285884));
#51979=CARTESIAN_POINT('Ctrl Pts',(-1.66840957407299,1.,-3.57362406285884));
#51980=CARTESIAN_POINT('Ctrl Pts',(-1.66740349220308,-1.,-3.56612465179429));
#51981=CARTESIAN_POINT('Ctrl Pts',(-1.66740349220308,1.,-3.56612465179429));
#51982=CARTESIAN_POINT('Ctrl Pts',(-1.66635023293121,-1.,-3.55864015233617));
#51983=CARTESIAN_POINT('Ctrl Pts',(-1.66635023293121,1.,-3.55864015233617));
#51984=CARTESIAN_POINT('Ctrl Pts',(-1.66525401569004,-1.,-3.5511812134288));
#51985=CARTESIAN_POINT('Ctrl Pts',(-1.66525401569004,1.,-3.5511812134288));
#51986=CARTESIAN_POINT('Ctrl Pts',(-1.66411849222334,-1.,-3.5437574747503));
#51987=CARTESIAN_POINT('Ctrl Pts',(-1.66411849222334,1.,-3.5437574747503));
#51988=CARTESIAN_POINT('Ctrl Pts',(-1.66294490916113,-1.,-3.53637385060225));
#51989=CARTESIAN_POINT('Ctrl Pts',(-1.66294490916113,1.,-3.53637385060225));
#51990=CARTESIAN_POINT('Ctrl Pts',(-1.66173058912365,-1.,-3.52902746211081));
#51991=CARTESIAN_POINT('Ctrl Pts',(-1.66173058912365,1.,-3.52902746211081));
#51992=CARTESIAN_POINT('Ctrl Pts',(-1.66046645222266,-1.,-3.52170261543787));
#51993=CARTESIAN_POINT('Ctrl Pts',(-1.66046645222266,1.,-3.52170261543787));
#51994=CARTESIAN_POINT('Ctrl Pts',(-1.65913971687324,-1.,-3.51437632188903));
#51995=CARTESIAN_POINT('Ctrl Pts',(-1.65913971687324,1.,-3.51437632188903));
#51996=CARTESIAN_POINT('Ctrl Pts',(-1.65773832633617,-1.,-3.5070273314651));
#51997=CARTESIAN_POINT('Ctrl Pts',(-1.65773832633617,1.,-3.5070273314651));
#51998=CARTESIAN_POINT('Ctrl Pts',(-1.65625517961583,-1.,-3.49964476477929));
#51999=CARTESIAN_POINT('Ctrl Pts',(-1.65625517961583,1.,-3.49964476477929));
#52000=CARTESIAN_POINT('Ctrl Pts',(-1.65469162644476,-1.,-3.49223525300194));
#52001=CARTESIAN_POINT('Ctrl Pts',(-1.65469162644476,1.,-3.49223525300194));
#52002=CARTESIAN_POINT('Ctrl Pts',(-1.65306335367762,-1.,-3.48483492840942));
#52003=CARTESIAN_POINT('Ctrl Pts',(-1.65306335367762,1.,-3.48483492840942));
#52004=CARTESIAN_POINT('Ctrl Pts',(-1.65139534930353,-1.,-3.47749926256543));
#52005=CARTESIAN_POINT('Ctrl Pts',(-1.65139534930353,1.,-3.47749926256543));
#52006=CARTESIAN_POINT('Ctrl Pts',(-1.64971118698285,-1.,-3.47028140996055));
#52007=CARTESIAN_POINT('Ctrl Pts',(-1.64971118698285,1.,-3.47028140996055));
#52008=CARTESIAN_POINT('Ctrl Pts',(-1.64802323352752,-1.,-3.46321237515029));
#52009=CARTESIAN_POINT('Ctrl Pts',(-1.64802323352752,1.,-3.46321237515029));
#52010=CARTESIAN_POINT('Ctrl Pts',(-1.64632429697506,-1.,-3.4562842106239));
#52011=CARTESIAN_POINT('Ctrl Pts',(-1.64632429697506,1.,-3.4562842106239));
#52012=CARTESIAN_POINT('Ctrl Pts',(-1.64457408708059,-1.,-3.44942242546693));
#52013=CARTESIAN_POINT('Ctrl Pts',(-1.64457408708059,1.,-3.44942242546693));
#52014=CARTESIAN_POINT('Ctrl Pts',(-1.64270733821042,-1.,-3.44250337701736));
#52015=CARTESIAN_POINT('Ctrl Pts',(-1.64270733821042,1.,-3.44250337701736));
#52016=CARTESIAN_POINT('Ctrl Pts',(-1.64065778701952,-1.,-3.43540451921397));
#52017=CARTESIAN_POINT('Ctrl Pts',(-1.64065778701952,1.,-3.43540451921397));
#52018=CARTESIAN_POINT('Ctrl Pts',(-1.6383787624689,-1.,-3.42804772926213));
#52019=CARTESIAN_POINT('Ctrl Pts',(-1.6383787624689,1.,-3.42804772926213));
#52020=CARTESIAN_POINT('Ctrl Pts',(-1.63586250099804,-1.,-3.4204397459095));
#52021=CARTESIAN_POINT('Ctrl Pts',(-1.63586250099804,1.,-3.4204397459095));
#52022=CARTESIAN_POINT('Ctrl Pts',(-1.63316667054156,-1.,-3.41272817148719));
#52023=CARTESIAN_POINT('Ctrl Pts',(-1.63316667054156,1.,-3.41272817148719));
#52024=CARTESIAN_POINT('Ctrl Pts',(-1.63041148964996,-1.,-3.40519422740596));
#52025=CARTESIAN_POINT('Ctrl Pts',(-1.63041148964996,1.,-3.40519422740596));
#52026=CARTESIAN_POINT('Ctrl Pts',(-1.62774916464571,-1.,-3.39818605298342));
#52027=CARTESIAN_POINT('Ctrl Pts',(-1.62774916464571,1.,-3.39818605298342));
#52028=CARTESIAN_POINT('Ctrl Pts',(-1.62533996116793,-1.,-3.39206617497078));
#52029=CARTESIAN_POINT('Ctrl Pts',(-1.62533996116793,1.,-3.39206617497078));
#52030=CARTESIAN_POINT('Ctrl Pts',(-1.62332788556183,-1.,-3.38715832178929));
#52031=CARTESIAN_POINT('Ctrl Pts',(-1.62332788556183,1.,-3.38715832178929));
#52032=CARTESIAN_POINT('Ctrl Pts',(-1.62181089631134,-1.,-3.38368201668123));
#52033=CARTESIAN_POINT('Ctrl Pts',(-1.62181089631134,1.,-3.38368201668123));
#52034=CARTESIAN_POINT('Ctrl Pts',(-1.62103022180917,-1.,-3.38212861099481));
#52035=CARTESIAN_POINT('Ctrl Pts',(-1.62103022180917,1.,-3.38212861099481));
#52036=CARTESIAN_POINT('Ctrl Pts',(-1.6206953236804,-1.,-3.38166984193496));
#52037=CARTESIAN_POINT('Ctrl Pts',(-1.6206953236804,1.,-3.38166984193496));
#52038=CARTESIAN_POINT('Ctrl Pts',(-1.62058335162421,-1.,-3.38167767992546));
#52039=CARTESIAN_POINT('Ctrl Pts',(-1.62058335162421,1.,-3.38167767992546));
#52040=CARTESIAN_POINT('Ctrl Pts',(-1.62055519152809,-1.,-3.38176002566879));
#52041=CARTESIAN_POINT('Ctrl Pts',(-1.62055519152809,1.,-3.38176002566879));
#52042=CARTESIAN_POINT('',(-1.67727921511438,1.,-3.85054988729471));
#52043=CARTESIAN_POINT('Ctrl Pts',(-1.67727921511438,1.,-3.85054988729471));
#52044=CARTESIAN_POINT('Ctrl Pts',(-1.6773605765671,1.,-3.84897939431104));
#52045=CARTESIAN_POINT('Ctrl Pts',(-1.67751991140661,1.,-3.84583912297567));
#52046=CARTESIAN_POINT('Ctrl Pts',(-1.67774874946867,1.,-3.8411308598706));
#52047=CARTESIAN_POINT('Ctrl Pts',(-1.67803353065273,1.,-3.83485746516115));
#52048=CARTESIAN_POINT('Ctrl Pts',(-1.67835555760094,1.,-3.82702289288453));
#52049=CARTESIAN_POINT('Ctrl Pts',(-1.67864354606363,1.,-3.81919554100522));
#52050=CARTESIAN_POINT('Ctrl Pts',(-1.67889737738311,1.,-3.81137549624273));
#52051=CARTESIAN_POINT('Ctrl Pts',(-1.67911690648128,1.,-3.80356289078481));
#52052=CARTESIAN_POINT('Ctrl Pts',(-1.67930196625203,1.,-3.7957579157763));
#52053=CARTESIAN_POINT('Ctrl Pts',(-1.67945236653175,1.,-3.78796080021026));
#52054=CARTESIAN_POINT('Ctrl Pts',(-1.67956789211943,1.,-3.78017178196859));
#52055=CARTESIAN_POINT('Ctrl Pts',(-1.67964830084946,1.,-3.77239107928394));
#52056=CARTESIAN_POINT('Ctrl Pts',(-1.67969332319322,1.,-3.76461886684523));
#52057=CARTESIAN_POINT('Ctrl Pts',(-1.67970265841379,1.,-3.75685523754816));
#52058=CARTESIAN_POINT('Ctrl Pts',(-1.67967598599665,1.,-3.74910022394845));
#52059=CARTESIAN_POINT('Ctrl Pts',(-1.67961298685316,1.,-3.74135385965622));
#52060=CARTESIAN_POINT('Ctrl Pts',(-1.67951336376434,1.,-3.73361623282617));
#52061=CARTESIAN_POINT('Ctrl Pts',(-1.67937685856627,1.,-3.72588753416339));
#52062=CARTESIAN_POINT('Ctrl Pts',(-1.6792032807165,1.,-3.71816812842188));
#52063=CARTESIAN_POINT('Ctrl Pts',(-1.67899249793398,1.,-3.71045854208195));
#52064=CARTESIAN_POINT('Ctrl Pts',(-1.6787443694862,1.,-3.70275932350998));
#52065=CARTESIAN_POINT('Ctrl Pts',(-1.67845869064304,1.,-3.69507092759545));
#52066=CARTESIAN_POINT('Ctrl Pts',(-1.67813513867973,1.,-3.68739360236505));
#52067=CARTESIAN_POINT('Ctrl Pts',(-1.67777320475872,1.,-3.6797272457918));
#52068=CARTESIAN_POINT('Ctrl Pts',(-1.67737217414901,1.,-3.67207136294639));
#52069=CARTESIAN_POINT('Ctrl Pts',(-1.67693128053153,1.,-3.66442538671018));
#52070=CARTESIAN_POINT('Ctrl Pts',(-1.67644983469459,1.,-3.65678894416442));
#52071=CARTESIAN_POINT('Ctrl Pts',(-1.6759273594669,1.,-3.64916213574663));
#52072=CARTESIAN_POINT('Ctrl Pts',(-1.67536373264839,1.,-3.6415458297232));
#52073=CARTESIAN_POINT('Ctrl Pts',(-1.67475929882962,1.,-3.63394189312902));
#52074=CARTESIAN_POINT('Ctrl Pts',(-1.67411452372265,1.,-3.62635249450908));
#52075=CARTESIAN_POINT('Ctrl Pts',(-1.67342968196223,1.,-3.61877947398179));
#52076=CARTESIAN_POINT('Ctrl Pts',(-1.67270452466968,1.,-3.61122367156182));
#52077=CARTESIAN_POINT('Ctrl Pts',(-1.67193797318598,1.,-3.60368430815203));
#52078=CARTESIAN_POINT('Ctrl Pts',(-1.67112775290706,1.,-3.59615824388808));
#52079=CARTESIAN_POINT('Ctrl Pts',(-1.67027110397601,1.,-3.5886414309783));
#52080=CARTESIAN_POINT('Ctrl Pts',(-1.66936552908228,1.,-3.58113044183823));
#52081=CARTESIAN_POINT('Ctrl Pts',(-1.66840957407299,1.,-3.57362406285884));
#52082=CARTESIAN_POINT('Ctrl Pts',(-1.66740349220308,1.,-3.56612465179429));
#52083=CARTESIAN_POINT('Ctrl Pts',(-1.66635023293121,1.,-3.55864015233617));
#52084=CARTESIAN_POINT('Ctrl Pts',(-1.66525401569004,1.,-3.5511812134288));
#52085=CARTESIAN_POINT('Ctrl Pts',(-1.66411849222334,1.,-3.5437574747503));
#52086=CARTESIAN_POINT('Ctrl Pts',(-1.66294490916113,1.,-3.53637385060225));
#52087=CARTESIAN_POINT('Ctrl Pts',(-1.66173058912365,1.,-3.52902746211081));
#52088=CARTESIAN_POINT('Ctrl Pts',(-1.66046645222266,1.,-3.52170261543787));
#52089=CARTESIAN_POINT('Ctrl Pts',(-1.65913971687324,1.,-3.51437632188903));
#52090=CARTESIAN_POINT('Ctrl Pts',(-1.65773832633617,1.,-3.5070273314651));
#52091=CARTESIAN_POINT('Ctrl Pts',(-1.65625517961583,1.,-3.49964476477929));
#52092=CARTESIAN_POINT('Ctrl Pts',(-1.65469162644476,1.,-3.49223525300194));
#52093=CARTESIAN_POINT('Ctrl Pts',(-1.65306335367762,1.,-3.48483492840942));
#52094=CARTESIAN_POINT('Ctrl Pts',(-1.65139534930353,1.,-3.47749926256543));
#52095=CARTESIAN_POINT('Ctrl Pts',(-1.64971118698285,1.,-3.47028140996055));
#52096=CARTESIAN_POINT('Ctrl Pts',(-1.64802323352752,1.,-3.46321237515029));
#52097=CARTESIAN_POINT('Ctrl Pts',(-1.64632429697506,1.,-3.4562842106239));
#52098=CARTESIAN_POINT('Ctrl Pts',(-1.64457408708059,1.,-3.44942242546693));
#52099=CARTESIAN_POINT('Ctrl Pts',(-1.64270733821042,1.,-3.44250337701736));
#52100=CARTESIAN_POINT('Ctrl Pts',(-1.64065778701952,1.,-3.43540451921397));
#52101=CARTESIAN_POINT('Ctrl Pts',(-1.6383787624689,1.,-3.42804772926213));
#52102=CARTESIAN_POINT('Ctrl Pts',(-1.63586250099804,1.,-3.4204397459095));
#52103=CARTESIAN_POINT('Ctrl Pts',(-1.63316667054156,1.,-3.41272817148719));
#52104=CARTESIAN_POINT('Ctrl Pts',(-1.63041148964996,1.,-3.40519422740596));
#52105=CARTESIAN_POINT('Ctrl Pts',(-1.62774916464571,1.,-3.39818605298342));
#52106=CARTESIAN_POINT('Ctrl Pts',(-1.62533996116793,1.,-3.39206617497078));
#52107=CARTESIAN_POINT('Ctrl Pts',(-1.62332788556183,1.,-3.38715832178929));
#52108=CARTESIAN_POINT('Ctrl Pts',(-1.62192472202795,1.,-3.3839428576331));
#52109=CARTESIAN_POINT('Ctrl Pts',(-1.62118047294574,1.,-3.38243080602536));
#52110=CARTESIAN_POINT('Ctrl Pts',(-1.62083271136059,1.,-3.38187506457001));
#52111=CARTESIAN_POINT('Ctrl Pts',(-1.62069086551626,1.,-3.38173802621243));
#52112=CARTESIAN_POINT('Ctrl Pts',(-1.62064718014256,1.,-3.38171594275687));
#52113=CARTESIAN_POINT('',(-1.67727921511438,0.,-3.85054988729471));
#52114=CARTESIAN_POINT('Ctrl Pts',(-1.24535988127942,-1.,-3.53717101171257));
#52115=CARTESIAN_POINT('Ctrl Pts',(-1.24535988127942,1.,-3.53717101171257));
#52116=CARTESIAN_POINT('Ctrl Pts',(-1.24528174185147,-1.,-3.53713269667534));
#52117=CARTESIAN_POINT('Ctrl Pts',(-1.24528174185147,1.,-3.53713269667534));
#52118=CARTESIAN_POINT('Ctrl Pts',(-1.2451970233558,-1.,-3.53720633058152));
#52119=CARTESIAN_POINT('Ctrl Pts',(-1.2451970233558,1.,-3.53720633058152));
#52120=CARTESIAN_POINT('Ctrl Pts',(-1.24528461333177,-1.,-3.53776753803428));
#52121=CARTESIAN_POINT('Ctrl Pts',(-1.24528461333177,1.,-3.53776753803428));
#52122=CARTESIAN_POINT('Ctrl Pts',(-1.24583101679199,-1.,-3.53941798196293));
#52123=CARTESIAN_POINT('Ctrl Pts',(-1.24583101679199,1.,-3.53941798196293));
#52124=CARTESIAN_POINT('Ctrl Pts',(-1.2472164623202,-1.,-3.54294877426113));
#52125=CARTESIAN_POINT('Ctrl Pts',(-1.2472164623202,1.,-3.54294877426113));
#52126=CARTESIAN_POINT('Ctrl Pts',(-1.24926408627938,-1.,-3.54784190282889));
#52127=CARTESIAN_POINT('Ctrl Pts',(-1.24926408627938,1.,-3.54784190282889));
#52128=CARTESIAN_POINT('Ctrl Pts',(-1.25188792940508,-1.,-3.5538728741862));
#52129=CARTESIAN_POINT('Ctrl Pts',(-1.25188792940508,1.,-3.5538728741862));
#52130=CARTESIAN_POINT('Ctrl Pts',(-1.25496090899873,-1.,-3.56071094990825));
#52131=CARTESIAN_POINT('Ctrl Pts',(-1.25496090899873,1.,-3.56071094990825));
#52132=CARTESIAN_POINT('Ctrl Pts',(-1.25834000485626,-1.,-3.56798645995025));
#52133=CARTESIAN_POINT('Ctrl Pts',(-1.25834000485626,1.,-3.56798645995025));
#52134=CARTESIAN_POINT('Ctrl Pts',(-1.26188667142784,-1.,-3.5753456065164));
#52135=CARTESIAN_POINT('Ctrl Pts',(-1.26188667142784,1.,-3.5753456065164));
#52136=CARTESIAN_POINT('Ctrl Pts',(-1.26548706249891,-1.,-3.58250452868699));
#52137=CARTESIAN_POINT('Ctrl Pts',(-1.26548706249891,1.,-3.58250452868699));
#52138=CARTESIAN_POINT('Ctrl Pts',(-1.26907758484766,-1.,-3.5893180784647));
#52139=CARTESIAN_POINT('Ctrl Pts',(-1.26907758484766,1.,-3.5893180784647));
#52140=CARTESIAN_POINT('Ctrl Pts',(-1.27264798379365,-1.,-3.59578698050164));
#52141=CARTESIAN_POINT('Ctrl Pts',(-1.27264798379365,1.,-3.59578698050164));
#52142=CARTESIAN_POINT('Ctrl Pts',(-1.27622049908664,-1.,-3.60199947736404));
#52143=CARTESIAN_POINT('Ctrl Pts',(-1.27622049908664,1.,-3.60199947736404));
#52144=CARTESIAN_POINT('Ctrl Pts',(-1.27983492861703,-1.,-3.60808907746372));
#52145=CARTESIAN_POINT('Ctrl Pts',(-1.27983492861703,1.,-3.60808907746372));
#52146=CARTESIAN_POINT('Ctrl Pts',(-1.28353255117754,-1.,-3.61418935913793));
#52147=CARTESIAN_POINT('Ctrl Pts',(-1.28353255117754,1.,-3.61418935913793));
#52148=CARTESIAN_POINT('Ctrl Pts',(-1.2873375502936,-1.,-3.62038148492295));
#52149=CARTESIAN_POINT('Ctrl Pts',(-1.2873375502936,1.,-3.62038148492295));
#52150=CARTESIAN_POINT('Ctrl Pts',(-1.29125046021853,-1.,-3.62667616004299));
#52151=CARTESIAN_POINT('Ctrl Pts',(-1.29125046021853,1.,-3.62667616004299));
#52152=CARTESIAN_POINT('Ctrl Pts',(-1.29525810207744,-1.,-3.63304271630995));
#52153=CARTESIAN_POINT('Ctrl Pts',(-1.29525810207744,1.,-3.63304271630995));
#52154=CARTESIAN_POINT('Ctrl Pts',(-1.29933955906463,-1.,-3.6394268987279));
#52155=CARTESIAN_POINT('Ctrl Pts',(-1.29933955906463,1.,-3.6394268987279));
#52156=CARTESIAN_POINT('Ctrl Pts',(-1.30347327603778,-1.,-3.64577181380125));
#52157=CARTESIAN_POINT('Ctrl Pts',(-1.30347327603778,1.,-3.64577181380125));
#52158=CARTESIAN_POINT('Ctrl Pts',(-1.30764479590051,-1.,-3.65204081987101));
#52159=CARTESIAN_POINT('Ctrl Pts',(-1.30764479590051,1.,-3.65204081987101));
#52160=CARTESIAN_POINT('Ctrl Pts',(-1.31185038411231,-1.,-3.65822827358655));
#52161=CARTESIAN_POINT('Ctrl Pts',(-1.31185038411231,1.,-3.65822827358655));
#52162=CARTESIAN_POINT('Ctrl Pts',(-1.31609271239922,-1.,-3.66434688899822));
#52163=CARTESIAN_POINT('Ctrl Pts',(-1.31609271239922,1.,-3.66434688899822));
#52164=CARTESIAN_POINT('Ctrl Pts',(-1.3203782813777,-1.,-3.67042021752668));
#52165=CARTESIAN_POINT('Ctrl Pts',(-1.3203782813777,1.,-3.67042021752668));
#52166=CARTESIAN_POINT('Ctrl Pts',(-1.32471430856413,-1.,-3.67647355257906));
#52167=CARTESIAN_POINT('Ctrl Pts',(-1.32471430856413,1.,-3.67647355257906));
#52168=CARTESIAN_POINT('Ctrl Pts',(-1.32910547072734,-1.,-3.68252441182534));
#52169=CARTESIAN_POINT('Ctrl Pts',(-1.32910547072734,1.,-3.68252441182534));
#52170=CARTESIAN_POINT('Ctrl Pts',(-1.33355191034515,-1.,-3.68857672413013));
#52171=CARTESIAN_POINT('Ctrl Pts',(-1.33355191034515,1.,-3.68857672413013));
#52172=CARTESIAN_POINT('Ctrl Pts',(-1.33805103398214,-1.,-3.69462613305692));
#52173=CARTESIAN_POINT('Ctrl Pts',(-1.33805103398214,1.,-3.69462613305692));
#52174=CARTESIAN_POINT('Ctrl Pts',(-1.3425986075293,-1.,-3.70066324015112));
#52175=CARTESIAN_POINT('Ctrl Pts',(-1.3425986075293,1.,-3.70066324015112));
#52176=CARTESIAN_POINT('Ctrl Pts',(-1.34719008463535,-1.,-3.7066775318825));
#52177=CARTESIAN_POINT('Ctrl Pts',(-1.34719008463535,1.,-3.7066775318825));
#52178=CARTESIAN_POINT('Ctrl Pts',(-1.35182193384426,-1.,-3.71266130563061));
#52179=CARTESIAN_POINT('Ctrl Pts',(-1.35182193384426,1.,-3.71266130563061));
#52180=CARTESIAN_POINT('Ctrl Pts',(-1.35649266705038,-1.,-3.71861271513318));
#52181=CARTESIAN_POINT('Ctrl Pts',(-1.35649266705038,1.,-3.71861271513318));
#52182=CARTESIAN_POINT('Ctrl Pts',(-1.36120211416353,-1.,-3.72453364678279));
#52183=CARTESIAN_POINT('Ctrl Pts',(-1.36120211416353,1.,-3.72453364678279));
#52184=CARTESIAN_POINT('Ctrl Pts',(-1.36595093298674,-1.,-3.73042829011293));
#52185=CARTESIAN_POINT('Ctrl Pts',(-1.36595093298674,1.,-3.73042829011293));
#52186=CARTESIAN_POINT('Ctrl Pts',(-1.37074003422739,-1.,-3.73630145885809));
#52187=CARTESIAN_POINT('Ctrl Pts',(-1.37074003422739,1.,-3.73630145885809));
#52188=CARTESIAN_POINT('Ctrl Pts',(-1.3755700297169,-1.,-3.7421569816256));
#52189=CARTESIAN_POINT('Ctrl Pts',(-1.3755700297169,1.,-3.7421569816256));
#52190=CARTESIAN_POINT('Ctrl Pts',(-1.38044070763302,-1.,-3.74799617204744));
#52191=CARTESIAN_POINT('Ctrl Pts',(-1.38044070763302,1.,-3.74799617204744));
#52192=CARTESIAN_POINT('Ctrl Pts',(-1.38535129801185,-1.,-3.75381861212728));
#52193=CARTESIAN_POINT('Ctrl Pts',(-1.38535129801185,1.,-3.75381861212728));
#52194=CARTESIAN_POINT('Ctrl Pts',(-1.39030069388926,-1.,-3.75962280650875));
#52195=CARTESIAN_POINT('Ctrl Pts',(-1.39030069388926,1.,-3.75962280650875));
#52196=CARTESIAN_POINT('Ctrl Pts',(-1.39528769118054,-1.,-3.76540689249078));
#52197=CARTESIAN_POINT('Ctrl Pts',(-1.39528769118054,1.,-3.76540689249078));
#52198=CARTESIAN_POINT('Ctrl Pts',(-1.40031121335495,-1.,-3.77116930621804));
#52199=CARTESIAN_POINT('Ctrl Pts',(-1.40031121335495,1.,-3.77116930621804));
#52200=CARTESIAN_POINT('Ctrl Pts',(-1.40537056004702,-1.,-3.77690952014209));
#52201=CARTESIAN_POINT('Ctrl Pts',(-1.40537056004702,1.,-3.77690952014209));
#52202=CARTESIAN_POINT('Ctrl Pts',(-1.41046532282567,-1.,-3.78262780065406));
#52203=CARTESIAN_POINT('Ctrl Pts',(-1.41046532282567,1.,-3.78262780065406));
#52204=CARTESIAN_POINT('Ctrl Pts',(-1.41559527803808,-1.,-3.78832489879369));
#52205=CARTESIAN_POINT('Ctrl Pts',(-1.41559527803808,1.,-3.78832489879369));
#52206=CARTESIAN_POINT('Ctrl Pts',(-1.42076028482828,-1.,-3.7940017574439));
#52207=CARTESIAN_POINT('Ctrl Pts',(-1.42076028482828,1.,-3.7940017574439));
#52208=CARTESIAN_POINT('Ctrl Pts',(-1.42596018777301,-1.,-3.79965923196365));
#52209=CARTESIAN_POINT('Ctrl Pts',(-1.42596018777301,1.,-3.79965923196365));
#52210=CARTESIAN_POINT('Ctrl Pts',(-1.43119469921364,-1.,-3.80529775429916));
#52211=CARTESIAN_POINT('Ctrl Pts',(-1.43119469921364,1.,-3.80529775429916));
#52212=CARTESIAN_POINT('Ctrl Pts',(-1.43646341556783,-1.,-3.81091737726965));
#52213=CARTESIAN_POINT('Ctrl Pts',(-1.43646341556783,1.,-3.81091737726965));
#52214=CARTESIAN_POINT('Ctrl Pts',(-1.44176587041401,-1.,-3.8165179239855));
#52215=CARTESIAN_POINT('Ctrl Pts',(-1.44176587041401,1.,-3.8165179239855));
#52216=CARTESIAN_POINT('Ctrl Pts',(-1.44710157648562,-1.,-3.82209910620591));
#52217=CARTESIAN_POINT('Ctrl Pts',(-1.44710157648562,1.,-3.82209910620591));
#52218=CARTESIAN_POINT('Ctrl Pts',(-1.45247006796807,-1.,-3.82766064519));
#52219=CARTESIAN_POINT('Ctrl Pts',(-1.45247006796807,1.,-3.82766064519));
#52220=CARTESIAN_POINT('Ctrl Pts',(-1.45787095220763,-1.,-3.83320241775199));
#52221=CARTESIAN_POINT('Ctrl Pts',(-1.45787095220763,1.,-3.83320241775199));
#52222=CARTESIAN_POINT('Ctrl Pts',(-1.46330391180621,-1.,-3.83872447159309));
#52223=CARTESIAN_POINT('Ctrl Pts',(-1.46330391180621,1.,-3.83872447159309));
#52224=CARTESIAN_POINT('Ctrl Pts',(-1.46876867426375,-1.,-3.84422695454469));
#52225=CARTESIAN_POINT('Ctrl Pts',(-1.46876867426375,1.,-3.84422695454469));
#52226=CARTESIAN_POINT('Ctrl Pts',(-1.47426499018467,-1.,-3.84971006847096));
#52227=CARTESIAN_POINT('Ctrl Pts',(-1.47426499018467,1.,-3.84971006847096));
#52228=CARTESIAN_POINT('Ctrl Pts',(-1.47979260991063,-1.,-3.85517401698952));
#52229=CARTESIAN_POINT('Ctrl Pts',(-1.47979260991063,1.,-3.85517401698952));
#52230=CARTESIAN_POINT('Ctrl Pts',(-1.48535125510102,-1.,-3.86061894706551));
#52231=CARTESIAN_POINT('Ctrl Pts',(-1.48535125510102,1.,-3.86061894706551));
#52232=CARTESIAN_POINT('Ctrl Pts',(-1.49094061164604,-1.,-3.86604492575933));
#52233=CARTESIAN_POINT('Ctrl Pts',(-1.49094061164604,1.,-3.86604492575933));
#52234=CARTESIAN_POINT('Ctrl Pts',(-1.4965603539944,-1.,-3.8714519699927));
#52235=CARTESIAN_POINT('Ctrl Pts',(-1.4965603539944,1.,-3.8714519699927));
#52236=CARTESIAN_POINT('Ctrl Pts',(-1.50221016176766,-1.,-3.87684006372665));
#52237=CARTESIAN_POINT('Ctrl Pts',(-1.50221016176766,1.,-3.87684006372665));
#52238=CARTESIAN_POINT('Ctrl Pts',(-1.50788973857719,-1.,-3.88220917950443));
#52239=CARTESIAN_POINT('Ctrl Pts',(-1.50788973857719,1.,-3.88220917950443));
#52240=CARTESIAN_POINT('Ctrl Pts',(-1.51359883110181,-1.,-3.88755930032927));
#52241=CARTESIAN_POINT('Ctrl Pts',(-1.51359883110181,1.,-3.88755930032927));
#52242=CARTESIAN_POINT('Ctrl Pts',(-1.51933724328609,-1.,-3.89289043531893));
#52243=CARTESIAN_POINT('Ctrl Pts',(-1.51933724328609,1.,-3.89289043531893));
#52244=CARTESIAN_POINT('Ctrl Pts',(-1.52510482990784,-1.,-3.8982026070607));
#52245=CARTESIAN_POINT('Ctrl Pts',(-1.52510482990784,1.,-3.8982026070607));
#52246=CARTESIAN_POINT('Ctrl Pts',(-1.5297421605556,-1.,-3.90243719629755));
#52247=CARTESIAN_POINT('Ctrl Pts',(-1.5297421605556,1.,-3.90243719629755));
#52248=CARTESIAN_POINT('Ctrl Pts',(-1.53323321827311,-1.,-3.90560462812846));
#52249=CARTESIAN_POINT('Ctrl Pts',(-1.53323321827311,1.,-3.90560462812846));
#52250=CARTESIAN_POINT('Ctrl Pts',(-1.53556639217742,-1.,-3.90771246854607));
#52251=CARTESIAN_POINT('Ctrl Pts',(-1.53556639217742,1.,-3.90771246854607));
#52252=CARTESIAN_POINT('Ctrl Pts',(-1.53673442965255,-1.,-3.90876544355381));
#52253=CARTESIAN_POINT('Ctrl Pts',(-1.53673442965255,1.,-3.90876544355381));
#52254=CARTESIAN_POINT('',(-1.24526366418208,1.,-3.5372048861591));
#52255=CARTESIAN_POINT('Ctrl Pts',(-1.24526366418208,-1.,-3.5372048861591));
#52256=CARTESIAN_POINT('Ctrl Pts',(-1.24526366418208,-0.666666666666667,
-3.5372048861591));
#52257=CARTESIAN_POINT('Ctrl Pts',(-1.24526366418208,-0.333333333333333,
-3.5372048861591));
#52258=CARTESIAN_POINT('Ctrl Pts',(-1.24526366418208,0.333333333333333,
-3.5372048861591));
#52259=CARTESIAN_POINT('Ctrl Pts',(-1.24526366418208,0.666666666666667,
-3.5372048861591));
#52260=CARTESIAN_POINT('Ctrl Pts',(-1.24526366418208,1.,-3.5372048861591));
#52261=CARTESIAN_POINT('',(-1.53673442965255,1.,-3.90876544355381));
#52262=CARTESIAN_POINT('',(-1.53673442965255,0.,-3.90876544355381));
#52263=CARTESIAN_POINT('Ctrl Pts',(-1.24526366418208,1.,-3.5372048861591));
#52264=CARTESIAN_POINT('Ctrl Pts',(-1.24524838931864,1.,-3.53725139174402));
#52265=CARTESIAN_POINT('Ctrl Pts',(-1.24524498991133,1.,-3.53744859265385));
#52266=CARTESIAN_POINT('Ctrl Pts',(-1.2453920538873,1.,-3.53808746578052));
#52267=CARTESIAN_POINT('Ctrl Pts',(-1.24593497225964,1.,-3.53968291129942));
#52268=CARTESIAN_POINT('Ctrl Pts',(-1.2472164623202,1.,-3.54294877426113));
#52269=CARTESIAN_POINT('Ctrl Pts',(-1.24926408627938,1.,-3.54784190282889));
#52270=CARTESIAN_POINT('Ctrl Pts',(-1.25188792940508,1.,-3.5538728741862));
#52271=CARTESIAN_POINT('Ctrl Pts',(-1.25496090899873,1.,-3.56071094990825));
#52272=CARTESIAN_POINT('Ctrl Pts',(-1.25834000485626,1.,-3.56798645995025));
#52273=CARTESIAN_POINT('Ctrl Pts',(-1.26188667142784,1.,-3.5753456065164));
#52274=CARTESIAN_POINT('Ctrl Pts',(-1.26548706249891,1.,-3.58250452868699));
#52275=CARTESIAN_POINT('Ctrl Pts',(-1.26907758484766,1.,-3.5893180784647));
#52276=CARTESIAN_POINT('Ctrl Pts',(-1.27264798379365,1.,-3.59578698050164));
#52277=CARTESIAN_POINT('Ctrl Pts',(-1.27622049908664,1.,-3.60199947736404));
#52278=CARTESIAN_POINT('Ctrl Pts',(-1.27983492861703,1.,-3.60808907746372));
#52279=CARTESIAN_POINT('Ctrl Pts',(-1.28353255117754,1.,-3.61418935913793));
#52280=CARTESIAN_POINT('Ctrl Pts',(-1.2873375502936,1.,-3.62038148492295));
#52281=CARTESIAN_POINT('Ctrl Pts',(-1.29125046021853,1.,-3.62667616004299));
#52282=CARTESIAN_POINT('Ctrl Pts',(-1.29525810207744,1.,-3.63304271630995));
#52283=CARTESIAN_POINT('Ctrl Pts',(-1.29933955906463,1.,-3.6394268987279));
#52284=CARTESIAN_POINT('Ctrl Pts',(-1.30347327603778,1.,-3.64577181380125));
#52285=CARTESIAN_POINT('Ctrl Pts',(-1.30764479590051,1.,-3.65204081987101));
#52286=CARTESIAN_POINT('Ctrl Pts',(-1.31185038411231,1.,-3.65822827358655));
#52287=CARTESIAN_POINT('Ctrl Pts',(-1.31609271239922,1.,-3.66434688899822));
#52288=CARTESIAN_POINT('Ctrl Pts',(-1.3203782813777,1.,-3.67042021752668));
#52289=CARTESIAN_POINT('Ctrl Pts',(-1.32471430856413,1.,-3.67647355257906));
#52290=CARTESIAN_POINT('Ctrl Pts',(-1.32910547072734,1.,-3.68252441182534));
#52291=CARTESIAN_POINT('Ctrl Pts',(-1.33355191034515,1.,-3.68857672413013));
#52292=CARTESIAN_POINT('Ctrl Pts',(-1.33805103398214,1.,-3.69462613305692));
#52293=CARTESIAN_POINT('Ctrl Pts',(-1.3425986075293,1.,-3.70066324015112));
#52294=CARTESIAN_POINT('Ctrl Pts',(-1.34719008463535,1.,-3.7066775318825));
#52295=CARTESIAN_POINT('Ctrl Pts',(-1.35182193384426,1.,-3.71266130563061));
#52296=CARTESIAN_POINT('Ctrl Pts',(-1.35649266705038,1.,-3.71861271513318));
#52297=CARTESIAN_POINT('Ctrl Pts',(-1.36120211416353,1.,-3.72453364678279));
#52298=CARTESIAN_POINT('Ctrl Pts',(-1.36595093298674,1.,-3.73042829011293));
#52299=CARTESIAN_POINT('Ctrl Pts',(-1.37074003422739,1.,-3.73630145885809));
#52300=CARTESIAN_POINT('Ctrl Pts',(-1.3755700297169,1.,-3.7421569816256));
#52301=CARTESIAN_POINT('Ctrl Pts',(-1.38044070763302,1.,-3.74799617204744));
#52302=CARTESIAN_POINT('Ctrl Pts',(-1.38535129801185,1.,-3.75381861212728));
#52303=CARTESIAN_POINT('Ctrl Pts',(-1.39030069388926,1.,-3.75962280650875));
#52304=CARTESIAN_POINT('Ctrl Pts',(-1.39528769118054,1.,-3.76540689249078));
#52305=CARTESIAN_POINT('Ctrl Pts',(-1.40031121335495,1.,-3.77116930621804));
#52306=CARTESIAN_POINT('Ctrl Pts',(-1.40537056004702,1.,-3.77690952014209));
#52307=CARTESIAN_POINT('Ctrl Pts',(-1.41046532282567,1.,-3.78262780065406));
#52308=CARTESIAN_POINT('Ctrl Pts',(-1.41559527803808,1.,-3.78832489879369));
#52309=CARTESIAN_POINT('Ctrl Pts',(-1.42076028482828,1.,-3.7940017574439));
#52310=CARTESIAN_POINT('Ctrl Pts',(-1.42596018777301,1.,-3.79965923196365));
#52311=CARTESIAN_POINT('Ctrl Pts',(-1.43119469921364,1.,-3.80529775429916));
#52312=CARTESIAN_POINT('Ctrl Pts',(-1.43646341556783,1.,-3.81091737726965));
#52313=CARTESIAN_POINT('Ctrl Pts',(-1.44176587041401,1.,-3.8165179239855));
#52314=CARTESIAN_POINT('Ctrl Pts',(-1.44710157648562,1.,-3.82209910620591));
#52315=CARTESIAN_POINT('Ctrl Pts',(-1.45247006796807,1.,-3.82766064519));
#52316=CARTESIAN_POINT('Ctrl Pts',(-1.45787095220763,1.,-3.83320241775199));
#52317=CARTESIAN_POINT('Ctrl Pts',(-1.46330391180621,1.,-3.83872447159309));
#52318=CARTESIAN_POINT('Ctrl Pts',(-1.46876867426375,1.,-3.84422695454469));
#52319=CARTESIAN_POINT('Ctrl Pts',(-1.47426499018467,1.,-3.84971006847096));
#52320=CARTESIAN_POINT('Ctrl Pts',(-1.47979260991063,1.,-3.85517401698952));
#52321=CARTESIAN_POINT('Ctrl Pts',(-1.48535125510102,1.,-3.86061894706551));
#52322=CARTESIAN_POINT('Ctrl Pts',(-1.49094061164604,1.,-3.86604492575933));
#52323=CARTESIAN_POINT('Ctrl Pts',(-1.4965603539944,1.,-3.8714519699927));
#52324=CARTESIAN_POINT('Ctrl Pts',(-1.50221016176766,1.,-3.87684006372665));
#52325=CARTESIAN_POINT('Ctrl Pts',(-1.50788973857719,1.,-3.88220917950443));
#52326=CARTESIAN_POINT('Ctrl Pts',(-1.51359883110181,1.,-3.88755930032927));
#52327=CARTESIAN_POINT('Ctrl Pts',(-1.51933724328609,1.,-3.89289043531893));
#52328=CARTESIAN_POINT('Ctrl Pts',(-1.52510482990784,1.,-3.8982026070607));
#52329=CARTESIAN_POINT('Ctrl Pts',(-1.5297421605556,1.,-3.90243719629755));
#52330=CARTESIAN_POINT('Ctrl Pts',(-1.53323321827311,1.,-3.90560462812846));
#52331=CARTESIAN_POINT('Ctrl Pts',(-1.53556639217742,1.,-3.90771246854607));
#52332=CARTESIAN_POINT('Ctrl Pts',(-1.53673442965255,1.,-3.90876544355381));
#52333=CARTESIAN_POINT('Origin',(-1.53673442965255,0.,-3.90876544355381));
#52334=CARTESIAN_POINT('',(-1.67727921511438,1.,-3.85054988729471));
#52335=CARTESIAN_POINT('Origin',(0.,0.,0.));
#52336=CARTESIAN_POINT('',(-1.071677399622,1.,-3.59360648251021));
#52337=CARTESIAN_POINT('Origin',(0.,1.,0.));
#52338=CARTESIAN_POINT('Ctrl Pts',(-1.071677399622,1.,-3.59360648251021));
#52339=CARTESIAN_POINT('Ctrl Pts',(-1.071677399622,0.666666666666667,-3.59360648251021));
#52340=CARTESIAN_POINT('Ctrl Pts',(-1.071677399622,0.333333333333333,-3.59360648251021));
#52341=CARTESIAN_POINT('Ctrl Pts',(-1.071677399622,-0.333333333333333,-3.59360648251021));
#52342=CARTESIAN_POINT('Ctrl Pts',(-1.071677399622,-0.666666666666667,-3.59360648251021));
#52343=CARTESIAN_POINT('Ctrl Pts',(-1.071677399622,-1.,-3.59360648251021));
#52344=CARTESIAN_POINT('Ctrl Pts',(-1.05427041296137,-1.,-4.06552750530042));
#52345=CARTESIAN_POINT('Ctrl Pts',(-1.05427041296137,1.,-4.06552750530042));
#52346=CARTESIAN_POINT('Ctrl Pts',(-1.05459645194934,-1.,-4.06398907542679));
#52347=CARTESIAN_POINT('Ctrl Pts',(-1.05459645194934,1.,-4.06398907542679));
#52348=CARTESIAN_POINT('Ctrl Pts',(-1.05524507177901,-1.,-4.06091239150293));
#52349=CARTESIAN_POINT('Ctrl Pts',(-1.05524507177901,1.,-4.06091239150293));
#52350=CARTESIAN_POINT('Ctrl Pts',(-1.0562076270849,-1.,-4.05629789308941));
#52351=CARTESIAN_POINT('Ctrl Pts',(-1.0562076270849,1.,-4.05629789308941));
#52352=CARTESIAN_POINT('Ctrl Pts',(-1.05747027728537,-1.,-4.05014628387112));
#52353=CARTESIAN_POINT('Ctrl Pts',(-1.05747027728537,1.,-4.05014628387112));
#52354=CARTESIAN_POINT('Ctrl Pts',(-1.05901393667039,-1.,-4.04245854429333));
#52355=CARTESIAN_POINT('Ctrl Pts',(-1.05901393667039,1.,-4.04245854429333));
#52356=CARTESIAN_POINT('Ctrl Pts',(-1.06052284712114,-1.,-4.03477261142549));
#52357=CARTESIAN_POINT('Ctrl Pts',(-1.06052284712114,1.,-4.03477261142549));
#52358=CARTESIAN_POINT('Ctrl Pts',(-1.06199687787488,-1.,-4.02708855235732));
#52359=CARTESIAN_POINT('Ctrl Pts',(-1.06199687787488,1.,-4.02708855235732));
#52360=CARTESIAN_POINT('Ctrl Pts',(-1.06343586496094,-1.,-4.0194064749539));
#52361=CARTESIAN_POINT('Ctrl Pts',(-1.06343586496094,1.,-4.0194064749539));
#52362=CARTESIAN_POINT('Ctrl Pts',(-1.06483961342894,-1.,-4.0117265418656));
#52363=CARTESIAN_POINT('Ctrl Pts',(-1.06483961342894,1.,-4.0117265418656));
#52364=CARTESIAN_POINT('Ctrl Pts',(-1.06620789963406,-1.,-4.00404894951804));
#52365=CARTESIAN_POINT('Ctrl Pts',(-1.06620789963406,1.,-4.00404894951804));
#52366=CARTESIAN_POINT('Ctrl Pts',(-1.06754047381188,-1.,-3.99637389919958));
#52367=CARTESIAN_POINT('Ctrl Pts',(-1.06754047381188,1.,-3.99637389919958));
#52368=CARTESIAN_POINT('Ctrl Pts',(-1.06883706263912,-1.,-3.98870156857298));
#52369=CARTESIAN_POINT('Ctrl Pts',(-1.06883706263912,1.,-3.98870156857298));
#52370=CARTESIAN_POINT('Ctrl Pts',(-1.07009737257815,-1.,-3.98103208801289));
#52371=CARTESIAN_POINT('Ctrl Pts',(-1.07009737257815,1.,-3.98103208801289));
#52372=CARTESIAN_POINT('Ctrl Pts',(-1.07132109206252,-1.,-3.97336550222571));
#52373=CARTESIAN_POINT('Ctrl Pts',(-1.07132109206252,1.,-3.97336550222571));
#52374=CARTESIAN_POINT('Ctrl Pts',(-1.07250789943095,-1.,-3.96570179322681));
#52375=CARTESIAN_POINT('Ctrl Pts',(-1.07250789943095,1.,-3.96570179322681));
#52376=CARTESIAN_POINT('Ctrl Pts',(-1.07365747426551,-1.,-3.95804094429606));
#52377=CARTESIAN_POINT('Ctrl Pts',(-1.07365747426551,1.,-3.95804094429606));
#52378=CARTESIAN_POINT('Ctrl Pts',(-1.07476950921607,-1.,-3.95038299600754));
#52379=CARTESIAN_POINT('Ctrl Pts',(-1.07476950921607,1.,-3.95038299600754));
#52380=CARTESIAN_POINT('Ctrl Pts',(-1.07584371946428,-1.,-3.94272809633271));
#52381=CARTESIAN_POINT('Ctrl Pts',(-1.07584371946428,1.,-3.94272809633271));
#52382=CARTESIAN_POINT('Ctrl Pts',(-1.07687985975348,-1.,-3.93507657572743));
#52383=CARTESIAN_POINT('Ctrl Pts',(-1.07687985975348,1.,-3.93507657572743));
#52384=CARTESIAN_POINT('Ctrl Pts',(-1.07787771707155,-1.,-3.92742893349684));
#52385=CARTESIAN_POINT('Ctrl Pts',(-1.07787771707155,1.,-3.92742893349684));
#52386=CARTESIAN_POINT('Ctrl Pts',(-1.07883706663524,-1.,-3.91978568924062));
#52387=CARTESIAN_POINT('Ctrl Pts',(-1.07883706663524,1.,-3.91978568924062));
#52388=CARTESIAN_POINT('Ctrl Pts',(-1.0797576350746,-1.,-3.91214726022096));
#52389=CARTESIAN_POINT('Ctrl Pts',(-1.0797576350746,1.,-3.91214726022096));
#52390=CARTESIAN_POINT('Ctrl Pts',(-1.08063906483822,-1.,-3.90451384092564));
#52391=CARTESIAN_POINT('Ctrl Pts',(-1.08063906483822,1.,-3.90451384092564));
#52392=CARTESIAN_POINT('Ctrl Pts',(-1.08148086931373,-1.,-3.89688525098408));
#52393=CARTESIAN_POINT('Ctrl Pts',(-1.08148086931373,1.,-3.89688525098408));
#52394=CARTESIAN_POINT('Ctrl Pts',(-1.08228241999363,-1.,-3.88926088975182));
#52395=CARTESIAN_POINT('Ctrl Pts',(-1.08228241999363,1.,-3.88926088975182));
#52396=CARTESIAN_POINT('Ctrl Pts',(-1.08304304871042,-1.,-3.88164007721365));
#52397=CARTESIAN_POINT('Ctrl Pts',(-1.08304304871042,1.,-3.88164007721365));
#52398=CARTESIAN_POINT('Ctrl Pts',(-1.0837621330751,-1.,-3.87402233722563));
#52399=CARTESIAN_POINT('Ctrl Pts',(-1.0837621330751,1.,-3.87402233722563));
#52400=CARTESIAN_POINT('Ctrl Pts',(-1.08443918607926,-1.,-3.86640769434269));
#52401=CARTESIAN_POINT('Ctrl Pts',(-1.08443918607926,1.,-3.86640769434269));
#52402=CARTESIAN_POINT('Ctrl Pts',(-1.08507395120054,-1.,-3.85879698702511));
#52403=CARTESIAN_POINT('Ctrl Pts',(-1.08507395120054,1.,-3.85879698702511));
#52404=CARTESIAN_POINT('Ctrl Pts',(-1.08566647671838,-1.,-3.85119211322732));
#52405=CARTESIAN_POINT('Ctrl Pts',(-1.08566647671838,1.,-3.85119211322732));
#52406=CARTESIAN_POINT('Ctrl Pts',(-1.08621688337601,-1.,-3.84359528764934));
#52407=CARTESIAN_POINT('Ctrl Pts',(-1.08621688337601,1.,-3.84359528764934));
#52408=CARTESIAN_POINT('Ctrl Pts',(-1.08672515456901,-1.,-3.83600837071702));
#52409=CARTESIAN_POINT('Ctrl Pts',(-1.08672515456901,1.,-3.83600837071702));
#52410=CARTESIAN_POINT('Ctrl Pts',(-1.08719091307558,-1.,-3.82843215316985));
#52411=CARTESIAN_POINT('Ctrl Pts',(-1.08719091307558,1.,-3.82843215316985));
#52412=CARTESIAN_POINT('Ctrl Pts',(-1.08761321539442,-1.,-3.82086569676321));
#52413=CARTESIAN_POINT('Ctrl Pts',(-1.08761321539442,1.,-3.82086569676321));
#52414=CARTESIAN_POINT('Ctrl Pts',(-1.08799030610861,-1.,-3.81330554446324));
#52415=CARTESIAN_POINT('Ctrl Pts',(-1.08799030610861,1.,-3.81330554446324));
#52416=CARTESIAN_POINT('Ctrl Pts',(-1.08832009255378,-1.,-3.80574726657656));
#52417=CARTESIAN_POINT('Ctrl Pts',(-1.08832009255378,1.,-3.80574726657656));
#52418=CARTESIAN_POINT('Ctrl Pts',(-1.08860064435776,-1.,-3.79818708705252));
#52419=CARTESIAN_POINT('Ctrl Pts',(-1.08860064435776,1.,-3.79818708705252));
#52420=CARTESIAN_POINT('Ctrl Pts',(-1.08883071512097,-1.,-3.79062357974401));
#52421=CARTESIAN_POINT('Ctrl Pts',(-1.08883071512097,1.,-3.79062357974401));
#52422=CARTESIAN_POINT('Ctrl Pts',(-1.08901018614638,-1.,-3.78305911299511));
#52423=CARTESIAN_POINT('Ctrl Pts',(-1.08901018614638,1.,-3.78305911299511));
#52424=CARTESIAN_POINT('Ctrl Pts',(-1.08914072791275,-1.,-3.7755019940944));
#52425=CARTESIAN_POINT('Ctrl Pts',(-1.08914072791275,1.,-3.7755019940944));
#52426=CARTESIAN_POINT('Ctrl Pts',(-1.08922484204263,-1.,-3.76796340094469));
#52427=CARTESIAN_POINT('Ctrl Pts',(-1.08922484204263,1.,-3.76796340094469));
#52428=CARTESIAN_POINT('Ctrl Pts',(-1.08926462734287,-1.,-3.76045342580226));
#52429=CARTESIAN_POINT('Ctrl Pts',(-1.08926462734287,1.,-3.76045342580226));
#52430=CARTESIAN_POINT('Ctrl Pts',(-1.08926054632927,-1.,-3.75297711748138));
#52431=CARTESIAN_POINT('Ctrl Pts',(-1.08926054632927,1.,-3.75297711748138));
#52432=CARTESIAN_POINT('Ctrl Pts',(-1.08921040494013,-1.,-3.74553121371745));
#52433=CARTESIAN_POINT('Ctrl Pts',(-1.08921040494013,1.,-3.74553121371745));
#52434=CARTESIAN_POINT('Ctrl Pts',(-1.08910769013288,-1.,-3.73809879348209));
#52435=CARTESIAN_POINT('Ctrl Pts',(-1.08910769013288,1.,-3.73809879348209));
#52436=CARTESIAN_POINT('Ctrl Pts',(-1.08894337390925,-1.,-3.73065515162949));
#52437=CARTESIAN_POINT('Ctrl Pts',(-1.08894337390925,1.,-3.73065515162949));
#52438=CARTESIAN_POINT('Ctrl Pts',(-1.08870887220072,-1.,-3.72317741369364));
#52439=CARTESIAN_POINT('Ctrl Pts',(-1.08870887220072,1.,-3.72317741369364));
#52440=CARTESIAN_POINT('Ctrl Pts',(-1.08839887334777,-1.,-3.71565372339063));
#52441=CARTESIAN_POINT('Ctrl Pts',(-1.08839887334777,1.,-3.71565372339063));
#52442=CARTESIAN_POINT('Ctrl Pts',(-1.0880136731219,-1.,-3.70809084139476));
#52443=CARTESIAN_POINT('Ctrl Pts',(-1.0880136731219,1.,-3.70809084139476));
#52444=CARTESIAN_POINT('Ctrl Pts',(-1.08756311291324,-1.,-3.70052690909884));
#52445=CARTESIAN_POINT('Ctrl Pts',(-1.08756311291324,1.,-3.70052690909884));
#52446=CARTESIAN_POINT('Ctrl Pts',(-1.08706319540292,-1.,-3.69302062410229));
#52447=CARTESIAN_POINT('Ctrl Pts',(-1.08706319540292,1.,-3.69302062410229));
#52448=CARTESIAN_POINT('Ctrl Pts',(-1.08652888882609,-1.,-3.68562817420864));
#52449=CARTESIAN_POINT('Ctrl Pts',(-1.08652888882609,1.,-3.68562817420864));
#52450=CARTESIAN_POINT('Ctrl Pts',(-1.08596755755768,-1.,-3.67838211685148));
#52451=CARTESIAN_POINT('Ctrl Pts',(-1.08596755755768,1.,-3.67838211685148));
#52452=CARTESIAN_POINT('Ctrl Pts',(-1.0853733414448,-1.,-3.67127347729632));
#52453=CARTESIAN_POINT('Ctrl Pts',(-1.0853733414448,1.,-3.67127347729632));
#52454=CARTESIAN_POINT('Ctrl Pts',(-1.0847180992287,-1.,-3.66422237895256));
#52455=CARTESIAN_POINT('Ctrl Pts',(-1.0847180992287,1.,-3.66422237895256));
#52456=CARTESIAN_POINT('Ctrl Pts',(-1.08395671077761,-1.,-3.65709649161004));
#52457=CARTESIAN_POINT('Ctrl Pts',(-1.08395671077761,1.,-3.65709649161004));
#52458=CARTESIAN_POINT('Ctrl Pts',(-1.08304289898577,-1.,-3.64976441208197));
#52459=CARTESIAN_POINT('Ctrl Pts',(-1.08304289898577,1.,-3.64976441208197));
#52460=CARTESIAN_POINT('Ctrl Pts',(-1.08194278850972,-1.,-3.64214167843595));
#52461=CARTESIAN_POINT('Ctrl Pts',(-1.08194278850972,1.,-3.64214167843595));
#52462=CARTESIAN_POINT('Ctrl Pts',(-1.08064765719887,-1.,-3.63423373196602));
#52463=CARTESIAN_POINT('Ctrl Pts',(-1.08064765719887,1.,-3.63423373196602));
#52464=CARTESIAN_POINT('Ctrl Pts',(-1.07919137290815,-1.,-3.62619537902616));
#52465=CARTESIAN_POINT('Ctrl Pts',(-1.07919137290815,1.,-3.62619537902616));
#52466=CARTESIAN_POINT('Ctrl Pts',(-1.07764868137729,-1.,-3.61832318504957));
#52467=CARTESIAN_POINT('Ctrl Pts',(-1.07764868137729,1.,-3.61832318504957));
#52468=CARTESIAN_POINT('Ctrl Pts',(-1.07611545402841,-1.,-3.61098481349577));
#52469=CARTESIAN_POINT('Ctrl Pts',(-1.07611545402841,1.,-3.61098481349577));
#52470=CARTESIAN_POINT('Ctrl Pts',(-1.0746932716863,-1.,-3.6045633988796));
#52471=CARTESIAN_POINT('Ctrl Pts',(-1.0746932716863,1.,-3.6045633988796));
#52472=CARTESIAN_POINT('Ctrl Pts',(-1.0734737254567,-1.,-3.59940121154383));
#52473=CARTESIAN_POINT('Ctrl Pts',(-1.0734737254567,1.,-3.59940121154383));
#52474=CARTESIAN_POINT('Ctrl Pts',(-1.07251922679108,-1.,-3.59573039611837));
#52475=CARTESIAN_POINT('Ctrl Pts',(-1.07251922679108,1.,-3.59573039611837));
#52476=CARTESIAN_POINT('Ctrl Pts',(-1.07199116987503,-1.,-3.59407399103556));
#52477=CARTESIAN_POINT('Ctrl Pts',(-1.07199116987503,1.,-3.59407399103556));
#52478=CARTESIAN_POINT('Ctrl Pts',(-1.07173216219041,-1.,-3.59356848057451));
#52479=CARTESIAN_POINT('Ctrl Pts',(-1.07173216219041,1.,-3.59356848057451));
#52480=CARTESIAN_POINT('Ctrl Pts',(-1.07162034256419,-1.,-3.59355870577763));
#52481=CARTESIAN_POINT('Ctrl Pts',(-1.07162034256419,1.,-3.59355870577763));
#52482=CARTESIAN_POINT('Ctrl Pts',(-1.07157964745328,-1.,-3.59363563249864));
#52483=CARTESIAN_POINT('Ctrl Pts',(-1.07157964745328,1.,-3.59363563249864));
#52484=CARTESIAN_POINT('',(-1.05427041296137,1.,-4.06552750530042));
#52485=CARTESIAN_POINT('Ctrl Pts',(-1.05427041296137,1.,-4.06552750530042));
#52486=CARTESIAN_POINT('Ctrl Pts',(-1.05459645194934,1.,-4.06398907542679));
#52487=CARTESIAN_POINT('Ctrl Pts',(-1.05524507177901,1.,-4.06091239150293));
#52488=CARTESIAN_POINT('Ctrl Pts',(-1.0562076270849,1.,-4.05629789308941));
#52489=CARTESIAN_POINT('Ctrl Pts',(-1.05747027728537,1.,-4.05014628387112));
#52490=CARTESIAN_POINT('Ctrl Pts',(-1.05901393667039,1.,-4.04245854429333));
#52491=CARTESIAN_POINT('Ctrl Pts',(-1.06052284712114,1.,-4.03477261142549));
#52492=CARTESIAN_POINT('Ctrl Pts',(-1.06199687787488,1.,-4.02708855235732));
#52493=CARTESIAN_POINT('Ctrl Pts',(-1.06343586496094,1.,-4.0194064749539));
#52494=CARTESIAN_POINT('Ctrl Pts',(-1.06483961342894,1.,-4.0117265418656));
#52495=CARTESIAN_POINT('Ctrl Pts',(-1.06620789963406,1.,-4.00404894951804));
#52496=CARTESIAN_POINT('Ctrl Pts',(-1.06754047381188,1.,-3.99637389919958));
#52497=CARTESIAN_POINT('Ctrl Pts',(-1.06883706263912,1.,-3.98870156857298));
#52498=CARTESIAN_POINT('Ctrl Pts',(-1.07009737257815,1.,-3.98103208801289));
#52499=CARTESIAN_POINT('Ctrl Pts',(-1.07132109206252,1.,-3.97336550222571));
#52500=CARTESIAN_POINT('Ctrl Pts',(-1.07250789943095,1.,-3.96570179322681));
#52501=CARTESIAN_POINT('Ctrl Pts',(-1.07365747426551,1.,-3.95804094429606));
#52502=CARTESIAN_POINT('Ctrl Pts',(-1.07476950921607,1.,-3.95038299600754));
#52503=CARTESIAN_POINT('Ctrl Pts',(-1.07584371946428,1.,-3.94272809633271));
#52504=CARTESIAN_POINT('Ctrl Pts',(-1.07687985975348,1.,-3.93507657572743));
#52505=CARTESIAN_POINT('Ctrl Pts',(-1.07787771707155,1.,-3.92742893349684));
#52506=CARTESIAN_POINT('Ctrl Pts',(-1.07883706663524,1.,-3.91978568924062));
#52507=CARTESIAN_POINT('Ctrl Pts',(-1.0797576350746,1.,-3.91214726022096));
#52508=CARTESIAN_POINT('Ctrl Pts',(-1.08063906483822,1.,-3.90451384092564));
#52509=CARTESIAN_POINT('Ctrl Pts',(-1.08148086931373,1.,-3.89688525098408));
#52510=CARTESIAN_POINT('Ctrl Pts',(-1.08228241999363,1.,-3.88926088975182));
#52511=CARTESIAN_POINT('Ctrl Pts',(-1.08304304871042,1.,-3.88164007721365));
#52512=CARTESIAN_POINT('Ctrl Pts',(-1.0837621330751,1.,-3.87402233722563));
#52513=CARTESIAN_POINT('Ctrl Pts',(-1.08443918607926,1.,-3.86640769434269));
#52514=CARTESIAN_POINT('Ctrl Pts',(-1.08507395120054,1.,-3.85879698702511));
#52515=CARTESIAN_POINT('Ctrl Pts',(-1.08566647671838,1.,-3.85119211322732));
#52516=CARTESIAN_POINT('Ctrl Pts',(-1.08621688337601,1.,-3.84359528764934));
#52517=CARTESIAN_POINT('Ctrl Pts',(-1.08672515456901,1.,-3.83600837071702));
#52518=CARTESIAN_POINT('Ctrl Pts',(-1.08719091307558,1.,-3.82843215316985));
#52519=CARTESIAN_POINT('Ctrl Pts',(-1.08761321539442,1.,-3.82086569676321));
#52520=CARTESIAN_POINT('Ctrl Pts',(-1.08799030610861,1.,-3.81330554446324));
#52521=CARTESIAN_POINT('Ctrl Pts',(-1.08832009255378,1.,-3.80574726657656));
#52522=CARTESIAN_POINT('Ctrl Pts',(-1.08860064435776,1.,-3.79818708705252));
#52523=CARTESIAN_POINT('Ctrl Pts',(-1.08883071512097,1.,-3.79062357974401));
#52524=CARTESIAN_POINT('Ctrl Pts',(-1.08901018614638,1.,-3.78305911299511));
#52525=CARTESIAN_POINT('Ctrl Pts',(-1.08914072791275,1.,-3.7755019940944));
#52526=CARTESIAN_POINT('Ctrl Pts',(-1.08922484204263,1.,-3.76796340094469));
#52527=CARTESIAN_POINT('Ctrl Pts',(-1.08926462734287,1.,-3.76045342580226));
#52528=CARTESIAN_POINT('Ctrl Pts',(-1.08926054632927,1.,-3.75297711748138));
#52529=CARTESIAN_POINT('Ctrl Pts',(-1.08921040494013,1.,-3.74553121371745));
#52530=CARTESIAN_POINT('Ctrl Pts',(-1.08910769013288,1.,-3.73809879348209));
#52531=CARTESIAN_POINT('Ctrl Pts',(-1.08894337390925,1.,-3.73065515162949));
#52532=CARTESIAN_POINT('Ctrl Pts',(-1.08870887220072,1.,-3.72317741369364));
#52533=CARTESIAN_POINT('Ctrl Pts',(-1.08839887334777,1.,-3.71565372339063));
#52534=CARTESIAN_POINT('Ctrl Pts',(-1.0880136731219,1.,-3.70809084139476));
#52535=CARTESIAN_POINT('Ctrl Pts',(-1.08756311291324,1.,-3.70052690909884));
#52536=CARTESIAN_POINT('Ctrl Pts',(-1.08706319540292,1.,-3.69302062410229));
#52537=CARTESIAN_POINT('Ctrl Pts',(-1.08652888882609,1.,-3.68562817420864));
#52538=CARTESIAN_POINT('Ctrl Pts',(-1.08596755755768,1.,-3.67838211685148));
#52539=CARTESIAN_POINT('Ctrl Pts',(-1.0853733414448,1.,-3.67127347729632));
#52540=CARTESIAN_POINT('Ctrl Pts',(-1.0847180992287,1.,-3.66422237895256));
#52541=CARTESIAN_POINT('Ctrl Pts',(-1.08395671077761,1.,-3.65709649161004));
#52542=CARTESIAN_POINT('Ctrl Pts',(-1.08304289898577,1.,-3.64976441208197));
#52543=CARTESIAN_POINT('Ctrl Pts',(-1.08194278850972,1.,-3.64214167843595));
#52544=CARTESIAN_POINT('Ctrl Pts',(-1.08064765719887,1.,-3.63423373196602));
#52545=CARTESIAN_POINT('Ctrl Pts',(-1.07919137290815,1.,-3.62619537902616));
#52546=CARTESIAN_POINT('Ctrl Pts',(-1.07764868137729,1.,-3.61832318504957));
#52547=CARTESIAN_POINT('Ctrl Pts',(-1.07611545402841,1.,-3.61098481349577));
#52548=CARTESIAN_POINT('Ctrl Pts',(-1.0746932716863,1.,-3.6045633988796));
#52549=CARTESIAN_POINT('Ctrl Pts',(-1.0734737254567,1.,-3.59940121154383));
#52550=CARTESIAN_POINT('Ctrl Pts',(-1.07259084660947,1.,-3.59600583195037));
#52551=CARTESIAN_POINT('Ctrl Pts',(-1.07209229745284,1.,-3.59439597));
#52552=CARTESIAN_POINT('Ctrl Pts',(-1.07183575450716,1.,-3.59379266874663));
#52553=CARTESIAN_POINT('Ctrl Pts',(-1.07171709254271,1.,-3.59363512797985));
#52554=CARTESIAN_POINT('Ctrl Pts',(-1.071677399622,1.,-3.59360648251021));
#52555=CARTESIAN_POINT('',(-1.05427041296137,0.,-4.06552750530042));
#52556=CARTESIAN_POINT('Ctrl Pts',(-0.676691979611561,-1.,-3.68843977377012));
#52557=CARTESIAN_POINT('Ctrl Pts',(-0.676691979611561,1.,-3.68843977377012));
#52558=CARTESIAN_POINT('Ctrl Pts',(-0.676620796001989,-1.,-3.68838970675497));
#52559=CARTESIAN_POINT('Ctrl Pts',(-0.676620796001989,1.,-3.68838970675497));
#52560=CARTESIAN_POINT('Ctrl Pts',(-0.676525601650856,-1.,-3.68844918121303));
#52561=CARTESIAN_POINT('Ctrl Pts',(-0.676525601650856,1.,-3.68844918121303));
#52562=CARTESIAN_POINT('Ctrl Pts',(-0.676524321061226,-1.,-3.68901718136181));
#52563=CARTESIAN_POINT('Ctrl Pts',(-0.676524321061226,1.,-3.68901718136181));
#52564=CARTESIAN_POINT('Ctrl Pts',(-0.676805811075091,-1.,-3.69073278191994));
#52565=CARTESIAN_POINT('Ctrl Pts',(-0.676805811075091,1.,-3.69073278191994));
#52566=CARTESIAN_POINT('Ctrl Pts',(-0.677621861865498,-1.,-3.69443683573598));
#52567=CARTESIAN_POINT('Ctrl Pts',(-0.677621861865498,1.,-3.69443683573598));
#52568=CARTESIAN_POINT('Ctrl Pts',(-0.678878822226026,-1.,-3.69959004073005));
#52569=CARTESIAN_POINT('Ctrl Pts',(-0.678878822226026,1.,-3.69959004073005));
#52570=CARTESIAN_POINT('Ctrl Pts',(-0.680526909710877,-1.,-3.70595722031785));
#52571=CARTESIAN_POINT('Ctrl Pts',(-0.680526909710877,1.,-3.70595722031785));
#52572=CARTESIAN_POINT('Ctrl Pts',(-0.68249234510893,-1.,-3.71319182789943));
#52573=CARTESIAN_POINT('Ctrl Pts',(-0.68249234510893,1.,-3.71319182789943));
#52574=CARTESIAN_POINT('Ctrl Pts',(-0.684691698167848,-1.,-3.7209063713926));
#52575=CARTESIAN_POINT('Ctrl Pts',(-0.684691698167848,1.,-3.7209063713926));
#52576=CARTESIAN_POINT('Ctrl Pts',(-0.687043475232355,-1.,-3.72872973554051));
#52577=CARTESIAN_POINT('Ctrl Pts',(-0.687043475232355,1.,-3.72872973554051));
#52578=CARTESIAN_POINT('Ctrl Pts',(-0.689479637354814,-1.,-3.73636374475077));
#52579=CARTESIAN_POINT('Ctrl Pts',(-0.689479637354814,1.,-3.73636374475077));
#52580=CARTESIAN_POINT('Ctrl Pts',(-0.69196008040082,-1.,-3.74365508986712));
#52581=CARTESIAN_POINT('Ctrl Pts',(-0.69196008040082,1.,-3.74365508986712));
#52582=CARTESIAN_POINT('Ctrl Pts',(-0.694474562581493,-1.,-3.75060288243455));
#52583=CARTESIAN_POINT('Ctrl Pts',(-0.694474562581493,1.,-3.75060288243455));
#52584=CARTESIAN_POINT('Ctrl Pts',(-0.697031245659744,-1.,-3.75729775767023));
#52585=CARTESIAN_POINT('Ctrl Pts',(-0.697031245659744,1.,-3.75729775767023));
#52586=CARTESIAN_POINT('Ctrl Pts',(-0.699648552230917,-1.,-3.76387780603759));
#52587=CARTESIAN_POINT('Ctrl Pts',(-0.699648552230917,1.,-3.76387780603759));
#52588=CARTESIAN_POINT('Ctrl Pts',(-0.702346356621552,-1.,-3.77048141872872));
#52589=CARTESIAN_POINT('Ctrl Pts',(-0.702346356621552,1.,-3.77048141872872));
#52590=CARTESIAN_POINT('Ctrl Pts',(-0.705135847999817,-1.,-3.77719254217129));
#52591=CARTESIAN_POINT('Ctrl Pts',(-0.705135847999817,1.,-3.77719254217129));
#52592=CARTESIAN_POINT('Ctrl Pts',(-0.708015879375459,-1.,-3.78402183336605));
#52593=CARTESIAN_POINT('Ctrl Pts',(-0.708015879375459,1.,-3.78402183336605));
#52594=CARTESIAN_POINT('Ctrl Pts',(-0.710978231689017,-1.,-3.79093694007094));
#52595=CARTESIAN_POINT('Ctrl Pts',(-0.710978231689017,1.,-3.79093694007094));
#52596=CARTESIAN_POINT('Ctrl Pts',(-0.714010733006641,-1.,-3.79788100314975));
#52597=CARTESIAN_POINT('Ctrl Pts',(-0.714010733006641,1.,-3.79788100314975));
#52598=CARTESIAN_POINT('Ctrl Pts',(-0.717100993669114,-1.,-3.80479445759309));
#52599=CARTESIAN_POINT('Ctrl Pts',(-0.717100993669114,1.,-3.80479445759309));
#52600=CARTESIAN_POINT('Ctrl Pts',(-0.720240466589236,-1.,-3.81163885127344));
#52601=CARTESIAN_POINT('Ctrl Pts',(-0.720240466589236,1.,-3.81163885127344));
#52602=CARTESIAN_POINT('Ctrl Pts',(-0.723426346019423,-1.,-3.81840802610835));
#52603=CARTESIAN_POINT('Ctrl Pts',(-0.723426346019423,1.,-3.81840802610835));
#52604=CARTESIAN_POINT('Ctrl Pts',(-0.726659281876664,-1.,-3.82511495756713));
#52605=CARTESIAN_POINT('Ctrl Pts',(-0.726659281876664,1.,-3.82511495756713));
#52606=CARTESIAN_POINT('Ctrl Pts',(-0.729942010490168,-1.,-3.83178392403383));
#52607=CARTESIAN_POINT('Ctrl Pts',(-0.729942010490168,1.,-3.83178392403383));
#52608=CARTESIAN_POINT('Ctrl Pts',(-0.733277703756078,-1.,-3.83844103658009));
#52609=CARTESIAN_POINT('Ctrl Pts',(-0.733277703756078,1.,-3.83844103658009));
#52610=CARTESIAN_POINT('Ctrl Pts',(-0.736668240497117,-1.,-3.84510432881213));
#52611=CARTESIAN_POINT('Ctrl Pts',(-0.736668240497117,1.,-3.84510432881213));
#52612=CARTESIAN_POINT('Ctrl Pts',(-0.740113146827137,-1.,-3.85177770351215));
#52613=CARTESIAN_POINT('Ctrl Pts',(-0.740113146827137,1.,-3.85177770351215));
#52614=CARTESIAN_POINT('Ctrl Pts',(-0.743610542737012,-1.,-3.85845645217594));
#52615=CARTESIAN_POINT('Ctrl Pts',(-0.743610542737012,1.,-3.85845645217594));
#52616=CARTESIAN_POINT('Ctrl Pts',(-0.747157716488871,-1.,-3.86513062969889));
#52617=CARTESIAN_POINT('Ctrl Pts',(-0.747157716488871,1.,-3.86513062969889));
#52618=CARTESIAN_POINT('Ctrl Pts',(-0.750751822383028,-1.,-3.87178914078374));
#52619=CARTESIAN_POINT('Ctrl Pts',(-0.750751822383028,1.,-3.87178914078374));
#52620=CARTESIAN_POINT('Ctrl Pts',(-0.754390577396856,-1.,-3.87842382520065));
#52621=CARTESIAN_POINT('Ctrl Pts',(-0.754390577396856,1.,-3.87842382520065));
#52622=CARTESIAN_POINT('Ctrl Pts',(-0.758072800564801,-1.,-3.88503262662689));
#52623=CARTESIAN_POINT('Ctrl Pts',(-0.758072800564801,1.,-3.88503262662689));
#52624=CARTESIAN_POINT('Ctrl Pts',(-0.76179802879397,-1.,-3.89161738162245));
#52625=CARTESIAN_POINT('Ctrl Pts',(-0.76179802879397,1.,-3.89161738162245));
#52626=CARTESIAN_POINT('Ctrl Pts',(-0.765566256401295,-1.,-3.89818233104378));
#52627=CARTESIAN_POINT('Ctrl Pts',(-0.765566256401295,1.,-3.89818233104378));
#52628=CARTESIAN_POINT('Ctrl Pts',(-0.769377629847874,-1.,-3.90473237182633));
#52629=CARTESIAN_POINT('Ctrl Pts',(-0.769377629847874,1.,-3.90473237182633));
#52630=CARTESIAN_POINT('Ctrl Pts',(-0.773232154506321,-1.,-3.91127138115243));
#52631=CARTESIAN_POINT('Ctrl Pts',(-0.773232154506321,1.,-3.91127138115243));
#52632=CARTESIAN_POINT('Ctrl Pts',(-0.777129415664956,-1.,-3.9178006233448));
#52633=CARTESIAN_POINT('Ctrl Pts',(-0.777129415664956,1.,-3.9178006233448));
#52634=CARTESIAN_POINT('Ctrl Pts',(-0.781068718228451,-1.,-3.92431956510441));
#52635=CARTESIAN_POINT('Ctrl Pts',(-0.781068718228451,1.,-3.92431956510441));
#52636=CARTESIAN_POINT('Ctrl Pts',(-0.785049202786507,-1.,-3.93082655631789));
#52637=CARTESIAN_POINT('Ctrl Pts',(-0.785049202786507,1.,-3.93082655631789));
#52638=CARTESIAN_POINT('Ctrl Pts',(-0.789069971469333,-1.,-3.93731956885676));
#52639=CARTESIAN_POINT('Ctrl Pts',(-0.789069971469333,1.,-3.93731956885676));
#52640=CARTESIAN_POINT('Ctrl Pts',(-0.793130205640961,-1.,-3.94379688971283));
#52641=CARTESIAN_POINT('Ctrl Pts',(-0.793130205640961,1.,-3.94379688971283));
#52642=CARTESIAN_POINT('Ctrl Pts',(-0.797229296085316,-1.,-3.95025788827136));
#52643=CARTESIAN_POINT('Ctrl Pts',(-0.797229296085316,1.,-3.95025788827136));
#52644=CARTESIAN_POINT('Ctrl Pts',(-0.801366797727049,-1.,-3.95670276375108));
#52645=CARTESIAN_POINT('Ctrl Pts',(-0.801366797727049,1.,-3.95670276375108));
#52646=CARTESIAN_POINT('Ctrl Pts',(-0.805542372178361,-1.,-3.96313222295815));
#52647=CARTESIAN_POINT('Ctrl Pts',(-0.805542372178361,1.,-3.96313222295815));
#52648=CARTESIAN_POINT('Ctrl Pts',(-0.809755732818091,-1.,-3.96954717513232));
#52649=CARTESIAN_POINT('Ctrl Pts',(-0.809755732818091,1.,-3.96954717513232));
#52650=CARTESIAN_POINT('Ctrl Pts',(-0.814006592328844,-1.,-3.97594844078811));
#52651=CARTESIAN_POINT('Ctrl Pts',(-0.814006592328844,1.,-3.97594844078811));
#52652=CARTESIAN_POINT('Ctrl Pts',(-0.818294599022293,-1.,-3.98233640155404));
#52653=CARTESIAN_POINT('Ctrl Pts',(-0.818294599022293,1.,-3.98233640155404));
#52654=CARTESIAN_POINT('Ctrl Pts',(-0.822619346022119,-1.,-3.98871104646485));
#52655=CARTESIAN_POINT('Ctrl Pts',(-0.822619346022119,1.,-3.98871104646485));
#52656=CARTESIAN_POINT('Ctrl Pts',(-0.826980400320789,-1.,-3.99507212784431));
#52657=CARTESIAN_POINT('Ctrl Pts',(-0.826980400320789,1.,-3.99507212784431));
#52658=CARTESIAN_POINT('Ctrl Pts',(-0.831377325741622,-1.,-4.00141928477507));
#52659=CARTESIAN_POINT('Ctrl Pts',(-0.831377325741622,1.,-4.00141928477507));
#52660=CARTESIAN_POINT('Ctrl Pts',(-0.835809705809646,-1.,-4.00775216907856));
#52661=CARTESIAN_POINT('Ctrl Pts',(-0.835809705809646,1.,-4.00775216907856));
#52662=CARTESIAN_POINT('Ctrl Pts',(-0.840277171975855,-1.,-4.01407059766103));
#52663=CARTESIAN_POINT('Ctrl Pts',(-0.840277171975855,1.,-4.01407059766103));
#52664=CARTESIAN_POINT('Ctrl Pts',(-0.844779403287745,-1.,-4.02037456798441));
#52665=CARTESIAN_POINT('Ctrl Pts',(-0.844779403287745,1.,-4.02037456798441));
#52666=CARTESIAN_POINT('Ctrl Pts',(-0.849316107474245,-1.,-4.02666418343164));
#52667=CARTESIAN_POINT('Ctrl Pts',(-0.849316107474245,1.,-4.02666418343164));
#52668=CARTESIAN_POINT('Ctrl Pts',(-0.853887006631755,-1.,-4.03293960436756));
#52669=CARTESIAN_POINT('Ctrl Pts',(-0.853887006631755,1.,-4.03293960436756));
#52670=CARTESIAN_POINT('Ctrl Pts',(-0.858491822322827,-1.,-4.03920099284773));
#52671=CARTESIAN_POINT('Ctrl Pts',(-0.858491822322827,1.,-4.03920099284773));
#52672=CARTESIAN_POINT('Ctrl Pts',(-0.863130256643259,-1.,-4.04544845048584));
#52673=CARTESIAN_POINT('Ctrl Pts',(-0.863130256643259,1.,-4.04544845048584));
#52674=CARTESIAN_POINT('Ctrl Pts',(-0.867801988859917,-1.,-4.05168199437909));
#52675=CARTESIAN_POINT('Ctrl Pts',(-0.867801988859917,1.,-4.05168199437909));
#52676=CARTESIAN_POINT('Ctrl Pts',(-0.872506694782446,-1.,-4.0579015903134));
#52677=CARTESIAN_POINT('Ctrl Pts',(-0.872506694782446,1.,-4.0579015903134));
#52678=CARTESIAN_POINT('Ctrl Pts',(-0.877244060485837,-1.,-4.06410717232905));
#52679=CARTESIAN_POINT('Ctrl Pts',(-0.877244060485837,1.,-4.06410717232905));
#52680=CARTESIAN_POINT('Ctrl Pts',(-0.882013797525692,-1.,-4.07029866694192));
#52681=CARTESIAN_POINT('Ctrl Pts',(-0.882013797525692,1.,-4.07029866694192));
#52682=CARTESIAN_POINT('Ctrl Pts',(-0.886815658358501,-1.,-4.07647601773635));
#52683=CARTESIAN_POINT('Ctrl Pts',(-0.886815658358501,1.,-4.07647601773635));
#52684=CARTESIAN_POINT('Ctrl Pts',(-0.891649447916278,-1.,-4.08263920304799));
#52685=CARTESIAN_POINT('Ctrl Pts',(-0.891649447916278,1.,-4.08263920304799));
#52686=CARTESIAN_POINT('Ctrl Pts',(-0.896515019231333,-1.,-4.08878822246833));
#52687=CARTESIAN_POINT('Ctrl Pts',(-0.896515019231333,1.,-4.08878822246833));
#52688=CARTESIAN_POINT('Ctrl Pts',(-0.900432820941675,-1.,-4.09369611522387));
#52689=CARTESIAN_POINT('Ctrl Pts',(-0.900432820941675,1.,-4.09369611522387));
#52690=CARTESIAN_POINT('Ctrl Pts',(-0.903385402441587,-1.,-4.09737067245935));
#52691=CARTESIAN_POINT('Ctrl Pts',(-0.903385402441587,1.,-4.09737067245935));
#52692=CARTESIAN_POINT('Ctrl Pts',(-0.905360112215337,-1.,-4.09981755067523));
#52693=CARTESIAN_POINT('Ctrl Pts',(-0.905360112215337,1.,-4.09981755067523));
#52694=CARTESIAN_POINT('Ctrl Pts',(-0.906349047628866,-1.,-4.10104028313088));
#52695=CARTESIAN_POINT('Ctrl Pts',(-0.906349047628866,1.,-4.10104028313088));
#52696=CARTESIAN_POINT('',(-0.676591647975427,1.,-3.68845817949586));
#52697=CARTESIAN_POINT('Ctrl Pts',(-0.676591647975428,-1.,-3.68845817949586));
#52698=CARTESIAN_POINT('Ctrl Pts',(-0.676591647975428,-0.666666666666667,
-3.68845817949586));
#52699=CARTESIAN_POINT('Ctrl Pts',(-0.676591647975428,-0.333333333333333,
-3.68845817949586));
#52700=CARTESIAN_POINT('Ctrl Pts',(-0.676591647975428,0.333333333333333,
-3.68845817949586));
#52701=CARTESIAN_POINT('Ctrl Pts',(-0.676591647975429,0.666666666666667,
-3.68845817949586));
#52702=CARTESIAN_POINT('Ctrl Pts',(-0.676591647975429,1.,-3.68845817949586));
#52703=CARTESIAN_POINT('',(-0.906349047628866,1.,-4.10104028313088));
#52704=CARTESIAN_POINT('',(-0.906349047628866,0.,-4.10104028313088));
#52705=CARTESIAN_POINT('Ctrl Pts',(-0.676591647975428,1.,-3.68845817949586));
#52706=CARTESIAN_POINT('Ctrl Pts',(-0.676569286094606,1.,-3.68850172300477));
#52707=CARTESIAN_POINT('Ctrl Pts',(-0.676535079520807,1.,-3.68869596425969));
#52708=CARTESIAN_POINT('Ctrl Pts',(-0.676580391119396,1.,-3.68934997767243));
#52709=CARTESIAN_POINT('Ctrl Pts',(-0.676867042599402,1.,-3.69101071175464));
#52710=CARTESIAN_POINT('Ctrl Pts',(-0.677621861865498,1.,-3.69443683573598));
#52711=CARTESIAN_POINT('Ctrl Pts',(-0.678878822226026,1.,-3.69959004073005));
#52712=CARTESIAN_POINT('Ctrl Pts',(-0.680526909710877,1.,-3.70595722031785));
#52713=CARTESIAN_POINT('Ctrl Pts',(-0.68249234510893,1.,-3.71319182789943));
#52714=CARTESIAN_POINT('Ctrl Pts',(-0.684691698167848,1.,-3.7209063713926));
#52715=CARTESIAN_POINT('Ctrl Pts',(-0.687043475232355,1.,-3.72872973554051));
#52716=CARTESIAN_POINT('Ctrl Pts',(-0.689479637354814,1.,-3.73636374475077));
#52717=CARTESIAN_POINT('Ctrl Pts',(-0.69196008040082,1.,-3.74365508986712));
#52718=CARTESIAN_POINT('Ctrl Pts',(-0.694474562581493,1.,-3.75060288243455));
#52719=CARTESIAN_POINT('Ctrl Pts',(-0.697031245659744,1.,-3.75729775767023));
#52720=CARTESIAN_POINT('Ctrl Pts',(-0.699648552230917,1.,-3.76387780603759));
#52721=CARTESIAN_POINT('Ctrl Pts',(-0.702346356621552,1.,-3.77048141872872));
#52722=CARTESIAN_POINT('Ctrl Pts',(-0.705135847999817,1.,-3.77719254217129));
#52723=CARTESIAN_POINT('Ctrl Pts',(-0.708015879375459,1.,-3.78402183336605));
#52724=CARTESIAN_POINT('Ctrl Pts',(-0.710978231689017,1.,-3.79093694007094));
#52725=CARTESIAN_POINT('Ctrl Pts',(-0.714010733006641,1.,-3.79788100314975));
#52726=CARTESIAN_POINT('Ctrl Pts',(-0.717100993669114,1.,-3.80479445759309));
#52727=CARTESIAN_POINT('Ctrl Pts',(-0.720240466589236,1.,-3.81163885127344));
#52728=CARTESIAN_POINT('Ctrl Pts',(-0.723426346019423,1.,-3.81840802610835));
#52729=CARTESIAN_POINT('Ctrl Pts',(-0.726659281876664,1.,-3.82511495756713));
#52730=CARTESIAN_POINT('Ctrl Pts',(-0.729942010490168,1.,-3.83178392403383));
#52731=CARTESIAN_POINT('Ctrl Pts',(-0.733277703756078,1.,-3.83844103658009));
#52732=CARTESIAN_POINT('Ctrl Pts',(-0.736668240497117,1.,-3.84510432881213));
#52733=CARTESIAN_POINT('Ctrl Pts',(-0.740113146827137,1.,-3.85177770351215));
#52734=CARTESIAN_POINT('Ctrl Pts',(-0.743610542737012,1.,-3.85845645217594));
#52735=CARTESIAN_POINT('Ctrl Pts',(-0.747157716488871,1.,-3.86513062969889));
#52736=CARTESIAN_POINT('Ctrl Pts',(-0.750751822383028,1.,-3.87178914078374));
#52737=CARTESIAN_POINT('Ctrl Pts',(-0.754390577396856,1.,-3.87842382520065));
#52738=CARTESIAN_POINT('Ctrl Pts',(-0.758072800564801,1.,-3.88503262662689));
#52739=CARTESIAN_POINT('Ctrl Pts',(-0.76179802879397,1.,-3.89161738162245));
#52740=CARTESIAN_POINT('Ctrl Pts',(-0.765566256401295,1.,-3.89818233104378));
#52741=CARTESIAN_POINT('Ctrl Pts',(-0.769377629847874,1.,-3.90473237182633));
#52742=CARTESIAN_POINT('Ctrl Pts',(-0.773232154506321,1.,-3.91127138115243));
#52743=CARTESIAN_POINT('Ctrl Pts',(-0.777129415664956,1.,-3.9178006233448));
#52744=CARTESIAN_POINT('Ctrl Pts',(-0.781068718228451,1.,-3.92431956510441));
#52745=CARTESIAN_POINT('Ctrl Pts',(-0.785049202786507,1.,-3.93082655631789));
#52746=CARTESIAN_POINT('Ctrl Pts',(-0.789069971469333,1.,-3.93731956885676));
#52747=CARTESIAN_POINT('Ctrl Pts',(-0.793130205640961,1.,-3.94379688971283));
#52748=CARTESIAN_POINT('Ctrl Pts',(-0.797229296085316,1.,-3.95025788827136));
#52749=CARTESIAN_POINT('Ctrl Pts',(-0.801366797727049,1.,-3.95670276375108));
#52750=CARTESIAN_POINT('Ctrl Pts',(-0.805542372178361,1.,-3.96313222295815));
#52751=CARTESIAN_POINT('Ctrl Pts',(-0.809755732818091,1.,-3.96954717513232));
#52752=CARTESIAN_POINT('Ctrl Pts',(-0.814006592328844,1.,-3.97594844078811));
#52753=CARTESIAN_POINT('Ctrl Pts',(-0.818294599022293,1.,-3.98233640155404));
#52754=CARTESIAN_POINT('Ctrl Pts',(-0.822619346022119,1.,-3.98871104646485));
#52755=CARTESIAN_POINT('Ctrl Pts',(-0.826980400320789,1.,-3.99507212784431));
#52756=CARTESIAN_POINT('Ctrl Pts',(-0.831377325741622,1.,-4.00141928477507));
#52757=CARTESIAN_POINT('Ctrl Pts',(-0.835809705809646,1.,-4.00775216907856));
#52758=CARTESIAN_POINT('Ctrl Pts',(-0.840277171975855,1.,-4.01407059766103));
#52759=CARTESIAN_POINT('Ctrl Pts',(-0.844779403287745,1.,-4.02037456798441));
#52760=CARTESIAN_POINT('Ctrl Pts',(-0.849316107474245,1.,-4.02666418343164));
#52761=CARTESIAN_POINT('Ctrl Pts',(-0.853887006631755,1.,-4.03293960436756));
#52762=CARTESIAN_POINT('Ctrl Pts',(-0.858491822322827,1.,-4.03920099284773));
#52763=CARTESIAN_POINT('Ctrl Pts',(-0.863130256643259,1.,-4.04544845048584));
#52764=CARTESIAN_POINT('Ctrl Pts',(-0.867801988859917,1.,-4.05168199437909));
#52765=CARTESIAN_POINT('Ctrl Pts',(-0.872506694782446,1.,-4.0579015903134));
#52766=CARTESIAN_POINT('Ctrl Pts',(-0.877244060485837,1.,-4.06410717232905));
#52767=CARTESIAN_POINT('Ctrl Pts',(-0.882013797525692,1.,-4.07029866694192));
#52768=CARTESIAN_POINT('Ctrl Pts',(-0.886815658358501,1.,-4.07647601773635));
#52769=CARTESIAN_POINT('Ctrl Pts',(-0.891649447916278,1.,-4.08263920304799));
#52770=CARTESIAN_POINT('Ctrl Pts',(-0.896515019231333,1.,-4.08878822246833));
#52771=CARTESIAN_POINT('Ctrl Pts',(-0.900432820941675,1.,-4.09369611522387));
#52772=CARTESIAN_POINT('Ctrl Pts',(-0.903385402441587,1.,-4.09737067245935));
#52773=CARTESIAN_POINT('Ctrl Pts',(-0.905360112215337,1.,-4.09981755067523));
#52774=CARTESIAN_POINT('Ctrl Pts',(-0.906349047628866,1.,-4.10104028313088));
#52775=CARTESIAN_POINT('Origin',(-0.906349047628866,0.,-4.10104028313088));
#52776=CARTESIAN_POINT('',(-1.05427041296137,1.,-4.06552750530042));
#52777=CARTESIAN_POINT('Origin',(0.,0.,0.));
#52778=CARTESIAN_POINT('',(-0.496319364829374,1.,-3.71701050416802));
#52779=CARTESIAN_POINT('Origin',(0.,1.,0.));
#52780=CARTESIAN_POINT('Ctrl Pts',(-0.496319364829374,1.,-3.71701050416802));
#52781=CARTESIAN_POINT('Ctrl Pts',(-0.496319364829374,0.666666666666667,
-3.71701050416802));
#52782=CARTESIAN_POINT('Ctrl Pts',(-0.496319364829374,0.333333333333333,
-3.71701050416802));
#52783=CARTESIAN_POINT('Ctrl Pts',(-0.496319364829374,-0.333333333333333,
-3.71701050416802));
#52784=CARTESIAN_POINT('Ctrl Pts',(-0.496319364829374,-0.666666666666667,
-3.71701050416802));
#52785=CARTESIAN_POINT('Ctrl Pts',(-0.496319364829374,-1.,-3.71701050416802));
#52786=CARTESIAN_POINT('Ctrl Pts',(-0.405301974318349,-1.,-4.18039834341342));
#52787=CARTESIAN_POINT('Ctrl Pts',(-0.405301974318349,1.,-4.18039834341342));
#52788=CARTESIAN_POINT('Ctrl Pts',(-0.405864662679631,-1.,-4.17892985789908));
#52789=CARTESIAN_POINT('Ctrl Pts',(-0.405864662679631,1.,-4.17892985789908));
#52790=CARTESIAN_POINT('Ctrl Pts',(-0.406986596326602,-1.,-4.17599251955585));
#52791=CARTESIAN_POINT('Ctrl Pts',(-0.406986596326602,1.,-4.17599251955585));
#52792=CARTESIAN_POINT('Ctrl Pts',(-0.408659167570153,-1.,-4.17158541009947));
#52793=CARTESIAN_POINT('Ctrl Pts',(-0.408659167570153,1.,-4.17158541009947));
#52794=CARTESIAN_POINT('Ctrl Pts',(-0.410868596148614,-1.,-4.16570705940731));
#52795=CARTESIAN_POINT('Ctrl Pts',(-0.410868596148614,1.,-4.16570705940731));
#52796=CARTESIAN_POINT('Ctrl Pts',(-0.413595877953269,-1.,-4.1583554501909));
#52797=CARTESIAN_POINT('Ctrl Pts',(-0.413595877953269,1.,-4.1583554501909));
#52798=CARTESIAN_POINT('Ctrl Pts',(-0.416288556008986,-1.,-4.15100018950989));
#52799=CARTESIAN_POINT('Ctrl Pts',(-0.416288556008986,1.,-4.15100018950989));
#52800=CARTESIAN_POINT('Ctrl Pts',(-0.4189464906678,-1.,-4.14364132317223));
#52801=CARTESIAN_POINT('Ctrl Pts',(-0.4189464906678,1.,-4.14364132317223));
#52802=CARTESIAN_POINT('Ctrl Pts',(-0.421569503103971,-1.,-4.13627893206433));
#52803=CARTESIAN_POINT('Ctrl Pts',(-0.421569503103971,1.,-4.13627893206433));
#52804=CARTESIAN_POINT('Ctrl Pts',(-0.424157375323155,-1.,-4.1289131463371));
#52805=CARTESIAN_POINT('Ctrl Pts',(-0.424157375323155,1.,-4.1289131463371));
#52806=CARTESIAN_POINT('Ctrl Pts',(-0.426709855706243,-1.,-4.1215441250121));
#52807=CARTESIAN_POINT('Ctrl Pts',(-0.426709855706243,1.,-4.1215441250121));
#52808=CARTESIAN_POINT('Ctrl Pts',(-0.429226666075372,-1.,-4.1141720278277));
#52809=CARTESIAN_POINT('Ctrl Pts',(-0.429226666075372,1.,-4.1141720278277));
#52810=CARTESIAN_POINT('Ctrl Pts',(-0.431707508679772,-1.,-4.10679698750219));
#52811=CARTESIAN_POINT('Ctrl Pts',(-0.431707508679772,1.,-4.10679698750219));
#52812=CARTESIAN_POINT('Ctrl Pts',(-0.434152073200643,-1.,-4.09941908688567));
#52813=CARTESIAN_POINT('Ctrl Pts',(-0.434152073200643,1.,-4.09941908688567));
#52814=CARTESIAN_POINT('Ctrl Pts',(-0.436560044913814,-1.,-4.09203832139439));
#52815=CARTESIAN_POINT('Ctrl Pts',(-0.436560044913814,1.,-4.09203832139439));
#52816=CARTESIAN_POINT('Ctrl Pts',(-0.438931108931613,-1.,-4.08465462294625));
#52817=CARTESIAN_POINT('Ctrl Pts',(-0.438931108931613,1.,-4.08465462294625));
#52818=CARTESIAN_POINT('Ctrl Pts',(-0.441264951396587,-1.,-4.07726792490256));
#52819=CARTESIAN_POINT('Ctrl Pts',(-0.441264951396587,1.,-4.07726792490256));
#52820=CARTESIAN_POINT('Ctrl Pts',(-0.443561262395408,-1.,-4.0698782192577));
#52821=CARTESIAN_POINT('Ctrl Pts',(-0.443561262395408,1.,-4.0698782192577));
#52822=CARTESIAN_POINT('Ctrl Pts',(-0.445819737468478,-1.,-4.06248560760596));
#52823=CARTESIAN_POINT('Ctrl Pts',(-0.445819737468478,1.,-4.06248560760596));
#52824=CARTESIAN_POINT('Ctrl Pts',(-0.448040082683976,-1.,-4.05509037796815));
#52825=CARTESIAN_POINT('Ctrl Pts',(-0.448040082683976,1.,-4.05509037796815));
#52826=CARTESIAN_POINT('Ctrl Pts',(-0.450222009543774,-1.,-4.0476929901797));
#52827=CARTESIAN_POINT('Ctrl Pts',(-0.450222009543774,1.,-4.0476929901797));
#52828=CARTESIAN_POINT('Ctrl Pts',(-0.452365214748779,-1.,-4.0402939222793));
#52829=CARTESIAN_POINT('Ctrl Pts',(-0.452365214748779,1.,-4.0402939222793));
#52830=CARTESIAN_POINT('Ctrl Pts',(-0.454469363020495,-1.,-4.03289354362745));
#52831=CARTESIAN_POINT('Ctrl Pts',(-0.454469363020495,1.,-4.03289354362745));
#52832=CARTESIAN_POINT('Ctrl Pts',(-0.456534070784968,-1.,-4.02549199038414));
#52833=CARTESIAN_POINT('Ctrl Pts',(-0.456534070784968,1.,-4.02549199038414));
#52834=CARTESIAN_POINT('Ctrl Pts',(-0.458558885637001,-1.,-4.01808900827647));
#52835=CARTESIAN_POINT('Ctrl Pts',(-0.458558885637001,1.,-4.01808900827647));
#52836=CARTESIAN_POINT('Ctrl Pts',(-0.460543280768577,-1.,-4.01068390573469));
#52837=CARTESIAN_POINT('Ctrl Pts',(-0.460543280768577,1.,-4.01068390573469));
#52838=CARTESIAN_POINT('Ctrl Pts',(-0.462486702616252,-1.,-4.00327590659129));
#52839=CARTESIAN_POINT('Ctrl Pts',(-0.462486702616252,1.,-4.00327590659129));
#52840=CARTESIAN_POINT('Ctrl Pts',(-0.464388610938995,-1.,-3.99586444320134));
#52841=CARTESIAN_POINT('Ctrl Pts',(-0.464388610938995,1.,-3.99586444320134));
#52842=CARTESIAN_POINT('Ctrl Pts',(-0.466248520883034,-1.,-3.98844946363258));
#52843=CARTESIAN_POINT('Ctrl Pts',(-0.466248520883034,1.,-3.98844946363258));
#52844=CARTESIAN_POINT('Ctrl Pts',(-0.46806604792014,-1.,-3.98103175589349));
#52845=CARTESIAN_POINT('Ctrl Pts',(-0.46806604792014,1.,-3.98103175589349));
#52846=CARTESIAN_POINT('Ctrl Pts',(-0.469840942829878,-1.,-3.97361320212413));
#52847=CARTESIAN_POINT('Ctrl Pts',(-0.469840942829878,1.,-3.97361320212413));
#52848=CARTESIAN_POINT('Ctrl Pts',(-0.471572978413493,-1.,-3.96619600864626));
#52849=CARTESIAN_POINT('Ctrl Pts',(-0.471572978413493,1.,-3.96619600864626));
#52850=CARTESIAN_POINT('Ctrl Pts',(-0.473261847236296,-1.,-3.95878201038332));
#52851=CARTESIAN_POINT('Ctrl Pts',(-0.473261847236296,1.,-3.95878201038332));
#52852=CARTESIAN_POINT('Ctrl Pts',(-0.47490705302179,-1.,-3.95137192932898));
#52853=CARTESIAN_POINT('Ctrl Pts',(-0.47490705302179,1.,-3.95137192932898));
#52854=CARTESIAN_POINT('Ctrl Pts',(-0.476507810658535,-1.,-3.94396469119385));
#52855=CARTESIAN_POINT('Ctrl Pts',(-0.476507810658535,1.,-3.94396469119385));
#52856=CARTESIAN_POINT('Ctrl Pts',(-0.478062927140957,-1.,-3.93655660689819));
#52857=CARTESIAN_POINT('Ctrl Pts',(-0.478062927140957,1.,-3.93655660689819));
#52858=CARTESIAN_POINT('Ctrl Pts',(-0.479571028525566,-1.,-3.92914297392067));
#52859=CARTESIAN_POINT('Ctrl Pts',(-0.479571028525566,1.,-3.92914297392067));
#52860=CARTESIAN_POINT('Ctrl Pts',(-0.481030798910735,-1.,-3.92171976072334));
#52861=CARTESIAN_POINT('Ctrl Pts',(-0.481030798910735,1.,-3.92171976072334));
#52862=CARTESIAN_POINT('Ctrl Pts',(-0.482441230340709,-1.,-3.91428536373749));
#52863=CARTESIAN_POINT('Ctrl Pts',(-0.482441230340709,1.,-3.91428536373749));
#52864=CARTESIAN_POINT('Ctrl Pts',(-0.483801835089161,-1.,-3.90684210358063));
#52865=CARTESIAN_POINT('Ctrl Pts',(-0.483801835089161,1.,-3.90684210358063));
#52866=CARTESIAN_POINT('Ctrl Pts',(-0.485112963522246,-1.,-3.89939844658529));
#52867=CARTESIAN_POINT('Ctrl Pts',(-0.485112963522246,1.,-3.89939844658529));
#52868=CARTESIAN_POINT('Ctrl Pts',(-0.486375337854133,-1.,-3.89196582437574));
#52869=CARTESIAN_POINT('Ctrl Pts',(-0.486375337854133,1.,-3.89196582437574));
#52870=CARTESIAN_POINT('Ctrl Pts',(-0.487589452275179,-1.,-3.88455453328156));
#52871=CARTESIAN_POINT('Ctrl Pts',(-0.487589452275179,1.,-3.88455453328156));
#52872=CARTESIAN_POINT('Ctrl Pts',(-0.488754973798281,-1.,-3.87716963231115));
#52873=CARTESIAN_POINT('Ctrl Pts',(-0.488754973798281,1.,-3.87716963231115));
#52874=CARTESIAN_POINT('Ctrl Pts',(-0.489870245704899,-1.,-3.86980755613694));
#52875=CARTESIAN_POINT('Ctrl Pts',(-0.489870245704899,1.,-3.86980755613694));
#52876=CARTESIAN_POINT('Ctrl Pts',(-0.490931482170849,-1.,-3.86245057319215));
#52877=CARTESIAN_POINT('Ctrl Pts',(-0.490931482170849,1.,-3.86245057319215));
#52878=CARTESIAN_POINT('Ctrl Pts',(-0.49193363108376,-1.,-3.85507287020223));
#52879=CARTESIAN_POINT('Ctrl Pts',(-0.49193363108376,1.,-3.85507287020223));
#52880=CARTESIAN_POINT('Ctrl Pts',(-0.492871792414095,-1.,-3.84765051147965));
#52881=CARTESIAN_POINT('Ctrl Pts',(-0.492871792414095,1.,-3.84765051147965));
#52882=CARTESIAN_POINT('Ctrl Pts',(-0.493742574629117,-1.,-3.84017095578438));
#52883=CARTESIAN_POINT('Ctrl Pts',(-0.493742574629117,1.,-3.84017095578438));
#52884=CARTESIAN_POINT('Ctrl Pts',(-0.494545212256425,-1.,-3.8326409268245));
#52885=CARTESIAN_POINT('Ctrl Pts',(-0.494545212256425,1.,-3.8326409268245));
#52886=CARTESIAN_POINT('Ctrl Pts',(-0.495283458893903,-1.,-3.82509963594156));
#52887=CARTESIAN_POINT('Ctrl Pts',(-0.495283458893903,1.,-3.82509963594156));
#52888=CARTESIAN_POINT('Ctrl Pts',(-0.495963937875572,-1.,-3.81760756144099));
#52889=CARTESIAN_POINT('Ctrl Pts',(-0.495963937875572,1.,-3.81760756144099));
#52890=CARTESIAN_POINT('Ctrl Pts',(-0.496592643443789,-1.,-3.81022254090909));
#52891=CARTESIAN_POINT('Ctrl Pts',(-0.496592643443789,1.,-3.81022254090909));
#52892=CARTESIAN_POINT('Ctrl Pts',(-0.497171756201091,-1.,-3.80297788298545));
#52893=CARTESIAN_POINT('Ctrl Pts',(-0.497171756201091,1.,-3.80297788298545));
#52894=CARTESIAN_POINT('Ctrl Pts',(-0.49769689210058,-1.,-3.79586380669959));
#52895=CARTESIAN_POINT('Ctrl Pts',(-0.49769689210058,1.,-3.79586380669959));
#52896=CARTESIAN_POINT('Ctrl Pts',(-0.498152751800819,-1.,-3.78879701661152));
#52897=CARTESIAN_POINT('Ctrl Pts',(-0.498152751800819,1.,-3.78879701661152));
#52898=CARTESIAN_POINT('Ctrl Pts',(-0.498515471679378,-1.,-3.78163975337189));
#52899=CARTESIAN_POINT('Ctrl Pts',(-0.498515471679378,1.,-3.78163975337189));
#52900=CARTESIAN_POINT('Ctrl Pts',(-0.498759900365687,-1.,-3.77425499225089));
#52901=CARTESIAN_POINT('Ctrl Pts',(-0.498759900365687,1.,-3.77425499225089));
#52902=CARTESIAN_POINT('Ctrl Pts',(-0.498865792335185,-1.,-3.76655401191144));
#52903=CARTESIAN_POINT('Ctrl Pts',(-0.498865792335185,1.,-3.76655401191144));
#52904=CARTESIAN_POINT('Ctrl Pts',(-0.498823681615513,-1.,-3.75854082221127));
#52905=CARTESIAN_POINT('Ctrl Pts',(-0.498823681615513,1.,-3.75854082221127));
#52906=CARTESIAN_POINT('Ctrl Pts',(-0.498642802042929,-1.,-3.75037362168103));
#52907=CARTESIAN_POINT('Ctrl Pts',(-0.498642802042929,1.,-3.75037362168103));
#52908=CARTESIAN_POINT('Ctrl Pts',(-0.498350586058176,-1.,-3.74235701735109));
#52909=CARTESIAN_POINT('Ctrl Pts',(-0.498350586058176,1.,-3.74235701735109));
#52910=CARTESIAN_POINT('Ctrl Pts',(-0.497984209510495,-1.,-3.73486914372834));
#52911=CARTESIAN_POINT('Ctrl Pts',(-0.497984209510495,1.,-3.73486914372834));
#52912=CARTESIAN_POINT('Ctrl Pts',(-0.497584067153279,-1.,-3.72830430904794));
#52913=CARTESIAN_POINT('Ctrl Pts',(-0.497584067153279,1.,-3.72830430904794));
#52914=CARTESIAN_POINT('Ctrl Pts',(-0.497187079575794,-1.,-3.72301489774241));
#52915=CARTESIAN_POINT('Ctrl Pts',(-0.497187079575794,1.,-3.72301489774241));
#52916=CARTESIAN_POINT('Ctrl Pts',(-0.496818574419989,-1.,-3.71923995965807));
#52917=CARTESIAN_POINT('Ctrl Pts',(-0.496818574419989,1.,-3.71923995965807));
#52918=CARTESIAN_POINT('Ctrl Pts',(-0.496556137603856,-1.,-3.71752134136931));
#52919=CARTESIAN_POINT('Ctrl Pts',(-0.496556137603856,1.,-3.71752134136931));
#52920=CARTESIAN_POINT('Ctrl Pts',(-0.496379397992182,-1.,-3.71698153685229));
#52921=CARTESIAN_POINT('Ctrl Pts',(-0.496379397992182,1.,-3.71698153685229));
#52922=CARTESIAN_POINT('Ctrl Pts',(-0.496270484166233,-1.,-3.71695438995598));
#52923=CARTESIAN_POINT('Ctrl Pts',(-0.496270484166233,1.,-3.71695438995598));
#52924=CARTESIAN_POINT('Ctrl Pts',(-0.496218256089212,-1.,-3.71702400346349));
#52925=CARTESIAN_POINT('Ctrl Pts',(-0.496218256089212,1.,-3.71702400346349));
#52926=CARTESIAN_POINT('',(-0.405301974318349,1.,-4.18039834341342));
#52927=CARTESIAN_POINT('Ctrl Pts',(-0.405301974318349,1.,-4.18039834341342));
#52928=CARTESIAN_POINT('Ctrl Pts',(-0.405864662679631,1.,-4.17892985789908));
#52929=CARTESIAN_POINT('Ctrl Pts',(-0.406986596326602,1.,-4.17599251955585));
#52930=CARTESIAN_POINT('Ctrl Pts',(-0.408659167570153,1.,-4.17158541009947));
#52931=CARTESIAN_POINT('Ctrl Pts',(-0.410868596148614,1.,-4.16570705940731));
#52932=CARTESIAN_POINT('Ctrl Pts',(-0.413595877953269,1.,-4.1583554501909));
#52933=CARTESIAN_POINT('Ctrl Pts',(-0.416288556008986,1.,-4.15100018950989));
#52934=CARTESIAN_POINT('Ctrl Pts',(-0.4189464906678,1.,-4.14364132317223));
#52935=CARTESIAN_POINT('Ctrl Pts',(-0.421569503103971,1.,-4.13627893206433));
#52936=CARTESIAN_POINT('Ctrl Pts',(-0.424157375323155,1.,-4.1289131463371));
#52937=CARTESIAN_POINT('Ctrl Pts',(-0.426709855706243,1.,-4.1215441250121));
#52938=CARTESIAN_POINT('Ctrl Pts',(-0.429226666075372,1.,-4.1141720278277));
#52939=CARTESIAN_POINT('Ctrl Pts',(-0.431707508679772,1.,-4.10679698750219));
#52940=CARTESIAN_POINT('Ctrl Pts',(-0.434152073200643,1.,-4.09941908688567));
#52941=CARTESIAN_POINT('Ctrl Pts',(-0.436560044913814,1.,-4.09203832139439));
#52942=CARTESIAN_POINT('Ctrl Pts',(-0.438931108931613,1.,-4.08465462294625));
#52943=CARTESIAN_POINT('Ctrl Pts',(-0.441264951396587,1.,-4.07726792490256));
#52944=CARTESIAN_POINT('Ctrl Pts',(-0.443561262395408,1.,-4.0698782192577));
#52945=CARTESIAN_POINT('Ctrl Pts',(-0.445819737468478,1.,-4.06248560760596));
#52946=CARTESIAN_POINT('Ctrl Pts',(-0.448040082683976,1.,-4.05509037796815));
#52947=CARTESIAN_POINT('Ctrl Pts',(-0.450222009543774,1.,-4.0476929901797));
#52948=CARTESIAN_POINT('Ctrl Pts',(-0.452365214748779,1.,-4.0402939222793));
#52949=CARTESIAN_POINT('Ctrl Pts',(-0.454469363020495,1.,-4.03289354362745));
#52950=CARTESIAN_POINT('Ctrl Pts',(-0.456534070784968,1.,-4.02549199038414));
#52951=CARTESIAN_POINT('Ctrl Pts',(-0.458558885637001,1.,-4.01808900827647));
#52952=CARTESIAN_POINT('Ctrl Pts',(-0.460543280768577,1.,-4.01068390573469));
#52953=CARTESIAN_POINT('Ctrl Pts',(-0.462486702616252,1.,-4.00327590659129));
#52954=CARTESIAN_POINT('Ctrl Pts',(-0.464388610938995,1.,-3.99586444320134));
#52955=CARTESIAN_POINT('Ctrl Pts',(-0.466248520883034,1.,-3.98844946363258));
#52956=CARTESIAN_POINT('Ctrl Pts',(-0.46806604792014,1.,-3.98103175589349));
#52957=CARTESIAN_POINT('Ctrl Pts',(-0.469840942829878,1.,-3.97361320212413));
#52958=CARTESIAN_POINT('Ctrl Pts',(-0.471572978413493,1.,-3.96619600864626));
#52959=CARTESIAN_POINT('Ctrl Pts',(-0.473261847236296,1.,-3.95878201038332));
#52960=CARTESIAN_POINT('Ctrl Pts',(-0.47490705302179,1.,-3.95137192932898));
#52961=CARTESIAN_POINT('Ctrl Pts',(-0.476507810658535,1.,-3.94396469119385));
#52962=CARTESIAN_POINT('Ctrl Pts',(-0.478062927140957,1.,-3.93655660689819));
#52963=CARTESIAN_POINT('Ctrl Pts',(-0.479571028525566,1.,-3.92914297392067));
#52964=CARTESIAN_POINT('Ctrl Pts',(-0.481030798910735,1.,-3.92171976072334));
#52965=CARTESIAN_POINT('Ctrl Pts',(-0.482441230340709,1.,-3.91428536373749));
#52966=CARTESIAN_POINT('Ctrl Pts',(-0.483801835089161,1.,-3.90684210358063));
#52967=CARTESIAN_POINT('Ctrl Pts',(-0.485112963522246,1.,-3.89939844658529));
#52968=CARTESIAN_POINT('Ctrl Pts',(-0.486375337854133,1.,-3.89196582437574));
#52969=CARTESIAN_POINT('Ctrl Pts',(-0.487589452275179,1.,-3.88455453328156));
#52970=CARTESIAN_POINT('Ctrl Pts',(-0.488754973798281,1.,-3.87716963231115));
#52971=CARTESIAN_POINT('Ctrl Pts',(-0.489870245704899,1.,-3.86980755613694));
#52972=CARTESIAN_POINT('Ctrl Pts',(-0.490931482170849,1.,-3.86245057319215));
#52973=CARTESIAN_POINT('Ctrl Pts',(-0.49193363108376,1.,-3.85507287020223));
#52974=CARTESIAN_POINT('Ctrl Pts',(-0.492871792414095,1.,-3.84765051147965));
#52975=CARTESIAN_POINT('Ctrl Pts',(-0.493742574629117,1.,-3.84017095578438));
#52976=CARTESIAN_POINT('Ctrl Pts',(-0.494545212256425,1.,-3.8326409268245));
#52977=CARTESIAN_POINT('Ctrl Pts',(-0.495283458893903,1.,-3.82509963594156));
#52978=CARTESIAN_POINT('Ctrl Pts',(-0.495963937875572,1.,-3.81760756144099));
#52979=CARTESIAN_POINT('Ctrl Pts',(-0.496592643443789,1.,-3.81022254090909));
#52980=CARTESIAN_POINT('Ctrl Pts',(-0.497171756201091,1.,-3.80297788298545));
#52981=CARTESIAN_POINT('Ctrl Pts',(-0.49769689210058,1.,-3.79586380669959));
#52982=CARTESIAN_POINT('Ctrl Pts',(-0.498152751800819,1.,-3.78879701661152));
#52983=CARTESIAN_POINT('Ctrl Pts',(-0.498515471679378,1.,-3.78163975337189));
#52984=CARTESIAN_POINT('Ctrl Pts',(-0.498759900365687,1.,-3.77425499225089));
#52985=CARTESIAN_POINT('Ctrl Pts',(-0.498865792335185,1.,-3.76655401191144));
#52986=CARTESIAN_POINT('Ctrl Pts',(-0.498823681615513,1.,-3.75854082221127));
#52987=CARTESIAN_POINT('Ctrl Pts',(-0.498642802042929,1.,-3.75037362168103));
#52988=CARTESIAN_POINT('Ctrl Pts',(-0.498350586058176,1.,-3.74235701735109));
#52989=CARTESIAN_POINT('Ctrl Pts',(-0.497984209510495,1.,-3.73486914372834));
#52990=CARTESIAN_POINT('Ctrl Pts',(-0.497584067153279,1.,-3.72830430904794));
#52991=CARTESIAN_POINT('Ctrl Pts',(-0.497187079575794,1.,-3.72301489774241));
#52992=CARTESIAN_POINT('Ctrl Pts',(-0.496846224822535,1.,-3.7195232082259));
#52993=CARTESIAN_POINT('Ctrl Pts',(-0.496605651526314,1.,-3.71785517607694));
#52994=CARTESIAN_POINT('Ctrl Pts',(-0.496446644158827,1.,-3.71721917030465));
#52995=CARTESIAN_POINT('Ctrl Pts',(-0.496354087925646,1.,-3.71704500630521));
#52996=CARTESIAN_POINT('Ctrl Pts',(-0.496319364829374,1.,-3.71701050416802));
#52997=CARTESIAN_POINT('',(-0.405301974318349,0.,-4.18039834341342));
#52998=CARTESIAN_POINT('Ctrl Pts',(-0.0913616755937422,-1.,-3.74888690736767));
#52999=CARTESIAN_POINT('Ctrl Pts',(-0.0913616755937422,1.,-3.74888690736767));
#53000=CARTESIAN_POINT('Ctrl Pts',(-0.0912992005792586,-1.,-3.74882632119067));
#53001=CARTESIAN_POINT('Ctrl Pts',(-0.0912992005792586,1.,-3.74882632119067));
#53002=CARTESIAN_POINT('Ctrl Pts',(-0.0911958743735236,-1.,-3.74887017174206));
#53003=CARTESIAN_POINT('Ctrl Pts',(-0.0911958743735236,1.,-3.74887017174206));
#53004=CARTESIAN_POINT('Ctrl Pts',(-0.0911057547506601,-1.,-3.74943097853811));
#53005=CARTESIAN_POINT('Ctrl Pts',(-0.0911057547506601,1.,-3.74943097853811));
#53006=CARTESIAN_POINT('Ctrl Pts',(-0.0911154000998143,-1.,-3.75116949194623));
#53007=CARTESIAN_POINT('Ctrl Pts',(-0.0911154000998143,1.,-3.75116949194623));
#53008=CARTESIAN_POINT('Ctrl Pts',(-0.09134196227364,-1.,-3.75495560118212));
#53009=CARTESIAN_POINT('Ctrl Pts',(-0.09134196227364,1.,-3.75495560118212));
#53010=CARTESIAN_POINT('Ctrl Pts',(-0.0917773084998337,-1.,-3.76024199359303));
#53011=CARTESIAN_POINT('Ctrl Pts',(-0.0917773084998337,1.,-3.76024199359303));
#53012=CARTESIAN_POINT('Ctrl Pts',(-0.0924090589602692,-1.,-3.76678860031841));
#53013=CARTESIAN_POINT('Ctrl Pts',(-0.0924090589602692,1.,-3.76678860031841));
#53014=CARTESIAN_POINT('Ctrl Pts',(-0.093218554620318,-1.,-3.77424159971059));
#53015=CARTESIAN_POINT('Ctrl Pts',(-0.093218554620318,1.,-3.77424159971059));
#53016=CARTESIAN_POINT('Ctrl Pts',(-0.0941840095090815,-1.,-3.782205218991));
#53017=CARTESIAN_POINT('Ctrl Pts',(-0.0941840095090815,1.,-3.782205218991));
#53018=CARTESIAN_POINT('Ctrl Pts',(-0.0952829885100802,-1.,-3.79030016353111));
#53019=CARTESIAN_POINT('Ctrl Pts',(-0.0952829885100802,1.,-3.79030016353111));
#53020=CARTESIAN_POINT('Ctrl Pts',(-0.0964949352873133,-1.,-3.79822128513845));
#53021=CARTESIAN_POINT('Ctrl Pts',(-0.0964949352873133,1.,-3.79822128513845));
#53022=CARTESIAN_POINT('Ctrl Pts',(-0.0978042222906645,-1.,-3.80581088847809));
#53023=CARTESIAN_POINT('Ctrl Pts',(-0.0978042222906645,1.,-3.80581088847809));
#53024=CARTESIAN_POINT('Ctrl Pts',(-0.0992008728096516,-1.,-3.81306649386461));
#53025=CARTESIAN_POINT('Ctrl Pts',(-0.0992008728096516,1.,-3.81306649386461));
#53026=CARTESIAN_POINT('Ctrl Pts',(-0.100678769650632,-1.,-3.82007889742625));
#53027=CARTESIAN_POINT('Ctrl Pts',(-0.100678769650632,1.,-3.82007889742625));
#53028=CARTESIAN_POINT('Ctrl Pts',(-0.102234506488456,-1.,-3.82698737143255));
#53029=CARTESIAN_POINT('Ctrl Pts',(-0.102234506488456,1.,-3.82698737143255));
#53030=CARTESIAN_POINT('Ctrl Pts',(-0.103866063811623,-1.,-3.83393171228002));
#53031=CARTESIAN_POINT('Ctrl Pts',(-0.103866063811623,1.,-3.83393171228002));
#53032=CARTESIAN_POINT('Ctrl Pts',(-0.105571360916569,-1.,-3.84099658324803));
#53033=CARTESIAN_POINT('Ctrl Pts',(-0.105571360916569,1.,-3.84099658324803));
#53034=CARTESIAN_POINT('Ctrl Pts',(-0.107347597812184,-1.,-3.84819233070317));
#53035=CARTESIAN_POINT('Ctrl Pts',(-0.107347597812184,1.,-3.84819233070317));
#53036=CARTESIAN_POINT('Ctrl Pts',(-0.109191717634944,-1.,-3.855485714969));
#53037=CARTESIAN_POINT('Ctrl Pts',(-0.109191717634944,1.,-3.855485714969));
#53038=CARTESIAN_POINT('Ctrl Pts',(-0.11110059303626,-1.,-3.86281867282965));
#53039=CARTESIAN_POINT('Ctrl Pts',(-0.11110059303626,1.,-3.86281867282965));
#53040=CARTESIAN_POINT('Ctrl Pts',(-0.113071304914562,-1.,-3.87013043445014));
#53041=CARTESIAN_POINT('Ctrl Pts',(-0.113071304914562,1.,-3.87013043445014));
#53042=CARTESIAN_POINT('Ctrl Pts',(-0.11510142664947,-1.,-3.87738168405343));
#53043=CARTESIAN_POINT('Ctrl Pts',(-0.11510142664947,1.,-3.87738168405343));
#53044=CARTESIAN_POINT('Ctrl Pts',(-0.117189150373144,-1.,-3.88456590045767));
#53045=CARTESIAN_POINT('Ctrl Pts',(-0.117189150373144,1.,-3.88456590045767));
#53046=CARTESIAN_POINT('Ctrl Pts',(-0.119333088190417,-1.,-3.89169600105201));
#53047=CARTESIAN_POINT('Ctrl Pts',(-0.119333088190417,1.,-3.89169600105201));
#53048=CARTESIAN_POINT('Ctrl Pts',(-0.121532144765723,-1.,-3.89879639336952));
#53049=CARTESIAN_POINT('Ctrl Pts',(-0.121532144765723,1.,-3.89879639336952));
#53050=CARTESIAN_POINT('Ctrl Pts',(-0.123785368272377,-1.,-3.90589336320508));
#53051=CARTESIAN_POINT('Ctrl Pts',(-0.123785368272377,1.,-3.90589336320508));
#53052=CARTESIAN_POINT('Ctrl Pts',(-0.126091793324137,-1.,-3.91300501605392));
#53053=CARTESIAN_POINT('Ctrl Pts',(-0.126091793324137,1.,-3.91300501605392));
#53054=CARTESIAN_POINT('Ctrl Pts',(-0.128450341339528,-1.,-3.92013513251642));
#53055=CARTESIAN_POINT('Ctrl Pts',(-0.128450341339528,1.,-3.92013513251642));
#53056=CARTESIAN_POINT('Ctrl Pts',(-0.130859892027799,-1.,-3.9272787679596));
#53057=CARTESIAN_POINT('Ctrl Pts',(-0.130859892027799,1.,-3.9272787679596));
#53058=CARTESIAN_POINT('Ctrl Pts',(-0.13331932279419,-1.,-3.93442567551035));
#53059=CARTESIAN_POINT('Ctrl Pts',(-0.13331932279419,1.,-3.93442567551035));
#53060=CARTESIAN_POINT('Ctrl Pts',(-0.135827558661188,-1.,-3.94156445130744));
#53061=CARTESIAN_POINT('Ctrl Pts',(-0.135827558661188,1.,-3.94156445130744));
#53062=CARTESIAN_POINT('Ctrl Pts',(-0.138383621255159,-1.,-3.94868667844355));
#53063=CARTESIAN_POINT('Ctrl Pts',(-0.138383621255159,1.,-3.94868667844355));
#53064=CARTESIAN_POINT('Ctrl Pts',(-0.140986665829937,-1.,-3.95579014116899));
#53065=CARTESIAN_POINT('Ctrl Pts',(-0.140986665829937,1.,-3.95579014116899));
#53066=CARTESIAN_POINT('Ctrl Pts',(-0.143635947692791,-1.,-3.96287658098896));
#53067=CARTESIAN_POINT('Ctrl Pts',(-0.143635947692791,1.,-3.96287658098896));
#53068=CARTESIAN_POINT('Ctrl Pts',(-0.146330797814513,-1.,-3.96995018565891));
#53069=CARTESIAN_POINT('Ctrl Pts',(-0.146330797814513,1.,-3.96995018565891));
#53070=CARTESIAN_POINT('Ctrl Pts',(-0.149070594803544,-1.,-3.97701581473643));
#53071=CARTESIAN_POINT('Ctrl Pts',(-0.149070594803544,1.,-3.97701581473643));
#53072=CARTESIAN_POINT('Ctrl Pts',(-0.151854737441405,-1.,-3.9840772985098));
#53073=CARTESIAN_POINT('Ctrl Pts',(-0.151854737441405,1.,-3.9840772985098));
#53074=CARTESIAN_POINT('Ctrl Pts',(-0.154682618338563,-1.,-3.99113582086059));
#53075=CARTESIAN_POINT('Ctrl Pts',(-0.154682618338563,1.,-3.99113582086059));
#53076=CARTESIAN_POINT('Ctrl Pts',(-0.15755363438381,-1.,-3.99819074631874));
#53077=CARTESIAN_POINT('Ctrl Pts',(-0.15755363438381,1.,-3.99819074631874));
#53078=CARTESIAN_POINT('Ctrl Pts',(-0.160467194882219,-1.,-4.00524031064509));
#53079=CARTESIAN_POINT('Ctrl Pts',(-0.160467194882219,1.,-4.00524031064509));
#53080=CARTESIAN_POINT('Ctrl Pts',(-0.163422730287459,-1.,-4.01228237022301));
#53081=CARTESIAN_POINT('Ctrl Pts',(-0.163422730287459,1.,-4.01228237022301));
#53082=CARTESIAN_POINT('Ctrl Pts',(-0.166419700015847,-1.,-4.01931510507143));
#53083=CARTESIAN_POINT('Ctrl Pts',(-0.166419700015847,1.,-4.01931510507143));
#53084=CARTESIAN_POINT('Ctrl Pts',(-0.169457601001653,-1.,-4.0263377970371));
#53085=CARTESIAN_POINT('Ctrl Pts',(-0.169457601001653,1.,-4.0263377970371));
#53086=CARTESIAN_POINT('Ctrl Pts',(-0.172535962484466,-1.,-4.03335057326093));
#53087=CARTESIAN_POINT('Ctrl Pts',(-0.172535962484466,1.,-4.03335057326093));
#53088=CARTESIAN_POINT('Ctrl Pts',(-0.175654339673757,-1.,-4.04035407891161));
#53089=CARTESIAN_POINT('Ctrl Pts',(-0.175654339673757,1.,-4.04035407891161));
#53090=CARTESIAN_POINT('Ctrl Pts',(-0.178812307240716,-1.,-4.04734916719722));
#53091=CARTESIAN_POINT('Ctrl Pts',(-0.178812307240716,1.,-4.04734916719722));
#53092=CARTESIAN_POINT('Ctrl Pts',(-0.18200945304855,-1.,-4.05433660358402));
#53093=CARTESIAN_POINT('Ctrl Pts',(-0.18200945304855,1.,-4.05433660358402));
#53094=CARTESIAN_POINT('Ctrl Pts',(-0.185245370038948,-1.,-4.06131670998589));
#53095=CARTESIAN_POINT('Ctrl Pts',(-0.185245370038948,1.,-4.06131670998589));
#53096=CARTESIAN_POINT('Ctrl Pts',(-0.188519658060255,-1.,-4.06828941192308));
#53097=CARTESIAN_POINT('Ctrl Pts',(-0.188519658060255,1.,-4.06828941192308));
#53098=CARTESIAN_POINT('Ctrl Pts',(-0.191831928181081,-1.,-4.07525439703137));
#53099=CARTESIAN_POINT('Ctrl Pts',(-0.191831928181081,1.,-4.07525439703137));
#53100=CARTESIAN_POINT('Ctrl Pts',(-0.195181806054714,-1.,-4.08221124060385));
#53101=CARTESIAN_POINT('Ctrl Pts',(-0.195181806054714,1.,-4.08221124060385));
#53102=CARTESIAN_POINT('Ctrl Pts',(-0.198568934800811,-1.,-4.08915953359753));
#53103=CARTESIAN_POINT('Ctrl Pts',(-0.198568934800811,1.,-4.08915953359753));
#53104=CARTESIAN_POINT('Ctrl Pts',(-0.201992979049984,-1.,-4.09609903751912));
#53105=CARTESIAN_POINT('Ctrl Pts',(-0.201992979049984,1.,-4.09609903751912));
#53106=CARTESIAN_POINT('Ctrl Pts',(-0.205453622198233,-1.,-4.10302969965374));
#53107=CARTESIAN_POINT('Ctrl Pts',(-0.205453622198233,1.,-4.10302969965374));
#53108=CARTESIAN_POINT('Ctrl Pts',(-0.208950559400172,-1.,-4.10995157639026));
#53109=CARTESIAN_POINT('Ctrl Pts',(-0.208950559400172,1.,-4.10995157639026));
#53110=CARTESIAN_POINT('Ctrl Pts',(-0.212483491087068,-1.,-4.11686478264545));
#53111=CARTESIAN_POINT('Ctrl Pts',(-0.212483491087068,1.,-4.11686478264545));
#53112=CARTESIAN_POINT('Ctrl Pts',(-0.216052116898425,-1.,-4.12376943492249));
#53113=CARTESIAN_POINT('Ctrl Pts',(-0.216052116898425,1.,-4.12376943492249));
#53114=CARTESIAN_POINT('Ctrl Pts',(-0.219656126701852,-1.,-4.13066558698156));
#53115=CARTESIAN_POINT('Ctrl Pts',(-0.219656126701852,1.,-4.13066558698156));
#53116=CARTESIAN_POINT('Ctrl Pts',(-0.223295201038383,-1.,-4.13755320553563));
#53117=CARTESIAN_POINT('Ctrl Pts',(-0.223295201038383,1.,-4.13755320553563));
#53118=CARTESIAN_POINT('Ctrl Pts',(-0.226969025061243,-1.,-4.14443220607733));
#53119=CARTESIAN_POINT('Ctrl Pts',(-0.226969025061243,1.,-4.14443220607733));
#53120=CARTESIAN_POINT('Ctrl Pts',(-0.230677299028738,-1.,-4.15130247435029));
#53121=CARTESIAN_POINT('Ctrl Pts',(-0.230677299028738,1.,-4.15130247435029));
#53122=CARTESIAN_POINT('Ctrl Pts',(-0.234419749543143,-1.,-4.1581638926525));
#53123=CARTESIAN_POINT('Ctrl Pts',(-0.234419749543143,1.,-4.1581638926525));
#53124=CARTESIAN_POINT('Ctrl Pts',(-0.238196140933977,-1.,-4.1650163665385));
#53125=CARTESIAN_POINT('Ctrl Pts',(-0.238196140933977,1.,-4.1650163665385));
#53126=CARTESIAN_POINT('Ctrl Pts',(-0.242006283923912,-1.,-4.17185984409533));
#53127=CARTESIAN_POINT('Ctrl Pts',(-0.242006283923912,1.,-4.17185984409533));
#53128=CARTESIAN_POINT('Ctrl Pts',(-0.245850033418583,-1.,-4.17869430192868));
#53129=CARTESIAN_POINT('Ctrl Pts',(-0.245850033418583,1.,-4.17869430192868));
#53130=CARTESIAN_POINT('Ctrl Pts',(-0.248951836910964,-1.,-4.18415464959491));
#53131=CARTESIAN_POINT('Ctrl Pts',(-0.248951836910964,1.,-4.18415464959491));
#53132=CARTESIAN_POINT('Ctrl Pts',(-0.251293239837693,-1.,-4.18824585244066));
#53133=CARTESIAN_POINT('Ctrl Pts',(-0.251293239837693,1.,-4.18824585244066));
#53134=CARTESIAN_POINT('Ctrl Pts',(-0.252860861572565,-1.,-4.19097151819241));
#53135=CARTESIAN_POINT('Ctrl Pts',(-0.252860861572565,1.,-4.19097151819241));
#53136=CARTESIAN_POINT('Ctrl Pts',(-0.253646344052521,-1.,-4.1923339003649));
#53137=CARTESIAN_POINT('Ctrl Pts',(-0.253646344052521,1.,-4.1923339003649));
#53138=CARTESIAN_POINT('',(-0.091259699916681,1.,-3.74888939116255));
#53139=CARTESIAN_POINT('Ctrl Pts',(-0.0912596999166824,-1.,-3.74888939116255));
#53140=CARTESIAN_POINT('Ctrl Pts',(-0.0912596999166824,-0.666666666666667,
-3.74888939116255));
#53141=CARTESIAN_POINT('Ctrl Pts',(-0.0912596999166824,-0.333333333333333,
-3.74888939116255));
#53142=CARTESIAN_POINT('Ctrl Pts',(-0.0912596999166824,0.333333333333333,
-3.74888939116255));
#53143=CARTESIAN_POINT('Ctrl Pts',(-0.0912596999166821,0.666666666666667,
-3.74888939116255));
#53144=CARTESIAN_POINT('Ctrl Pts',(-0.0912596999166821,1.,-3.74888939116255));
#53145=CARTESIAN_POINT('',(-0.253646344052521,1.,-4.1923339003649));
#53146=CARTESIAN_POINT('',(-0.253646344052521,0.,-4.1923339003649));
#53147=CARTESIAN_POINT('Ctrl Pts',(-0.0912596999166819,1.,-3.74888939116255));
#53148=CARTESIAN_POINT('Ctrl Pts',(-0.0912308016421982,1.,-3.74892890040975));
#53149=CARTESIAN_POINT('Ctrl Pts',(-0.0911666301812818,1.,-3.74911539914543));
#53150=CARTESIAN_POINT('Ctrl Pts',(-0.0911090736805512,1.,-3.74976844886347));
#53151=CARTESIAN_POINT('Ctrl Pts',(-0.0911323999574429,1.,-3.75145357872422));
#53152=CARTESIAN_POINT('Ctrl Pts',(-0.09134196227364,1.,-3.75495560118212));
#53153=CARTESIAN_POINT('Ctrl Pts',(-0.0917773084998337,1.,-3.76024199359303));
#53154=CARTESIAN_POINT('Ctrl Pts',(-0.0924090589602692,1.,-3.76678860031841));
#53155=CARTESIAN_POINT('Ctrl Pts',(-0.093218554620318,1.,-3.77424159971059));
#53156=CARTESIAN_POINT('Ctrl Pts',(-0.0941840095090815,1.,-3.782205218991));
#53157=CARTESIAN_POINT('Ctrl Pts',(-0.0952829885100802,1.,-3.79030016353111));
#53158=CARTESIAN_POINT('Ctrl Pts',(-0.0964949352873133,1.,-3.79822128513845));
#53159=CARTESIAN_POINT('Ctrl Pts',(-0.0978042222906645,1.,-3.80581088847809));
#53160=CARTESIAN_POINT('Ctrl Pts',(-0.0992008728096516,1.,-3.81306649386461));
#53161=CARTESIAN_POINT('Ctrl Pts',(-0.100678769650632,1.,-3.82007889742625));
#53162=CARTESIAN_POINT('Ctrl Pts',(-0.102234506488456,1.,-3.82698737143255));
#53163=CARTESIAN_POINT('Ctrl Pts',(-0.103866063811623,1.,-3.83393171228002));
#53164=CARTESIAN_POINT('Ctrl Pts',(-0.105571360916569,1.,-3.84099658324803));
#53165=CARTESIAN_POINT('Ctrl Pts',(-0.107347597812184,1.,-3.84819233070317));
#53166=CARTESIAN_POINT('Ctrl Pts',(-0.109191717634944,1.,-3.855485714969));
#53167=CARTESIAN_POINT('Ctrl Pts',(-0.11110059303626,1.,-3.86281867282965));
#53168=CARTESIAN_POINT('Ctrl Pts',(-0.113071304914562,1.,-3.87013043445014));
#53169=CARTESIAN_POINT('Ctrl Pts',(-0.11510142664947,1.,-3.87738168405343));
#53170=CARTESIAN_POINT('Ctrl Pts',(-0.117189150373144,1.,-3.88456590045767));
#53171=CARTESIAN_POINT('Ctrl Pts',(-0.119333088190417,1.,-3.89169600105201));
#53172=CARTESIAN_POINT('Ctrl Pts',(-0.121532144765723,1.,-3.89879639336952));
#53173=CARTESIAN_POINT('Ctrl Pts',(-0.123785368272377,1.,-3.90589336320508));
#53174=CARTESIAN_POINT('Ctrl Pts',(-0.126091793324137,1.,-3.91300501605392));
#53175=CARTESIAN_POINT('Ctrl Pts',(-0.128450341339528,1.,-3.92013513251642));
#53176=CARTESIAN_POINT('Ctrl Pts',(-0.130859892027799,1.,-3.9272787679596));
#53177=CARTESIAN_POINT('Ctrl Pts',(-0.13331932279419,1.,-3.93442567551035));
#53178=CARTESIAN_POINT('Ctrl Pts',(-0.135827558661188,1.,-3.94156445130744));
#53179=CARTESIAN_POINT('Ctrl Pts',(-0.138383621255159,1.,-3.94868667844355));
#53180=CARTESIAN_POINT('Ctrl Pts',(-0.140986665829937,1.,-3.95579014116899));
#53181=CARTESIAN_POINT('Ctrl Pts',(-0.143635947692791,1.,-3.96287658098896));
#53182=CARTESIAN_POINT('Ctrl Pts',(-0.146330797814513,1.,-3.96995018565891));
#53183=CARTESIAN_POINT('Ctrl Pts',(-0.149070594803544,1.,-3.97701581473643));
#53184=CARTESIAN_POINT('Ctrl Pts',(-0.151854737441405,1.,-3.9840772985098));
#53185=CARTESIAN_POINT('Ctrl Pts',(-0.154682618338563,1.,-3.99113582086059));
#53186=CARTESIAN_POINT('Ctrl Pts',(-0.15755363438381,1.,-3.99819074631874));
#53187=CARTESIAN_POINT('Ctrl Pts',(-0.160467194882219,1.,-4.00524031064509));
#53188=CARTESIAN_POINT('Ctrl Pts',(-0.163422730287459,1.,-4.01228237022301));
#53189=CARTESIAN_POINT('Ctrl Pts',(-0.166419700015847,1.,-4.01931510507143));
#53190=CARTESIAN_POINT('Ctrl Pts',(-0.169457601001653,1.,-4.0263377970371));
#53191=CARTESIAN_POINT('Ctrl Pts',(-0.172535962484466,1.,-4.03335057326093));
#53192=CARTESIAN_POINT('Ctrl Pts',(-0.175654339673757,1.,-4.04035407891161));
#53193=CARTESIAN_POINT('Ctrl Pts',(-0.178812307240716,1.,-4.04734916719722));
#53194=CARTESIAN_POINT('Ctrl Pts',(-0.18200945304855,1.,-4.05433660358402));
#53195=CARTESIAN_POINT('Ctrl Pts',(-0.185245370038948,1.,-4.06131670998589));
#53196=CARTESIAN_POINT('Ctrl Pts',(-0.188519658060255,1.,-4.06828941192308));
#53197=CARTESIAN_POINT('Ctrl Pts',(-0.191831928181081,1.,-4.07525439703137));
#53198=CARTESIAN_POINT('Ctrl Pts',(-0.195181806054714,1.,-4.08221124060385));
#53199=CARTESIAN_POINT('Ctrl Pts',(-0.198568934800811,1.,-4.08915953359753));
#53200=CARTESIAN_POINT('Ctrl Pts',(-0.201992979049984,1.,-4.09609903751912));
#53201=CARTESIAN_POINT('Ctrl Pts',(-0.205453622198233,1.,-4.10302969965374));
#53202=CARTESIAN_POINT('Ctrl Pts',(-0.208950559400172,1.,-4.10995157639026));
#53203=CARTESIAN_POINT('Ctrl Pts',(-0.212483491087068,1.,-4.11686478264545));
#53204=CARTESIAN_POINT('Ctrl Pts',(-0.216052116898425,1.,-4.12376943492249));
#53205=CARTESIAN_POINT('Ctrl Pts',(-0.219656126701852,1.,-4.13066558698156));
#53206=CARTESIAN_POINT('Ctrl Pts',(-0.223295201038383,1.,-4.13755320553563));
#53207=CARTESIAN_POINT('Ctrl Pts',(-0.226969025061243,1.,-4.14443220607733));
#53208=CARTESIAN_POINT('Ctrl Pts',(-0.230677299028738,1.,-4.15130247435029));
#53209=CARTESIAN_POINT('Ctrl Pts',(-0.234419749543143,1.,-4.1581638926525));
#53210=CARTESIAN_POINT('Ctrl Pts',(-0.238196140933977,1.,-4.1650163665385));
#53211=CARTESIAN_POINT('Ctrl Pts',(-0.242006283923912,1.,-4.17185984409533));
#53212=CARTESIAN_POINT('Ctrl Pts',(-0.245850033418583,1.,-4.17869430192868));
#53213=CARTESIAN_POINT('Ctrl Pts',(-0.248951836910964,1.,-4.18415464959491));
#53214=CARTESIAN_POINT('Ctrl Pts',(-0.251293239837693,1.,-4.18824585244066));
#53215=CARTESIAN_POINT('Ctrl Pts',(-0.252860861572565,1.,-4.19097151819241));
#53216=CARTESIAN_POINT('Ctrl Pts',(-0.253646344052521,1.,-4.1923339003649));
#53217=CARTESIAN_POINT('Origin',(-0.253646344052521,0.,-4.1923339003649));
#53218=CARTESIAN_POINT('',(-0.405301974318349,1.,-4.18039834341342));
#53219=CARTESIAN_POINT('Origin',(0.,0.,0.));
#53220=CARTESIAN_POINT('',(0.0912596999148849,1.,-3.74888939116259));
#53221=CARTESIAN_POINT('Origin',(0.,1.,0.));
#53222=CARTESIAN_POINT('Ctrl Pts',(0.0912596999148859,1.,-3.74888939116259));
#53223=CARTESIAN_POINT('Ctrl Pts',(0.0912596999148859,0.666666666666667,
-3.74888939116259));
#53224=CARTESIAN_POINT('Ctrl Pts',(0.091259699914886,0.333333333333333,
-3.74888939116259));
#53225=CARTESIAN_POINT('Ctrl Pts',(0.091259699914886,-0.333333333333333,
-3.74888939116259));
#53226=CARTESIAN_POINT('Ctrl Pts',(0.091259699914886,-0.666666666666667,
-3.74888939116259));
#53227=CARTESIAN_POINT('Ctrl Pts',(0.091259699914886,-1.,-3.74888939116259));
#53228=CARTESIAN_POINT('Ctrl Pts',(0.253646344052522,-1.,-4.1923339003649));
#53229=CARTESIAN_POINT('Ctrl Pts',(0.253646344052522,1.,-4.1923339003649));
#53230=CARTESIAN_POINT('Ctrl Pts',(0.25286086157284,-1.,-4.19097151819684));
#53231=CARTESIAN_POINT('Ctrl Pts',(0.25286086157284,1.,-4.19097151819684));
#53232=CARTESIAN_POINT('Ctrl Pts',(0.25129323983844,-1.,-4.18824585245272));
#53233=CARTESIAN_POINT('Ctrl Pts',(0.25129323983844,1.,-4.18824585245272));
#53234=CARTESIAN_POINT('Ctrl Pts',(0.248951836912189,-1.,-4.18415464961466));
#53235=CARTESIAN_POINT('Ctrl Pts',(0.248951836912189,1.,-4.18415464961466));
#53236=CARTESIAN_POINT('Ctrl Pts',(0.245850033420019,-1.,-4.1786943019518));
#53237=CARTESIAN_POINT('Ctrl Pts',(0.245850033420019,1.,-4.1786943019518));
#53238=CARTESIAN_POINT('Ctrl Pts',(0.242006283925088,-1.,-4.17185984411426));
#53239=CARTESIAN_POINT('Ctrl Pts',(0.242006283925088,1.,-4.17185984411426));
#53240=CARTESIAN_POINT('Ctrl Pts',(0.238196140934616,-1.,-4.16501636654877));
#53241=CARTESIAN_POINT('Ctrl Pts',(0.238196140934616,1.,-4.16501636654877));
#53242=CARTESIAN_POINT('Ctrl Pts',(0.234419749543207,-1.,-4.15816389265352));
#53243=CARTESIAN_POINT('Ctrl Pts',(0.234419749543207,1.,-4.15816389265352));
#53244=CARTESIAN_POINT('Ctrl Pts',(0.230677299028383,-1.,-4.15130247434459));
#53245=CARTESIAN_POINT('Ctrl Pts',(0.230677299028383,1.,-4.15130247434459));
#53246=CARTESIAN_POINT('Ctrl Pts',(0.226969025060705,-1.,-4.14443220606869));
#53247=CARTESIAN_POINT('Ctrl Pts',(0.226969025060705,1.,-4.14443220606869));
#53248=CARTESIAN_POINT('Ctrl Pts',(0.223295201037885,-1.,-4.13755320552764));
#53249=CARTESIAN_POINT('Ctrl Pts',(0.223295201037885,1.,-4.13755320552764));
#53250=CARTESIAN_POINT('Ctrl Pts',(0.219656126701541,-1.,-4.13066558697658));
#53251=CARTESIAN_POINT('Ctrl Pts',(0.219656126701541,1.,-4.13066558697658));
#53252=CARTESIAN_POINT('Ctrl Pts',(0.216052116898351,-1.,-4.12376943492132));
#53253=CARTESIAN_POINT('Ctrl Pts',(0.216052116898351,1.,-4.12376943492132));
#53254=CARTESIAN_POINT('Ctrl Pts',(0.212483491087189,-1.,-4.11686478264739));
#53255=CARTESIAN_POINT('Ctrl Pts',(0.212483491087189,1.,-4.11686478264739));
#53256=CARTESIAN_POINT('Ctrl Pts',(0.208950559400392,-1.,-4.10995157639377));
#53257=CARTESIAN_POINT('Ctrl Pts',(0.208950559400392,1.,-4.10995157639377));
#53258=CARTESIAN_POINT('Ctrl Pts',(0.205453622198454,-1.,-4.10302969965728));
#53259=CARTESIAN_POINT('Ctrl Pts',(0.205453622198454,1.,-4.10302969965728));
#53260=CARTESIAN_POINT('Ctrl Pts',(0.201992979050135,-1.,-4.09609903752152));
#53261=CARTESIAN_POINT('Ctrl Pts',(0.201992979050135,1.,-4.09609903752152));
#53262=CARTESIAN_POINT('Ctrl Pts',(0.198568934800861,-1.,-4.08915953359833));
#53263=CARTESIAN_POINT('Ctrl Pts',(0.198568934800861,1.,-4.08915953359833));
#53264=CARTESIAN_POINT('Ctrl Pts',(0.195181806054675,-1.,-4.08221124060322));
#53265=CARTESIAN_POINT('Ctrl Pts',(0.195181806054675,1.,-4.08221124060322));
#53266=CARTESIAN_POINT('Ctrl Pts',(0.19183192818099,-1.,-4.07525439702992));
#53267=CARTESIAN_POINT('Ctrl Pts',(0.19183192818099,1.,-4.07525439702992));
#53268=CARTESIAN_POINT('Ctrl Pts',(0.188519658060155,-1.,-4.06828941192147));
#53269=CARTESIAN_POINT('Ctrl Pts',(0.188519658060155,1.,-4.06828941192147));
#53270=CARTESIAN_POINT('Ctrl Pts',(0.185245370038873,-1.,-4.06131670998469));
#53271=CARTESIAN_POINT('Ctrl Pts',(0.185245370038873,1.,-4.06131670998469));
#53272=CARTESIAN_POINT('Ctrl Pts',(0.182009453048519,-1.,-4.05433660358353));
#53273=CARTESIAN_POINT('Ctrl Pts',(0.182009453048519,1.,-4.05433660358353));
#53274=CARTESIAN_POINT('Ctrl Pts',(0.178812307240728,-1.,-4.04734916719741));
#53275=CARTESIAN_POINT('Ctrl Pts',(0.178812307240728,1.,-4.04734916719741));
#53276=CARTESIAN_POINT('Ctrl Pts',(0.175654339673797,-1.,-4.04035407891222));
#53277=CARTESIAN_POINT('Ctrl Pts',(0.175654339673797,1.,-4.04035407891222));
#53278=CARTESIAN_POINT('Ctrl Pts',(0.172535962484514,-1.,-4.03335057326163));
#53279=CARTESIAN_POINT('Ctrl Pts',(0.172535962484514,1.,-4.03335057326163));
#53280=CARTESIAN_POINT('Ctrl Pts',(0.169457601001691,-1.,-4.02633779703764));
#53281=CARTESIAN_POINT('Ctrl Pts',(0.169457601001691,1.,-4.02633779703764));
#53282=CARTESIAN_POINT('Ctrl Pts',(0.166419700015865,-1.,-4.01931510507167));
#53283=CARTESIAN_POINT('Ctrl Pts',(0.166419700015865,1.,-4.01931510507167));
#53284=CARTESIAN_POINT('Ctrl Pts',(0.163422730287456,-1.,-4.01228237022296));
#53285=CARTESIAN_POINT('Ctrl Pts',(0.163422730287456,1.,-4.01228237022296));
#53286=CARTESIAN_POINT('Ctrl Pts',(0.160467194882202,-1.,-4.00524031064487));
#53287=CARTESIAN_POINT('Ctrl Pts',(0.160467194882202,1.,-4.00524031064487));
#53288=CARTESIAN_POINT('Ctrl Pts',(0.15755363438379,-1.,-3.9981907463185));
#53289=CARTESIAN_POINT('Ctrl Pts',(0.15755363438379,1.,-3.9981907463185));
#53290=CARTESIAN_POINT('Ctrl Pts',(0.154682618338547,-1.,-3.99113582086043));
#53291=CARTESIAN_POINT('Ctrl Pts',(0.154682618338547,1.,-3.99113582086043));
#53292=CARTESIAN_POINT('Ctrl Pts',(0.151854737441398,-1.,-3.98407729850975));
#53293=CARTESIAN_POINT('Ctrl Pts',(0.151854737441398,1.,-3.98407729850975));
#53294=CARTESIAN_POINT('Ctrl Pts',(0.149070594803544,-1.,-3.97701581473644));
#53295=CARTESIAN_POINT('Ctrl Pts',(0.149070594803544,1.,-3.97701581473644));
#53296=CARTESIAN_POINT('Ctrl Pts',(0.14633079781452,-1.,-3.96995018565893));
#53297=CARTESIAN_POINT('Ctrl Pts',(0.14633079781452,1.,-3.96995018565893));
#53298=CARTESIAN_POINT('Ctrl Pts',(0.143635947692798,-1.,-3.96287658098896));
#53299=CARTESIAN_POINT('Ctrl Pts',(0.143635947692798,1.,-3.96287658098896));
#53300=CARTESIAN_POINT('Ctrl Pts',(0.140986665829942,-1.,-3.95579014116894));
#53301=CARTESIAN_POINT('Ctrl Pts',(0.140986665829942,1.,-3.95579014116894));
#53302=CARTESIAN_POINT('Ctrl Pts',(0.138383621255161,-1.,-3.94868667844347));
#53303=CARTESIAN_POINT('Ctrl Pts',(0.138383621255161,1.,-3.94868667844347));
#53304=CARTESIAN_POINT('Ctrl Pts',(0.135827558661188,-1.,-3.94156445130741));
#53305=CARTESIAN_POINT('Ctrl Pts',(0.135827558661188,1.,-3.94156445130741));
#53306=CARTESIAN_POINT('Ctrl Pts',(0.13331932279419,-1.,-3.93442567551042));
#53307=CARTESIAN_POINT('Ctrl Pts',(0.13331932279419,1.,-3.93442567551042));
#53308=CARTESIAN_POINT('Ctrl Pts',(0.130859892027801,-1.,-3.92727876795977));
#53309=CARTESIAN_POINT('Ctrl Pts',(0.130859892027801,1.,-3.92727876795977));
#53310=CARTESIAN_POINT('Ctrl Pts',(0.128450341339532,-1.,-3.92013513251664));
#53311=CARTESIAN_POINT('Ctrl Pts',(0.128450341339532,1.,-3.92013513251664));
#53312=CARTESIAN_POINT('Ctrl Pts',(0.126091793324141,-1.,-3.91300501605411));
#53313=CARTESIAN_POINT('Ctrl Pts',(0.126091793324141,1.,-3.91300501605411));
#53314=CARTESIAN_POINT('Ctrl Pts',(0.123785368272379,-1.,-3.90589336320515));
#53315=CARTESIAN_POINT('Ctrl Pts',(0.123785368272379,1.,-3.90589336320515));
#53316=CARTESIAN_POINT('Ctrl Pts',(0.121532144765721,-1.,-3.89879639336939));
#53317=CARTESIAN_POINT('Ctrl Pts',(0.121532144765721,1.,-3.89879639336939));
#53318=CARTESIAN_POINT('Ctrl Pts',(0.11933308819041,-1.,-3.8916960010517));
#53319=CARTESIAN_POINT('Ctrl Pts',(0.11933308819041,1.,-3.8916960010517));
#53320=CARTESIAN_POINT('Ctrl Pts',(0.117189150373134,-1.,-3.88456590045726));
#53321=CARTESIAN_POINT('Ctrl Pts',(0.117189150373134,1.,-3.88456590045726));
#53322=CARTESIAN_POINT('Ctrl Pts',(0.11510142664946,-1.,-3.87738168405308));
#53323=CARTESIAN_POINT('Ctrl Pts',(0.11510142664946,1.,-3.87738168405308));
#53324=CARTESIAN_POINT('Ctrl Pts',(0.113071304914558,-1.,-3.87013043445001));
#53325=CARTESIAN_POINT('Ctrl Pts',(0.113071304914558,1.,-3.87013043445001));
#53326=CARTESIAN_POINT('Ctrl Pts',(0.111100593036266,-1.,-3.86281867282984));
#53327=CARTESIAN_POINT('Ctrl Pts',(0.111100593036266,1.,-3.86281867282984));
#53328=CARTESIAN_POINT('Ctrl Pts',(0.10919171763496,-1.,-3.85548571496953));
#53329=CARTESIAN_POINT('Ctrl Pts',(0.10919171763496,1.,-3.85548571496953));
#53330=CARTESIAN_POINT('Ctrl Pts',(0.107347597812208,-1.,-3.84819233070391));
#53331=CARTESIAN_POINT('Ctrl Pts',(0.107347597812208,1.,-3.84819233070391));
#53332=CARTESIAN_POINT('Ctrl Pts',(0.105571360916593,-1.,-3.84099658324873));
#53333=CARTESIAN_POINT('Ctrl Pts',(0.105571360916593,1.,-3.84099658324873));
#53334=CARTESIAN_POINT('Ctrl Pts',(0.103866063811634,-1.,-3.83393171228034));
#53335=CARTESIAN_POINT('Ctrl Pts',(0.103866063811634,1.,-3.83393171228034));
#53336=CARTESIAN_POINT('Ctrl Pts',(0.102234506488445,-1.,-3.8269873714322));
#53337=CARTESIAN_POINT('Ctrl Pts',(0.102234506488445,1.,-3.8269873714322));
#53338=CARTESIAN_POINT('Ctrl Pts',(0.100678769650594,-1.,-3.82007889742512));
#53339=CARTESIAN_POINT('Ctrl Pts',(0.100678769650594,1.,-3.82007889742512));
#53340=CARTESIAN_POINT('Ctrl Pts',(0.099200872809594,-1.,-3.81306649386293));
#53341=CARTESIAN_POINT('Ctrl Pts',(0.099200872809594,1.,-3.81306649386293));
#53342=CARTESIAN_POINT('Ctrl Pts',(0.0978042222906071,-1.,-3.80581088847642));
#53343=CARTESIAN_POINT('Ctrl Pts',(0.0978042222906071,1.,-3.80581088847642));
#53344=CARTESIAN_POINT('Ctrl Pts',(0.0964949352872842,-1.,-3.7982212851376));
#53345=CARTESIAN_POINT('Ctrl Pts',(0.0964949352872842,1.,-3.7982212851376));
#53346=CARTESIAN_POINT('Ctrl Pts',(0.0952829885101065,-1.,-3.79030016353186));
#53347=CARTESIAN_POINT('Ctrl Pts',(0.0952829885101065,1.,-3.79030016353186));
#53348=CARTESIAN_POINT('Ctrl Pts',(0.094184009509174,-1.,-3.78220521899366));
#53349=CARTESIAN_POINT('Ctrl Pts',(0.094184009509174,1.,-3.78220521899366));
#53350=CARTESIAN_POINT('Ctrl Pts',(0.0932185546204571,-1.,-3.77424159971456));
#53351=CARTESIAN_POINT('Ctrl Pts',(0.0932185546204571,1.,-3.77424159971456));
#53352=CARTESIAN_POINT('Ctrl Pts',(0.0924090589604052,-1.,-3.76678860032228));
#53353=CARTESIAN_POINT('Ctrl Pts',(0.0924090589604052,1.,-3.76678860032228));
#53354=CARTESIAN_POINT('Ctrl Pts',(0.0917773084999005,-1.,-3.76024199359493));
#53355=CARTESIAN_POINT('Ctrl Pts',(0.0917773084999005,1.,-3.76024199359493));
#53356=CARTESIAN_POINT('Ctrl Pts',(0.0913419622735849,-1.,-3.75495560118053));
#53357=CARTESIAN_POINT('Ctrl Pts',(0.0913419622735849,1.,-3.75495560118053));
#53358=CARTESIAN_POINT('Ctrl Pts',(0.0911154000996403,-1.,-3.75116949194125));
#53359=CARTESIAN_POINT('Ctrl Pts',(0.0911154000996403,1.,-3.75116949194125));
#53360=CARTESIAN_POINT('Ctrl Pts',(0.0911057547504657,-1.,-3.74943097853257));
#53361=CARTESIAN_POINT('Ctrl Pts',(0.0911057547504657,1.,-3.74943097853257));
#53362=CARTESIAN_POINT('Ctrl Pts',(0.0911958743733922,-1.,-3.7488701717383));
#53363=CARTESIAN_POINT('Ctrl Pts',(0.0911958743733922,1.,-3.7488701717383));
#53364=CARTESIAN_POINT('Ctrl Pts',(0.0912992005792088,-1.,-3.74882632118923));
#53365=CARTESIAN_POINT('Ctrl Pts',(0.0912992005792088,1.,-3.74882632118923));
#53366=CARTESIAN_POINT('Ctrl Pts',(0.0913616755937425,-1.,-3.74888690736767));
#53367=CARTESIAN_POINT('Ctrl Pts',(0.0913616755937425,1.,-3.74888690736767));
#53368=CARTESIAN_POINT('',(0.253646344052522,1.,-4.1923339003649));
#53369=CARTESIAN_POINT('Ctrl Pts',(0.253646344052522,1.,-4.1923339003649));
#53370=CARTESIAN_POINT('Ctrl Pts',(0.25286086157284,1.,-4.19097151819684));
#53371=CARTESIAN_POINT('Ctrl Pts',(0.25129323983844,1.,-4.18824585245272));
#53372=CARTESIAN_POINT('Ctrl Pts',(0.248951836912189,1.,-4.18415464961466));
#53373=CARTESIAN_POINT('Ctrl Pts',(0.245850033420019,1.,-4.1786943019518));
#53374=CARTESIAN_POINT('Ctrl Pts',(0.242006283925088,1.,-4.17185984411426));
#53375=CARTESIAN_POINT('Ctrl Pts',(0.238196140934616,1.,-4.16501636654877));
#53376=CARTESIAN_POINT('Ctrl Pts',(0.234419749543207,1.,-4.15816389265352));
#53377=CARTESIAN_POINT('Ctrl Pts',(0.230677299028383,1.,-4.15130247434459));
#53378=CARTESIAN_POINT('Ctrl Pts',(0.226969025060705,1.,-4.14443220606869));
#53379=CARTESIAN_POINT('Ctrl Pts',(0.223295201037885,1.,-4.13755320552764));
#53380=CARTESIAN_POINT('Ctrl Pts',(0.219656126701541,1.,-4.13066558697658));
#53381=CARTESIAN_POINT('Ctrl Pts',(0.216052116898351,1.,-4.12376943492132));
#53382=CARTESIAN_POINT('Ctrl Pts',(0.212483491087189,1.,-4.11686478264739));
#53383=CARTESIAN_POINT('Ctrl Pts',(0.208950559400392,1.,-4.10995157639377));
#53384=CARTESIAN_POINT('Ctrl Pts',(0.205453622198454,1.,-4.10302969965728));
#53385=CARTESIAN_POINT('Ctrl Pts',(0.201992979050135,1.,-4.09609903752152));
#53386=CARTESIAN_POINT('Ctrl Pts',(0.198568934800861,1.,-4.08915953359833));
#53387=CARTESIAN_POINT('Ctrl Pts',(0.195181806054675,1.,-4.08221124060322));
#53388=CARTESIAN_POINT('Ctrl Pts',(0.19183192818099,1.,-4.07525439702992));
#53389=CARTESIAN_POINT('Ctrl Pts',(0.188519658060155,1.,-4.06828941192147));
#53390=CARTESIAN_POINT('Ctrl Pts',(0.185245370038873,1.,-4.06131670998469));
#53391=CARTESIAN_POINT('Ctrl Pts',(0.182009453048519,1.,-4.05433660358353));
#53392=CARTESIAN_POINT('Ctrl Pts',(0.178812307240728,1.,-4.04734916719741));
#53393=CARTESIAN_POINT('Ctrl Pts',(0.175654339673797,1.,-4.04035407891222));
#53394=CARTESIAN_POINT('Ctrl Pts',(0.172535962484514,1.,-4.03335057326163));
#53395=CARTESIAN_POINT('Ctrl Pts',(0.169457601001691,1.,-4.02633779703764));
#53396=CARTESIAN_POINT('Ctrl Pts',(0.166419700015865,1.,-4.01931510507167));
#53397=CARTESIAN_POINT('Ctrl Pts',(0.163422730287456,1.,-4.01228237022296));
#53398=CARTESIAN_POINT('Ctrl Pts',(0.160467194882202,1.,-4.00524031064487));
#53399=CARTESIAN_POINT('Ctrl Pts',(0.15755363438379,1.,-3.9981907463185));
#53400=CARTESIAN_POINT('Ctrl Pts',(0.154682618338547,1.,-3.99113582086043));
#53401=CARTESIAN_POINT('Ctrl Pts',(0.151854737441398,1.,-3.98407729850975));
#53402=CARTESIAN_POINT('Ctrl Pts',(0.149070594803544,1.,-3.97701581473644));
#53403=CARTESIAN_POINT('Ctrl Pts',(0.14633079781452,1.,-3.96995018565893));
#53404=CARTESIAN_POINT('Ctrl Pts',(0.143635947692798,1.,-3.96287658098896));
#53405=CARTESIAN_POINT('Ctrl Pts',(0.140986665829942,1.,-3.95579014116894));
#53406=CARTESIAN_POINT('Ctrl Pts',(0.138383621255161,1.,-3.94868667844347));
#53407=CARTESIAN_POINT('Ctrl Pts',(0.135827558661188,1.,-3.94156445130741));
#53408=CARTESIAN_POINT('Ctrl Pts',(0.13331932279419,1.,-3.93442567551042));
#53409=CARTESIAN_POINT('Ctrl Pts',(0.130859892027801,1.,-3.92727876795977));
#53410=CARTESIAN_POINT('Ctrl Pts',(0.128450341339532,1.,-3.92013513251664));
#53411=CARTESIAN_POINT('Ctrl Pts',(0.126091793324141,1.,-3.91300501605411));
#53412=CARTESIAN_POINT('Ctrl Pts',(0.123785368272379,1.,-3.90589336320515));
#53413=CARTESIAN_POINT('Ctrl Pts',(0.121532144765721,1.,-3.89879639336939));
#53414=CARTESIAN_POINT('Ctrl Pts',(0.11933308819041,1.,-3.8916960010517));
#53415=CARTESIAN_POINT('Ctrl Pts',(0.117189150373134,1.,-3.88456590045726));
#53416=CARTESIAN_POINT('Ctrl Pts',(0.11510142664946,1.,-3.87738168405308));
#53417=CARTESIAN_POINT('Ctrl Pts',(0.113071304914558,1.,-3.87013043445001));
#53418=CARTESIAN_POINT('Ctrl Pts',(0.111100593036266,1.,-3.86281867282984));
#53419=CARTESIAN_POINT('Ctrl Pts',(0.10919171763496,1.,-3.85548571496953));
#53420=CARTESIAN_POINT('Ctrl Pts',(0.107347597812208,1.,-3.84819233070391));
#53421=CARTESIAN_POINT('Ctrl Pts',(0.105571360916593,1.,-3.84099658324873));
#53422=CARTESIAN_POINT('Ctrl Pts',(0.103866063811634,1.,-3.83393171228034));
#53423=CARTESIAN_POINT('Ctrl Pts',(0.102234506488445,1.,-3.8269873714322));
#53424=CARTESIAN_POINT('Ctrl Pts',(0.100678769650594,1.,-3.82007889742512));
#53425=CARTESIAN_POINT('Ctrl Pts',(0.099200872809594,1.,-3.81306649386293));
#53426=CARTESIAN_POINT('Ctrl Pts',(0.0978042222906071,1.,-3.80581088847642));
#53427=CARTESIAN_POINT('Ctrl Pts',(0.0964949352872842,1.,-3.7982212851376));
#53428=CARTESIAN_POINT('Ctrl Pts',(0.0952829885101065,1.,-3.79030016353186));
#53429=CARTESIAN_POINT('Ctrl Pts',(0.094184009509174,1.,-3.78220521899366));
#53430=CARTESIAN_POINT('Ctrl Pts',(0.0932185546204571,1.,-3.77424159971456));
#53431=CARTESIAN_POINT('Ctrl Pts',(0.0924090589604052,1.,-3.76678860032228));
#53432=CARTESIAN_POINT('Ctrl Pts',(0.0917773084999005,1.,-3.76024199359493));
#53433=CARTESIAN_POINT('Ctrl Pts',(0.0913419622735849,1.,-3.75495560118053));
#53434=CARTESIAN_POINT('Ctrl Pts',(0.0911323999576141,1.,-3.75145357872511));
#53435=CARTESIAN_POINT('Ctrl Pts',(0.0911090736804567,1.,-3.74976844886495));
#53436=CARTESIAN_POINT('Ctrl Pts',(0.0911666301806421,1.,-3.74911539914664));
#53437=CARTESIAN_POINT('Ctrl Pts',(0.0912308016409228,1.,-3.74892890041021));
#53438=CARTESIAN_POINT('Ctrl Pts',(0.0912596999148853,1.,-3.74888939116259));
#53439=CARTESIAN_POINT('',(0.253646344052522,0.,-4.1923339003649));
#53440=CARTESIAN_POINT('Ctrl Pts',(0.496218256089212,-1.,-3.71702400346349));
#53441=CARTESIAN_POINT('Ctrl Pts',(0.496218256089212,1.,-3.71702400346349));
#53442=CARTESIAN_POINT('Ctrl Pts',(0.496270484166408,-1.,-3.7169543899574));
#53443=CARTESIAN_POINT('Ctrl Pts',(0.496270484166408,1.,-3.7169543899574));
#53444=CARTESIAN_POINT('Ctrl Pts',(0.496379397992639,-1.,-3.71698153685602));
#53445=CARTESIAN_POINT('Ctrl Pts',(0.496379397992639,1.,-3.71698153685602));
#53446=CARTESIAN_POINT('Ctrl Pts',(0.496556137604532,-1.,-3.71752134137482));
#53447=CARTESIAN_POINT('Ctrl Pts',(0.496556137604532,1.,-3.71752134137482));
#53448=CARTESIAN_POINT('Ctrl Pts',(0.496818574420595,-1.,-3.71923995966302));
#53449=CARTESIAN_POINT('Ctrl Pts',(0.496818574420595,1.,-3.71923995966302));
#53450=CARTESIAN_POINT('Ctrl Pts',(0.497187079575988,-1.,-3.72301489774398));
#53451=CARTESIAN_POINT('Ctrl Pts',(0.497187079575988,1.,-3.72301489774398));
#53452=CARTESIAN_POINT('Ctrl Pts',(0.497584067153049,-1.,-3.72830430904606));
#53453=CARTESIAN_POINT('Ctrl Pts',(0.497584067153049,1.,-3.72830430904606));
#53454=CARTESIAN_POINT('Ctrl Pts',(0.497984209510024,-1.,-3.73486914372449));
#53455=CARTESIAN_POINT('Ctrl Pts',(0.497984209510024,1.,-3.73486914372449));
#53456=CARTESIAN_POINT('Ctrl Pts',(0.498350586057692,-1.,-3.74235701734714));
#53457=CARTESIAN_POINT('Ctrl Pts',(0.498350586057692,1.,-3.74235701734714));
#53458=CARTESIAN_POINT('Ctrl Pts',(0.498642802042605,-1.,-3.75037362167839));
#53459=CARTESIAN_POINT('Ctrl Pts',(0.498642802042605,1.,-3.75037362167839));
#53460=CARTESIAN_POINT('Ctrl Pts',(0.498823681615421,-1.,-3.75854082221052));
#53461=CARTESIAN_POINT('Ctrl Pts',(0.498823681615421,1.,-3.75854082221052));
#53462=CARTESIAN_POINT('Ctrl Pts',(0.49886579233529,-1.,-3.76655401191229));
#53463=CARTESIAN_POINT('Ctrl Pts',(0.49886579233529,1.,-3.76655401191229));
#53464=CARTESIAN_POINT('Ctrl Pts',(0.498759900365891,-1.,-3.77425499225255));
#53465=CARTESIAN_POINT('Ctrl Pts',(0.498759900365891,1.,-3.77425499225255));
#53466=CARTESIAN_POINT('Ctrl Pts',(0.498515471679584,-1.,-3.78163975337356));
#53467=CARTESIAN_POINT('Ctrl Pts',(0.498515471679584,1.,-3.78163975337356));
#53468=CARTESIAN_POINT('Ctrl Pts',(0.498152751800958,-1.,-3.78879701661264));
#53469=CARTESIAN_POINT('Ctrl Pts',(0.498152751800958,1.,-3.78879701661264));
#53470=CARTESIAN_POINT('Ctrl Pts',(0.497696892100624,-1.,-3.79586380669994));
#53471=CARTESIAN_POINT('Ctrl Pts',(0.497696892100624,1.,-3.79586380669994));
#53472=CARTESIAN_POINT('Ctrl Pts',(0.497171756201051,-1.,-3.80297788298514));
#53473=CARTESIAN_POINT('Ctrl Pts',(0.497171756201051,1.,-3.80297788298514));
#53474=CARTESIAN_POINT('Ctrl Pts',(0.496592643443704,-1.,-3.81022254090839));
#53475=CARTESIAN_POINT('Ctrl Pts',(0.496592643443704,1.,-3.81022254090839));
#53476=CARTESIAN_POINT('Ctrl Pts',(0.495963937875479,-1.,-3.81760756144025));
#53477=CARTESIAN_POINT('Ctrl Pts',(0.495963937875479,1.,-3.81760756144025));
#53478=CARTESIAN_POINT('Ctrl Pts',(0.495283458893837,-1.,-3.82509963594103));
#53479=CARTESIAN_POINT('Ctrl Pts',(0.495283458893837,1.,-3.82509963594103));
#53480=CARTESIAN_POINT('Ctrl Pts',(0.494545212256401,-1.,-3.83264092682431));
#53481=CARTESIAN_POINT('Ctrl Pts',(0.494545212256401,1.,-3.83264092682431));
#53482=CARTESIAN_POINT('Ctrl Pts',(0.493742574629134,-1.,-3.84017095578451));
#53483=CARTESIAN_POINT('Ctrl Pts',(0.493742574629134,1.,-3.84017095578451));
#53484=CARTESIAN_POINT('Ctrl Pts',(0.49287179241414,-1.,-3.84765051147999));
#53485=CARTESIAN_POINT('Ctrl Pts',(0.49287179241414,1.,-3.84765051147999));
#53486=CARTESIAN_POINT('Ctrl Pts',(0.491933631083813,-1.,-3.85507287020263));
#53487=CARTESIAN_POINT('Ctrl Pts',(0.491933631083813,1.,-3.85507287020263));
#53488=CARTESIAN_POINT('Ctrl Pts',(0.490931482170891,-1.,-3.86245057319246));
#53489=CARTESIAN_POINT('Ctrl Pts',(0.490931482170891,1.,-3.86245057319246));
#53490=CARTESIAN_POINT('Ctrl Pts',(0.489870245704917,-1.,-3.86980755613707));
#53491=CARTESIAN_POINT('Ctrl Pts',(0.489870245704917,1.,-3.86980755613707));
#53492=CARTESIAN_POINT('Ctrl Pts',(0.488754973798273,-1.,-3.87716963231109));
#53493=CARTESIAN_POINT('Ctrl Pts',(0.488754973798273,1.,-3.87716963231109));
#53494=CARTESIAN_POINT('Ctrl Pts',(0.487589452275154,-1.,-3.88455453328138));
#53495=CARTESIAN_POINT('Ctrl Pts',(0.487589452275154,1.,-3.88455453328138));
#53496=CARTESIAN_POINT('Ctrl Pts',(0.486375337854103,-1.,-3.89196582437552));
#53497=CARTESIAN_POINT('Ctrl Pts',(0.486375337854103,1.,-3.89196582437552));
#53498=CARTESIAN_POINT('Ctrl Pts',(0.485112963522222,-1.,-3.89939844658513));
#53499=CARTESIAN_POINT('Ctrl Pts',(0.485112963522222,1.,-3.89939844658513));
#53500=CARTESIAN_POINT('Ctrl Pts',(0.48380183508915,-1.,-3.90684210358056));
#53501=CARTESIAN_POINT('Ctrl Pts',(0.48380183508915,1.,-3.90684210358056));
#53502=CARTESIAN_POINT('Ctrl Pts',(0.482441230340713,-1.,-3.91428536373751));
#53503=CARTESIAN_POINT('Ctrl Pts',(0.482441230340713,1.,-3.91428536373751));
#53504=CARTESIAN_POINT('Ctrl Pts',(0.481030798910748,-1.,-3.92171976072341));
#53505=CARTESIAN_POINT('Ctrl Pts',(0.481030798910748,1.,-3.92171976072341));
#53506=CARTESIAN_POINT('Ctrl Pts',(0.479571028525578,-1.,-3.92914297392071));
#53507=CARTESIAN_POINT('Ctrl Pts',(0.479571028525578,1.,-3.92914297392071));
#53508=CARTESIAN_POINT('Ctrl Pts',(0.478062927140964,-1.,-3.93655660689819));
#53509=CARTESIAN_POINT('Ctrl Pts',(0.478062927140964,1.,-3.93655660689819));
#53510=CARTESIAN_POINT('Ctrl Pts',(0.476507810658537,-1.,-3.94396469119383));
#53511=CARTESIAN_POINT('Ctrl Pts',(0.476507810658537,1.,-3.94396469119383));
#53512=CARTESIAN_POINT('Ctrl Pts',(0.47490705302179,-1.,-3.95137192932897));
#53513=CARTESIAN_POINT('Ctrl Pts',(0.47490705302179,1.,-3.95137192932897));
#53514=CARTESIAN_POINT('Ctrl Pts',(0.473261847236297,-1.,-3.95878201038338));
#53515=CARTESIAN_POINT('Ctrl Pts',(0.473261847236297,1.,-3.95878201038338));
#53516=CARTESIAN_POINT('Ctrl Pts',(0.471572978413503,-1.,-3.96619600864643));
#53517=CARTESIAN_POINT('Ctrl Pts',(0.471572978413503,1.,-3.96619600864643));
#53518=CARTESIAN_POINT('Ctrl Pts',(0.469840942829895,-1.,-3.97361320212436));
#53519=CARTESIAN_POINT('Ctrl Pts',(0.469840942829895,1.,-3.97361320212436));
#53520=CARTESIAN_POINT('Ctrl Pts',(0.468066047920157,-1.,-3.98103175589371));
#53521=CARTESIAN_POINT('Ctrl Pts',(0.468066047920157,1.,-3.98103175589371));
#53522=CARTESIAN_POINT('Ctrl Pts',(0.466248520883039,-1.,-3.98844946363262));
#53523=CARTESIAN_POINT('Ctrl Pts',(0.466248520883039,1.,-3.98844946363262));
#53524=CARTESIAN_POINT('Ctrl Pts',(0.464388610938975,-1.,-3.9958644432011));
#53525=CARTESIAN_POINT('Ctrl Pts',(0.464388610938975,1.,-3.9958644432011));
#53526=CARTESIAN_POINT('Ctrl Pts',(0.462486702616204,-1.,-4.00327590659075));
#53527=CARTESIAN_POINT('Ctrl Pts',(0.462486702616204,1.,-4.00327590659075));
#53528=CARTESIAN_POINT('Ctrl Pts',(0.460543280768514,-1.,-4.01068390573399));
#53529=CARTESIAN_POINT('Ctrl Pts',(0.460543280768514,1.,-4.01068390573399));
#53530=CARTESIAN_POINT('Ctrl Pts',(0.458558885636945,-1.,-4.01808900827587));
#53531=CARTESIAN_POINT('Ctrl Pts',(0.458558885636945,1.,-4.01808900827587));
#53532=CARTESIAN_POINT('Ctrl Pts',(0.45653407078495,-1.,-4.02549199038394));
#53533=CARTESIAN_POINT('Ctrl Pts',(0.45653407078495,1.,-4.02549199038394));
#53534=CARTESIAN_POINT('Ctrl Pts',(0.454469363020541,-1.,-4.03289354362794));
#53535=CARTESIAN_POINT('Ctrl Pts',(0.454469363020541,1.,-4.03289354362794));
#53536=CARTESIAN_POINT('Ctrl Pts',(0.452365214748892,-1.,-4.04029392228049));
#53537=CARTESIAN_POINT('Ctrl Pts',(0.452365214748892,1.,-4.04029392228049));
#53538=CARTESIAN_POINT('Ctrl Pts',(0.450222009543926,-1.,-4.0476929901813));
#53539=CARTESIAN_POINT('Ctrl Pts',(0.450222009543926,1.,-4.0476929901813));
#53540=CARTESIAN_POINT('Ctrl Pts',(0.448040082684114,-1.,-4.0550903779696));
#53541=CARTESIAN_POINT('Ctrl Pts',(0.448040082684114,1.,-4.0550903779696));
#53542=CARTESIAN_POINT('Ctrl Pts',(0.445819737468537,-1.,-4.06248560760659));
#53543=CARTESIAN_POINT('Ctrl Pts',(0.445819737468537,1.,-4.06248560760659));
#53544=CARTESIAN_POINT('Ctrl Pts',(0.443561262395332,-1.,-4.0698782192569));
#53545=CARTESIAN_POINT('Ctrl Pts',(0.443561262395332,1.,-4.0698782192569));
#53546=CARTESIAN_POINT('Ctrl Pts',(0.44126495139636,-1.,-4.07726792490016));
#53547=CARTESIAN_POINT('Ctrl Pts',(0.44126495139636,1.,-4.07726792490016));
#53548=CARTESIAN_POINT('Ctrl Pts',(0.438931108931279,-1.,-4.08465462294273));
#53549=CARTESIAN_POINT('Ctrl Pts',(0.438931108931279,1.,-4.08465462294273));
#53550=CARTESIAN_POINT('Ctrl Pts',(0.436560044913482,-1.,-4.09203832139089));
#53551=CARTESIAN_POINT('Ctrl Pts',(0.436560044913482,1.,-4.09203832139089));
#53552=CARTESIAN_POINT('Ctrl Pts',(0.43415207320046,-1.,-4.09941908688373));
#53553=CARTESIAN_POINT('Ctrl Pts',(0.43415207320046,1.,-4.09941908688373));
#53554=CARTESIAN_POINT('Ctrl Pts',(0.431707508679883,-1.,-4.10679698750336));
#53555=CARTESIAN_POINT('Ctrl Pts',(0.431707508679883,1.,-4.10679698750336));
#53556=CARTESIAN_POINT('Ctrl Pts',(0.429226666075844,-1.,-4.11417202783267));
#53557=CARTESIAN_POINT('Ctrl Pts',(0.429226666075844,1.,-4.11417202783267));
#53558=CARTESIAN_POINT('Ctrl Pts',(0.426709855707,-1.,-4.12154412502007));
#53559=CARTESIAN_POINT('Ctrl Pts',(0.426709855707,1.,-4.12154412502007));
#53560=CARTESIAN_POINT('Ctrl Pts',(0.424157375323975,-1.,-4.12891314634572));
#53561=CARTESIAN_POINT('Ctrl Pts',(0.424157375323975,1.,-4.12891314634572));
#53562=CARTESIAN_POINT('Ctrl Pts',(0.421569503104512,-1.,-4.13627893207002));
#53563=CARTESIAN_POINT('Ctrl Pts',(0.421569503104512,1.,-4.13627893207002));
#53564=CARTESIAN_POINT('Ctrl Pts',(0.418946490667702,-1.,-4.14364132317121));
#53565=CARTESIAN_POINT('Ctrl Pts',(0.418946490667702,1.,-4.14364132317121));
#53566=CARTESIAN_POINT('Ctrl Pts',(0.416288556008011,-1.,-4.15100018949965));
#53567=CARTESIAN_POINT('Ctrl Pts',(0.416288556008011,1.,-4.15100018949965));
#53568=CARTESIAN_POINT('Ctrl Pts',(0.41359587795147,-1.,-4.15835545017202));
#53569=CARTESIAN_POINT('Ctrl Pts',(0.41359587795147,1.,-4.15835545017202));
#53570=CARTESIAN_POINT('Ctrl Pts',(0.410868596146414,-1.,-4.16570705938425));
#53571=CARTESIAN_POINT('Ctrl Pts',(0.410868596146414,1.,-4.16570705938425));
#53572=CARTESIAN_POINT('Ctrl Pts',(0.408659167568273,-1.,-4.17158541007977));
#53573=CARTESIAN_POINT('Ctrl Pts',(0.408659167568273,1.,-4.17158541007977));
#53574=CARTESIAN_POINT('Ctrl Pts',(0.406986596325454,-1.,-4.17599251954382));
#53575=CARTESIAN_POINT('Ctrl Pts',(0.406986596325454,1.,-4.17599251954382));
#53576=CARTESIAN_POINT('Ctrl Pts',(0.405864662679209,-1.,-4.17892985789466));
#53577=CARTESIAN_POINT('Ctrl Pts',(0.405864662679209,1.,-4.17892985789466));
#53578=CARTESIAN_POINT('Ctrl Pts',(0.40530197431835,-1.,-4.18039834341342));
#53579=CARTESIAN_POINT('Ctrl Pts',(0.40530197431835,1.,-4.18039834341342));
#53580=CARTESIAN_POINT('',(0.496319364827593,1.,-3.71701050416825));
#53581=CARTESIAN_POINT('Ctrl Pts',(0.496319364827592,-1.,-3.71701050416825));
#53582=CARTESIAN_POINT('Ctrl Pts',(0.496319364827592,-0.666666666666667,
-3.71701050416825));
#53583=CARTESIAN_POINT('Ctrl Pts',(0.496319364827592,-0.333333333333333,
-3.71701050416825));
#53584=CARTESIAN_POINT('Ctrl Pts',(0.496319364827592,0.333333333333333,
-3.71701050416825));
#53585=CARTESIAN_POINT('Ctrl Pts',(0.496319364827592,0.666666666666667,
-3.71701050416825));
#53586=CARTESIAN_POINT('Ctrl Pts',(0.496319364827592,1.,-3.71701050416825));
#53587=CARTESIAN_POINT('',(0.40530197431835,1.,-4.18039834341342));
#53588=CARTESIAN_POINT('',(0.40530197431835,0.,-4.18039834341342));
#53589=CARTESIAN_POINT('Ctrl Pts',(0.496319364827593,1.,-3.71701050416825));
#53590=CARTESIAN_POINT('Ctrl Pts',(0.496354087924312,1.,-3.71704500630495));
#53591=CARTESIAN_POINT('Ctrl Pts',(0.496446644158005,1.,-3.71721917030355));
#53592=CARTESIAN_POINT('Ctrl Pts',(0.496605651525989,1.,-3.71785517607549));
#53593=CARTESIAN_POINT('Ctrl Pts',(0.496846224822564,1.,-3.71952320822499));
#53594=CARTESIAN_POINT('Ctrl Pts',(0.497187079575988,1.,-3.72301489774398));
#53595=CARTESIAN_POINT('Ctrl Pts',(0.497584067153049,1.,-3.72830430904606));
#53596=CARTESIAN_POINT('Ctrl Pts',(0.497984209510024,1.,-3.73486914372449));
#53597=CARTESIAN_POINT('Ctrl Pts',(0.498350586057692,1.,-3.74235701734714));
#53598=CARTESIAN_POINT('Ctrl Pts',(0.498642802042605,1.,-3.75037362167839));
#53599=CARTESIAN_POINT('Ctrl Pts',(0.498823681615421,1.,-3.75854082221052));
#53600=CARTESIAN_POINT('Ctrl Pts',(0.49886579233529,1.,-3.76655401191229));
#53601=CARTESIAN_POINT('Ctrl Pts',(0.498759900365891,1.,-3.77425499225255));
#53602=CARTESIAN_POINT('Ctrl Pts',(0.498515471679584,1.,-3.78163975337356));
#53603=CARTESIAN_POINT('Ctrl Pts',(0.498152751800958,1.,-3.78879701661264));
#53604=CARTESIAN_POINT('Ctrl Pts',(0.497696892100624,1.,-3.79586380669994));
#53605=CARTESIAN_POINT('Ctrl Pts',(0.497171756201051,1.,-3.80297788298514));
#53606=CARTESIAN_POINT('Ctrl Pts',(0.496592643443704,1.,-3.81022254090839));
#53607=CARTESIAN_POINT('Ctrl Pts',(0.495963937875479,1.,-3.81760756144025));
#53608=CARTESIAN_POINT('Ctrl Pts',(0.495283458893837,1.,-3.82509963594103));
#53609=CARTESIAN_POINT('Ctrl Pts',(0.494545212256401,1.,-3.83264092682431));
#53610=CARTESIAN_POINT('Ctrl Pts',(0.493742574629134,1.,-3.84017095578451));
#53611=CARTESIAN_POINT('Ctrl Pts',(0.49287179241414,1.,-3.84765051147999));
#53612=CARTESIAN_POINT('Ctrl Pts',(0.491933631083813,1.,-3.85507287020263));
#53613=CARTESIAN_POINT('Ctrl Pts',(0.490931482170891,1.,-3.86245057319246));
#53614=CARTESIAN_POINT('Ctrl Pts',(0.489870245704917,1.,-3.86980755613707));
#53615=CARTESIAN_POINT('Ctrl Pts',(0.488754973798273,1.,-3.87716963231109));
#53616=CARTESIAN_POINT('Ctrl Pts',(0.487589452275154,1.,-3.88455453328138));
#53617=CARTESIAN_POINT('Ctrl Pts',(0.486375337854103,1.,-3.89196582437552));
#53618=CARTESIAN_POINT('Ctrl Pts',(0.485112963522222,1.,-3.89939844658513));
#53619=CARTESIAN_POINT('Ctrl Pts',(0.48380183508915,1.,-3.90684210358056));
#53620=CARTESIAN_POINT('Ctrl Pts',(0.482441230340713,1.,-3.91428536373751));
#53621=CARTESIAN_POINT('Ctrl Pts',(0.481030798910748,1.,-3.92171976072341));
#53622=CARTESIAN_POINT('Ctrl Pts',(0.479571028525578,1.,-3.92914297392071));
#53623=CARTESIAN_POINT('Ctrl Pts',(0.478062927140964,1.,-3.93655660689819));
#53624=CARTESIAN_POINT('Ctrl Pts',(0.476507810658537,1.,-3.94396469119383));
#53625=CARTESIAN_POINT('Ctrl Pts',(0.47490705302179,1.,-3.95137192932897));
#53626=CARTESIAN_POINT('Ctrl Pts',(0.473261847236297,1.,-3.95878201038338));
#53627=CARTESIAN_POINT('Ctrl Pts',(0.471572978413503,1.,-3.96619600864643));
#53628=CARTESIAN_POINT('Ctrl Pts',(0.469840942829895,1.,-3.97361320212436));
#53629=CARTESIAN_POINT('Ctrl Pts',(0.468066047920157,1.,-3.98103175589371));
#53630=CARTESIAN_POINT('Ctrl Pts',(0.466248520883039,1.,-3.98844946363262));
#53631=CARTESIAN_POINT('Ctrl Pts',(0.464388610938975,1.,-3.9958644432011));
#53632=CARTESIAN_POINT('Ctrl Pts',(0.462486702616204,1.,-4.00327590659075));
#53633=CARTESIAN_POINT('Ctrl Pts',(0.460543280768514,1.,-4.01068390573399));
#53634=CARTESIAN_POINT('Ctrl Pts',(0.458558885636945,1.,-4.01808900827587));
#53635=CARTESIAN_POINT('Ctrl Pts',(0.45653407078495,1.,-4.02549199038394));
#53636=CARTESIAN_POINT('Ctrl Pts',(0.454469363020541,1.,-4.03289354362794));
#53637=CARTESIAN_POINT('Ctrl Pts',(0.452365214748892,1.,-4.04029392228049));
#53638=CARTESIAN_POINT('Ctrl Pts',(0.450222009543926,1.,-4.0476929901813));
#53639=CARTESIAN_POINT('Ctrl Pts',(0.448040082684114,1.,-4.0550903779696));
#53640=CARTESIAN_POINT('Ctrl Pts',(0.445819737468537,1.,-4.06248560760659));
#53641=CARTESIAN_POINT('Ctrl Pts',(0.443561262395332,1.,-4.0698782192569));
#53642=CARTESIAN_POINT('Ctrl Pts',(0.44126495139636,1.,-4.07726792490016));
#53643=CARTESIAN_POINT('Ctrl Pts',(0.438931108931279,1.,-4.08465462294273));
#53644=CARTESIAN_POINT('Ctrl Pts',(0.436560044913482,1.,-4.09203832139089));
#53645=CARTESIAN_POINT('Ctrl Pts',(0.43415207320046,1.,-4.09941908688373));
#53646=CARTESIAN_POINT('Ctrl Pts',(0.431707508679883,1.,-4.10679698750336));
#53647=CARTESIAN_POINT('Ctrl Pts',(0.429226666075844,1.,-4.11417202783267));
#53648=CARTESIAN_POINT('Ctrl Pts',(0.426709855707,1.,-4.12154412502007));
#53649=CARTESIAN_POINT('Ctrl Pts',(0.424157375323975,1.,-4.12891314634572));
#53650=CARTESIAN_POINT('Ctrl Pts',(0.421569503104512,1.,-4.13627893207002));
#53651=CARTESIAN_POINT('Ctrl Pts',(0.418946490667702,1.,-4.14364132317121));
#53652=CARTESIAN_POINT('Ctrl Pts',(0.416288556008011,1.,-4.15100018949965));
#53653=CARTESIAN_POINT('Ctrl Pts',(0.41359587795147,1.,-4.15835545017202));
#53654=CARTESIAN_POINT('Ctrl Pts',(0.410868596146414,1.,-4.16570705938425));
#53655=CARTESIAN_POINT('Ctrl Pts',(0.408659167568273,1.,-4.17158541007977));
#53656=CARTESIAN_POINT('Ctrl Pts',(0.406986596325454,1.,-4.17599251954382));
#53657=CARTESIAN_POINT('Ctrl Pts',(0.405864662679209,1.,-4.17892985789466));
#53658=CARTESIAN_POINT('Ctrl Pts',(0.40530197431835,1.,-4.18039834341342));
#53659=CARTESIAN_POINT('Origin',(0.40530197431835,0.,-4.18039834341342));
#53660=CARTESIAN_POINT('',(0.253646344052522,1.,-4.1923339003649));
#53661=CARTESIAN_POINT('Origin',(0.,0.,0.));
#53662=CARTESIAN_POINT('',(0.67659164797366,1.,-3.68845817949618));
#53663=CARTESIAN_POINT('Origin',(0.,1.,0.));
#53664=CARTESIAN_POINT('Ctrl Pts',(0.67659164797366,1.,-3.68845817949618));
#53665=CARTESIAN_POINT('Ctrl Pts',(0.67659164797366,0.666666666666667,-3.68845817949618));
#53666=CARTESIAN_POINT('Ctrl Pts',(0.67659164797366,0.333333333333333,-3.68845817949618));
#53667=CARTESIAN_POINT('Ctrl Pts',(0.67659164797366,-0.333333333333333,
-3.68845817949618));
#53668=CARTESIAN_POINT('Ctrl Pts',(0.676591647973661,-0.666666666666667,
-3.68845817949618));
#53669=CARTESIAN_POINT('Ctrl Pts',(0.676591647973661,-1.,-3.68845817949618));
#53670=CARTESIAN_POINT('Ctrl Pts',(0.906349047628866,-1.,-4.10104028313088));
#53671=CARTESIAN_POINT('Ctrl Pts',(0.906349047628866,1.,-4.10104028313088));
#53672=CARTESIAN_POINT('Ctrl Pts',(0.905360112216302,-1.,-4.09981755067956));
#53673=CARTESIAN_POINT('Ctrl Pts',(0.905360112216302,1.,-4.09981755067956));
#53674=CARTESIAN_POINT('Ctrl Pts',(0.903385402444212,-1.,-4.09737067247114));
#53675=CARTESIAN_POINT('Ctrl Pts',(0.903385402444212,1.,-4.09737067247114));
#53676=CARTESIAN_POINT('Ctrl Pts',(0.900432820945975,-1.,-4.09369611524319));
#53677=CARTESIAN_POINT('Ctrl Pts',(0.900432820945975,1.,-4.09369611524319));
#53678=CARTESIAN_POINT('Ctrl Pts',(0.896515019236368,-1.,-4.08878822249095));
#53679=CARTESIAN_POINT('Ctrl Pts',(0.896515019236368,1.,-4.08878822249095));
#53680=CARTESIAN_POINT('Ctrl Pts',(0.891649447920401,-1.,-4.08263920306651));
#53681=CARTESIAN_POINT('Ctrl Pts',(0.891649447920401,1.,-4.08263920306651));
#53682=CARTESIAN_POINT('Ctrl Pts',(0.886815658360739,-1.,-4.07647601774639));
#53683=CARTESIAN_POINT('Ctrl Pts',(0.886815658360739,1.,-4.07647601774639));
#53684=CARTESIAN_POINT('Ctrl Pts',(0.882013797525916,-1.,-4.07029866694292));
#53685=CARTESIAN_POINT('Ctrl Pts',(0.882013797525916,1.,-4.07029866694292));
#53686=CARTESIAN_POINT('Ctrl Pts',(0.877244060484595,-1.,-4.06410717232347));
#53687=CARTESIAN_POINT('Ctrl Pts',(0.877244060484595,1.,-4.06410717232347));
#53688=CARTESIAN_POINT('Ctrl Pts',(0.872506694780563,-1.,-4.05790159030495));
#53689=CARTESIAN_POINT('Ctrl Pts',(0.872506694780563,1.,-4.05790159030495));
#53690=CARTESIAN_POINT('Ctrl Pts',(0.867801988858176,-1.,-4.05168199437128));
#53691=CARTESIAN_POINT('Ctrl Pts',(0.867801988858176,1.,-4.05168199437128));
#53692=CARTESIAN_POINT('Ctrl Pts',(0.863130256642173,-1.,-4.04544845048097));
#53693=CARTESIAN_POINT('Ctrl Pts',(0.863130256642173,1.,-4.04544845048097));
#53694=CARTESIAN_POINT('Ctrl Pts',(0.858491822322571,-1.,-4.03920099284658));
#53695=CARTESIAN_POINT('Ctrl Pts',(0.858491822322571,1.,-4.03920099284658));
#53696=CARTESIAN_POINT('Ctrl Pts',(0.853887006632178,-1.,-4.03293960436946));
#53697=CARTESIAN_POINT('Ctrl Pts',(0.853887006632178,1.,-4.03293960436946));
#53698=CARTESIAN_POINT('Ctrl Pts',(0.849316107475012,-1.,-4.02666418343508));
#53699=CARTESIAN_POINT('Ctrl Pts',(0.849316107475012,1.,-4.02666418343508));
#53700=CARTESIAN_POINT('Ctrl Pts',(0.844779403288517,-1.,-4.02037456798787));
#53701=CARTESIAN_POINT('Ctrl Pts',(0.844779403288517,1.,-4.02037456798787));
#53702=CARTESIAN_POINT('Ctrl Pts',(0.84027717197638,-1.,-4.01407059766338));
#53703=CARTESIAN_POINT('Ctrl Pts',(0.84027717197638,1.,-4.01407059766338));
#53704=CARTESIAN_POINT('Ctrl Pts',(0.835809705809821,-1.,-4.00775216907934));
#53705=CARTESIAN_POINT('Ctrl Pts',(0.835809705809821,1.,-4.00775216907934));
#53706=CARTESIAN_POINT('Ctrl Pts',(0.831377325741487,-1.,-4.00141928477447));
#53707=CARTESIAN_POINT('Ctrl Pts',(0.831377325741487,1.,-4.00141928477447));
#53708=CARTESIAN_POINT('Ctrl Pts',(0.826980400320473,-1.,-3.99507212784289));
#53709=CARTESIAN_POINT('Ctrl Pts',(0.826980400320473,1.,-3.99507212784289));
#53710=CARTESIAN_POINT('Ctrl Pts',(0.822619346021769,-1.,-3.98871104646328));
#53711=CARTESIAN_POINT('Ctrl Pts',(0.822619346021769,1.,-3.98871104646328));
#53712=CARTESIAN_POINT('Ctrl Pts',(0.818294599022033,-1.,-3.98233640155287));
#53713=CARTESIAN_POINT('Ctrl Pts',(0.818294599022033,1.,-3.98233640155287));
#53714=CARTESIAN_POINT('Ctrl Pts',(0.814006592328737,-1.,-3.97594844078763));
#53715=CARTESIAN_POINT('Ctrl Pts',(0.814006592328737,1.,-3.97594844078763));
#53716=CARTESIAN_POINT('Ctrl Pts',(0.809755732818134,-1.,-3.96954717513251));
#53717=CARTESIAN_POINT('Ctrl Pts',(0.809755732818134,1.,-3.96954717513251));
#53718=CARTESIAN_POINT('Ctrl Pts',(0.805542372178495,-1.,-3.96313222295874));
#53719=CARTESIAN_POINT('Ctrl Pts',(0.805542372178495,1.,-3.96313222295874));
#53720=CARTESIAN_POINT('Ctrl Pts',(0.801366797727206,-1.,-3.95670276375176));
#53721=CARTESIAN_POINT('Ctrl Pts',(0.801366797727206,1.,-3.95670276375176));
#53722=CARTESIAN_POINT('Ctrl Pts',(0.797229296085438,-1.,-3.95025788827189));
#53723=CARTESIAN_POINT('Ctrl Pts',(0.797229296085438,1.,-3.95025788827189));
#53724=CARTESIAN_POINT('Ctrl Pts',(0.793130205641017,-1.,-3.94379688971307));
#53725=CARTESIAN_POINT('Ctrl Pts',(0.793130205641017,1.,-3.94379688971307));
#53726=CARTESIAN_POINT('Ctrl Pts',(0.789069971469323,-1.,-3.93731956885671));
#53727=CARTESIAN_POINT('Ctrl Pts',(0.789069971469323,1.,-3.93731956885671));
#53728=CARTESIAN_POINT('Ctrl Pts',(0.785049202786458,-1.,-3.93082655631769));
#53729=CARTESIAN_POINT('Ctrl Pts',(0.785049202786458,1.,-3.93082655631769));
#53730=CARTESIAN_POINT('Ctrl Pts',(0.781068718228395,-1.,-3.92431956510418));
#53731=CARTESIAN_POINT('Ctrl Pts',(0.781068718228395,1.,-3.92431956510418));
#53732=CARTESIAN_POINT('Ctrl Pts',(0.777129415664915,-1.,-3.91780062334464));
#53733=CARTESIAN_POINT('Ctrl Pts',(0.777129415664915,1.,-3.91780062334464));
#53734=CARTESIAN_POINT('Ctrl Pts',(0.773232154506305,-1.,-3.91127138115238));
#53735=CARTESIAN_POINT('Ctrl Pts',(0.773232154506305,1.,-3.91127138115238));
#53736=CARTESIAN_POINT('Ctrl Pts',(0.769377629847876,-1.,-3.90473237182634));
#53737=CARTESIAN_POINT('Ctrl Pts',(0.769377629847876,1.,-3.90473237182634));
#53738=CARTESIAN_POINT('Ctrl Pts',(0.765566256401306,-1.,-3.89818233104381));
#53739=CARTESIAN_POINT('Ctrl Pts',(0.765566256401306,1.,-3.89818233104381));
#53740=CARTESIAN_POINT('Ctrl Pts',(0.761798028793978,-1.,-3.89161738162245));
#53741=CARTESIAN_POINT('Ctrl Pts',(0.761798028793978,1.,-3.89161738162245));
#53742=CARTESIAN_POINT('Ctrl Pts',(0.758072800564798,-1.,-3.88503262662684));
#53743=CARTESIAN_POINT('Ctrl Pts',(0.758072800564798,1.,-3.88503262662684));
#53744=CARTESIAN_POINT('Ctrl Pts',(0.754390577396846,-1.,-3.87842382520058));
#53745=CARTESIAN_POINT('Ctrl Pts',(0.754390577396846,1.,-3.87842382520058));
#53746=CARTESIAN_POINT('Ctrl Pts',(0.750751822383023,-1.,-3.87178914078372));
#53747=CARTESIAN_POINT('Ctrl Pts',(0.750751822383023,1.,-3.87178914078372));
#53748=CARTESIAN_POINT('Ctrl Pts',(0.747157716488884,-1.,-3.86513062969896));
#53749=CARTESIAN_POINT('Ctrl Pts',(0.747157716488884,1.,-3.86513062969896));
#53750=CARTESIAN_POINT('Ctrl Pts',(0.743610542737041,-1.,-3.85845645217611));
#53751=CARTESIAN_POINT('Ctrl Pts',(0.743610542737041,1.,-3.85845645217611));
#53752=CARTESIAN_POINT('Ctrl Pts',(0.740113146827176,-1.,-3.85177770351237));
#53753=CARTESIAN_POINT('Ctrl Pts',(0.740113146827176,1.,-3.85177770351237));
#53754=CARTESIAN_POINT('Ctrl Pts',(0.736668240497151,-1.,-3.84510432881231));
#53755=CARTESIAN_POINT('Ctrl Pts',(0.736668240497151,1.,-3.84510432881231));
#53756=CARTESIAN_POINT('Ctrl Pts',(0.73327770375609,-1.,-3.83844103658016));
#53757=CARTESIAN_POINT('Ctrl Pts',(0.73327770375609,1.,-3.83844103658016));
#53758=CARTESIAN_POINT('Ctrl Pts',(0.729942010490145,-1.,-3.83178392403371));
#53759=CARTESIAN_POINT('Ctrl Pts',(0.729942010490145,1.,-3.83178392403371));
#53760=CARTESIAN_POINT('Ctrl Pts',(0.726659281876608,-1.,-3.82511495756682));
#53761=CARTESIAN_POINT('Ctrl Pts',(0.726659281876608,1.,-3.82511495756682));
#53762=CARTESIAN_POINT('Ctrl Pts',(0.723426346019349,-1.,-3.81840802610795));
#53763=CARTESIAN_POINT('Ctrl Pts',(0.723426346019349,1.,-3.81840802610795));
#53764=CARTESIAN_POINT('Ctrl Pts',(0.720240466589172,-1.,-3.81163885127309));
#53765=CARTESIAN_POINT('Ctrl Pts',(0.720240466589172,1.,-3.81163885127309));
#53766=CARTESIAN_POINT('Ctrl Pts',(0.717100993669091,-1.,-3.80479445759296));
#53767=CARTESIAN_POINT('Ctrl Pts',(0.717100993669091,1.,-3.80479445759296));
#53768=CARTESIAN_POINT('Ctrl Pts',(0.714010733006677,-1.,-3.79788100314994));
#53769=CARTESIAN_POINT('Ctrl Pts',(0.714010733006677,1.,-3.79788100314994));
#53770=CARTESIAN_POINT('Ctrl Pts',(0.710978231689117,-1.,-3.79093694007146));
#53771=CARTESIAN_POINT('Ctrl Pts',(0.710978231689117,1.,-3.79093694007146));
#53772=CARTESIAN_POINT('Ctrl Pts',(0.7080158793756,-1.,-3.78402183336678));
#53773=CARTESIAN_POINT('Ctrl Pts',(0.7080158793756,1.,-3.78402183336678));
#53774=CARTESIAN_POINT('Ctrl Pts',(0.705135847999949,-1.,-3.77719254217197));
#53775=CARTESIAN_POINT('Ctrl Pts',(0.705135847999949,1.,-3.77719254217197));
#53776=CARTESIAN_POINT('Ctrl Pts',(0.702346356621613,-1.,-3.77048141872904));
#53777=CARTESIAN_POINT('Ctrl Pts',(0.702346356621613,1.,-3.77048141872904));
#53778=CARTESIAN_POINT('Ctrl Pts',(0.699648552230851,-1.,-3.76387780603725));
#53779=CARTESIAN_POINT('Ctrl Pts',(0.699648552230851,1.,-3.76387780603725));
#53780=CARTESIAN_POINT('Ctrl Pts',(0.69703124565953,-1.,-3.75729775766913));
#53781=CARTESIAN_POINT('Ctrl Pts',(0.69703124565953,1.,-3.75729775766913));
#53782=CARTESIAN_POINT('Ctrl Pts',(0.694474562581173,-1.,-3.7506028824329));
#53783=CARTESIAN_POINT('Ctrl Pts',(0.694474562581173,1.,-3.7506028824329));
#53784=CARTESIAN_POINT('Ctrl Pts',(0.691960080400503,-1.,-3.74365508986548));
#53785=CARTESIAN_POINT('Ctrl Pts',(0.691960080400503,1.,-3.74365508986548));
#53786=CARTESIAN_POINT('Ctrl Pts',(0.689479637354651,-1.,-3.73636374474993));
#53787=CARTESIAN_POINT('Ctrl Pts',(0.689479637354651,1.,-3.73636374474993));
#53788=CARTESIAN_POINT('Ctrl Pts',(0.687043475232499,-1.,-3.72872973554125));
#53789=CARTESIAN_POINT('Ctrl Pts',(0.687043475232499,1.,-3.72872973554125));
#53790=CARTESIAN_POINT('Ctrl Pts',(0.684691698168355,-1.,-3.7209063713952));
#53791=CARTESIAN_POINT('Ctrl Pts',(0.684691698168355,1.,-3.7209063713952));
#53792=CARTESIAN_POINT('Ctrl Pts',(0.682492345109689,-1.,-3.71319182790334));
#53793=CARTESIAN_POINT('Ctrl Pts',(0.682492345109689,1.,-3.71319182790334));
#53794=CARTESIAN_POINT('Ctrl Pts',(0.680526909711617,-1.,-3.70595722032165));
#53795=CARTESIAN_POINT('Ctrl Pts',(0.680526909711617,1.,-3.70595722032165));
#53796=CARTESIAN_POINT('Ctrl Pts',(0.678878822226389,-1.,-3.69959004073192));
#53797=CARTESIAN_POINT('Ctrl Pts',(0.678878822226389,1.,-3.69959004073192));
#53798=CARTESIAN_POINT('Ctrl Pts',(0.677621861865196,-1.,-3.69443683573443));
#53799=CARTESIAN_POINT('Ctrl Pts',(0.677621861865196,1.,-3.69443683573443));
#53800=CARTESIAN_POINT('Ctrl Pts',(0.67680581107414,-1.,-3.69073278191505));
#53801=CARTESIAN_POINT('Ctrl Pts',(0.67680581107414,1.,-3.69073278191505));
#53802=CARTESIAN_POINT('Ctrl Pts',(0.676524321060166,-1.,-3.68901718135636));
#53803=CARTESIAN_POINT('Ctrl Pts',(0.676524321060166,1.,-3.68901718135636));
#53804=CARTESIAN_POINT('Ctrl Pts',(0.676525601650139,-1.,-3.68844918120934));
#53805=CARTESIAN_POINT('Ctrl Pts',(0.676525601650139,1.,-3.68844918120934));
#53806=CARTESIAN_POINT('Ctrl Pts',(0.676620796001716,-1.,-3.68838970675356));
#53807=CARTESIAN_POINT('Ctrl Pts',(0.676620796001716,1.,-3.68838970675356));
#53808=CARTESIAN_POINT('Ctrl Pts',(0.676691979611562,-1.,-3.68843977377012));
#53809=CARTESIAN_POINT('Ctrl Pts',(0.676691979611562,1.,-3.68843977377012));
#53810=CARTESIAN_POINT('',(0.906349047628866,1.,-4.10104028313088));
#53811=CARTESIAN_POINT('Ctrl Pts',(0.906349047628866,1.,-4.10104028313088));
#53812=CARTESIAN_POINT('Ctrl Pts',(0.905360112216302,1.,-4.09981755067956));
#53813=CARTESIAN_POINT('Ctrl Pts',(0.903385402444212,1.,-4.09737067247114));
#53814=CARTESIAN_POINT('Ctrl Pts',(0.900432820945975,1.,-4.09369611524319));
#53815=CARTESIAN_POINT('Ctrl Pts',(0.896515019236368,1.,-4.08878822249095));
#53816=CARTESIAN_POINT('Ctrl Pts',(0.891649447920401,1.,-4.08263920306651));
#53817=CARTESIAN_POINT('Ctrl Pts',(0.886815658360739,1.,-4.07647601774639));
#53818=CARTESIAN_POINT('Ctrl Pts',(0.882013797525916,1.,-4.07029866694292));
#53819=CARTESIAN_POINT('Ctrl Pts',(0.877244060484595,1.,-4.06410717232347));
#53820=CARTESIAN_POINT('Ctrl Pts',(0.872506694780563,1.,-4.05790159030495));
#53821=CARTESIAN_POINT('Ctrl Pts',(0.867801988858176,1.,-4.05168199437128));
#53822=CARTESIAN_POINT('Ctrl Pts',(0.863130256642173,1.,-4.04544845048097));
#53823=CARTESIAN_POINT('Ctrl Pts',(0.858491822322571,1.,-4.03920099284658));
#53824=CARTESIAN_POINT('Ctrl Pts',(0.853887006632178,1.,-4.03293960436946));
#53825=CARTESIAN_POINT('Ctrl Pts',(0.849316107475012,1.,-4.02666418343508));
#53826=CARTESIAN_POINT('Ctrl Pts',(0.844779403288517,1.,-4.02037456798787));
#53827=CARTESIAN_POINT('Ctrl Pts',(0.84027717197638,1.,-4.01407059766338));
#53828=CARTESIAN_POINT('Ctrl Pts',(0.835809705809821,1.,-4.00775216907934));
#53829=CARTESIAN_POINT('Ctrl Pts',(0.831377325741487,1.,-4.00141928477447));
#53830=CARTESIAN_POINT('Ctrl Pts',(0.826980400320473,1.,-3.99507212784289));
#53831=CARTESIAN_POINT('Ctrl Pts',(0.822619346021769,1.,-3.98871104646328));
#53832=CARTESIAN_POINT('Ctrl Pts',(0.818294599022033,1.,-3.98233640155287));
#53833=CARTESIAN_POINT('Ctrl Pts',(0.814006592328737,1.,-3.97594844078763));
#53834=CARTESIAN_POINT('Ctrl Pts',(0.809755732818134,1.,-3.96954717513251));
#53835=CARTESIAN_POINT('Ctrl Pts',(0.805542372178495,1.,-3.96313222295874));
#53836=CARTESIAN_POINT('Ctrl Pts',(0.801366797727206,1.,-3.95670276375176));
#53837=CARTESIAN_POINT('Ctrl Pts',(0.797229296085438,1.,-3.95025788827189));
#53838=CARTESIAN_POINT('Ctrl Pts',(0.793130205641017,1.,-3.94379688971307));
#53839=CARTESIAN_POINT('Ctrl Pts',(0.789069971469323,1.,-3.93731956885671));
#53840=CARTESIAN_POINT('Ctrl Pts',(0.785049202786458,1.,-3.93082655631769));
#53841=CARTESIAN_POINT('Ctrl Pts',(0.781068718228395,1.,-3.92431956510418));
#53842=CARTESIAN_POINT('Ctrl Pts',(0.777129415664915,1.,-3.91780062334464));
#53843=CARTESIAN_POINT('Ctrl Pts',(0.773232154506305,1.,-3.91127138115238));
#53844=CARTESIAN_POINT('Ctrl Pts',(0.769377629847876,1.,-3.90473237182634));
#53845=CARTESIAN_POINT('Ctrl Pts',(0.765566256401306,1.,-3.89818233104381));
#53846=CARTESIAN_POINT('Ctrl Pts',(0.761798028793978,1.,-3.89161738162245));
#53847=CARTESIAN_POINT('Ctrl Pts',(0.758072800564798,1.,-3.88503262662684));
#53848=CARTESIAN_POINT('Ctrl Pts',(0.754390577396846,1.,-3.87842382520058));
#53849=CARTESIAN_POINT('Ctrl Pts',(0.750751822383023,1.,-3.87178914078372));
#53850=CARTESIAN_POINT('Ctrl Pts',(0.747157716488884,1.,-3.86513062969896));
#53851=CARTESIAN_POINT('Ctrl Pts',(0.743610542737041,1.,-3.85845645217611));
#53852=CARTESIAN_POINT('Ctrl Pts',(0.740113146827176,1.,-3.85177770351237));
#53853=CARTESIAN_POINT('Ctrl Pts',(0.736668240497151,1.,-3.84510432881231));
#53854=CARTESIAN_POINT('Ctrl Pts',(0.73327770375609,1.,-3.83844103658016));
#53855=CARTESIAN_POINT('Ctrl Pts',(0.729942010490145,1.,-3.83178392403371));
#53856=CARTESIAN_POINT('Ctrl Pts',(0.726659281876608,1.,-3.82511495756682));
#53857=CARTESIAN_POINT('Ctrl Pts',(0.723426346019349,1.,-3.81840802610795));
#53858=CARTESIAN_POINT('Ctrl Pts',(0.720240466589172,1.,-3.81163885127309));
#53859=CARTESIAN_POINT('Ctrl Pts',(0.717100993669091,1.,-3.80479445759296));
#53860=CARTESIAN_POINT('Ctrl Pts',(0.714010733006677,1.,-3.79788100314994));
#53861=CARTESIAN_POINT('Ctrl Pts',(0.710978231689117,1.,-3.79093694007146));
#53862=CARTESIAN_POINT('Ctrl Pts',(0.7080158793756,1.,-3.78402183336678));
#53863=CARTESIAN_POINT('Ctrl Pts',(0.705135847999949,1.,-3.77719254217197));
#53864=CARTESIAN_POINT('Ctrl Pts',(0.702346356621613,1.,-3.77048141872904));
#53865=CARTESIAN_POINT('Ctrl Pts',(0.699648552230851,1.,-3.76387780603725));
#53866=CARTESIAN_POINT('Ctrl Pts',(0.69703124565953,1.,-3.75729775766913));
#53867=CARTESIAN_POINT('Ctrl Pts',(0.694474562581173,1.,-3.7506028824329));
#53868=CARTESIAN_POINT('Ctrl Pts',(0.691960080400503,1.,-3.74365508986548));
#53869=CARTESIAN_POINT('Ctrl Pts',(0.689479637354651,1.,-3.73636374474993));
#53870=CARTESIAN_POINT('Ctrl Pts',(0.687043475232499,1.,-3.72872973554125));
#53871=CARTESIAN_POINT('Ctrl Pts',(0.684691698168355,1.,-3.7209063713952));
#53872=CARTESIAN_POINT('Ctrl Pts',(0.682492345109689,1.,-3.71319182790334));
#53873=CARTESIAN_POINT('Ctrl Pts',(0.680526909711617,1.,-3.70595722032165));
#53874=CARTESIAN_POINT('Ctrl Pts',(0.678878822226389,1.,-3.69959004073192));
#53875=CARTESIAN_POINT('Ctrl Pts',(0.677621861865196,1.,-3.69443683573443));
#53876=CARTESIAN_POINT('Ctrl Pts',(0.676867042599711,1.,-3.6910107117555));
#53877=CARTESIAN_POINT('Ctrl Pts',(0.676580391119535,1.,-3.68934997767391));
#53878=CARTESIAN_POINT('Ctrl Pts',(0.676535079520365,1.,-3.68869596426099));
#53879=CARTESIAN_POINT('Ctrl Pts',(0.67656928609342,1.,-3.68850172300543));
#53880=CARTESIAN_POINT('Ctrl Pts',(0.676591647973661,1.,-3.68845817949618));
#53881=CARTESIAN_POINT('',(0.906349047628866,0.,-4.10104028313088));
#53882=CARTESIAN_POINT('Ctrl Pts',(1.07157964745328,-1.,-3.59363563249864));
#53883=CARTESIAN_POINT('Ctrl Pts',(1.07157964745328,1.,-3.59363563249864));
#53884=CARTESIAN_POINT('Ctrl Pts',(1.07162034256459,-1.,-3.59355870577901));
#53885=CARTESIAN_POINT('Ctrl Pts',(1.07162034256459,1.,-3.59355870577901));
#53886=CARTESIAN_POINT('Ctrl Pts',(1.07173216219145,-1.,-3.59356848057812));
#53887=CARTESIAN_POINT('Ctrl Pts',(1.07173216219145,1.,-3.59356848057812));
#53888=CARTESIAN_POINT('Ctrl Pts',(1.07199116987656,-1.,-3.5940739910409));
#53889=CARTESIAN_POINT('Ctrl Pts',(1.07199116987656,1.,-3.5940739910409));
#53890=CARTESIAN_POINT('Ctrl Pts',(1.07251922679245,-1.,-3.59573039612316));
#53891=CARTESIAN_POINT('Ctrl Pts',(1.07251922679245,1.,-3.59573039612316));
#53892=CARTESIAN_POINT('Ctrl Pts',(1.07347372545714,-1.,-3.59940121154535));
#53893=CARTESIAN_POINT('Ctrl Pts',(1.07347372545714,1.,-3.59940121154535));
#53894=CARTESIAN_POINT('Ctrl Pts',(1.07469327168578,-1.,-3.60456339887778));
#53895=CARTESIAN_POINT('Ctrl Pts',(1.07469327168578,1.,-3.60456339887778));
#53896=CARTESIAN_POINT('Ctrl Pts',(1.07611545402734,-1.,-3.61098481349204));
#53897=CARTESIAN_POINT('Ctrl Pts',(1.07611545402734,1.,-3.61098481349204));
#53898=CARTESIAN_POINT('Ctrl Pts',(1.07764868137619,-1.,-3.61832318504575));
#53899=CARTESIAN_POINT('Ctrl Pts',(1.07764868137619,1.,-3.61832318504575));
#53900=CARTESIAN_POINT('Ctrl Pts',(1.07919137290742,-1.,-3.62619537902361));
#53901=CARTESIAN_POINT('Ctrl Pts',(1.07919137290742,1.,-3.62619537902361));
#53902=CARTESIAN_POINT('Ctrl Pts',(1.08064765719867,-1.,-3.63423373196529));
#53903=CARTESIAN_POINT('Ctrl Pts',(1.08064765719867,1.,-3.63423373196529));
#53904=CARTESIAN_POINT('Ctrl Pts',(1.08194278850996,-1.,-3.64214167843677));
#53905=CARTESIAN_POINT('Ctrl Pts',(1.08194278850996,1.,-3.64214167843677));
#53906=CARTESIAN_POINT('Ctrl Pts',(1.08304289898623,-1.,-3.64976441208358));
#53907=CARTESIAN_POINT('Ctrl Pts',(1.08304289898623,1.,-3.64976441208358));
#53908=CARTESIAN_POINT('Ctrl Pts',(1.08395671077807,-1.,-3.65709649161166));
#53909=CARTESIAN_POINT('Ctrl Pts',(1.08395671077807,1.,-3.65709649161166));
#53910=CARTESIAN_POINT('Ctrl Pts',(1.08471809922901,-1.,-3.66422237895365));
#53911=CARTESIAN_POINT('Ctrl Pts',(1.08471809922901,1.,-3.66422237895365));
#53912=CARTESIAN_POINT('Ctrl Pts',(1.0853733414449,-1.,-3.67127347729666));
#53913=CARTESIAN_POINT('Ctrl Pts',(1.0853733414449,1.,-3.67127347729666));
#53914=CARTESIAN_POINT('Ctrl Pts',(1.0859675575576,-1.,-3.67838211685118));
#53915=CARTESIAN_POINT('Ctrl Pts',(1.0859675575576,1.,-3.67838211685118));
#53916=CARTESIAN_POINT('Ctrl Pts',(1.0865288888259,-1.,-3.68562817420797));
#53917=CARTESIAN_POINT('Ctrl Pts',(1.0865288888259,1.,-3.68562817420797));
#53918=CARTESIAN_POINT('Ctrl Pts',(1.08706319540271,-1.,-3.69302062410157));
#53919=CARTESIAN_POINT('Ctrl Pts',(1.08706319540271,1.,-3.69302062410157));
#53920=CARTESIAN_POINT('Ctrl Pts',(1.08756311291309,-1.,-3.70052690909833));
#53921=CARTESIAN_POINT('Ctrl Pts',(1.08756311291309,1.,-3.70052690909833));
#53922=CARTESIAN_POINT('Ctrl Pts',(1.08801367312185,-1.,-3.70809084139457));
#53923=CARTESIAN_POINT('Ctrl Pts',(1.08801367312185,1.,-3.70809084139457));
#53924=CARTESIAN_POINT('Ctrl Pts',(1.0883988733478,-1.,-3.71565372339075));
#53925=CARTESIAN_POINT('Ctrl Pts',(1.0883988733478,1.,-3.71565372339075));
#53926=CARTESIAN_POINT('Ctrl Pts',(1.08870887220082,-1.,-3.72317741369398));
#53927=CARTESIAN_POINT('Ctrl Pts',(1.08870887220082,1.,-3.72317741369398));
#53928=CARTESIAN_POINT('Ctrl Pts',(1.08894337390937,-1.,-3.73065515162988));
#53929=CARTESIAN_POINT('Ctrl Pts',(1.08894337390937,1.,-3.73065515162988));
#53930=CARTESIAN_POINT('Ctrl Pts',(1.08910769013297,-1.,-3.73809879348239));
#53931=CARTESIAN_POINT('Ctrl Pts',(1.08910769013297,1.,-3.73809879348239));
#53932=CARTESIAN_POINT('Ctrl Pts',(1.08921040494017,-1.,-3.74553121371757));
#53933=CARTESIAN_POINT('Ctrl Pts',(1.08921040494017,1.,-3.74553121371757));
#53934=CARTESIAN_POINT('Ctrl Pts',(1.08926054632925,-1.,-3.75297711748132));
#53935=CARTESIAN_POINT('Ctrl Pts',(1.08926054632925,1.,-3.75297711748132));
#53936=CARTESIAN_POINT('Ctrl Pts',(1.08926462734281,-1.,-3.76045342580208));
#53937=CARTESIAN_POINT('Ctrl Pts',(1.08926462734281,1.,-3.76045342580208));
#53938=CARTESIAN_POINT('Ctrl Pts',(1.08922484204256,-1.,-3.76796340094448));
#53939=CARTESIAN_POINT('Ctrl Pts',(1.08922484204256,1.,-3.76796340094448));
#53940=CARTESIAN_POINT('Ctrl Pts',(1.0891407279127,-1.,-3.77550199409424));
#53941=CARTESIAN_POINT('Ctrl Pts',(1.0891407279127,1.,-3.77550199409424));
#53942=CARTESIAN_POINT('Ctrl Pts',(1.08901018614636,-1.,-3.78305911299504));
#53943=CARTESIAN_POINT('Ctrl Pts',(1.08901018614636,1.,-3.78305911299504));
#53944=CARTESIAN_POINT('Ctrl Pts',(1.08883071512098,-1.,-3.79062357974404));
#53945=CARTESIAN_POINT('Ctrl Pts',(1.08883071512098,1.,-3.79062357974404));
#53946=CARTESIAN_POINT('Ctrl Pts',(1.08860064435778,-1.,-3.79818708705259));
#53947=CARTESIAN_POINT('Ctrl Pts',(1.08860064435778,1.,-3.79818708705259));
#53948=CARTESIAN_POINT('Ctrl Pts',(1.0883200925538,-1.,-3.8057472665766));
#53949=CARTESIAN_POINT('Ctrl Pts',(1.0883200925538,1.,-3.8057472665766));
#53950=CARTESIAN_POINT('Ctrl Pts',(1.08799030610862,-1.,-3.81330554446323));
#53951=CARTESIAN_POINT('Ctrl Pts',(1.08799030610862,1.,-3.81330554446323));
#53952=CARTESIAN_POINT('Ctrl Pts',(1.08761321539442,-1.,-3.82086569676319));
#53953=CARTESIAN_POINT('Ctrl Pts',(1.08761321539442,1.,-3.82086569676319));
#53954=CARTESIAN_POINT('Ctrl Pts',(1.08719091307558,-1.,-3.82843215316984));
#53955=CARTESIAN_POINT('Ctrl Pts',(1.08719091307558,1.,-3.82843215316984));
#53956=CARTESIAN_POINT('Ctrl Pts',(1.08672515456902,-1.,-3.83600837071708));
#53957=CARTESIAN_POINT('Ctrl Pts',(1.08672515456902,1.,-3.83600837071708));
#53958=CARTESIAN_POINT('Ctrl Pts',(1.08621688337604,-1.,-3.8435952876495));
#53959=CARTESIAN_POINT('Ctrl Pts',(1.08621688337604,1.,-3.8435952876495));
#53960=CARTESIAN_POINT('Ctrl Pts',(1.08566647671844,-1.,-3.85119211322755));
#53961=CARTESIAN_POINT('Ctrl Pts',(1.08566647671844,1.,-3.85119211322755));
#53962=CARTESIAN_POINT('Ctrl Pts',(1.08507395120059,-1.,-3.85879698702532));
#53963=CARTESIAN_POINT('Ctrl Pts',(1.08507395120059,1.,-3.85879698702532));
#53964=CARTESIAN_POINT('Ctrl Pts',(1.08443918607927,-1.,-3.86640769434274));
#53965=CARTESIAN_POINT('Ctrl Pts',(1.08443918607927,1.,-3.86640769434274));
#53966=CARTESIAN_POINT('Ctrl Pts',(1.08376213307504,-1.,-3.8740223372254));
#53967=CARTESIAN_POINT('Ctrl Pts',(1.08376213307504,1.,-3.8740223372254));
#53968=CARTESIAN_POINT('Ctrl Pts',(1.08304304871028,-1.,-3.88164007721313));
#53969=CARTESIAN_POINT('Ctrl Pts',(1.08304304871028,1.,-3.88164007721313));
#53970=CARTESIAN_POINT('Ctrl Pts',(1.08228241999346,-1.,-3.88926088975114));
#53971=CARTESIAN_POINT('Ctrl Pts',(1.08228241999346,1.,-3.88926088975114));
#53972=CARTESIAN_POINT('Ctrl Pts',(1.08148086931358,-1.,-3.8968852509835));
#53973=CARTESIAN_POINT('Ctrl Pts',(1.08148086931358,1.,-3.8968852509835));
#53974=CARTESIAN_POINT('Ctrl Pts',(1.08063906483818,-1.,-3.90451384092545));
#53975=CARTESIAN_POINT('Ctrl Pts',(1.08063906483818,1.,-3.90451384092545));
#53976=CARTESIAN_POINT('Ctrl Pts',(1.07975763507473,-1.,-3.91214726022143));
#53977=CARTESIAN_POINT('Ctrl Pts',(1.07975763507473,1.,-3.91214726022143));
#53978=CARTESIAN_POINT('Ctrl Pts',(1.07883706663554,-1.,-3.91978568924178));
#53979=CARTESIAN_POINT('Ctrl Pts',(1.07883706663554,1.,-3.91978568924178));
#53980=CARTESIAN_POINT('Ctrl Pts',(1.07787771707195,-1.,-3.9274289334984));
#53981=CARTESIAN_POINT('Ctrl Pts',(1.07787771707195,1.,-3.9274289334984));
#53982=CARTESIAN_POINT('Ctrl Pts',(1.07687985975384,-1.,-3.93507657572883));
#53983=CARTESIAN_POINT('Ctrl Pts',(1.07687985975384,1.,-3.93507657572883));
#53984=CARTESIAN_POINT('Ctrl Pts',(1.07584371946443,-1.,-3.94272809633331));
#53985=CARTESIAN_POINT('Ctrl Pts',(1.07584371946443,1.,-3.94272809633331));
#53986=CARTESIAN_POINT('Ctrl Pts',(1.07476950921587,-1.,-3.95038299600676));
#53987=CARTESIAN_POINT('Ctrl Pts',(1.07476950921587,1.,-3.95038299600676));
#53988=CARTESIAN_POINT('Ctrl Pts',(1.07365747426491,-1.,-3.95804094429373));
#53989=CARTESIAN_POINT('Ctrl Pts',(1.07365747426491,1.,-3.95804094429373));
#53990=CARTESIAN_POINT('Ctrl Pts',(1.07250789943007,-1.,-3.96570179322338));
#53991=CARTESIAN_POINT('Ctrl Pts',(1.07250789943007,1.,-3.96570179322338));
#53992=CARTESIAN_POINT('Ctrl Pts',(1.07132109206164,-1.,-3.9733655022223));
#53993=CARTESIAN_POINT('Ctrl Pts',(1.07132109206164,1.,-3.9733655022223));
#53994=CARTESIAN_POINT('Ctrl Pts',(1.07009737257767,-1.,-3.98103208801101));
#53995=CARTESIAN_POINT('Ctrl Pts',(1.07009737257767,1.,-3.98103208801101));
#53996=CARTESIAN_POINT('Ctrl Pts',(1.06883706263941,-1.,-3.98870156857412));
#53997=CARTESIAN_POINT('Ctrl Pts',(1.06883706263941,1.,-3.98870156857412));
#53998=CARTESIAN_POINT('Ctrl Pts',(1.06754047381312,-1.,-3.99637389920441));
#53999=CARTESIAN_POINT('Ctrl Pts',(1.06754047381312,1.,-3.99637389920441));
#54000=CARTESIAN_POINT('Ctrl Pts',(1.06620789963606,-1.,-4.00404894952579));
#54001=CARTESIAN_POINT('Ctrl Pts',(1.06620789963606,1.,-4.00404894952579));
#54002=CARTESIAN_POINT('Ctrl Pts',(1.06483961343109,-1.,-4.01172654187398));
#54003=CARTESIAN_POINT('Ctrl Pts',(1.06483961343109,1.,-4.01172654187398));
#54004=CARTESIAN_POINT('Ctrl Pts',(1.06343586496236,-1.,-4.01940647495943));
#54005=CARTESIAN_POINT('Ctrl Pts',(1.06343586496236,1.,-4.01940647495943));
#54006=CARTESIAN_POINT('Ctrl Pts',(1.06199687787462,-1.,-4.02708855235633));
#54007=CARTESIAN_POINT('Ctrl Pts',(1.06199687787462,1.,-4.02708855235633));
#54008=CARTESIAN_POINT('Ctrl Pts',(1.06052284711857,-1.,-4.03477261141553));
#54009=CARTESIAN_POINT('Ctrl Pts',(1.06052284711857,1.,-4.03477261141553));
#54010=CARTESIAN_POINT('Ctrl Pts',(1.05901393666566,-1.,-4.04245854427496));
#54011=CARTESIAN_POINT('Ctrl Pts',(1.05901393666566,1.,-4.04245854427496));
#54012=CARTESIAN_POINT('Ctrl Pts',(1.05747027727959,-1.,-4.05014628384869));
#54013=CARTESIAN_POINT('Ctrl Pts',(1.05747027727959,1.,-4.05014628384869));
#54014=CARTESIAN_POINT('Ctrl Pts',(1.05620762707996,-1.,-4.05629789307025));
#54015=CARTESIAN_POINT('Ctrl Pts',(1.05620762707996,1.,-4.05629789307025));
#54016=CARTESIAN_POINT('Ctrl Pts',(1.05524507177599,-1.,-4.06091239149123));
#54017=CARTESIAN_POINT('Ctrl Pts',(1.05524507177599,1.,-4.06091239149123));
#54018=CARTESIAN_POINT('Ctrl Pts',(1.05459645194823,-1.,-4.06398907542249));
#54019=CARTESIAN_POINT('Ctrl Pts',(1.05459645194823,1.,-4.06398907542249));
#54020=CARTESIAN_POINT('Ctrl Pts',(1.05427041296137,-1.,-4.06552750530042));
#54021=CARTESIAN_POINT('Ctrl Pts',(1.05427041296137,1.,-4.06552750530042));
#54022=CARTESIAN_POINT('',(1.07167739962028,1.,-3.59360648251073));
#54023=CARTESIAN_POINT('Ctrl Pts',(1.07167739962028,-1.,-3.59360648251073));
#54024=CARTESIAN_POINT('Ctrl Pts',(1.07167739962028,-0.666666666666667,
-3.59360648251073));
#54025=CARTESIAN_POINT('Ctrl Pts',(1.07167739962028,-0.333333333333333,
-3.59360648251073));
#54026=CARTESIAN_POINT('Ctrl Pts',(1.07167739962028,0.333333333333333,-3.59360648251073));
#54027=CARTESIAN_POINT('Ctrl Pts',(1.07167739962028,0.666666666666667,-3.59360648251073));
#54028=CARTESIAN_POINT('Ctrl Pts',(1.07167739962028,1.,-3.59360648251073));
#54029=CARTESIAN_POINT('',(1.05427041296137,1.,-4.06552750530042));
#54030=CARTESIAN_POINT('',(1.05427041296137,0.,-4.06552750530042));
#54031=CARTESIAN_POINT('Ctrl Pts',(1.07167739962028,1.,-3.59360648251073));
#54032=CARTESIAN_POINT('Ctrl Pts',(1.07171709254135,1.,-3.5936351279798));
#54033=CARTESIAN_POINT('Ctrl Pts',(1.07183575450617,1.,-3.59379266874567));
#54034=CARTESIAN_POINT('Ctrl Pts',(1.07209229745229,1.,-3.59439596999862));
#54035=CARTESIAN_POINT('Ctrl Pts',(1.07259084660936,1.,-3.59600583194946));
#54036=CARTESIAN_POINT('Ctrl Pts',(1.07347372545714,1.,-3.59940121154535));
#54037=CARTESIAN_POINT('Ctrl Pts',(1.07469327168578,1.,-3.60456339887778));
#54038=CARTESIAN_POINT('Ctrl Pts',(1.07611545402734,1.,-3.61098481349204));
#54039=CARTESIAN_POINT('Ctrl Pts',(1.07764868137619,1.,-3.61832318504575));
#54040=CARTESIAN_POINT('Ctrl Pts',(1.07919137290742,1.,-3.62619537902361));
#54041=CARTESIAN_POINT('Ctrl Pts',(1.08064765719867,1.,-3.63423373196529));
#54042=CARTESIAN_POINT('Ctrl Pts',(1.08194278850996,1.,-3.64214167843677));
#54043=CARTESIAN_POINT('Ctrl Pts',(1.08304289898623,1.,-3.64976441208358));
#54044=CARTESIAN_POINT('Ctrl Pts',(1.08395671077807,1.,-3.65709649161166));
#54045=CARTESIAN_POINT('Ctrl Pts',(1.08471809922901,1.,-3.66422237895365));
#54046=CARTESIAN_POINT('Ctrl Pts',(1.0853733414449,1.,-3.67127347729666));
#54047=CARTESIAN_POINT('Ctrl Pts',(1.0859675575576,1.,-3.67838211685118));
#54048=CARTESIAN_POINT('Ctrl Pts',(1.0865288888259,1.,-3.68562817420797));
#54049=CARTESIAN_POINT('Ctrl Pts',(1.08706319540271,1.,-3.69302062410157));
#54050=CARTESIAN_POINT('Ctrl Pts',(1.08756311291309,1.,-3.70052690909833));
#54051=CARTESIAN_POINT('Ctrl Pts',(1.08801367312185,1.,-3.70809084139457));
#54052=CARTESIAN_POINT('Ctrl Pts',(1.0883988733478,1.,-3.71565372339075));
#54053=CARTESIAN_POINT('Ctrl Pts',(1.08870887220082,1.,-3.72317741369398));
#54054=CARTESIAN_POINT('Ctrl Pts',(1.08894337390937,1.,-3.73065515162988));
#54055=CARTESIAN_POINT('Ctrl Pts',(1.08910769013297,1.,-3.73809879348239));
#54056=CARTESIAN_POINT('Ctrl Pts',(1.08921040494017,1.,-3.74553121371757));
#54057=CARTESIAN_POINT('Ctrl Pts',(1.08926054632925,1.,-3.75297711748132));
#54058=CARTESIAN_POINT('Ctrl Pts',(1.08926462734281,1.,-3.76045342580208));
#54059=CARTESIAN_POINT('Ctrl Pts',(1.08922484204256,1.,-3.76796340094448));
#54060=CARTESIAN_POINT('Ctrl Pts',(1.0891407279127,1.,-3.77550199409424));
#54061=CARTESIAN_POINT('Ctrl Pts',(1.08901018614636,1.,-3.78305911299504));
#54062=CARTESIAN_POINT('Ctrl Pts',(1.08883071512098,1.,-3.79062357974404));
#54063=CARTESIAN_POINT('Ctrl Pts',(1.08860064435778,1.,-3.79818708705259));
#54064=CARTESIAN_POINT('Ctrl Pts',(1.0883200925538,1.,-3.8057472665766));
#54065=CARTESIAN_POINT('Ctrl Pts',(1.08799030610862,1.,-3.81330554446323));
#54066=CARTESIAN_POINT('Ctrl Pts',(1.08761321539442,1.,-3.82086569676319));
#54067=CARTESIAN_POINT('Ctrl Pts',(1.08719091307558,1.,-3.82843215316984));
#54068=CARTESIAN_POINT('Ctrl Pts',(1.08672515456902,1.,-3.83600837071708));
#54069=CARTESIAN_POINT('Ctrl Pts',(1.08621688337604,1.,-3.8435952876495));
#54070=CARTESIAN_POINT('Ctrl Pts',(1.08566647671844,1.,-3.85119211322755));
#54071=CARTESIAN_POINT('Ctrl Pts',(1.08507395120059,1.,-3.85879698702532));
#54072=CARTESIAN_POINT('Ctrl Pts',(1.08443918607927,1.,-3.86640769434274));
#54073=CARTESIAN_POINT('Ctrl Pts',(1.08376213307504,1.,-3.8740223372254));
#54074=CARTESIAN_POINT('Ctrl Pts',(1.08304304871028,1.,-3.88164007721313));
#54075=CARTESIAN_POINT('Ctrl Pts',(1.08228241999346,1.,-3.88926088975114));
#54076=CARTESIAN_POINT('Ctrl Pts',(1.08148086931358,1.,-3.8968852509835));
#54077=CARTESIAN_POINT('Ctrl Pts',(1.08063906483818,1.,-3.90451384092545));
#54078=CARTESIAN_POINT('Ctrl Pts',(1.07975763507473,1.,-3.91214726022143));
#54079=CARTESIAN_POINT('Ctrl Pts',(1.07883706663554,1.,-3.91978568924178));
#54080=CARTESIAN_POINT('Ctrl Pts',(1.07787771707195,1.,-3.9274289334984));
#54081=CARTESIAN_POINT('Ctrl Pts',(1.07687985975384,1.,-3.93507657572883));
#54082=CARTESIAN_POINT('Ctrl Pts',(1.07584371946443,1.,-3.94272809633331));
#54083=CARTESIAN_POINT('Ctrl Pts',(1.07476950921587,1.,-3.95038299600676));
#54084=CARTESIAN_POINT('Ctrl Pts',(1.07365747426491,1.,-3.95804094429373));
#54085=CARTESIAN_POINT('Ctrl Pts',(1.07250789943007,1.,-3.96570179322338));
#54086=CARTESIAN_POINT('Ctrl Pts',(1.07132109206164,1.,-3.9733655022223));
#54087=CARTESIAN_POINT('Ctrl Pts',(1.07009737257767,1.,-3.98103208801101));
#54088=CARTESIAN_POINT('Ctrl Pts',(1.06883706263941,1.,-3.98870156857412));
#54089=CARTESIAN_POINT('Ctrl Pts',(1.06754047381312,1.,-3.99637389920441));
#54090=CARTESIAN_POINT('Ctrl Pts',(1.06620789963606,1.,-4.00404894952579));
#54091=CARTESIAN_POINT('Ctrl Pts',(1.06483961343109,1.,-4.01172654187398));
#54092=CARTESIAN_POINT('Ctrl Pts',(1.06343586496236,1.,-4.01940647495943));
#54093=CARTESIAN_POINT('Ctrl Pts',(1.06199687787462,1.,-4.02708855235633));
#54094=CARTESIAN_POINT('Ctrl Pts',(1.06052284711857,1.,-4.03477261141553));
#54095=CARTESIAN_POINT('Ctrl Pts',(1.05901393666566,1.,-4.04245854427496));
#54096=CARTESIAN_POINT('Ctrl Pts',(1.05747027727959,1.,-4.05014628384869));
#54097=CARTESIAN_POINT('Ctrl Pts',(1.05620762707996,1.,-4.05629789307025));
#54098=CARTESIAN_POINT('Ctrl Pts',(1.05524507177599,1.,-4.06091239149123));
#54099=CARTESIAN_POINT('Ctrl Pts',(1.05459645194823,1.,-4.06398907542249));
#54100=CARTESIAN_POINT('Ctrl Pts',(1.05427041296137,1.,-4.06552750530042));
#54101=CARTESIAN_POINT('Origin',(1.05427041296137,0.,-4.06552750530042));
#54102=CARTESIAN_POINT('',(0.906349047628866,1.,-4.10104028313088));
#54103=CARTESIAN_POINT('Origin',(0.,0.,0.));
#54104=CARTESIAN_POINT('',(1.24526366418038,1.,-3.5372048861597));
#54105=CARTESIAN_POINT('Origin',(0.,1.,0.));
#54106=CARTESIAN_POINT('Ctrl Pts',(1.24526366418038,1.,-3.5372048861597));
#54107=CARTESIAN_POINT('Ctrl Pts',(1.24526366418038,0.666666666666667,-3.5372048861597));
#54108=CARTESIAN_POINT('Ctrl Pts',(1.24526366418038,0.333333333333333,-3.5372048861597));
#54109=CARTESIAN_POINT('Ctrl Pts',(1.24526366418038,-0.333333333333333,
-3.5372048861597));
#54110=CARTESIAN_POINT('Ctrl Pts',(1.24526366418038,-0.666666666666667,
-3.5372048861597));
#54111=CARTESIAN_POINT('Ctrl Pts',(1.24526366418038,-1.,-3.5372048861597));
#54112=CARTESIAN_POINT('Ctrl Pts',(1.53673442965256,-1.,-3.90876544355381));
#54113=CARTESIAN_POINT('Ctrl Pts',(1.53673442965256,1.,-3.90876544355381));
#54114=CARTESIAN_POINT('Ctrl Pts',(1.53556639217905,-1.,-3.90771246855019));
#54115=CARTESIAN_POINT('Ctrl Pts',(1.53556639217905,1.,-3.90771246855019));
#54116=CARTESIAN_POINT('Ctrl Pts',(1.53323321827755,-1.,-3.90560462813969));
#54117=CARTESIAN_POINT('Ctrl Pts',(1.53323321827755,1.,-3.90560462813969));
#54118=CARTESIAN_POINT('Ctrl Pts',(1.52974216056287,-1.,-3.90243719631596));
#54119=CARTESIAN_POINT('Ctrl Pts',(1.52974216056287,1.,-3.90243719631596));
#54120=CARTESIAN_POINT('Ctrl Pts',(1.52510482991635,-1.,-3.89820260708225));
#54121=CARTESIAN_POINT('Ctrl Pts',(1.52510482991635,1.,-3.89820260708225));
#54122=CARTESIAN_POINT('Ctrl Pts',(1.51933724329305,-1.,-3.89289043533657));
#54123=CARTESIAN_POINT('Ctrl Pts',(1.51933724329305,1.,-3.89289043533657));
#54124=CARTESIAN_POINT('Ctrl Pts',(1.51359883110559,-1.,-3.88755930033884));
#54125=CARTESIAN_POINT('Ctrl Pts',(1.51359883110559,1.,-3.88755930033884));
#54126=CARTESIAN_POINT('Ctrl Pts',(1.50788973857757,-1.,-3.88220917950538));
#54127=CARTESIAN_POINT('Ctrl Pts',(1.50788973857757,1.,-3.88220917950538));
#54128=CARTESIAN_POINT('Ctrl Pts',(1.50221016176556,-1.,-3.87684006372134));
#54129=CARTESIAN_POINT('Ctrl Pts',(1.50221016176556,1.,-3.87684006372134));
#54130=CARTESIAN_POINT('Ctrl Pts',(1.49656035399122,-1.,-3.87145196998465));
#54131=CARTESIAN_POINT('Ctrl Pts',(1.49656035399122,1.,-3.87145196998465));
#54132=CARTESIAN_POINT('Ctrl Pts',(1.4909406116431,-1.,-3.86604492575189));
#54133=CARTESIAN_POINT('Ctrl Pts',(1.4909406116431,1.,-3.86604492575189));
#54134=CARTESIAN_POINT('Ctrl Pts',(1.48535125509919,-1.,-3.86061894706087));
#54135=CARTESIAN_POINT('Ctrl Pts',(1.48535125509919,1.,-3.86061894706087));
#54136=CARTESIAN_POINT('Ctrl Pts',(1.4797926099102,-1.,-3.85517401698843));
#54137=CARTESIAN_POINT('Ctrl Pts',(1.4797926099102,1.,-3.85517401698843));
#54138=CARTESIAN_POINT('Ctrl Pts',(1.47426499018538,-1.,-3.84971006847277));
#54139=CARTESIAN_POINT('Ctrl Pts',(1.47426499018538,1.,-3.84971006847277));
#54140=CARTESIAN_POINT('Ctrl Pts',(1.46876867426504,-1.,-3.84422695454796));
#54141=CARTESIAN_POINT('Ctrl Pts',(1.46876867426504,1.,-3.84422695454796));
#54142=CARTESIAN_POINT('Ctrl Pts',(1.46330391180752,-1.,-3.83872447159639));
#54143=CARTESIAN_POINT('Ctrl Pts',(1.46330391180752,1.,-3.83872447159639));
#54144=CARTESIAN_POINT('Ctrl Pts',(1.45787095220852,-1.,-3.83320241775423));
#54145=CARTESIAN_POINT('Ctrl Pts',(1.45787095220852,1.,-3.83320241775423));
#54146=CARTESIAN_POINT('Ctrl Pts',(1.45247006796836,-1.,-3.82766064519075));
#54147=CARTESIAN_POINT('Ctrl Pts',(1.45247006796836,1.,-3.82766064519075));
#54148=CARTESIAN_POINT('Ctrl Pts',(1.44710157648539,-1.,-3.82209910620533));
#54149=CARTESIAN_POINT('Ctrl Pts',(1.44710157648539,1.,-3.82209910620533));
#54150=CARTESIAN_POINT('Ctrl Pts',(1.44176587041347,-1.,-3.81651792398414));
#54151=CARTESIAN_POINT('Ctrl Pts',(1.44176587041347,1.,-3.81651792398414));
#54152=CARTESIAN_POINT('Ctrl Pts',(1.43646341556724,-1.,-3.81091737726815));
#54153=CARTESIAN_POINT('Ctrl Pts',(1.43646341556724,1.,-3.81091737726815));
#54154=CARTESIAN_POINT('Ctrl Pts',(1.4311946992132,-1.,-3.80529775429805));
#54155=CARTESIAN_POINT('Ctrl Pts',(1.4311946992132,1.,-3.80529775429805));
#54156=CARTESIAN_POINT('Ctrl Pts',(1.42596018777283,-1.,-3.7996592319632));
#54157=CARTESIAN_POINT('Ctrl Pts',(1.42596018777283,1.,-3.7996592319632));
#54158=CARTESIAN_POINT('Ctrl Pts',(1.42076028482836,-1.,-3.79400175744408));
#54159=CARTESIAN_POINT('Ctrl Pts',(1.42076028482836,1.,-3.79400175744408));
#54160=CARTESIAN_POINT('Ctrl Pts',(1.4155952780383,-1.,-3.78832489879426));
#54161=CARTESIAN_POINT('Ctrl Pts',(1.4155952780383,1.,-3.78832489879426));
#54162=CARTESIAN_POINT('Ctrl Pts',(1.41046532282593,-1.,-3.78262780065471));
#54163=CARTESIAN_POINT('Ctrl Pts',(1.41046532282593,1.,-3.78262780065471));
#54164=CARTESIAN_POINT('Ctrl Pts',(1.40537056004722,-1.,-3.77690952014259));
#54165=CARTESIAN_POINT('Ctrl Pts',(1.40537056004722,1.,-3.77690952014259));
#54166=CARTESIAN_POINT('Ctrl Pts',(1.40031121335505,-1.,-3.77116930621827));
#54167=CARTESIAN_POINT('Ctrl Pts',(1.40031121335505,1.,-3.77116930621827));
#54168=CARTESIAN_POINT('Ctrl Pts',(1.39528769118052,-1.,-3.76540689249074));
#54169=CARTESIAN_POINT('Ctrl Pts',(1.39528769118052,1.,-3.76540689249074));
#54170=CARTESIAN_POINT('Ctrl Pts',(1.39030069388918,-1.,-3.75962280650855));
#54171=CARTESIAN_POINT('Ctrl Pts',(1.39030069388918,1.,-3.75962280650855));
#54172=CARTESIAN_POINT('Ctrl Pts',(1.38535129801176,-1.,-3.75381861212707));
#54173=CARTESIAN_POINT('Ctrl Pts',(1.38535129801176,1.,-3.75381861212707));
#54174=CARTESIAN_POINT('Ctrl Pts',(1.38044070763295,-1.,-3.74799617204729));
#54175=CARTESIAN_POINT('Ctrl Pts',(1.38044070763295,1.,-3.74799617204729));
#54176=CARTESIAN_POINT('Ctrl Pts',(1.37557002971687,-1.,-3.74215698162555));
#54177=CARTESIAN_POINT('Ctrl Pts',(1.37557002971687,1.,-3.74215698162555));
#54178=CARTESIAN_POINT('Ctrl Pts',(1.37074003422739,-1.,-3.7363014588581));
#54179=CARTESIAN_POINT('Ctrl Pts',(1.37074003422739,1.,-3.7363014588581));
#54180=CARTESIAN_POINT('Ctrl Pts',(1.36595093298676,-1.,-3.73042829011295));
#54181=CARTESIAN_POINT('Ctrl Pts',(1.36595093298676,1.,-3.73042829011295));
#54182=CARTESIAN_POINT('Ctrl Pts',(1.36120211416354,-1.,-3.72453364678279));
#54183=CARTESIAN_POINT('Ctrl Pts',(1.36120211416354,1.,-3.72453364678279));
#54184=CARTESIAN_POINT('Ctrl Pts',(1.35649266705037,-1.,-3.71861271513313));
#54185=CARTESIAN_POINT('Ctrl Pts',(1.35649266705037,1.,-3.71861271513313));
#54186=CARTESIAN_POINT('Ctrl Pts',(1.35182193384424,-1.,-3.71266130563054));
#54187=CARTESIAN_POINT('Ctrl Pts',(1.35182193384424,1.,-3.71266130563054));
#54188=CARTESIAN_POINT('Ctrl Pts',(1.34719008463534,-1.,-3.70667753188248));
#54189=CARTESIAN_POINT('Ctrl Pts',(1.34719008463534,1.,-3.70667753188248));
#54190=CARTESIAN_POINT('Ctrl Pts',(1.34259860752933,-1.,-3.70066324015119));
#54191=CARTESIAN_POINT('Ctrl Pts',(1.34259860752933,1.,-3.70066324015119));
#54192=CARTESIAN_POINT('Ctrl Pts',(1.33805103398219,-1.,-3.69462613305708));
#54193=CARTESIAN_POINT('Ctrl Pts',(1.33805103398219,1.,-3.69462613305708));
#54194=CARTESIAN_POINT('Ctrl Pts',(1.33355191034523,-1.,-3.68857672413033));
#54195=CARTESIAN_POINT('Ctrl Pts',(1.33355191034523,1.,-3.68857672413033));
#54196=CARTESIAN_POINT('Ctrl Pts',(1.3291054707274,-1.,-3.68252441182551));
#54197=CARTESIAN_POINT('Ctrl Pts',(1.3291054707274,1.,-3.68252441182551));
#54198=CARTESIAN_POINT('Ctrl Pts',(1.32471430856415,-1.,-3.67647355257912));
#54199=CARTESIAN_POINT('Ctrl Pts',(1.32471430856415,1.,-3.67647355257912));
#54200=CARTESIAN_POINT('Ctrl Pts',(1.32037828137766,-1.,-3.67042021752656));
#54201=CARTESIAN_POINT('Ctrl Pts',(1.32037828137766,1.,-3.67042021752656));
#54202=CARTESIAN_POINT('Ctrl Pts',(1.31609271239911,-1.,-3.66434688899793));
#54203=CARTESIAN_POINT('Ctrl Pts',(1.31609271239911,1.,-3.66434688899793));
#54204=CARTESIAN_POINT('Ctrl Pts',(1.31185038411218,-1.,-3.65822827358617));
#54205=CARTESIAN_POINT('Ctrl Pts',(1.31185038411218,1.,-3.65822827358617));
#54206=CARTESIAN_POINT('Ctrl Pts',(1.30764479590039,-1.,-3.65204081987068));
#54207=CARTESIAN_POINT('Ctrl Pts',(1.30764479590039,1.,-3.65204081987068));
#54208=CARTESIAN_POINT('Ctrl Pts',(1.30347327603774,-1.,-3.64577181380113));
#54209=CARTESIAN_POINT('Ctrl Pts',(1.30347327603774,1.,-3.64577181380113));
#54210=CARTESIAN_POINT('Ctrl Pts',(1.2993395590647,-1.,-3.63942689872808));
#54211=CARTESIAN_POINT('Ctrl Pts',(1.2993395590647,1.,-3.63942689872808));
#54212=CARTESIAN_POINT('Ctrl Pts',(1.29525810207762,-1.,-3.63304271631046));
#54213=CARTESIAN_POINT('Ctrl Pts',(1.29525810207762,1.,-3.63304271631046));
#54214=CARTESIAN_POINT('Ctrl Pts',(1.29125046021878,-1.,-3.62667616004369));
#54215=CARTESIAN_POINT('Ctrl Pts',(1.29125046021878,1.,-3.62667616004369));
#54216=CARTESIAN_POINT('Ctrl Pts',(1.28733755029384,-1.,-3.6203814849236));
#54217=CARTESIAN_POINT('Ctrl Pts',(1.28733755029384,1.,-3.6203814849236));
#54218=CARTESIAN_POINT('Ctrl Pts',(1.28353255117765,-1.,-3.61418935913823));
#54219=CARTESIAN_POINT('Ctrl Pts',(1.28353255117765,1.,-3.61418935913823));
#54220=CARTESIAN_POINT('Ctrl Pts',(1.27983492861691,-1.,-3.60808907746339));
#54221=CARTESIAN_POINT('Ctrl Pts',(1.27983492861691,1.,-3.60808907746339));
#54222=CARTESIAN_POINT('Ctrl Pts',(1.27622049908625,-1.,-3.60199947736298));
#54223=CARTESIAN_POINT('Ctrl Pts',(1.27622049908625,1.,-3.60199947736298));
#54224=CARTESIAN_POINT('Ctrl Pts',(1.27264798379307,-1.,-3.59578698050006));
#54225=CARTESIAN_POINT('Ctrl Pts',(1.27264798379307,1.,-3.59578698050006));
#54226=CARTESIAN_POINT('Ctrl Pts',(1.26907758484709,-1.,-3.58931807846313));
#54227=CARTESIAN_POINT('Ctrl Pts',(1.26907758484709,1.,-3.58931807846313));
#54228=CARTESIAN_POINT('Ctrl Pts',(1.26548706249862,-1.,-3.58250452868618));
#54229=CARTESIAN_POINT('Ctrl Pts',(1.26548706249862,1.,-3.58250452868618));
#54230=CARTESIAN_POINT('Ctrl Pts',(1.2618866714281,-1.,-3.5753456065171));
#54231=CARTESIAN_POINT('Ctrl Pts',(1.2618866714281,1.,-3.5753456065171));
#54232=CARTESIAN_POINT('Ctrl Pts',(1.25834000485716,-1.,-3.56798645995275));
#54233=CARTESIAN_POINT('Ctrl Pts',(1.25834000485716,1.,-3.56798645995275));
#54234=CARTESIAN_POINT('Ctrl Pts',(1.25496090900009,-1.,-3.56071094991199));
#54235=CARTESIAN_POINT('Ctrl Pts',(1.25496090900009,1.,-3.56071094991199));
#54236=CARTESIAN_POINT('Ctrl Pts',(1.2518879294064,-1.,-3.55387287418985));
#54237=CARTESIAN_POINT('Ctrl Pts',(1.2518879294064,1.,-3.55387287418985));
#54238=CARTESIAN_POINT('Ctrl Pts',(1.24926408628003,-1.,-3.54784190283068));
#54239=CARTESIAN_POINT('Ctrl Pts',(1.24926408628003,1.,-3.54784190283068));
#54240=CARTESIAN_POINT('Ctrl Pts',(1.24721646231966,-1.,-3.54294877425964));
#54241=CARTESIAN_POINT('Ctrl Pts',(1.24721646231966,1.,-3.54294877425964));
#54242=CARTESIAN_POINT('Ctrl Pts',(1.24583101679029,-1.,-3.53941798195825));
#54243=CARTESIAN_POINT('Ctrl Pts',(1.24583101679029,1.,-3.53941798195825));
#54244=CARTESIAN_POINT('Ctrl Pts',(1.24528461332987,-1.,-3.53776753802906));
#54245=CARTESIAN_POINT('Ctrl Pts',(1.24528461332987,1.,-3.53776753802906));
#54246=CARTESIAN_POINT('Ctrl Pts',(1.24519702335451,-1.,-3.53720633057798));
#54247=CARTESIAN_POINT('Ctrl Pts',(1.24519702335451,1.,-3.53720633057798));
#54248=CARTESIAN_POINT('Ctrl Pts',(1.24528174185098,-1.,-3.53713269667399));
#54249=CARTESIAN_POINT('Ctrl Pts',(1.24528174185098,1.,-3.53713269667399));
#54250=CARTESIAN_POINT('Ctrl Pts',(1.24535988127942,-1.,-3.53717101171257));
#54251=CARTESIAN_POINT('Ctrl Pts',(1.24535988127942,1.,-3.53717101171257));
#54252=CARTESIAN_POINT('',(1.53673442965256,1.,-3.90876544355381));
#54253=CARTESIAN_POINT('Ctrl Pts',(1.53673442965256,1.,-3.90876544355381));
#54254=CARTESIAN_POINT('Ctrl Pts',(1.53556639217905,1.,-3.90771246855019));
#54255=CARTESIAN_POINT('Ctrl Pts',(1.53323321827755,1.,-3.90560462813969));
#54256=CARTESIAN_POINT('Ctrl Pts',(1.52974216056287,1.,-3.90243719631596));
#54257=CARTESIAN_POINT('Ctrl Pts',(1.52510482991635,1.,-3.89820260708225));
#54258=CARTESIAN_POINT('Ctrl Pts',(1.51933724329305,1.,-3.89289043533657));
#54259=CARTESIAN_POINT('Ctrl Pts',(1.51359883110559,1.,-3.88755930033884));
#54260=CARTESIAN_POINT('Ctrl Pts',(1.50788973857757,1.,-3.88220917950538));
#54261=CARTESIAN_POINT('Ctrl Pts',(1.50221016176556,1.,-3.87684006372134));
#54262=CARTESIAN_POINT('Ctrl Pts',(1.49656035399122,1.,-3.87145196998465));
#54263=CARTESIAN_POINT('Ctrl Pts',(1.4909406116431,1.,-3.86604492575189));
#54264=CARTESIAN_POINT('Ctrl Pts',(1.48535125509919,1.,-3.86061894706087));
#54265=CARTESIAN_POINT('Ctrl Pts',(1.4797926099102,1.,-3.85517401698843));
#54266=CARTESIAN_POINT('Ctrl Pts',(1.47426499018538,1.,-3.84971006847277));
#54267=CARTESIAN_POINT('Ctrl Pts',(1.46876867426504,1.,-3.84422695454796));
#54268=CARTESIAN_POINT('Ctrl Pts',(1.46330391180752,1.,-3.83872447159639));
#54269=CARTESIAN_POINT('Ctrl Pts',(1.45787095220852,1.,-3.83320241775423));
#54270=CARTESIAN_POINT('Ctrl Pts',(1.45247006796836,1.,-3.82766064519075));
#54271=CARTESIAN_POINT('Ctrl Pts',(1.44710157648539,1.,-3.82209910620533));
#54272=CARTESIAN_POINT('Ctrl Pts',(1.44176587041347,1.,-3.81651792398414));
#54273=CARTESIAN_POINT('Ctrl Pts',(1.43646341556724,1.,-3.81091737726815));
#54274=CARTESIAN_POINT('Ctrl Pts',(1.4311946992132,1.,-3.80529775429805));
#54275=CARTESIAN_POINT('Ctrl Pts',(1.42596018777283,1.,-3.7996592319632));
#54276=CARTESIAN_POINT('Ctrl Pts',(1.42076028482836,1.,-3.79400175744408));
#54277=CARTESIAN_POINT('Ctrl Pts',(1.4155952780383,1.,-3.78832489879426));
#54278=CARTESIAN_POINT('Ctrl Pts',(1.41046532282593,1.,-3.78262780065471));
#54279=CARTESIAN_POINT('Ctrl Pts',(1.40537056004722,1.,-3.77690952014259));
#54280=CARTESIAN_POINT('Ctrl Pts',(1.40031121335505,1.,-3.77116930621827));
#54281=CARTESIAN_POINT('Ctrl Pts',(1.39528769118052,1.,-3.76540689249074));
#54282=CARTESIAN_POINT('Ctrl Pts',(1.39030069388918,1.,-3.75962280650855));
#54283=CARTESIAN_POINT('Ctrl Pts',(1.38535129801176,1.,-3.75381861212707));
#54284=CARTESIAN_POINT('Ctrl Pts',(1.38044070763295,1.,-3.74799617204729));
#54285=CARTESIAN_POINT('Ctrl Pts',(1.37557002971687,1.,-3.74215698162555));
#54286=CARTESIAN_POINT('Ctrl Pts',(1.37074003422739,1.,-3.7363014588581));
#54287=CARTESIAN_POINT('Ctrl Pts',(1.36595093298676,1.,-3.73042829011295));
#54288=CARTESIAN_POINT('Ctrl Pts',(1.36120211416354,1.,-3.72453364678279));
#54289=CARTESIAN_POINT('Ctrl Pts',(1.35649266705037,1.,-3.71861271513313));
#54290=CARTESIAN_POINT('Ctrl Pts',(1.35182193384424,1.,-3.71266130563054));
#54291=CARTESIAN_POINT('Ctrl Pts',(1.34719008463534,1.,-3.70667753188248));
#54292=CARTESIAN_POINT('Ctrl Pts',(1.34259860752933,1.,-3.70066324015119));
#54293=CARTESIAN_POINT('Ctrl Pts',(1.33805103398219,1.,-3.69462613305708));
#54294=CARTESIAN_POINT('Ctrl Pts',(1.33355191034523,1.,-3.68857672413033));
#54295=CARTESIAN_POINT('Ctrl Pts',(1.3291054707274,1.,-3.68252441182551));
#54296=CARTESIAN_POINT('Ctrl Pts',(1.32471430856415,1.,-3.67647355257912));
#54297=CARTESIAN_POINT('Ctrl Pts',(1.32037828137766,1.,-3.67042021752656));
#54298=CARTESIAN_POINT('Ctrl Pts',(1.31609271239911,1.,-3.66434688899793));
#54299=CARTESIAN_POINT('Ctrl Pts',(1.31185038411218,1.,-3.65822827358617));
#54300=CARTESIAN_POINT('Ctrl Pts',(1.30764479590039,1.,-3.65204081987068));
#54301=CARTESIAN_POINT('Ctrl Pts',(1.30347327603774,1.,-3.64577181380113));
#54302=CARTESIAN_POINT('Ctrl Pts',(1.2993395590647,1.,-3.63942689872808));
#54303=CARTESIAN_POINT('Ctrl Pts',(1.29525810207762,1.,-3.63304271631046));
#54304=CARTESIAN_POINT('Ctrl Pts',(1.29125046021878,1.,-3.62667616004369));
#54305=CARTESIAN_POINT('Ctrl Pts',(1.28733755029384,1.,-3.6203814849236));
#54306=CARTESIAN_POINT('Ctrl Pts',(1.28353255117765,1.,-3.61418935913823));
#54307=CARTESIAN_POINT('Ctrl Pts',(1.27983492861691,1.,-3.60808907746339));
#54308=CARTESIAN_POINT('Ctrl Pts',(1.27622049908625,1.,-3.60199947736298));
#54309=CARTESIAN_POINT('Ctrl Pts',(1.27264798379307,1.,-3.59578698050006));
#54310=CARTESIAN_POINT('Ctrl Pts',(1.26907758484709,1.,-3.58931807846313));
#54311=CARTESIAN_POINT('Ctrl Pts',(1.26548706249862,1.,-3.58250452868618));
#54312=CARTESIAN_POINT('Ctrl Pts',(1.2618866714281,1.,-3.5753456065171));
#54313=CARTESIAN_POINT('Ctrl Pts',(1.25834000485716,1.,-3.56798645995275));
#54314=CARTESIAN_POINT('Ctrl Pts',(1.25496090900009,1.,-3.56071094991199));
#54315=CARTESIAN_POINT('Ctrl Pts',(1.2518879294064,1.,-3.55387287418985));
#54316=CARTESIAN_POINT('Ctrl Pts',(1.24926408628003,1.,-3.54784190283068));
#54317=CARTESIAN_POINT('Ctrl Pts',(1.24721646231966,1.,-3.54294877425964));
#54318=CARTESIAN_POINT('Ctrl Pts',(1.24593497226008,1.,-3.53968291130022));
#54319=CARTESIAN_POINT('Ctrl Pts',(1.24539205388767,1.,-3.53808746578196));
#54320=CARTESIAN_POINT('Ctrl Pts',(1.2452449899111,1.,-3.5374485926552));
#54321=CARTESIAN_POINT('Ctrl Pts',(1.24524838931757,1.,-3.53725139174486));
#54322=CARTESIAN_POINT('Ctrl Pts',(1.24526366418038,1.,-3.5372048861597));
#54323=CARTESIAN_POINT('',(1.53673442965256,0.,-3.90876544355381));
#54324=CARTESIAN_POINT('Ctrl Pts',(1.62055519152809,-1.,-3.38176002566879));
#54325=CARTESIAN_POINT('Ctrl Pts',(1.62055519152809,1.,-3.38176002566879));
#54326=CARTESIAN_POINT('Ctrl Pts',(1.62058335162482,-1.,-3.38167767992676));
#54327=CARTESIAN_POINT('Ctrl Pts',(1.62058335162482,1.,-3.38167767992676));
#54328=CARTESIAN_POINT('Ctrl Pts',(1.62069532368199,-1.,-3.38166984193836));
#54329=CARTESIAN_POINT('Ctrl Pts',(1.62069532368199,1.,-3.38166984193836));
#54330=CARTESIAN_POINT('Ctrl Pts',(1.62103022181151,-1.,-3.38212861099984));
#54331=CARTESIAN_POINT('Ctrl Pts',(1.62103022181151,1.,-3.38212861099984));
#54332=CARTESIAN_POINT('Ctrl Pts',(1.62181089631344,-1.,-3.38368201668574));
#54333=CARTESIAN_POINT('Ctrl Pts',(1.62181089631344,1.,-3.38368201668574));
#54334=CARTESIAN_POINT('Ctrl Pts',(1.6233278855625,-1.,-3.38715832179072));
#54335=CARTESIAN_POINT('Ctrl Pts',(1.6233278855625,1.,-3.38715832179072));
#54336=CARTESIAN_POINT('Ctrl Pts',(1.62533996116713,-1.,-3.39206617496906));
#54337=CARTESIAN_POINT('Ctrl Pts',(1.62533996116713,1.,-3.39206617496906));
#54338=CARTESIAN_POINT('Ctrl Pts',(1.62774916464408,-1.,-3.39818605297991));
#54339=CARTESIAN_POINT('Ctrl Pts',(1.62774916464408,1.,-3.39818605297991));
#54340=CARTESIAN_POINT('Ctrl Pts',(1.63041148964828,-1.,-3.40519422740235));
#54341=CARTESIAN_POINT('Ctrl Pts',(1.63041148964828,1.,-3.40519422740235));
#54342=CARTESIAN_POINT('Ctrl Pts',(1.63316667054044,-1.,-3.41272817148478));
#54343=CARTESIAN_POINT('Ctrl Pts',(1.63316667054044,1.,-3.41272817148478));
#54344=CARTESIAN_POINT('Ctrl Pts',(1.63586250099773,-1.,-3.42043974590882));
#54345=CARTESIAN_POINT('Ctrl Pts',(1.63586250099773,1.,-3.42043974590882));
#54346=CARTESIAN_POINT('Ctrl Pts',(1.63837876246926,-1.,-3.42804772926291));
#54347=CARTESIAN_POINT('Ctrl Pts',(1.63837876246926,1.,-3.42804772926291));
#54348=CARTESIAN_POINT('Ctrl Pts',(1.64065778702023,-1.,-3.43540451921548));
#54349=CARTESIAN_POINT('Ctrl Pts',(1.64065778702023,1.,-3.43540451921548));
#54350=CARTESIAN_POINT('Ctrl Pts',(1.64270733821113,-1.,-3.44250337701888));
#54351=CARTESIAN_POINT('Ctrl Pts',(1.64270733821113,1.,-3.44250337701888));
#54352=CARTESIAN_POINT('Ctrl Pts',(1.64457408708107,-1.,-3.44942242546795));
#54353=CARTESIAN_POINT('Ctrl Pts',(1.64457408708107,1.,-3.44942242546795));
#54354=CARTESIAN_POINT('Ctrl Pts',(1.64632429697521,-1.,-3.45628421062422));
#54355=CARTESIAN_POINT('Ctrl Pts',(1.64632429697521,1.,-3.45628421062422));
#54356=CARTESIAN_POINT('Ctrl Pts',(1.64802323352738,-1.,-3.46321237515));
#54357=CARTESIAN_POINT('Ctrl Pts',(1.64802323352738,1.,-3.46321237515));
#54358=CARTESIAN_POINT('Ctrl Pts',(1.64971118698256,-1.,-3.47028140995992));
#54359=CARTESIAN_POINT('Ctrl Pts',(1.64971118698256,1.,-3.47028140995992));
#54360=CARTESIAN_POINT('Ctrl Pts',(1.65139534930322,-1.,-3.47749926256476));
#54361=CARTESIAN_POINT('Ctrl Pts',(1.65139534930322,1.,-3.47749926256476));
#54362=CARTESIAN_POINT('Ctrl Pts',(1.65306335367739,-1.,-3.48483492840894));
#54363=CARTESIAN_POINT('Ctrl Pts',(1.65306335367739,1.,-3.48483492840894));
#54364=CARTESIAN_POINT('Ctrl Pts',(1.65469162644468,-1.,-3.49223525300176));
#54365=CARTESIAN_POINT('Ctrl Pts',(1.65469162644468,1.,-3.49223525300176));
#54366=CARTESIAN_POINT('Ctrl Pts',(1.65625517961588,-1.,-3.4996447647794));
#54367=CARTESIAN_POINT('Ctrl Pts',(1.65625517961588,1.,-3.4996447647794));
#54368=CARTESIAN_POINT('Ctrl Pts',(1.65773832633632,-1.,-3.50702733146542));
#54369=CARTESIAN_POINT('Ctrl Pts',(1.65773832633632,1.,-3.50702733146542));
#54370=CARTESIAN_POINT('Ctrl Pts',(1.65913971687342,-1.,-3.5143763218894));
#54371=CARTESIAN_POINT('Ctrl Pts',(1.65913971687342,1.,-3.5143763218894));
#54372=CARTESIAN_POINT('Ctrl Pts',(1.66046645222279,-1.,-3.52170261543816));
#54373=CARTESIAN_POINT('Ctrl Pts',(1.66046645222279,1.,-3.52170261543816));
#54374=CARTESIAN_POINT('Ctrl Pts',(1.66173058912371,-1.,-3.52902746211093));
#54375=CARTESIAN_POINT('Ctrl Pts',(1.66173058912371,1.,-3.52902746211093));
#54376=CARTESIAN_POINT('Ctrl Pts',(1.66294490916111,-1.,-3.5363738506022));
#54377=CARTESIAN_POINT('Ctrl Pts',(1.66294490916111,1.,-3.5363738506022));
#54378=CARTESIAN_POINT('Ctrl Pts',(1.66411849222326,-1.,-3.54375747475014));
#54379=CARTESIAN_POINT('Ctrl Pts',(1.66411849222326,1.,-3.54375747475014));
#54380=CARTESIAN_POINT('Ctrl Pts',(1.66525401568994,-1.,-3.55118121342861));
#54381=CARTESIAN_POINT('Ctrl Pts',(1.66525401568994,1.,-3.55118121342861));
#54382=CARTESIAN_POINT('Ctrl Pts',(1.66635023293114,-1.,-3.55864015233602));
#54383=CARTESIAN_POINT('Ctrl Pts',(1.66635023293114,1.,-3.55864015233602));
#54384=CARTESIAN_POINT('Ctrl Pts',(1.66740349220305,-1.,-3.56612465179422));
#54385=CARTESIAN_POINT('Ctrl Pts',(1.66740349220305,1.,-3.56612465179422));
#54386=CARTESIAN_POINT('Ctrl Pts',(1.668409574073,-1.,-3.57362406285887));
#54387=CARTESIAN_POINT('Ctrl Pts',(1.668409574073,1.,-3.57362406285887));
#54388=CARTESIAN_POINT('Ctrl Pts',(1.66936552908232,-1.,-3.58113044183829));
#54389=CARTESIAN_POINT('Ctrl Pts',(1.66936552908232,1.,-3.58113044183829));
#54390=CARTESIAN_POINT('Ctrl Pts',(1.67027110397604,-1.,-3.58864143097834));
#54391=CARTESIAN_POINT('Ctrl Pts',(1.67027110397604,1.,-3.58864143097834));
#54392=CARTESIAN_POINT('Ctrl Pts',(1.67112775290707,-1.,-3.59615824388807));
#54393=CARTESIAN_POINT('Ctrl Pts',(1.67112775290707,1.,-3.59615824388807));
#54394=CARTESIAN_POINT('Ctrl Pts',(1.67193797318597,-1.,-3.60368430815201));
#54395=CARTESIAN_POINT('Ctrl Pts',(1.67193797318597,1.,-3.60368430815201));
#54396=CARTESIAN_POINT('Ctrl Pts',(1.67270452466968,-1.,-3.61122367156181));
#54397=CARTESIAN_POINT('Ctrl Pts',(1.67270452466968,1.,-3.61122367156181));
#54398=CARTESIAN_POINT('Ctrl Pts',(1.67342968196224,-1.,-3.61877947398184));
#54399=CARTESIAN_POINT('Ctrl Pts',(1.67342968196224,1.,-3.61877947398184));
#54400=CARTESIAN_POINT('Ctrl Pts',(1.67411452372271,-1.,-3.62635249450923));
#54401=CARTESIAN_POINT('Ctrl Pts',(1.67411452372271,1.,-3.62635249450923));
#54402=CARTESIAN_POINT('Ctrl Pts',(1.67475929882971,-1.,-3.63394189312924));
#54403=CARTESIAN_POINT('Ctrl Pts',(1.67475929882971,1.,-3.63394189312924));
#54404=CARTESIAN_POINT('Ctrl Pts',(1.67536373264848,-1.,-3.6415458297234));
#54405=CARTESIAN_POINT('Ctrl Pts',(1.67536373264848,1.,-3.6415458297234));
#54406=CARTESIAN_POINT('Ctrl Pts',(1.67592735946692,-1.,-3.64916213574667));
#54407=CARTESIAN_POINT('Ctrl Pts',(1.67592735946692,1.,-3.64916213574667));
#54408=CARTESIAN_POINT('Ctrl Pts',(1.67644983469449,-1.,-3.6567889441642));
#54409=CARTESIAN_POINT('Ctrl Pts',(1.67644983469449,1.,-3.6567889441642));
#54410=CARTESIAN_POINT('Ctrl Pts',(1.67693128053132,-1.,-3.66442538670968));
#54411=CARTESIAN_POINT('Ctrl Pts',(1.67693128053132,1.,-3.66442538670968));
#54412=CARTESIAN_POINT('Ctrl Pts',(1.67737217414874,-1.,-3.67207136294575));
#54413=CARTESIAN_POINT('Ctrl Pts',(1.67737217414874,1.,-3.67207136294575));
#54414=CARTESIAN_POINT('Ctrl Pts',(1.67777320475848,-1.,-3.67972724579124));
#54415=CARTESIAN_POINT('Ctrl Pts',(1.67777320475848,1.,-3.67972724579124));
#54416=CARTESIAN_POINT('Ctrl Pts',(1.67813513867965,-1.,-3.68739360236487));
#54417=CARTESIAN_POINT('Ctrl Pts',(1.67813513867965,1.,-3.68739360236487));
#54418=CARTESIAN_POINT('Ctrl Pts',(1.67845869064323,-1.,-3.6950709275959));
#54419=CARTESIAN_POINT('Ctrl Pts',(1.67845869064323,1.,-3.6950709275959));
#54420=CARTESIAN_POINT('Ctrl Pts',(1.67874436948667,-1.,-3.70275932351108));
#54421=CARTESIAN_POINT('Ctrl Pts',(1.67874436948667,1.,-3.70275932351108));
#54422=CARTESIAN_POINT('Ctrl Pts',(1.67899249793462,-1.,-3.71045854208343));
#54423=CARTESIAN_POINT('Ctrl Pts',(1.67899249793462,1.,-3.71045854208343));
#54424=CARTESIAN_POINT('Ctrl Pts',(1.67920328071708,-1.,-3.71816812842322));
#54425=CARTESIAN_POINT('Ctrl Pts',(1.67920328071708,1.,-3.71816812842322));
#54426=CARTESIAN_POINT('Ctrl Pts',(1.67937685856652,-1.,-3.72588753416396));
#54427=CARTESIAN_POINT('Ctrl Pts',(1.67937685856652,1.,-3.72588753416396));
#54428=CARTESIAN_POINT('Ctrl Pts',(1.67951336376402,-1.,-3.73361623282543));
#54429=CARTESIAN_POINT('Ctrl Pts',(1.67951336376402,1.,-3.73361623282543));
#54430=CARTESIAN_POINT('Ctrl Pts',(1.6796129868522,-1.,-3.74135385965401));
#54431=CARTESIAN_POINT('Ctrl Pts',(1.6796129868522,1.,-3.74135385965401));
#54432=CARTESIAN_POINT('Ctrl Pts',(1.67967598599525,-1.,-3.7491002239452));
#54433=CARTESIAN_POINT('Ctrl Pts',(1.67967598599525,1.,-3.7491002239452));
#54434=CARTESIAN_POINT('Ctrl Pts',(1.67970265841239,-1.,-3.75685523754493));
#54435=CARTESIAN_POINT('Ctrl Pts',(1.67970265841239,1.,-3.75685523754493));
#54436=CARTESIAN_POINT('Ctrl Pts',(1.67969332319245,-1.,-3.76461886684344));
#54437=CARTESIAN_POINT('Ctrl Pts',(1.67969332319245,1.,-3.76461886684344));
#54438=CARTESIAN_POINT('Ctrl Pts',(1.67964830084993,-1.,-3.77239107928502));
#54439=CARTESIAN_POINT('Ctrl Pts',(1.67964830084993,1.,-3.77239107928502));
#54440=CARTESIAN_POINT('Ctrl Pts',(1.67956789212141,-1.,-3.78017178197317));
#54441=CARTESIAN_POINT('Ctrl Pts',(1.67956789212141,1.,-3.78017178197317));
#54442=CARTESIAN_POINT('Ctrl Pts',(1.67945236653493,-1.,-3.7879608002176));
#54443=CARTESIAN_POINT('Ctrl Pts',(1.67945236653493,1.,-3.7879608002176));
#54444=CARTESIAN_POINT('Ctrl Pts',(1.67930196625548,-1.,-3.79575791578424));
#54445=CARTESIAN_POINT('Ctrl Pts',(1.67930196625548,1.,-3.79575791578424));
#54446=CARTESIAN_POINT('Ctrl Pts',(1.67911690648355,-1.,-3.80356289079005));
#54447=CARTESIAN_POINT('Ctrl Pts',(1.67911690648355,1.,-3.80356289079005));
#54448=CARTESIAN_POINT('Ctrl Pts',(1.6788973773827,-1.,-3.81137549624179));
#54449=CARTESIAN_POINT('Ctrl Pts',(1.6788973773827,1.,-3.81137549624179));
#54450=CARTESIAN_POINT('Ctrl Pts',(1.67864354605954,-1.,-3.81919554099578));
#54451=CARTESIAN_POINT('Ctrl Pts',(1.67864354605954,1.,-3.81919554099578));
#54452=CARTESIAN_POINT('Ctrl Pts',(1.6783555575934,-1.,-3.82702289286713));
#54453=CARTESIAN_POINT('Ctrl Pts',(1.6783555575934,1.,-3.82702289286713));
#54454=CARTESIAN_POINT('Ctrl Pts',(1.67803353064351,-1.,-3.8348574651399));
#54455=CARTESIAN_POINT('Ctrl Pts',(1.67803353064351,1.,-3.8348574651399));
#54456=CARTESIAN_POINT('Ctrl Pts',(1.67774874946079,-1.,-3.84113085985244));
#54457=CARTESIAN_POINT('Ctrl Pts',(1.67774874946079,1.,-3.84113085985244));
#54458=CARTESIAN_POINT('Ctrl Pts',(1.6775199114018,-1.,-3.84583912296459));
#54459=CARTESIAN_POINT('Ctrl Pts',(1.6775199114018,1.,-3.84583912296459));
#54460=CARTESIAN_POINT('Ctrl Pts',(1.67736057656533,-1.,-3.84897939430696));
#54461=CARTESIAN_POINT('Ctrl Pts',(1.67736057656533,1.,-3.84897939430696));
#54462=CARTESIAN_POINT('Ctrl Pts',(1.67727921511438,-1.,-3.85054988729471));
#54463=CARTESIAN_POINT('Ctrl Pts',(1.67727921511438,1.,-3.85054988729471));
#54464=CARTESIAN_POINT('',(1.62064718014094,1.,-3.38171594275765));
#54465=CARTESIAN_POINT('Ctrl Pts',(1.62064718014093,-1.,-3.38171594275765));
#54466=CARTESIAN_POINT('Ctrl Pts',(1.62064718014093,-0.666666666666667,
-3.38171594275765));
#54467=CARTESIAN_POINT('Ctrl Pts',(1.62064718014093,-0.333333333333333,
-3.38171594275765));
#54468=CARTESIAN_POINT('Ctrl Pts',(1.62064718014093,0.333333333333333,-3.38171594275765));
#54469=CARTESIAN_POINT('Ctrl Pts',(1.62064718014093,0.666666666666667,-3.38171594275765));
#54470=CARTESIAN_POINT('Ctrl Pts',(1.62064718014093,1.,-3.38171594275765));
#54471=CARTESIAN_POINT('',(1.67727921511438,1.,-3.85054988729471));
#54472=CARTESIAN_POINT('',(1.67727921511438,0.,-3.85054988729471));
#54473=CARTESIAN_POINT('Ctrl Pts',(1.62064718014094,1.,-3.38171594275765));
#54474=CARTESIAN_POINT('Ctrl Pts',(1.62069086551492,1.,-3.38173802621259));
#54475=CARTESIAN_POINT('Ctrl Pts',(1.62083271135947,1.,-3.38187506456922));
#54476=CARTESIAN_POINT('Ctrl Pts',(1.62118047294498,1.,-3.38243080602409));
#54477=CARTESIAN_POINT('Ctrl Pts',(1.62192472202769,1.,-3.38394285763222));
#54478=CARTESIAN_POINT('Ctrl Pts',(1.6233278855625,1.,-3.38715832179072));
#54479=CARTESIAN_POINT('Ctrl Pts',(1.62533996116713,1.,-3.39206617496906));
#54480=CARTESIAN_POINT('Ctrl Pts',(1.62774916464408,1.,-3.39818605297991));
#54481=CARTESIAN_POINT('Ctrl Pts',(1.63041148964828,1.,-3.40519422740235));
#54482=CARTESIAN_POINT('Ctrl Pts',(1.63316667054044,1.,-3.41272817148478));
#54483=CARTESIAN_POINT('Ctrl Pts',(1.63586250099773,1.,-3.42043974590882));
#54484=CARTESIAN_POINT('Ctrl Pts',(1.63837876246926,1.,-3.42804772926291));
#54485=CARTESIAN_POINT('Ctrl Pts',(1.64065778702023,1.,-3.43540451921548));
#54486=CARTESIAN_POINT('Ctrl Pts',(1.64270733821113,1.,-3.44250337701888));
#54487=CARTESIAN_POINT('Ctrl Pts',(1.64457408708107,1.,-3.44942242546795));
#54488=CARTESIAN_POINT('Ctrl Pts',(1.64632429697521,1.,-3.45628421062422));
#54489=CARTESIAN_POINT('Ctrl Pts',(1.64802323352738,1.,-3.46321237515));
#54490=CARTESIAN_POINT('Ctrl Pts',(1.64971118698256,1.,-3.47028140995992));
#54491=CARTESIAN_POINT('Ctrl Pts',(1.65139534930322,1.,-3.47749926256476));
#54492=CARTESIAN_POINT('Ctrl Pts',(1.65306335367739,1.,-3.48483492840894));
#54493=CARTESIAN_POINT('Ctrl Pts',(1.65469162644468,1.,-3.49223525300176));
#54494=CARTESIAN_POINT('Ctrl Pts',(1.65625517961588,1.,-3.4996447647794));
#54495=CARTESIAN_POINT('Ctrl Pts',(1.65773832633632,1.,-3.50702733146542));
#54496=CARTESIAN_POINT('Ctrl Pts',(1.65913971687342,1.,-3.5143763218894));
#54497=CARTESIAN_POINT('Ctrl Pts',(1.66046645222279,1.,-3.52170261543816));
#54498=CARTESIAN_POINT('Ctrl Pts',(1.66173058912371,1.,-3.52902746211093));
#54499=CARTESIAN_POINT('Ctrl Pts',(1.66294490916111,1.,-3.5363738506022));
#54500=CARTESIAN_POINT('Ctrl Pts',(1.66411849222326,1.,-3.54375747475014));
#54501=CARTESIAN_POINT('Ctrl Pts',(1.66525401568994,1.,-3.55118121342861));
#54502=CARTESIAN_POINT('Ctrl Pts',(1.66635023293114,1.,-3.55864015233602));
#54503=CARTESIAN_POINT('Ctrl Pts',(1.66740349220305,1.,-3.56612465179422));
#54504=CARTESIAN_POINT('Ctrl Pts',(1.668409574073,1.,-3.57362406285887));
#54505=CARTESIAN_POINT('Ctrl Pts',(1.66936552908232,1.,-3.58113044183829));
#54506=CARTESIAN_POINT('Ctrl Pts',(1.67027110397604,1.,-3.58864143097834));
#54507=CARTESIAN_POINT('Ctrl Pts',(1.67112775290707,1.,-3.59615824388807));
#54508=CARTESIAN_POINT('Ctrl Pts',(1.67193797318597,1.,-3.60368430815201));
#54509=CARTESIAN_POINT('Ctrl Pts',(1.67270452466968,1.,-3.61122367156181));
#54510=CARTESIAN_POINT('Ctrl Pts',(1.67342968196224,1.,-3.61877947398184));
#54511=CARTESIAN_POINT('Ctrl Pts',(1.67411452372271,1.,-3.62635249450923));
#54512=CARTESIAN_POINT('Ctrl Pts',(1.67475929882971,1.,-3.63394189312924));
#54513=CARTESIAN_POINT('Ctrl Pts',(1.67536373264848,1.,-3.6415458297234));
#54514=CARTESIAN_POINT('Ctrl Pts',(1.67592735946692,1.,-3.64916213574667));
#54515=CARTESIAN_POINT('Ctrl Pts',(1.67644983469449,1.,-3.6567889441642));
#54516=CARTESIAN_POINT('Ctrl Pts',(1.67693128053132,1.,-3.66442538670968));
#54517=CARTESIAN_POINT('Ctrl Pts',(1.67737217414874,1.,-3.67207136294575));
#54518=CARTESIAN_POINT('Ctrl Pts',(1.67777320475848,1.,-3.67972724579124));
#54519=CARTESIAN_POINT('Ctrl Pts',(1.67813513867965,1.,-3.68739360236487));
#54520=CARTESIAN_POINT('Ctrl Pts',(1.67845869064323,1.,-3.6950709275959));
#54521=CARTESIAN_POINT('Ctrl Pts',(1.67874436948667,1.,-3.70275932351108));
#54522=CARTESIAN_POINT('Ctrl Pts',(1.67899249793462,1.,-3.71045854208343));
#54523=CARTESIAN_POINT('Ctrl Pts',(1.67920328071708,1.,-3.71816812842322));
#54524=CARTESIAN_POINT('Ctrl Pts',(1.67937685856652,1.,-3.72588753416396));
#54525=CARTESIAN_POINT('Ctrl Pts',(1.67951336376402,1.,-3.73361623282543));
#54526=CARTESIAN_POINT('Ctrl Pts',(1.6796129868522,1.,-3.74135385965401));
#54527=CARTESIAN_POINT('Ctrl Pts',(1.67967598599525,1.,-3.7491002239452));
#54528=CARTESIAN_POINT('Ctrl Pts',(1.67970265841239,1.,-3.75685523754493));
#54529=CARTESIAN_POINT('Ctrl Pts',(1.67969332319245,1.,-3.76461886684344));
#54530=CARTESIAN_POINT('Ctrl Pts',(1.67964830084993,1.,-3.77239107928502));
#54531=CARTESIAN_POINT('Ctrl Pts',(1.67956789212141,1.,-3.78017178197317));
#54532=CARTESIAN_POINT('Ctrl Pts',(1.67945236653493,1.,-3.7879608002176));
#54533=CARTESIAN_POINT('Ctrl Pts',(1.67930196625548,1.,-3.79575791578424));
#54534=CARTESIAN_POINT('Ctrl Pts',(1.67911690648355,1.,-3.80356289079005));
#54535=CARTESIAN_POINT('Ctrl Pts',(1.6788973773827,1.,-3.81137549624179));
#54536=CARTESIAN_POINT('Ctrl Pts',(1.67864354605954,1.,-3.81919554099578));
#54537=CARTESIAN_POINT('Ctrl Pts',(1.6783555575934,1.,-3.82702289286713));
#54538=CARTESIAN_POINT('Ctrl Pts',(1.67803353064351,1.,-3.8348574651399));
#54539=CARTESIAN_POINT('Ctrl Pts',(1.67774874946079,1.,-3.84113085985244));
#54540=CARTESIAN_POINT('Ctrl Pts',(1.6775199114018,1.,-3.84583912296459));
#54541=CARTESIAN_POINT('Ctrl Pts',(1.67736057656533,1.,-3.84897939430696));
#54542=CARTESIAN_POINT('Ctrl Pts',(1.67727921511438,1.,-3.85054988729471));
#54543=CARTESIAN_POINT('Origin',(1.67727921511438,0.,-3.85054988729471));
#54544=CARTESIAN_POINT('',(1.53673442965256,1.,-3.90876544355381));
#54545=CARTESIAN_POINT('Origin',(0.,0.,0.));
#54546=CARTESIAN_POINT('',(1.78327315618183,1.,-3.29885386921599));
#54547=CARTESIAN_POINT('Origin',(0.,1.,0.));
#54548=CARTESIAN_POINT('Ctrl Pts',(1.78327315618183,1.,-3.29885386921599));
#54549=CARTESIAN_POINT('Ctrl Pts',(1.78327315618183,0.666666666666667,-3.29885386921599));
#54550=CARTESIAN_POINT('Ctrl Pts',(1.78327315618183,0.333333333333333,-3.29885386921599));
#54551=CARTESIAN_POINT('Ctrl Pts',(1.78327315618183,-0.333333333333333,
-3.29885386921599));
#54552=CARTESIAN_POINT('Ctrl Pts',(1.78327315618183,-0.666666666666667,
-3.29885386921599));
#54553=CARTESIAN_POINT('Ctrl Pts',(1.78327315618183,-1.,-3.29885386921599));
#54554=CARTESIAN_POINT('Ctrl Pts',(2.12928030988903,-1.,-3.62024382630768));
#54555=CARTESIAN_POINT('Ctrl Pts',(2.12928030988903,1.,-3.62024382630768));
#54556=CARTESIAN_POINT('Ctrl Pts',(2.12796193131368,-1.,-3.61938653649098));
#54557=CARTESIAN_POINT('Ctrl Pts',(2.12796193131368,1.,-3.61938653649098));
#54558=CARTESIAN_POINT('Ctrl Pts',(2.12532774376758,-1.,-3.61766963590482));
#54559=CARTESIAN_POINT('Ctrl Pts',(2.12532774376758,1.,-3.61766963590482));
#54560=CARTESIAN_POINT('Ctrl Pts',(2.12138417126355,-1.,-3.61508732216891));
#54561=CARTESIAN_POINT('Ctrl Pts',(2.12138417126355,1.,-3.61508732216891));
#54562=CARTESIAN_POINT('Ctrl Pts',(2.11614149815106,-1.,-3.61163030609447));
#54563=CARTESIAN_POINT('Ctrl Pts',(2.11614149815106,1.,-3.61163030609447));
#54564=CARTESIAN_POINT('Ctrl Pts',(2.10961391334462,-1.,-3.60728578532601));
#54565=CARTESIAN_POINT('Ctrl Pts',(2.10961391334462,1.,-3.60728578532601));
#54566=CARTESIAN_POINT('Ctrl Pts',(2.1031121772821,-1.,-3.60291797088734));
#54567=CARTESIAN_POINT('Ctrl Pts',(2.1031121772821,1.,-3.60291797088734));
#54568=CARTESIAN_POINT('Ctrl Pts',(2.09663642986631,-1.,-3.59852681775485));
#54569=CARTESIAN_POINT('Ctrl Pts',(2.09663642986631,1.,-3.59852681775485));
#54570=CARTESIAN_POINT('Ctrl Pts',(2.09018686331416,-1.,-3.59411228625588));
#54571=CARTESIAN_POINT('Ctrl Pts',(2.09018686331416,1.,-3.59411228625588));
#54572=CARTESIAN_POINT('Ctrl Pts',(2.08376373048756,-1.,-3.58967435355088));
#54573=CARTESIAN_POINT('Ctrl Pts',(2.08376373048756,1.,-3.58967435355088));
#54574=CARTESIAN_POINT('Ctrl Pts',(2.07736732842117,-1.,-3.58521300039299));
#54575=CARTESIAN_POINT('Ctrl Pts',(2.07736732842117,1.,-3.58521300039299));
#54576=CARTESIAN_POINT('Ctrl Pts',(2.07099797605747,-1.,-3.58072819250442));
#54577=CARTESIAN_POINT('Ctrl Pts',(2.07099797605747,1.,-3.58072819250442));
#54578=CARTESIAN_POINT('Ctrl Pts',(2.06465599229174,-1.,-3.576219862243));
#54579=CARTESIAN_POINT('Ctrl Pts',(2.06465599229174,1.,-3.576219862243));
#54580=CARTESIAN_POINT('Ctrl Pts',(2.05834167687523,-1.,-3.57168789423507));
#54581=CARTESIAN_POINT('Ctrl Pts',(2.05834167687523,1.,-3.57168789423507));
#54582=CARTESIAN_POINT('Ctrl Pts',(2.0520552817309,-1.,-3.56713209978208));
#54583=CARTESIAN_POINT('Ctrl Pts',(2.0520552817309,1.,-3.56713209978208));
#54584=CARTESIAN_POINT('Ctrl Pts',(2.04579702159056,-1.,-3.5625522387181));
#54585=CARTESIAN_POINT('Ctrl Pts',(2.04579702159056,1.,-3.5625522387181));
#54586=CARTESIAN_POINT('Ctrl Pts',(2.03956711120099,-1.,-3.55794807265052));
#54587=CARTESIAN_POINT('Ctrl Pts',(2.03956711120099,1.,-3.55794807265052));
#54588=CARTESIAN_POINT('Ctrl Pts',(2.03336579658174,-1.,-3.55331941294018));
#54589=CARTESIAN_POINT('Ctrl Pts',(2.03336579658174,1.,-3.55331941294018));
#54590=CARTESIAN_POINT('Ctrl Pts',(2.02719338376144,-1.,-3.54866616282173));
#54591=CARTESIAN_POINT('Ctrl Pts',(2.02719338376144,1.,-3.54866616282173));
#54592=CARTESIAN_POINT('Ctrl Pts',(2.0210502798303,-1.,-3.54398838254011));
#54593=CARTESIAN_POINT('Ctrl Pts',(2.0210502798303,1.,-3.54398838254011));
#54594=CARTESIAN_POINT('Ctrl Pts',(2.0149369884727,-1.,-3.53928627453503));
#54595=CARTESIAN_POINT('Ctrl Pts',(2.0149369884727,1.,-3.53928627453503));
#54596=CARTESIAN_POINT('Ctrl Pts',(2.00885403604685,-1.,-3.53456004727321));
#54597=CARTESIAN_POINT('Ctrl Pts',(2.00885403604685,1.,-3.53456004727321));
#54598=CARTESIAN_POINT('Ctrl Pts',(2.00280191090341,-1.,-3.52980980250181));
#54599=CARTESIAN_POINT('Ctrl Pts',(2.00280191090341,1.,-3.52980980250181));
#54600=CARTESIAN_POINT('Ctrl Pts',(1.99678100339305,-1.,-3.52503542491745));
#54601=CARTESIAN_POINT('Ctrl Pts',(1.99678100339305,1.,-3.52503542491745));
#54602=CARTESIAN_POINT('Ctrl Pts',(1.99079153006143,-1.,-3.52023644289195));
#54603=CARTESIAN_POINT('Ctrl Pts',(1.99079153006143,1.,-3.52023644289195));
#54604=CARTESIAN_POINT('Ctrl Pts',(1.98483351061066,-1.,-3.51541198728362));
#54605=CARTESIAN_POINT('Ctrl Pts',(1.98483351061066,1.,-3.51541198728362));
#54606=CARTESIAN_POINT('Ctrl Pts',(1.97890693666316,-1.,-3.51056110478334));
#54607=CARTESIAN_POINT('Ctrl Pts',(1.97890693666316,1.,-3.51056110478334));
#54608=CARTESIAN_POINT('Ctrl Pts',(1.9730119116298,-1.,-3.505683018611));
#54609=CARTESIAN_POINT('Ctrl Pts',(1.9730119116298,1.,-3.505683018611));
#54610=CARTESIAN_POINT('Ctrl Pts',(1.9671487972405,-1.,-3.50077740176262));
#54611=CARTESIAN_POINT('Ctrl Pts',(1.9671487972405,1.,-3.50077740176262));
#54612=CARTESIAN_POINT('Ctrl Pts',(1.96131836776489,-1.,-3.49584466573045));
#54613=CARTESIAN_POINT('Ctrl Pts',(1.96131836776489,1.,-3.49584466573045));
#54614=CARTESIAN_POINT('Ctrl Pts',(1.95552193112071,-1.,-3.49088618670967));
#54615=CARTESIAN_POINT('Ctrl Pts',(1.95552193112071,1.,-3.49088618670967));
#54616=CARTESIAN_POINT('Ctrl Pts',(1.94976096795902,-1.,-3.485903616108));
#54617=CARTESIAN_POINT('Ctrl Pts',(1.94976096795902,1.,-3.485903616108));
#54618=CARTESIAN_POINT('Ctrl Pts',(1.94403680554062,-1.,-3.48089825770412));
#54619=CARTESIAN_POINT('Ctrl Pts',(1.94403680554062,1.,-3.48089825770412));
#54620=CARTESIAN_POINT('Ctrl Pts',(1.93835026973888,-1.,-3.47587040389916));
#54621=CARTESIAN_POINT('Ctrl Pts',(1.93835026973888,1.,-3.47587040389916));
#54622=CARTESIAN_POINT('Ctrl Pts',(1.93270136427083,-1.,-3.47081872409783));
#54623=CARTESIAN_POINT('Ctrl Pts',(1.93270136427083,1.,-3.47081872409783));
#54624=CARTESIAN_POINT('Ctrl Pts',(1.92708888591159,-1.,-3.46573953254084));
#54625=CARTESIAN_POINT('Ctrl Pts',(1.92708888591159,1.,-3.46573953254084));
#54626=CARTESIAN_POINT('Ctrl Pts',(1.9215111821321,-1.,-3.4606282172248));
#54627=CARTESIAN_POINT('Ctrl Pts',(1.9215111821321,1.,-3.4606282172248));
#54628=CARTESIAN_POINT('Ctrl Pts',(1.9159669478406,-1.,-3.45548074309943));
#54629=CARTESIAN_POINT('Ctrl Pts',(1.9159669478406,1.,-3.45548074309943));
#54630=CARTESIAN_POINT('Ctrl Pts',(1.91045605593638,-1.,-3.45029522038885));
#54631=CARTESIAN_POINT('Ctrl Pts',(1.91045605593638,1.,-3.45029522038885));
#54632=CARTESIAN_POINT('Ctrl Pts',(1.90498026502308,-1.,-3.44507323983374));
#54633=CARTESIAN_POINT('Ctrl Pts',(1.90498026502308,1.,-3.44507323983374));
#54634=CARTESIAN_POINT('Ctrl Pts',(1.89954426803392,-1.,-3.43982185678105));
#54635=CARTESIAN_POINT('Ctrl Pts',(1.89954426803392,1.,-3.43982185678105));
#54636=CARTESIAN_POINT('Ctrl Pts',(1.89415420002553,-1.,-3.43455074411591));
#54637=CARTESIAN_POINT('Ctrl Pts',(1.89415420002553,1.,-3.43455074411591));
#54638=CARTESIAN_POINT('Ctrl Pts',(1.88881571322018,-1.,-3.42926852222174));
#54639=CARTESIAN_POINT('Ctrl Pts',(1.88881571322018,1.,-3.42926852222174));
#54640=CARTESIAN_POINT('Ctrl Pts',(1.88353205062063,-1.,-3.42397908819741));
#54641=CARTESIAN_POINT('Ctrl Pts',(1.88353205062063,1.,-3.42397908819741));
#54642=CARTESIAN_POINT('Ctrl Pts',(1.87830245689338,-1.,-3.4186785838376));
#54643=CARTESIAN_POINT('Ctrl Pts',(1.87830245689338,1.,-3.4186785838376));
#54644=CARTESIAN_POINT('Ctrl Pts',(1.87311957248106,-1.,-3.41335043875182));
#54645=CARTESIAN_POINT('Ctrl Pts',(1.87311957248106,1.,-3.41335043875182));
#54646=CARTESIAN_POINT('Ctrl Pts',(1.86797231196635,-1.,-3.40797080000513));
#54647=CARTESIAN_POINT('Ctrl Pts',(1.86797231196635,1.,-3.40797080000513));
#54648=CARTESIAN_POINT('Ctrl Pts',(1.86285057051228,-1.,-3.40251742305445));
#54649=CARTESIAN_POINT('Ctrl Pts',(1.86285057051228,1.,-3.40251742305445));
#54650=CARTESIAN_POINT('Ctrl Pts',(1.85774972037055,-1.,-3.39697816833056));
#54651=CARTESIAN_POINT('Ctrl Pts',(1.85774972037055,1.,-3.39697816833056));
#54652=CARTESIAN_POINT('Ctrl Pts',(1.85267433291778,-1.,-3.39135802549415));
#54653=CARTESIAN_POINT('Ctrl Pts',(1.85267433291778,1.,-3.39135802549415));
#54654=CARTESIAN_POINT('Ctrl Pts',(1.84764441927778,-1.,-3.38569092349639));
#54655=CARTESIAN_POINT('Ctrl Pts',(1.84764441927778,1.,-3.38569092349639));
#54656=CARTESIAN_POINT('Ctrl Pts',(1.84269016931679,-1.,-3.38002968341222));
#54657=CARTESIAN_POINT('Ctrl Pts',(1.84269016931679,1.,-3.38002968341222));
#54658=CARTESIAN_POINT('Ctrl Pts',(1.83784072967111,-1.,-3.37442462015914));
#54659=CARTESIAN_POINT('Ctrl Pts',(1.83784072967111,1.,-3.37442462015914));
#54660=CARTESIAN_POINT('Ctrl Pts',(1.83311391452338,-1.,-3.36890396271864));
#54661=CARTESIAN_POINT('Ctrl Pts',(1.83311391452338,1.,-3.36890396271864));
#54662=CARTESIAN_POINT('Ctrl Pts',(1.82850752153182,-1.,-3.36345722124127));
#54663=CARTESIAN_POINT('Ctrl Pts',(1.82850752153182,1.,-3.36345722124127));
#54664=CARTESIAN_POINT('Ctrl Pts',(1.82398496829247,-1.,-3.35800801557326));
#54665=CARTESIAN_POINT('Ctrl Pts',(1.82398496829247,1.,-3.35800801557326));
#54666=CARTESIAN_POINT('Ctrl Pts',(1.81948458796748,-1.,-3.35243086937451));
#54667=CARTESIAN_POINT('Ctrl Pts',(1.81948458796748,1.,-3.35243086937451));
#54668=CARTESIAN_POINT('Ctrl Pts',(1.81494618732772,-1.,-3.34660014370527));
#54669=CARTESIAN_POINT('Ctrl Pts',(1.81494618732772,1.,-3.34660014370527));
#54670=CARTESIAN_POINT('Ctrl Pts',(1.81033399625311,-1.,-3.34043216147532));
#54671=CARTESIAN_POINT('Ctrl Pts',(1.81033399625311,1.,-3.34043216147532));
#54672=CARTESIAN_POINT('Ctrl Pts',(1.80565802981138,-1.,-3.33392460276874));
#54673=CARTESIAN_POINT('Ctrl Pts',(1.80565802981138,1.,-3.33392460276874));
#54674=CARTESIAN_POINT('Ctrl Pts',(1.80100380443535,-1.,-3.3272108803981));
#54675=CARTESIAN_POINT('Ctrl Pts',(1.80100380443535,1.,-3.3272108803981));
#54676=CARTESIAN_POINT('Ctrl Pts',(1.79652817033444,-1.,-3.32055355101168));
#54677=CARTESIAN_POINT('Ctrl Pts',(1.79652817033444,1.,-3.32055355101168));
#54678=CARTESIAN_POINT('Ctrl Pts',(1.79242331350137,-1.,-3.31428038326763));
#54679=CARTESIAN_POINT('Ctrl Pts',(1.79242331350137,1.,-3.31428038326763));
#54680=CARTESIAN_POINT('Ctrl Pts',(1.78888832245965,-1.,-3.30873412266954));
#54681=CARTESIAN_POINT('Ctrl Pts',(1.78888832245965,1.,-3.30873412266954));
#54682=CARTESIAN_POINT('Ctrl Pts',(1.78610045419769,-1.,-3.30422155558973));
#54683=CARTESIAN_POINT('Ctrl Pts',(1.78610045419769,1.,-3.30422155558973));
#54684=CARTESIAN_POINT('Ctrl Pts',(1.78417972819696,-1.,-3.30095096463082));
#54685=CARTESIAN_POINT('Ctrl Pts',(1.78417972819696,1.,-3.30095096463082));
#54686=CARTESIAN_POINT('Ctrl Pts',(1.78338186555671,-1.,-3.29940631673818));
#54687=CARTESIAN_POINT('Ctrl Pts',(1.78338186555671,1.,-3.29940631673818));
#54688=CARTESIAN_POINT('Ctrl Pts',(1.78320756177191,-1.,-3.29886572077303));
#54689=CARTESIAN_POINT('Ctrl Pts',(1.78320756177191,1.,-3.29886572077303));
#54690=CARTESIAN_POINT('Ctrl Pts',(1.78327971836272,-1.,-3.29877974053191));
#54691=CARTESIAN_POINT('Ctrl Pts',(1.78327971836272,1.,-3.29877974053191));
#54692=CARTESIAN_POINT('Ctrl Pts',(1.7833628895577,-1.,-3.2988053601491));
#54693=CARTESIAN_POINT('Ctrl Pts',(1.7833628895577,1.,-3.2988053601491));
#54694=CARTESIAN_POINT('',(2.12928030988903,1.,-3.62024382630768));
#54695=CARTESIAN_POINT('Ctrl Pts',(2.12928030988903,1.,-3.62024382630768));
#54696=CARTESIAN_POINT('Ctrl Pts',(2.12796193131368,1.,-3.61938653649098));
#54697=CARTESIAN_POINT('Ctrl Pts',(2.12532774376758,1.,-3.61766963590482));
#54698=CARTESIAN_POINT('Ctrl Pts',(2.12138417126355,1.,-3.61508732216891));
#54699=CARTESIAN_POINT('Ctrl Pts',(2.11614149815106,1.,-3.61163030609447));
#54700=CARTESIAN_POINT('Ctrl Pts',(2.10961391334462,1.,-3.60728578532601));
#54701=CARTESIAN_POINT('Ctrl Pts',(2.1031121772821,1.,-3.60291797088734));
#54702=CARTESIAN_POINT('Ctrl Pts',(2.09663642986631,1.,-3.59852681775485));
#54703=CARTESIAN_POINT('Ctrl Pts',(2.09018686331416,1.,-3.59411228625588));
#54704=CARTESIAN_POINT('Ctrl Pts',(2.08376373048756,1.,-3.58967435355088));
#54705=CARTESIAN_POINT('Ctrl Pts',(2.07736732842117,1.,-3.58521300039299));
#54706=CARTESIAN_POINT('Ctrl Pts',(2.07099797605747,1.,-3.58072819250442));
#54707=CARTESIAN_POINT('Ctrl Pts',(2.06465599229174,1.,-3.576219862243));
#54708=CARTESIAN_POINT('Ctrl Pts',(2.05834167687523,1.,-3.57168789423507));
#54709=CARTESIAN_POINT('Ctrl Pts',(2.0520552817309,1.,-3.56713209978208));
#54710=CARTESIAN_POINT('Ctrl Pts',(2.04579702159056,1.,-3.5625522387181));
#54711=CARTESIAN_POINT('Ctrl Pts',(2.03956711120099,1.,-3.55794807265052));
#54712=CARTESIAN_POINT('Ctrl Pts',(2.03336579658174,1.,-3.55331941294018));
#54713=CARTESIAN_POINT('Ctrl Pts',(2.02719338376144,1.,-3.54866616282173));
#54714=CARTESIAN_POINT('Ctrl Pts',(2.0210502798303,1.,-3.54398838254011));
#54715=CARTESIAN_POINT('Ctrl Pts',(2.0149369884727,1.,-3.53928627453503));
#54716=CARTESIAN_POINT('Ctrl Pts',(2.00885403604685,1.,-3.53456004727321));
#54717=CARTESIAN_POINT('Ctrl Pts',(2.00280191090341,1.,-3.52980980250181));
#54718=CARTESIAN_POINT('Ctrl Pts',(1.99678100339305,1.,-3.52503542491745));
#54719=CARTESIAN_POINT('Ctrl Pts',(1.99079153006143,1.,-3.52023644289195));
#54720=CARTESIAN_POINT('Ctrl Pts',(1.98483351061066,1.,-3.51541198728362));
#54721=CARTESIAN_POINT('Ctrl Pts',(1.97890693666316,1.,-3.51056110478334));
#54722=CARTESIAN_POINT('Ctrl Pts',(1.9730119116298,1.,-3.505683018611));
#54723=CARTESIAN_POINT('Ctrl Pts',(1.9671487972405,1.,-3.50077740176262));
#54724=CARTESIAN_POINT('Ctrl Pts',(1.96131836776489,1.,-3.49584466573045));
#54725=CARTESIAN_POINT('Ctrl Pts',(1.95552193112071,1.,-3.49088618670967));
#54726=CARTESIAN_POINT('Ctrl Pts',(1.94976096795902,1.,-3.485903616108));
#54727=CARTESIAN_POINT('Ctrl Pts',(1.94403680554062,1.,-3.48089825770412));
#54728=CARTESIAN_POINT('Ctrl Pts',(1.93835026973888,1.,-3.47587040389916));
#54729=CARTESIAN_POINT('Ctrl Pts',(1.93270136427083,1.,-3.47081872409783));
#54730=CARTESIAN_POINT('Ctrl Pts',(1.92708888591159,1.,-3.46573953254084));
#54731=CARTESIAN_POINT('Ctrl Pts',(1.9215111821321,1.,-3.4606282172248));
#54732=CARTESIAN_POINT('Ctrl Pts',(1.9159669478406,1.,-3.45548074309943));
#54733=CARTESIAN_POINT('Ctrl Pts',(1.91045605593638,1.,-3.45029522038885));
#54734=CARTESIAN_POINT('Ctrl Pts',(1.90498026502308,1.,-3.44507323983374));
#54735=CARTESIAN_POINT('Ctrl Pts',(1.89954426803392,1.,-3.43982185678105));
#54736=CARTESIAN_POINT('Ctrl Pts',(1.89415420002553,1.,-3.43455074411591));
#54737=CARTESIAN_POINT('Ctrl Pts',(1.88881571322018,1.,-3.42926852222174));
#54738=CARTESIAN_POINT('Ctrl Pts',(1.88353205062063,1.,-3.42397908819741));
#54739=CARTESIAN_POINT('Ctrl Pts',(1.87830245689338,1.,-3.4186785838376));
#54740=CARTESIAN_POINT('Ctrl Pts',(1.87311957248106,1.,-3.41335043875182));
#54741=CARTESIAN_POINT('Ctrl Pts',(1.86797231196635,1.,-3.40797080000513));
#54742=CARTESIAN_POINT('Ctrl Pts',(1.86285057051228,1.,-3.40251742305445));
#54743=CARTESIAN_POINT('Ctrl Pts',(1.85774972037055,1.,-3.39697816833056));
#54744=CARTESIAN_POINT('Ctrl Pts',(1.85267433291778,1.,-3.39135802549415));
#54745=CARTESIAN_POINT('Ctrl Pts',(1.84764441927778,1.,-3.38569092349639));
#54746=CARTESIAN_POINT('Ctrl Pts',(1.84269016931679,1.,-3.38002968341222));
#54747=CARTESIAN_POINT('Ctrl Pts',(1.83784072967111,1.,-3.37442462015914));
#54748=CARTESIAN_POINT('Ctrl Pts',(1.83311391452338,1.,-3.36890396271864));
#54749=CARTESIAN_POINT('Ctrl Pts',(1.82850752153182,1.,-3.36345722124127));
#54750=CARTESIAN_POINT('Ctrl Pts',(1.82398496829247,1.,-3.35800801557326));
#54751=CARTESIAN_POINT('Ctrl Pts',(1.81948458796748,1.,-3.35243086937451));
#54752=CARTESIAN_POINT('Ctrl Pts',(1.81494618732772,1.,-3.34660014370527));
#54753=CARTESIAN_POINT('Ctrl Pts',(1.81033399625311,1.,-3.34043216147532));
#54754=CARTESIAN_POINT('Ctrl Pts',(1.80565802981138,1.,-3.33392460276874));
#54755=CARTESIAN_POINT('Ctrl Pts',(1.80100380443535,1.,-3.3272108803981));
#54756=CARTESIAN_POINT('Ctrl Pts',(1.79652817033444,1.,-3.32055355101168));
#54757=CARTESIAN_POINT('Ctrl Pts',(1.79242331350137,1.,-3.31428038326763));
#54758=CARTESIAN_POINT('Ctrl Pts',(1.78888832245965,1.,-3.30873412266954));
#54759=CARTESIAN_POINT('Ctrl Pts',(1.78610045419769,1.,-3.30422155558973));
#54760=CARTESIAN_POINT('Ctrl Pts',(1.7843238478823,1.,-3.30119637003466));
#54761=CARTESIAN_POINT('Ctrl Pts',(1.78353803106983,1.,-3.29970549824336));
#54762=CARTESIAN_POINT('Ctrl Pts',(1.78329283591903,1.,-3.29909749657945));
#54763=CARTESIAN_POINT('Ctrl Pts',(1.78326534445426,1.,-3.29890219175522));
#54764=CARTESIAN_POINT('Ctrl Pts',(1.78327315618183,1.,-3.29885386921599));
#54765=CARTESIAN_POINT('',(2.12928030988903,0.,-3.62024382630768));
#54766=CARTESIAN_POINT('Ctrl Pts',(2.12962728847314,-1.,-3.08661426358891));
#54767=CARTESIAN_POINT('Ctrl Pts',(2.12962728847314,1.,-3.08661426358891));
#54768=CARTESIAN_POINT('Ctrl Pts',(2.12964222016025,-1.,-3.08652852644995));
#54769=CARTESIAN_POINT('Ctrl Pts',(2.12964222016025,1.,-3.08652852644995));
#54770=CARTESIAN_POINT('Ctrl Pts',(2.12975158752407,-1.,-3.08650326867133));
#54771=CARTESIAN_POINT('Ctrl Pts',(2.12975158752407,1.,-3.08650326867133));
#54772=CARTESIAN_POINT('Ctrl Pts',(2.1301541297946,-1.,-3.08690399991464));
#54773=CARTESIAN_POINT('Ctrl Pts',(2.1301541297946,1.,-3.08690399991464));
#54774=CARTESIAN_POINT('Ctrl Pts',(2.13116819908542,-1.,-3.08831615620074));
#54775=CARTESIAN_POINT('Ctrl Pts',(2.13116819908542,1.,-3.08831615620074));
#54776=CARTESIAN_POINT('Ctrl Pts',(2.13321032560893,-1.,-3.09151235281963));
#54777=CARTESIAN_POINT('Ctrl Pts',(2.13321032560893,1.,-3.09151235281963));
#54778=CARTESIAN_POINT('Ctrl Pts',(2.13596538661048,-1.,-3.0960450242104));
#54779=CARTESIAN_POINT('Ctrl Pts',(2.13596538661048,1.,-3.0960450242104));
#54780=CARTESIAN_POINT('Ctrl Pts',(2.13930228863751,-1.,-3.10171267391049));
#54781=CARTESIAN_POINT('Ctrl Pts',(2.13930228863751,1.,-3.10171267391049));
#54782=CARTESIAN_POINT('Ctrl Pts',(2.14302815601973,-1.,-3.1082180866886));
#54783=CARTESIAN_POINT('Ctrl Pts',(2.14302815601973,1.,-3.1082180866886));
#54784=CARTESIAN_POINT('Ctrl Pts',(2.14692798457532,-1.,-3.11522827016855));
#54785=CARTESIAN_POINT('Ctrl Pts',(2.14692798457532,1.,-3.11522827016855));
#54786=CARTESIAN_POINT('Ctrl Pts',(2.15079698090584,-1.,-3.12242318151938));
#54787=CARTESIAN_POINT('Ctrl Pts',(2.15079698090584,1.,-3.12242318151938));
#54788=CARTESIAN_POINT('Ctrl Pts',(2.1544724138292,-1.,-3.12954386795646));
#54789=CARTESIAN_POINT('Ctrl Pts',(2.1544724138292,1.,-3.12954386795646));
#54790=CARTESIAN_POINT('Ctrl Pts',(2.15787423530676,-1.,-3.13645356563038));
#54791=CARTESIAN_POINT('Ctrl Pts',(2.15787423530676,1.,-3.13645356563038));
#54792=CARTESIAN_POINT('Ctrl Pts',(2.16100905914435,-1.,-3.14314440427022));
#54793=CARTESIAN_POINT('Ctrl Pts',(2.16100905914435,1.,-3.14314440427022));
#54794=CARTESIAN_POINT('Ctrl Pts',(2.16393520288072,-1.,-3.14968624389054));
#54795=CARTESIAN_POINT('Ctrl Pts',(2.16393520288072,1.,-3.14968624389054));
#54796=CARTESIAN_POINT('Ctrl Pts',(2.16673728447689,-1.,-3.15618975593656));
#54797=CARTESIAN_POINT('Ctrl Pts',(2.16673728447689,1.,-3.15618975593656));
#54798=CARTESIAN_POINT('Ctrl Pts',(2.16949910801219,-1.,-3.16276685102972));
#54799=CARTESIAN_POINT('Ctrl Pts',(2.16949910801219,1.,-3.16276685102972));
#54800=CARTESIAN_POINT('Ctrl Pts',(2.17227212063817,-1.,-3.16948480019497));
#54801=CARTESIAN_POINT('Ctrl Pts',(2.17227212063817,1.,-3.16948480019497));
#54802=CARTESIAN_POINT('Ctrl Pts',(2.17506466903694,-1.,-3.17635032802523));
#54803=CARTESIAN_POINT('Ctrl Pts',(2.17506466903694,1.,-3.17635032802523));
#54804=CARTESIAN_POINT('Ctrl Pts',(2.17785968847142,-1.,-3.18333474627807));
#54805=CARTESIAN_POINT('Ctrl Pts',(2.17785968847142,1.,-3.18333474627807));
#54806=CARTESIAN_POINT('Ctrl Pts',(2.18062558031778,-1.,-3.19038924261573));
#54807=CARTESIAN_POINT('Ctrl Pts',(2.18062558031778,1.,-3.19038924261573));
#54808=CARTESIAN_POINT('Ctrl Pts',(2.18332898656602,-1.,-3.19746293740411));
#54809=CARTESIAN_POINT('Ctrl Pts',(2.18332898656602,1.,-3.19746293740411));
#54810=CARTESIAN_POINT('Ctrl Pts',(2.18594876115934,-1.,-3.20452259717976));
#54811=CARTESIAN_POINT('Ctrl Pts',(2.18594876115934,1.,-3.20452259717976));
#54812=CARTESIAN_POINT('Ctrl Pts',(2.18848253363901,-1.,-3.21156188355769));
#54813=CARTESIAN_POINT('Ctrl Pts',(2.18848253363901,1.,-3.21156188355769));
#54814=CARTESIAN_POINT('Ctrl Pts',(2.19093901948667,-1.,-3.21859043114095));
#54815=CARTESIAN_POINT('Ctrl Pts',(2.19093901948667,1.,-3.21859043114095));
#54816=CARTESIAN_POINT('Ctrl Pts',(2.19333345123538,-1.,-3.22562734221646));
#54817=CARTESIAN_POINT('Ctrl Pts',(2.19333345123538,1.,-3.22562734221646));
#54818=CARTESIAN_POINT('Ctrl Pts',(2.19568204933168,-1.,-3.23269332296933));
#54819=CARTESIAN_POINT('Ctrl Pts',(2.19568204933168,1.,-3.23269332296933));
#54820=CARTESIAN_POINT('Ctrl Pts',(2.19799623693253,-1.,-3.23980245361308));
#54821=CARTESIAN_POINT('Ctrl Pts',(2.19799623693253,1.,-3.23980245361308));
#54822=CARTESIAN_POINT('Ctrl Pts',(2.20027910880981,-1.,-3.24695715874338));
#54823=CARTESIAN_POINT('Ctrl Pts',(2.20027910880981,1.,-3.24695715874338));
#54824=CARTESIAN_POINT('Ctrl Pts',(2.20252866491545,-1.,-3.25415277957775));
#54825=CARTESIAN_POINT('Ctrl Pts',(2.20252866491545,1.,-3.25415277957775));
#54826=CARTESIAN_POINT('Ctrl Pts',(2.20473979048678,-1.,-3.26138036637705));
#54827=CARTESIAN_POINT('Ctrl Pts',(2.20473979048678,1.,-3.26138036637705));
#54828=CARTESIAN_POINT('Ctrl Pts',(2.20690665217742,-1.,-3.26863006136782));
#54829=CARTESIAN_POINT('Ctrl Pts',(2.20690665217742,1.,-3.26863006136782));
#54830=CARTESIAN_POINT('Ctrl Pts',(2.2090250941743,-1.,-3.2758944800554));
#54831=CARTESIAN_POINT('Ctrl Pts',(2.2090250941743,1.,-3.2758944800554));
#54832=CARTESIAN_POINT('Ctrl Pts',(2.21109449750641,-1.,-3.28317133333131));
#54833=CARTESIAN_POINT('Ctrl Pts',(2.21109449750641,1.,-3.28317133333131));
#54834=CARTESIAN_POINT('Ctrl Pts',(2.21311648827391,-1.,-3.29046159238343));
#54835=CARTESIAN_POINT('Ctrl Pts',(2.21311648827391,1.,-3.29046159238343));
#54836=CARTESIAN_POINT('Ctrl Pts',(2.21509406923368,-1.,-3.29776825193159));
#54837=CARTESIAN_POINT('Ctrl Pts',(2.21509406923368,1.,-3.29776825193159));
#54838=CARTESIAN_POINT('Ctrl Pts',(2.21703059947836,-1.,-3.30509487819569));
#54839=CARTESIAN_POINT('Ctrl Pts',(2.21703059947836,1.,-3.30509487819569));
#54840=CARTESIAN_POINT('Ctrl Pts',(2.21892881679086,-1.,-3.31244421655666));
#54841=CARTESIAN_POINT('Ctrl Pts',(2.21892881679086,1.,-3.31244421655666));
#54842=CARTESIAN_POINT('Ctrl Pts',(2.22078990842776,-1.,-3.31981686778022));
#54843=CARTESIAN_POINT('Ctrl Pts',(2.22078990842776,1.,-3.31981686778022));
#54844=CARTESIAN_POINT('Ctrl Pts',(2.22261398879635,-1.,-3.3272119632604));
#54845=CARTESIAN_POINT('Ctrl Pts',(2.22261398879635,1.,-3.3272119632604));
#54846=CARTESIAN_POINT('Ctrl Pts',(2.22440049878511,-1.,-3.33462772849598));
#54847=CARTESIAN_POINT('Ctrl Pts',(2.22440049878511,1.,-3.33462772849598));
#54848=CARTESIAN_POINT('Ctrl Pts',(2.22614863918047,-1.,-3.34206209449375));
#54849=CARTESIAN_POINT('Ctrl Pts',(2.22614863918047,1.,-3.34206209449375));
#54850=CARTESIAN_POINT('Ctrl Pts',(2.22785777756576,-1.,-3.34951327111096));
#54851=CARTESIAN_POINT('Ctrl Pts',(2.22785777756576,1.,-3.34951327111096));
#54852=CARTESIAN_POINT('Ctrl Pts',(2.22952789880982,-1.,-3.35698038165483));
#54853=CARTESIAN_POINT('Ctrl Pts',(2.22952789880982,1.,-3.35698038165483));
#54854=CARTESIAN_POINT('Ctrl Pts',(2.23115945849739,-1.,-3.36446325227848));
#54855=CARTESIAN_POINT('Ctrl Pts',(2.23115945849739,1.,-3.36446325227848));
#54856=CARTESIAN_POINT('Ctrl Pts',(2.23275319569221,-1.,-3.37196214349304));
#54857=CARTESIAN_POINT('Ctrl Pts',(2.23275319569221,1.,-3.37196214349304));
#54858=CARTESIAN_POINT('Ctrl Pts',(2.23430995599561,-1.,-3.37947749555632));
#54859=CARTESIAN_POINT('Ctrl Pts',(2.23430995599561,1.,-3.37947749555632));
#54860=CARTESIAN_POINT('Ctrl Pts',(2.23583052276308,-1.,-3.38700968549563));
#54861=CARTESIAN_POINT('Ctrl Pts',(2.23583052276308,1.,-3.38700968549563));
#54862=CARTESIAN_POINT('Ctrl Pts',(2.23731541452791,-1.,-3.39455873448189));
#54863=CARTESIAN_POINT('Ctrl Pts',(2.23731541452791,1.,-3.39455873448189));
#54864=CARTESIAN_POINT('Ctrl Pts',(2.2387649112415,-1.,-3.40212434705647));
#54865=CARTESIAN_POINT('Ctrl Pts',(2.2387649112415,1.,-3.40212434705647));
#54866=CARTESIAN_POINT('Ctrl Pts',(2.24017914395289,-1.,-3.40970604190328));
#54867=CARTESIAN_POINT('Ctrl Pts',(2.24017914395289,1.,-3.40970604190328));
#54868=CARTESIAN_POINT('Ctrl Pts',(2.24155816587844,-1.,-3.41730325539172));
#54869=CARTESIAN_POINT('Ctrl Pts',(2.24155816587844,1.,-3.41730325539172));
#54870=CARTESIAN_POINT('Ctrl Pts',(2.24290202531101,-1.,-3.42491544683008));
#54871=CARTESIAN_POINT('Ctrl Pts',(2.24290202531101,1.,-3.42491544683008));
#54872=CARTESIAN_POINT('Ctrl Pts',(2.24421085338727,-1.,-3.43254222614803));
#54873=CARTESIAN_POINT('Ctrl Pts',(2.24421085338727,1.,-3.43254222614803));
#54874=CARTESIAN_POINT('Ctrl Pts',(2.24548487526022,-1.,-3.4401833646032));
#54875=CARTESIAN_POINT('Ctrl Pts',(2.24548487526022,1.,-3.4401833646032));
#54876=CARTESIAN_POINT('Ctrl Pts',(2.2467243706995,-1.,-3.44783872863151));
#54877=CARTESIAN_POINT('Ctrl Pts',(2.2467243706995,1.,-3.44783872863151));
#54878=CARTESIAN_POINT('Ctrl Pts',(2.2479296496077,-1.,-3.45550823512049));
#54879=CARTESIAN_POINT('Ctrl Pts',(2.2479296496077,1.,-3.45550823512049));
#54880=CARTESIAN_POINT('Ctrl Pts',(2.2491010234604,-1.,-3.46319180177573));
#54881=CARTESIAN_POINT('Ctrl Pts',(2.2491010234604,1.,-3.46319180177573));
#54882=CARTESIAN_POINT('Ctrl Pts',(2.25023877475942,-1.,-3.47088928979889));
#54883=CARTESIAN_POINT('Ctrl Pts',(2.25023877475942,1.,-3.47088928979889));
#54884=CARTESIAN_POINT('Ctrl Pts',(2.25134314238687,-1.,-3.47860048448691));
#54885=CARTESIAN_POINT('Ctrl Pts',(2.25134314238687,1.,-3.47860048448691));
#54886=CARTESIAN_POINT('Ctrl Pts',(2.25241433138695,-1.,-3.48632513240961));
#54887=CARTESIAN_POINT('Ctrl Pts',(2.25241433138695,1.,-3.48632513240961));
#54888=CARTESIAN_POINT('Ctrl Pts',(2.25345251709759,-1.,-3.49406296494791));
#54889=CARTESIAN_POINT('Ctrl Pts',(2.25345251709759,1.,-3.49406296494791));
#54890=CARTESIAN_POINT('Ctrl Pts',(2.25445785151868,-1.,-3.50181372617971));
#54891=CARTESIAN_POINT('Ctrl Pts',(2.25445785151868,1.,-3.50181372617971));
#54892=CARTESIAN_POINT('Ctrl Pts',(2.25543046979799,-1.,-3.50957720117341));
#54893=CARTESIAN_POINT('Ctrl Pts',(2.25543046979799,1.,-3.50957720117341));
#54894=CARTESIAN_POINT('Ctrl Pts',(2.25637049455044,-1.,-3.51735323667612));
#54895=CARTESIAN_POINT('Ctrl Pts',(2.25637049455044,1.,-3.51735323667612));
#54896=CARTESIAN_POINT('Ctrl Pts',(2.25727802940898,-1.,-3.52514172847711));
#54897=CARTESIAN_POINT('Ctrl Pts',(2.25727802940898,1.,-3.52514172847711));
#54898=CARTESIAN_POINT('Ctrl Pts',(2.25797812950104,-1.,-3.53138243688262));
#54899=CARTESIAN_POINT('Ctrl Pts',(2.25797812950104,1.,-3.53138243688262));
#54900=CARTESIAN_POINT('Ctrl Pts',(2.25848864343951,-1.,-3.53606853162228));
#54901=CARTESIAN_POINT('Ctrl Pts',(2.25848864343951,1.,-3.53606853162228));
#54902=CARTESIAN_POINT('Ctrl Pts',(2.2588225169468,-1.,-3.53919506647335));
#54903=CARTESIAN_POINT('Ctrl Pts',(2.2588225169468,1.,-3.53919506647335));
#54904=CARTESIAN_POINT('Ctrl Pts',(2.25898783642071,-1.,-3.54075895182139));
#54905=CARTESIAN_POINT('Ctrl Pts',(2.25898783642071,1.,-3.54075895182139));
#54906=CARTESIAN_POINT('',(2.1297112484669,1.,-3.08655633322212));
#54907=CARTESIAN_POINT('Ctrl Pts',(2.1297112484669,-1.,-3.08655633322212));
#54908=CARTESIAN_POINT('Ctrl Pts',(2.1297112484669,-0.666666666666667,-3.08655633322212));
#54909=CARTESIAN_POINT('Ctrl Pts',(2.1297112484669,-0.333333333333333,-3.08655633322212));
#54910=CARTESIAN_POINT('Ctrl Pts',(2.1297112484669,0.333333333333333,-3.08655633322212));
#54911=CARTESIAN_POINT('Ctrl Pts',(2.1297112484669,0.666666666666667,-3.08655633322212));
#54912=CARTESIAN_POINT('Ctrl Pts',(2.1297112484669,1.,-3.08655633322212));
#54913=CARTESIAN_POINT('',(2.25898783642071,1.,-3.54075895182139));
#54914=CARTESIAN_POINT('',(2.25898783642071,0.,-3.54075895182139));
#54915=CARTESIAN_POINT('Ctrl Pts',(2.1297112484669,1.,-3.08655633322212));
#54916=CARTESIAN_POINT('Ctrl Pts',(2.1297578506149,1.,-3.08657131089497));
#54917=CARTESIAN_POINT('Ctrl Pts',(2.12991938762373,1.,-3.08668447250322));
#54918=CARTESIAN_POINT('Ctrl Pts',(2.13034980480424,1.,-3.08717896996098));
#54919=CARTESIAN_POINT('Ctrl Pts',(2.13132142793017,1.,-3.08855597949761));
#54920=CARTESIAN_POINT('Ctrl Pts',(2.13321032560893,1.,-3.09151235281963));
#54921=CARTESIAN_POINT('Ctrl Pts',(2.13596538661048,1.,-3.0960450242104));
#54922=CARTESIAN_POINT('Ctrl Pts',(2.13930228863751,1.,-3.10171267391049));
#54923=CARTESIAN_POINT('Ctrl Pts',(2.14302815601973,1.,-3.1082180866886));
#54924=CARTESIAN_POINT('Ctrl Pts',(2.14692798457532,1.,-3.11522827016855));
#54925=CARTESIAN_POINT('Ctrl Pts',(2.15079698090584,1.,-3.12242318151938));
#54926=CARTESIAN_POINT('Ctrl Pts',(2.1544724138292,1.,-3.12954386795646));
#54927=CARTESIAN_POINT('Ctrl Pts',(2.15787423530676,1.,-3.13645356563038));
#54928=CARTESIAN_POINT('Ctrl Pts',(2.16100905914435,1.,-3.14314440427022));
#54929=CARTESIAN_POINT('Ctrl Pts',(2.16393520288072,1.,-3.14968624389054));
#54930=CARTESIAN_POINT('Ctrl Pts',(2.16673728447689,1.,-3.15618975593656));
#54931=CARTESIAN_POINT('Ctrl Pts',(2.16949910801219,1.,-3.16276685102972));
#54932=CARTESIAN_POINT('Ctrl Pts',(2.17227212063817,1.,-3.16948480019497));
#54933=CARTESIAN_POINT('Ctrl Pts',(2.17506466903694,1.,-3.17635032802523));
#54934=CARTESIAN_POINT('Ctrl Pts',(2.17785968847142,1.,-3.18333474627807));
#54935=CARTESIAN_POINT('Ctrl Pts',(2.18062558031778,1.,-3.19038924261573));
#54936=CARTESIAN_POINT('Ctrl Pts',(2.18332898656602,1.,-3.19746293740411));
#54937=CARTESIAN_POINT('Ctrl Pts',(2.18594876115934,1.,-3.20452259717976));
#54938=CARTESIAN_POINT('Ctrl Pts',(2.18848253363901,1.,-3.21156188355769));
#54939=CARTESIAN_POINT('Ctrl Pts',(2.19093901948667,1.,-3.21859043114095));
#54940=CARTESIAN_POINT('Ctrl Pts',(2.19333345123538,1.,-3.22562734221646));
#54941=CARTESIAN_POINT('Ctrl Pts',(2.19568204933168,1.,-3.23269332296933));
#54942=CARTESIAN_POINT('Ctrl Pts',(2.19799623693253,1.,-3.23980245361308));
#54943=CARTESIAN_POINT('Ctrl Pts',(2.20027910880981,1.,-3.24695715874338));
#54944=CARTESIAN_POINT('Ctrl Pts',(2.20252866491545,1.,-3.25415277957775));
#54945=CARTESIAN_POINT('Ctrl Pts',(2.20473979048678,1.,-3.26138036637705));
#54946=CARTESIAN_POINT('Ctrl Pts',(2.20690665217742,1.,-3.26863006136782));
#54947=CARTESIAN_POINT('Ctrl Pts',(2.2090250941743,1.,-3.2758944800554));
#54948=CARTESIAN_POINT('Ctrl Pts',(2.21109449750641,1.,-3.28317133333131));
#54949=CARTESIAN_POINT('Ctrl Pts',(2.21311648827391,1.,-3.29046159238343));
#54950=CARTESIAN_POINT('Ctrl Pts',(2.21509406923368,1.,-3.29776825193159));
#54951=CARTESIAN_POINT('Ctrl Pts',(2.21703059947836,1.,-3.30509487819569));
#54952=CARTESIAN_POINT('Ctrl Pts',(2.21892881679086,1.,-3.31244421655666));
#54953=CARTESIAN_POINT('Ctrl Pts',(2.22078990842776,1.,-3.31981686778022));
#54954=CARTESIAN_POINT('Ctrl Pts',(2.22261398879635,1.,-3.3272119632604));
#54955=CARTESIAN_POINT('Ctrl Pts',(2.22440049878511,1.,-3.33462772849598));
#54956=CARTESIAN_POINT('Ctrl Pts',(2.22614863918047,1.,-3.34206209449375));
#54957=CARTESIAN_POINT('Ctrl Pts',(2.22785777756576,1.,-3.34951327111096));
#54958=CARTESIAN_POINT('Ctrl Pts',(2.22952789880982,1.,-3.35698038165483));
#54959=CARTESIAN_POINT('Ctrl Pts',(2.23115945849739,1.,-3.36446325227848));
#54960=CARTESIAN_POINT('Ctrl Pts',(2.23275319569221,1.,-3.37196214349304));
#54961=CARTESIAN_POINT('Ctrl Pts',(2.23430995599561,1.,-3.37947749555632));
#54962=CARTESIAN_POINT('Ctrl Pts',(2.23583052276308,1.,-3.38700968549563));
#54963=CARTESIAN_POINT('Ctrl Pts',(2.23731541452791,1.,-3.39455873448189));
#54964=CARTESIAN_POINT('Ctrl Pts',(2.2387649112415,1.,-3.40212434705647));
#54965=CARTESIAN_POINT('Ctrl Pts',(2.24017914395289,1.,-3.40970604190328));
#54966=CARTESIAN_POINT('Ctrl Pts',(2.24155816587844,1.,-3.41730325539172));
#54967=CARTESIAN_POINT('Ctrl Pts',(2.24290202531101,1.,-3.42491544683008));
#54968=CARTESIAN_POINT('Ctrl Pts',(2.24421085338727,1.,-3.43254222614803));
#54969=CARTESIAN_POINT('Ctrl Pts',(2.24548487526022,1.,-3.4401833646032));
#54970=CARTESIAN_POINT('Ctrl Pts',(2.2467243706995,1.,-3.44783872863151));
#54971=CARTESIAN_POINT('Ctrl Pts',(2.2479296496077,1.,-3.45550823512049));
#54972=CARTESIAN_POINT('Ctrl Pts',(2.2491010234604,1.,-3.46319180177573));
#54973=CARTESIAN_POINT('Ctrl Pts',(2.25023877475942,1.,-3.47088928979889));
#54974=CARTESIAN_POINT('Ctrl Pts',(2.25134314238687,1.,-3.47860048448691));
#54975=CARTESIAN_POINT('Ctrl Pts',(2.25241433138695,1.,-3.48632513240961));
#54976=CARTESIAN_POINT('Ctrl Pts',(2.25345251709759,1.,-3.49406296494791));
#54977=CARTESIAN_POINT('Ctrl Pts',(2.25445785151868,1.,-3.50181372617971));
#54978=CARTESIAN_POINT('Ctrl Pts',(2.25543046979799,1.,-3.50957720117341));
#54979=CARTESIAN_POINT('Ctrl Pts',(2.25637049455044,1.,-3.51735323667612));
#54980=CARTESIAN_POINT('Ctrl Pts',(2.25727802940898,1.,-3.52514172847711));
#54981=CARTESIAN_POINT('Ctrl Pts',(2.25797812950104,1.,-3.53138243688262));
#54982=CARTESIAN_POINT('Ctrl Pts',(2.25848864343951,1.,-3.53606853162228));
#54983=CARTESIAN_POINT('Ctrl Pts',(2.2588225169468,1.,-3.53919506647335));
#54984=CARTESIAN_POINT('Ctrl Pts',(2.25898783642071,1.,-3.54075895182139));
#54985=CARTESIAN_POINT('Origin',(2.25898783642071,0.,-3.54075895182139));
#54986=CARTESIAN_POINT('',(2.12928030988903,1.,-3.62024382630768));
#54987=CARTESIAN_POINT('Origin',(0.,0.,0.));
#54988=CARTESIAN_POINT('',(2.27737254473378,1.,-2.97927412174388));
#54989=CARTESIAN_POINT('Origin',(0.,1.,0.));
#54990=CARTESIAN_POINT('Ctrl Pts',(2.27737254473378,1.,-2.97927412174388));
#54991=CARTESIAN_POINT('Ctrl Pts',(2.27737254473378,0.666666666666667,-2.97927412174388));
#54992=CARTESIAN_POINT('Ctrl Pts',(2.27737254473378,0.333333333333333,-2.97927412174388));
#54993=CARTESIAN_POINT('Ctrl Pts',(2.27737254473378,-0.333333333333333,
-2.97927412174388));
#54994=CARTESIAN_POINT('Ctrl Pts',(2.27737254473378,-0.666666666666667,
-2.97927412174388));
#54995=CARTESIAN_POINT('Ctrl Pts',(2.27737254473378,-1.,-2.97927412174388));
#54996=CARTESIAN_POINT('Ctrl Pts',(2.66939624221984,-1.,-3.24257979115744));
#54997=CARTESIAN_POINT('Ctrl Pts',(2.66939624221984,1.,-3.24257979115744));
#54998=CARTESIAN_POINT('Ctrl Pts',(2.66795998539861,-1.,-3.24193929584813));
#54999=CARTESIAN_POINT('Ctrl Pts',(2.66795998539861,1.,-3.24193929584813));
#55000=CARTESIAN_POINT('Ctrl Pts',(2.66508964664767,-1.,-3.24065561087681));
#55001=CARTESIAN_POINT('Ctrl Pts',(2.66508964664767,1.,-3.24065561087681));
#55002=CARTESIAN_POINT('Ctrl Pts',(2.6607906631973,-1.,-3.23872200036311));
#55003=CARTESIAN_POINT('Ctrl Pts',(2.6607906631973,1.,-3.23872200036311));
#55004=CARTESIAN_POINT('Ctrl Pts',(2.6550717396303,-1.,-3.23612768065687));
#55005=CARTESIAN_POINT('Ctrl Pts',(2.6550717396303,1.,-3.23612768065687));
#55006=CARTESIAN_POINT('Ctrl Pts',(2.64794488744246,-1.,-3.23285778738558));
#55007=CARTESIAN_POINT('Ctrl Pts',(2.64794488744246,1.,-3.23285778738558));
#55008=CARTESIAN_POINT('Ctrl Pts',(2.64083992182478,-1.,-3.2295608435934));
#55009=CARTESIAN_POINT('Ctrl Pts',(2.64083992182478,1.,-3.2295608435934));
#55010=CARTESIAN_POINT('Ctrl Pts',(2.63375697391438,-1.,-3.22623678292539));
#55011=CARTESIAN_POINT('Ctrl Pts',(2.63375697391438,1.,-3.22623678292539));
#55012=CARTESIAN_POINT('Ctrl Pts',(2.62669622735548,-1.,-3.222885536128));
#55013=CARTESIAN_POINT('Ctrl Pts',(2.62669622735548,1.,-3.222885536128));
#55014=CARTESIAN_POINT('Ctrl Pts',(2.61965792832396,-1.,-3.21950704108654));
#55015=CARTESIAN_POINT('Ctrl Pts',(2.61965792832396,1.,-3.21950704108654));
#55016=CARTESIAN_POINT('Ctrl Pts',(2.61264236718662,-1.,-3.21610123232465));
#55017=CARTESIAN_POINT('Ctrl Pts',(2.61264236718662,1.,-3.21610123232465));
#55018=CARTESIAN_POINT('Ctrl Pts',(2.60564985359699,-1.,-3.21266802609297));
#55019=CARTESIAN_POINT('Ctrl Pts',(2.60564985359699,1.,-3.21266802609297));
#55020=CARTESIAN_POINT('Ctrl Pts',(2.59868069194267,-1.,-3.2092073056959));
#55021=CARTESIAN_POINT('Ctrl Pts',(2.59868069194267,1.,-3.2092073056959));
#55022=CARTESIAN_POINT('Ctrl Pts',(2.59173516023605,-1.,-3.20571891028879));
#55023=CARTESIAN_POINT('Ctrl Pts',(2.59173516023605,1.,-3.20571891028879));
#55024=CARTESIAN_POINT('Ctrl Pts',(2.58481347777953,-1.,-3.20220261408685));
#55025=CARTESIAN_POINT('Ctrl Pts',(2.58481347777953,1.,-3.20220261408685));
#55026=CARTESIAN_POINT('Ctrl Pts',(2.577915819091,-1.,-3.19865814628955));
#55027=CARTESIAN_POINT('Ctrl Pts',(2.577915819091,1.,-3.19865814628955));
#55028=CARTESIAN_POINT('Ctrl Pts',(2.57104235898053,-1.,-3.19508523784548));
#55029=CARTESIAN_POINT('Ctrl Pts',(2.57104235898053,1.,-3.19508523784548));
#55030=CARTESIAN_POINT('Ctrl Pts',(2.56419331092909,-1.,-3.19148366395201));
#55031=CARTESIAN_POINT('Ctrl Pts',(2.56419331092909,1.,-3.19148366395201));
#55032=CARTESIAN_POINT('Ctrl Pts',(2.55736896206016,-1.,-3.1878532811617));
#55033=CARTESIAN_POINT('Ctrl Pts',(2.55736896206016,1.,-3.1878532811617));
#55034=CARTESIAN_POINT('Ctrl Pts',(2.55056972387638,-1.,-3.18419408529482));
#55035=CARTESIAN_POINT('Ctrl Pts',(2.55056972387638,1.,-3.18419408529482));
#55036=CARTESIAN_POINT('Ctrl Pts',(2.54379612552948,-1.,-3.18050619750515));
#55037=CARTESIAN_POINT('Ctrl Pts',(2.54379612552948,1.,-3.18050619750515));
#55038=CARTESIAN_POINT('Ctrl Pts',(2.53704871950871,-1.,-3.17678974135225));
#55039=CARTESIAN_POINT('Ctrl Pts',(2.53704871950871,1.,-3.17678974135225));
#55040=CARTESIAN_POINT('Ctrl Pts',(2.5303280040691,-1.,-3.17304474093574));
#55041=CARTESIAN_POINT('Ctrl Pts',(2.5303280040691,1.,-3.17304474093574));
#55042=CARTESIAN_POINT('Ctrl Pts',(2.523634346718,-1.,-3.16927102130751));
#55043=CARTESIAN_POINT('Ctrl Pts',(2.523634346718,1.,-3.16927102130751));
#55044=CARTESIAN_POINT('Ctrl Pts',(2.51696788755615,-1.,-3.16546808277069));
#55045=CARTESIAN_POINT('Ctrl Pts',(2.51696788755615,1.,-3.16546808277069));
#55046=CARTESIAN_POINT('Ctrl Pts',(2.51032851007939,-1.,-3.16163506380211));
#55047=CARTESIAN_POINT('Ctrl Pts',(2.51032851007939,1.,-3.16163506380211));
#55048=CARTESIAN_POINT('Ctrl Pts',(2.50371605688287,-1.,-3.15777102413998));
#55049=CARTESIAN_POINT('Ctrl Pts',(2.50371605688287,1.,-3.15777102413998));
#55050=CARTESIAN_POINT('Ctrl Pts',(2.49713050858911,-1.,-3.15387518039064));
#55051=CARTESIAN_POINT('Ctrl Pts',(2.49713050858911,1.,-3.15387518039064));
#55052=CARTESIAN_POINT('Ctrl Pts',(2.49057217131985,-1.,-3.14994715298903));
#55053=CARTESIAN_POINT('Ctrl Pts',(2.49057217131985,1.,-3.14994715298903));
#55054=CARTESIAN_POINT('Ctrl Pts',(2.48404187418376,-1.,-3.1459872272388));
#55055=CARTESIAN_POINT('Ctrl Pts',(2.48404187418376,1.,-3.1459872272388));
#55056=CARTESIAN_POINT('Ctrl Pts',(2.47754112428027,-1.,-3.14199655778845));
#55057=CARTESIAN_POINT('Ctrl Pts',(2.47754112428027,1.,-3.14199655778845));
#55058=CARTESIAN_POINT('Ctrl Pts',(2.47107164236827,-1.,-3.13797654408931));
#55059=CARTESIAN_POINT('Ctrl Pts',(2.47107164236827,1.,-3.13797654408931));
#55060=CARTESIAN_POINT('Ctrl Pts',(2.4646349433237,-1.,-3.13392826623902));
#55061=CARTESIAN_POINT('Ctrl Pts',(2.4646349433237,1.,-3.13392826623902));
#55062=CARTESIAN_POINT('Ctrl Pts',(2.45823188859366,-1.,-3.12985188384372));
#55063=CARTESIAN_POINT('Ctrl Pts',(2.45823188859366,1.,-3.12985188384372));
#55064=CARTESIAN_POINT('Ctrl Pts',(2.45186227369848,-1.,-3.12574608210849));
#55065=CARTESIAN_POINT('Ctrl Pts',(2.45186227369848,1.,-3.12574608210849));
#55066=CARTESIAN_POINT('Ctrl Pts',(2.44552433364716,-1.,-3.12160740887768));
#55067=CARTESIAN_POINT('Ctrl Pts',(2.44552433364716,1.,-3.12160740887768));
#55068=CARTESIAN_POINT('Ctrl Pts',(2.43921571477975,-1.,-3.11743156744182));
#55069=CARTESIAN_POINT('Ctrl Pts',(2.43921571477975,1.,-3.11743156744182));
#55070=CARTESIAN_POINT('Ctrl Pts',(2.4329344968514,-1.,-3.11321477659012));
#55071=CARTESIAN_POINT('Ctrl Pts',(2.4329344968514,1.,-3.11321477659012));
#55072=CARTESIAN_POINT('Ctrl Pts',(2.42668025870013,-1.,-3.10895518969592));
#55073=CARTESIAN_POINT('Ctrl Pts',(2.42668025870013,1.,-3.10895518969592));
#55074=CARTESIAN_POINT('Ctrl Pts',(2.42045498612494,-1.,-3.10465410280902));
#55075=CARTESIAN_POINT('Ctrl Pts',(2.42045498612494,1.,-3.10465410280902));
#55076=CARTESIAN_POINT('Ctrl Pts',(2.41426441798067,-1.,-3.10031775027683));
#55077=CARTESIAN_POINT('Ctrl Pts',(2.41426441798067,1.,-3.10031775027683));
#55078=CARTESIAN_POINT('Ctrl Pts',(2.40811612696382,-1.,-3.09595472616093));
#55079=CARTESIAN_POINT('Ctrl Pts',(2.40811612696382,1.,-3.09595472616093));
#55080=CARTESIAN_POINT('Ctrl Pts',(2.40201704423352,-1.,-3.09157266051115));
#55081=CARTESIAN_POINT('Ctrl Pts',(2.40201704423352,1.,-3.09157266051115));
#55082=CARTESIAN_POINT('Ctrl Pts',(2.39597098250635,-1.,-3.08717489512919));
#55083=CARTESIAN_POINT('Ctrl Pts',(2.39597098250635,1.,-3.08717489512919));
#55084=CARTESIAN_POINT('Ctrl Pts',(2.38997659219192,-1.,-3.08275773747083));
#55085=CARTESIAN_POINT('Ctrl Pts',(2.38997659219192,1.,-3.08275773747083));
#55086=CARTESIAN_POINT('Ctrl Pts',(2.38402401216107,-1.,-3.07830597244301));
#55087=CARTESIAN_POINT('Ctrl Pts',(2.38402401216107,1.,-3.07830597244301));
#55088=CARTESIAN_POINT('Ctrl Pts',(2.37809856205524,-1.,-3.07379777492133));
#55089=CARTESIAN_POINT('Ctrl Pts',(2.37809856205524,1.,-3.07379777492133));
#55090=CARTESIAN_POINT('Ctrl Pts',(2.37218678163157,-1.,-3.06921275497472));
#55091=CARTESIAN_POINT('Ctrl Pts',(2.37218678163157,1.,-3.06921275497472));
#55092=CARTESIAN_POINT('Ctrl Pts',(2.36628220107001,-1.,-3.06453964643152));
#55093=CARTESIAN_POINT('Ctrl Pts',(2.36628220107001,1.,-3.06453964643152));
#55094=CARTESIAN_POINT('Ctrl Pts',(2.36039011602084,-1.,-3.05978266240056));
#55095=CARTESIAN_POINT('Ctrl Pts',(2.36039011602084,1.,-3.05978266240056));
#55096=CARTESIAN_POINT('Ctrl Pts',(2.35453559889506,-1.,-3.05497218368188));
#55097=CARTESIAN_POINT('Ctrl Pts',(2.35453559889506,1.,-3.05497218368188));
#55098=CARTESIAN_POINT('Ctrl Pts',(2.34875673090816,-1.,-3.05015565829976));
#55099=CARTESIAN_POINT('Ctrl Pts',(2.34875673090816,1.,-3.05015565829976));
#55100=CARTESIAN_POINT('Ctrl Pts',(2.3430901708402,-1.,-3.04537822217311));
#55101=CARTESIAN_POINT('Ctrl Pts',(2.3430901708402,1.,-3.04537822217311));
#55102=CARTESIAN_POINT('Ctrl Pts',(2.33755792953726,-1.,-3.04066496998569));
#55103=CARTESIAN_POINT('Ctrl Pts',(2.33755792953726,1.,-3.04066496998569));
#55104=CARTESIAN_POINT('Ctrl Pts',(2.33215619079807,-1.,-3.03600588555765));
#55105=CARTESIAN_POINT('Ctrl Pts',(2.33215619079807,1.,-3.03600588555765));
#55106=CARTESIAN_POINT('Ctrl Pts',(2.32683687412027,-1.,-3.03133125185047));
#55107=CARTESIAN_POINT('Ctrl Pts',(2.32683687412027,1.,-3.03133125185047));
#55108=CARTESIAN_POINT('Ctrl Pts',(2.32151944306299,-1.,-3.02652678416478));
#55109=CARTESIAN_POINT('Ctrl Pts',(2.32151944306299,1.,-3.02652678416478));
#55110=CARTESIAN_POINT('Ctrl Pts',(2.31612479121528,-1.,-3.02147780668029));
#55111=CARTESIAN_POINT('Ctrl Pts',(2.31612479121528,1.,-3.02147780668029));
#55112=CARTESIAN_POINT('Ctrl Pts',(2.31060449886577,-1.,-3.01610726819019));
#55113=CARTESIAN_POINT('Ctrl Pts',(2.31060449886577,1.,-3.01610726819019));
#55114=CARTESIAN_POINT('Ctrl Pts',(2.30496809486528,-1.,-3.01041131063882));
#55115=CARTESIAN_POINT('Ctrl Pts',(2.30496809486528,1.,-3.01041131063882));
#55116=CARTESIAN_POINT('Ctrl Pts',(2.29932091315939,-1.,-3.00450832658822));
#55117=CARTESIAN_POINT('Ctrl Pts',(2.29932091315939,1.,-3.00450832658822));
#55118=CARTESIAN_POINT('Ctrl Pts',(2.29385894577999,-1.,-2.99863310340004));
#55119=CARTESIAN_POINT('Ctrl Pts',(2.29385894577999,1.,-2.99863310340004));
#55120=CARTESIAN_POINT('Ctrl Pts',(2.28882328690601,-1.,-2.9930793098434));
#55121=CARTESIAN_POINT('Ctrl Pts',(2.28882328690601,1.,-2.9930793098434));
#55122=CARTESIAN_POINT('Ctrl Pts',(2.28446419116036,-1.,-2.98815432734929));
#55123=CARTESIAN_POINT('Ctrl Pts',(2.28446419116036,1.,-2.98815432734929));
#55124=CARTESIAN_POINT('Ctrl Pts',(2.28100472516582,-1.,-2.98413343613858));
#55125=CARTESIAN_POINT('Ctrl Pts',(2.28100472516582,1.,-2.98413343613858));
#55126=CARTESIAN_POINT('Ctrl Pts',(2.2785960133424,-1.,-2.98120357932601));
#55127=CARTESIAN_POINT('Ctrl Pts',(2.2785960133424,1.,-2.98120357932601));
#55128=CARTESIAN_POINT('Ctrl Pts',(2.27756633754846,-1.,-2.97980276182744));
#55129=CARTESIAN_POINT('Ctrl Pts',(2.27756633754846,1.,-2.97980276182744));
#55130=CARTESIAN_POINT('Ctrl Pts',(2.27730961189188,-1.,-2.97929608861502));
#55131=CARTESIAN_POINT('Ctrl Pts',(2.27730961189188,1.,-2.97929608861502));
#55132=CARTESIAN_POINT('Ctrl Pts',(2.2773674298423,-1.,-2.97919987915565));
#55133=CARTESIAN_POINT('Ctrl Pts',(2.2773674298423,1.,-2.97919987915565));
#55134=CARTESIAN_POINT('Ctrl Pts',(2.27745358485296,-1.,-2.97921217251145));
#55135=CARTESIAN_POINT('Ctrl Pts',(2.27745358485296,1.,-2.97921217251145));
#55136=CARTESIAN_POINT('',(2.66939624221984,1.,-3.24257979115744));
#55137=CARTESIAN_POINT('Ctrl Pts',(2.66939624221984,1.,-3.24257979115744));
#55138=CARTESIAN_POINT('Ctrl Pts',(2.66795998539861,1.,-3.24193929584813));
#55139=CARTESIAN_POINT('Ctrl Pts',(2.66508964664767,1.,-3.24065561087681));
#55140=CARTESIAN_POINT('Ctrl Pts',(2.6607906631973,1.,-3.23872200036311));
#55141=CARTESIAN_POINT('Ctrl Pts',(2.6550717396303,1.,-3.23612768065687));
#55142=CARTESIAN_POINT('Ctrl Pts',(2.64794488744246,1.,-3.23285778738558));
#55143=CARTESIAN_POINT('Ctrl Pts',(2.64083992182478,1.,-3.2295608435934));
#55144=CARTESIAN_POINT('Ctrl Pts',(2.63375697391438,1.,-3.22623678292539));
#55145=CARTESIAN_POINT('Ctrl Pts',(2.62669622735548,1.,-3.222885536128));
#55146=CARTESIAN_POINT('Ctrl Pts',(2.61965792832396,1.,-3.21950704108654));
#55147=CARTESIAN_POINT('Ctrl Pts',(2.61264236718662,1.,-3.21610123232465));
#55148=CARTESIAN_POINT('Ctrl Pts',(2.60564985359699,1.,-3.21266802609297));
#55149=CARTESIAN_POINT('Ctrl Pts',(2.59868069194267,1.,-3.2092073056959));
#55150=CARTESIAN_POINT('Ctrl Pts',(2.59173516023605,1.,-3.20571891028879));
#55151=CARTESIAN_POINT('Ctrl Pts',(2.58481347777953,1.,-3.20220261408685));
#55152=CARTESIAN_POINT('Ctrl Pts',(2.577915819091,1.,-3.19865814628955));
#55153=CARTESIAN_POINT('Ctrl Pts',(2.57104235898053,1.,-3.19508523784548));
#55154=CARTESIAN_POINT('Ctrl Pts',(2.56419331092909,1.,-3.19148366395201));
#55155=CARTESIAN_POINT('Ctrl Pts',(2.55736896206016,1.,-3.1878532811617));
#55156=CARTESIAN_POINT('Ctrl Pts',(2.55056972387638,1.,-3.18419408529482));
#55157=CARTESIAN_POINT('Ctrl Pts',(2.54379612552948,1.,-3.18050619750515));
#55158=CARTESIAN_POINT('Ctrl Pts',(2.53704871950871,1.,-3.17678974135225));
#55159=CARTESIAN_POINT('Ctrl Pts',(2.5303280040691,1.,-3.17304474093574));
#55160=CARTESIAN_POINT('Ctrl Pts',(2.523634346718,1.,-3.16927102130751));
#55161=CARTESIAN_POINT('Ctrl Pts',(2.51696788755615,1.,-3.16546808277069));
#55162=CARTESIAN_POINT('Ctrl Pts',(2.51032851007939,1.,-3.16163506380211));
#55163=CARTESIAN_POINT('Ctrl Pts',(2.50371605688287,1.,-3.15777102413998));
#55164=CARTESIAN_POINT('Ctrl Pts',(2.49713050858911,1.,-3.15387518039064));
#55165=CARTESIAN_POINT('Ctrl Pts',(2.49057217131985,1.,-3.14994715298903));
#55166=CARTESIAN_POINT('Ctrl Pts',(2.48404187418376,1.,-3.1459872272388));
#55167=CARTESIAN_POINT('Ctrl Pts',(2.47754112428027,1.,-3.14199655778845));
#55168=CARTESIAN_POINT('Ctrl Pts',(2.47107164236827,1.,-3.13797654408931));
#55169=CARTESIAN_POINT('Ctrl Pts',(2.4646349433237,1.,-3.13392826623902));
#55170=CARTESIAN_POINT('Ctrl Pts',(2.45823188859366,1.,-3.12985188384372));
#55171=CARTESIAN_POINT('Ctrl Pts',(2.45186227369848,1.,-3.12574608210849));
#55172=CARTESIAN_POINT('Ctrl Pts',(2.44552433364716,1.,-3.12160740887768));
#55173=CARTESIAN_POINT('Ctrl Pts',(2.43921571477975,1.,-3.11743156744182));
#55174=CARTESIAN_POINT('Ctrl Pts',(2.4329344968514,1.,-3.11321477659012));
#55175=CARTESIAN_POINT('Ctrl Pts',(2.42668025870013,1.,-3.10895518969592));
#55176=CARTESIAN_POINT('Ctrl Pts',(2.42045498612494,1.,-3.10465410280902));
#55177=CARTESIAN_POINT('Ctrl Pts',(2.41426441798067,1.,-3.10031775027683));
#55178=CARTESIAN_POINT('Ctrl Pts',(2.40811612696382,1.,-3.09595472616093));
#55179=CARTESIAN_POINT('Ctrl Pts',(2.40201704423352,1.,-3.09157266051115));
#55180=CARTESIAN_POINT('Ctrl Pts',(2.39597098250635,1.,-3.08717489512919));
#55181=CARTESIAN_POINT('Ctrl Pts',(2.38997659219192,1.,-3.08275773747083));
#55182=CARTESIAN_POINT('Ctrl Pts',(2.38402401216107,1.,-3.07830597244301));
#55183=CARTESIAN_POINT('Ctrl Pts',(2.37809856205524,1.,-3.07379777492133));
#55184=CARTESIAN_POINT('Ctrl Pts',(2.37218678163157,1.,-3.06921275497472));
#55185=CARTESIAN_POINT('Ctrl Pts',(2.36628220107001,1.,-3.06453964643152));
#55186=CARTESIAN_POINT('Ctrl Pts',(2.36039011602084,1.,-3.05978266240056));
#55187=CARTESIAN_POINT('Ctrl Pts',(2.35453559889506,1.,-3.05497218368188));
#55188=CARTESIAN_POINT('Ctrl Pts',(2.34875673090816,1.,-3.05015565829976));
#55189=CARTESIAN_POINT('Ctrl Pts',(2.3430901708402,1.,-3.04537822217311));
#55190=CARTESIAN_POINT('Ctrl Pts',(2.33755792953726,1.,-3.04066496998569));
#55191=CARTESIAN_POINT('Ctrl Pts',(2.33215619079807,1.,-3.03600588555765));
#55192=CARTESIAN_POINT('Ctrl Pts',(2.32683687412027,1.,-3.03133125185047));
#55193=CARTESIAN_POINT('Ctrl Pts',(2.32151944306299,1.,-3.02652678416478));
#55194=CARTESIAN_POINT('Ctrl Pts',(2.31612479121528,1.,-3.02147780668029));
#55195=CARTESIAN_POINT('Ctrl Pts',(2.31060449886577,1.,-3.01610726819019));
#55196=CARTESIAN_POINT('Ctrl Pts',(2.30496809486528,1.,-3.01041131063882));
#55197=CARTESIAN_POINT('Ctrl Pts',(2.29932091315939,1.,-3.00450832658822));
#55198=CARTESIAN_POINT('Ctrl Pts',(2.29385894577999,1.,-2.99863310340004));
#55199=CARTESIAN_POINT('Ctrl Pts',(2.28882328690601,1.,-2.9930793098434));
#55200=CARTESIAN_POINT('Ctrl Pts',(2.28446419116036,1.,-2.98815432734929));
#55201=CARTESIAN_POINT('Ctrl Pts',(2.28100472516582,1.,-2.98413343613858));
#55202=CARTESIAN_POINT('Ctrl Pts',(2.27877674853833,1.,-2.98142341809623));
#55203=CARTESIAN_POINT('Ctrl Pts',(2.27776738270369,1.,-2.98007383024333));
#55204=CARTESIAN_POINT('Ctrl Pts',(2.27743009389704,1.,-2.97951167106106));
#55205=CARTESIAN_POINT('Ctrl Pts',(2.27737238849212,1.,-2.97932307137589));
#55206=CARTESIAN_POINT('Ctrl Pts',(2.27737254473378,1.,-2.97927412174388));
#55207=CARTESIAN_POINT('',(2.66939624221984,0.,-3.24257979115744));
#55208=CARTESIAN_POINT('Ctrl Pts',(2.58626089374824,-1.,-2.71546581445404));
#55209=CARTESIAN_POINT('Ctrl Pts',(2.58626089374824,1.,-2.71546581445404));
#55210=CARTESIAN_POINT('Ctrl Pts',(2.58626222935803,-1.,-2.71537879705104));
#55211=CARTESIAN_POINT('Ctrl Pts',(2.58626222935803,1.,-2.71537879705104));
#55212=CARTESIAN_POINT('Ctrl Pts',(2.58636629904103,-1.,-2.71533674141254));
#55213=CARTESIAN_POINT('Ctrl Pts',(2.58636629904103,1.,-2.71533674141254));
#55214=CARTESIAN_POINT('Ctrl Pts',(2.5868265735259,-1.,-2.71566956750452));
#55215=CARTESIAN_POINT('Ctrl Pts',(2.5868265735259,1.,-2.71566956750452));
#55216=CARTESIAN_POINT('Ctrl Pts',(2.58804906785417,-1.,-2.71690570241638));
#55217=CARTESIAN_POINT('Ctrl Pts',(2.58804906785417,1.,-2.71690570241638));
#55218=CARTESIAN_POINT('Ctrl Pts',(2.59056604771971,-1.,-2.71974308958086));
#55219=CARTESIAN_POINT('Ctrl Pts',(2.59056604771971,1.,-2.71974308958086));
#55220=CARTESIAN_POINT('Ctrl Pts',(2.59399625537278,-1.,-2.72378896977134));
#55221=CARTESIAN_POINT('Ctrl Pts',(2.59399625537278,1.,-2.72378896977134));
#55222=CARTESIAN_POINT('Ctrl Pts',(2.59817869034746,-1.,-2.7288648348152));
#55223=CARTESIAN_POINT('Ctrl Pts',(2.59817869034746,1.,-2.7288648348152));
#55224=CARTESIAN_POINT('Ctrl Pts',(2.60287635688728,-1.,-2.73470730109615));
#55225=CARTESIAN_POINT('Ctrl Pts',(2.60287635688728,1.,-2.73470730109615));
#55226=CARTESIAN_POINT('Ctrl Pts',(2.60782480638448,-1.,-2.7410211099909));
#55227=CARTESIAN_POINT('Ctrl Pts',(2.60782480638448,1.,-2.7410211099909));
#55228=CARTESIAN_POINT('Ctrl Pts',(2.61277170105813,-1.,-2.74752219567252));
#55229=CARTESIAN_POINT('Ctrl Pts',(2.61277170105813,1.,-2.74752219567252));
#55230=CARTESIAN_POINT('Ctrl Pts',(2.61751580407667,-1.,-2.7539802502603));
#55231=CARTESIAN_POINT('Ctrl Pts',(2.61751580407667,1.,-2.7539802502603));
#55232=CARTESIAN_POINT('Ctrl Pts',(2.62195665834605,-1.,-2.76027271596686));
#55233=CARTESIAN_POINT('Ctrl Pts',(2.62195665834605,1.,-2.76027271596686));
#55234=CARTESIAN_POINT('Ctrl Pts',(2.62609956506355,-1.,-2.76639078479021));
#55235=CARTESIAN_POINT('Ctrl Pts',(2.62609956506355,1.,-2.76639078479021));
#55236=CARTESIAN_POINT('Ctrl Pts',(2.63001305229625,-1.,-2.77239433377921));
#55237=CARTESIAN_POINT('Ctrl Pts',(2.63001305229625,1.,-2.77239433377921));
#55238=CARTESIAN_POINT('Ctrl Pts',(2.63379800904599,-1.,-2.77837943466449));
#55239=CARTESIAN_POINT('Ctrl Pts',(2.63379800904599,1.,-2.77837943466449));
#55240=CARTESIAN_POINT('Ctrl Pts',(2.637554714303,-1.,-2.78444351041571));
#55241=CARTESIAN_POINT('Ctrl Pts',(2.637554714303,1.,-2.78444351041571));
#55242=CARTESIAN_POINT('Ctrl Pts',(2.64134450532584,-1.,-2.79064495573224));
#55243=CARTESIAN_POINT('Ctrl Pts',(2.64134450532584,1.,-2.79064495573224));
#55244=CARTESIAN_POINT('Ctrl Pts',(2.64517667799319,-1.,-2.79698910670736));
#55245=CARTESIAN_POINT('Ctrl Pts',(2.64517667799319,1.,-2.79698910670736));
#55246=CARTESIAN_POINT('Ctrl Pts',(2.64902988983337,-1.,-2.80345029781152));
#55247=CARTESIAN_POINT('Ctrl Pts',(2.64902988983337,1.,-2.80345029781152));
#55248=CARTESIAN_POINT('Ctrl Pts',(2.65286529532208,-1.,-2.80998526078165));
#55249=CARTESIAN_POINT('Ctrl Pts',(2.65286529532208,1.,-2.80998526078165));
#55250=CARTESIAN_POINT('Ctrl Pts',(2.65664198781344,-1.,-2.81654896073883));
#55251=CARTESIAN_POINT('Ctrl Pts',(2.65664198781344,1.,-2.81654896073883));
#55252=CARTESIAN_POINT('Ctrl Pts',(2.66033388273461,-1.,-2.82311188135078));
#55253=CARTESIAN_POINT('Ctrl Pts',(2.66033388273461,1.,-2.82311188135078));
#55254=CARTESIAN_POINT('Ctrl Pts',(2.6639376472693,-1.,-2.82966813308998));
#55255=CARTESIAN_POINT('Ctrl Pts',(2.6639376472693,1.,-2.82966813308998));
#55256=CARTESIAN_POINT('Ctrl Pts',(2.66746339678107,-1.,-2.83622586853982));
#55257=CARTESIAN_POINT('Ctrl Pts',(2.66746339678107,1.,-2.83622586853982));
#55258=CARTESIAN_POINT('Ctrl Pts',(2.67092916452125,-1.,-2.84280157191323));
#55259=CARTESIAN_POINT('Ctrl Pts',(2.67092916452125,1.,-2.84280157191323));
#55260=CARTESIAN_POINT('Ctrl Pts',(2.67435421039677,-1.,-2.84941315703092));
#55261=CARTESIAN_POINT('Ctrl Pts',(2.67435421039677,1.,-2.84941315703092));
#55262=CARTESIAN_POINT('Ctrl Pts',(2.67775201955724,-1.,-2.85607274378018));
#55263=CARTESIAN_POINT('Ctrl Pts',(2.67775201955724,1.,-2.85607274378018));
#55264=CARTESIAN_POINT('Ctrl Pts',(2.68112602796308,-1.,-2.86278224277689));
#55265=CARTESIAN_POINT('Ctrl Pts',(2.68112602796308,1.,-2.86278224277689));
#55266=CARTESIAN_POINT('Ctrl Pts',(2.68447353139599,-1.,-2.86953736547238));
#55267=CARTESIAN_POINT('Ctrl Pts',(2.68447353139599,1.,-2.86953736547238));
#55268=CARTESIAN_POINT('Ctrl Pts',(2.68778807801686,-1.,-2.8763300724388));
#55269=CARTESIAN_POINT('Ctrl Pts',(2.68778807801686,1.,-2.8763300724388));
#55270=CARTESIAN_POINT('Ctrl Pts',(2.69106236420198,-1.,-2.88315153980466));
#55271=CARTESIAN_POINT('Ctrl Pts',(2.69106236420198,1.,-2.88315153980466));
#55272=CARTESIAN_POINT('Ctrl Pts',(2.69429113011374,-1.,-2.88999512410309));
#55273=CARTESIAN_POINT('Ctrl Pts',(2.69429113011374,1.,-2.88999512410309));
#55274=CARTESIAN_POINT('Ctrl Pts',(2.69747340630625,-1.,-2.89685866123671));
#55275=CARTESIAN_POINT('Ctrl Pts',(2.69747340630625,1.,-2.89685866123671));
#55276=CARTESIAN_POINT('Ctrl Pts',(2.70061095078692,-1.,-2.90374285605838));
#55277=CARTESIAN_POINT('Ctrl Pts',(2.70061095078692,1.,-2.90374285605838));
#55278=CARTESIAN_POINT('Ctrl Pts',(2.70370719782113,-1.,-2.91065019668329));
#55279=CARTESIAN_POINT('Ctrl Pts',(2.70370719782113,1.,-2.91065019668329));
#55280=CARTESIAN_POINT('Ctrl Pts',(2.70676602302518,-1.,-2.91758367994737));
#55281=CARTESIAN_POINT('Ctrl Pts',(2.70676602302518,1.,-2.91758367994737));
#55282=CARTESIAN_POINT('Ctrl Pts',(2.70979055994754,-1.,-2.92454558914778));
#55283=CARTESIAN_POINT('Ctrl Pts',(2.70979055994754,1.,-2.92454558914778));
#55284=CARTESIAN_POINT('Ctrl Pts',(2.71278207520817,-1.,-2.93153633192595));
#55285=CARTESIAN_POINT('Ctrl Pts',(2.71278207520817,1.,-2.93153633192595));
#55286=CARTESIAN_POINT('Ctrl Pts',(2.7157405459259,-1.,-2.93855503247266));
#55287=CARTESIAN_POINT('Ctrl Pts',(2.7157405459259,1.,-2.93855503247266));
#55288=CARTESIAN_POINT('Ctrl Pts',(2.71866514227965,-1.,-2.94560002559806));
#55289=CARTESIAN_POINT('Ctrl Pts',(2.71866514227965,1.,-2.94560002559806));
#55290=CARTESIAN_POINT('Ctrl Pts',(2.72155475123364,-1.,-2.95266939280621));
#55291=CARTESIAN_POINT('Ctrl Pts',(2.72155475123364,1.,-2.95266939280621));
#55292=CARTESIAN_POINT('Ctrl Pts',(2.72440846811729,-1.,-2.95976146492576));
#55293=CARTESIAN_POINT('Ctrl Pts',(2.72440846811729,1.,-2.95976146492576));
#55294=CARTESIAN_POINT('Ctrl Pts',(2.72722614084076,-1.,-2.96687537842451));
#55295=CARTESIAN_POINT('Ctrl Pts',(2.72722614084076,1.,-2.96687537842451));
#55296=CARTESIAN_POINT('Ctrl Pts',(2.73000819218414,-1.,-2.97401089032677));
#55297=CARTESIAN_POINT('Ctrl Pts',(2.73000819218414,1.,-2.97401089032677));
#55298=CARTESIAN_POINT('Ctrl Pts',(2.73275539286497,-1.,-2.98116814232129));
#55299=CARTESIAN_POINT('Ctrl Pts',(2.73275539286497,1.,-2.98116814232129));
#55300=CARTESIAN_POINT('Ctrl Pts',(2.73546864694536,-1.,-2.9883474369644));
#55301=CARTESIAN_POINT('Ctrl Pts',(2.73546864694536,1.,-2.9883474369644));
#55302=CARTESIAN_POINT('Ctrl Pts',(2.73814878711641,-1.,-2.99554902409778));
#55303=CARTESIAN_POINT('Ctrl Pts',(2.73814878711641,1.,-2.99554902409778));
#55304=CARTESIAN_POINT('Ctrl Pts',(2.74079632883931,-1.,-3.00277284351521));
#55305=CARTESIAN_POINT('Ctrl Pts',(2.74079632883931,1.,-3.00277284351521));
#55306=CARTESIAN_POINT('Ctrl Pts',(2.74341150239887,-1.,-3.01001855960162));
#55307=CARTESIAN_POINT('Ctrl Pts',(2.74341150239887,1.,-3.01001855960162));
#55308=CARTESIAN_POINT('Ctrl Pts',(2.74599436193625,-1.,-3.01728567646611));
#55309=CARTESIAN_POINT('Ctrl Pts',(2.74599436193625,1.,-3.01728567646611));
#55310=CARTESIAN_POINT('Ctrl Pts',(2.7485448718414,-1.,-3.02457362909245));
#55311=CARTESIAN_POINT('Ctrl Pts',(2.7485448718414,1.,-3.02457362909245));
#55312=CARTESIAN_POINT('Ctrl Pts',(2.75106299522979,-1.,-3.03188187589107));
#55313=CARTESIAN_POINT('Ctrl Pts',(2.75106299522979,1.,-3.03188187589107));
#55314=CARTESIAN_POINT('Ctrl Pts',(2.75354880060314,-1.,-3.03921001107977));
#55315=CARTESIAN_POINT('Ctrl Pts',(2.75354880060314,1.,-3.03921001107977));
#55316=CARTESIAN_POINT('Ctrl Pts',(2.75600247455925,-1.,-3.04655777351067));
#55317=CARTESIAN_POINT('Ctrl Pts',(2.75600247455925,1.,-3.04655777351067));
#55318=CARTESIAN_POINT('Ctrl Pts',(2.75842427252931,-1.,-3.05392498749847));
#55319=CARTESIAN_POINT('Ctrl Pts',(2.75842427252931,1.,-3.05392498749847));
#55320=CARTESIAN_POINT('Ctrl Pts',(2.76081448759882,-1.,-3.06131152247454));
#55321=CARTESIAN_POINT('Ctrl Pts',(2.76081448759882,1.,-3.06131152247454));
#55322=CARTESIAN_POINT('Ctrl Pts',(2.76317341453493,-1.,-3.0687172484321));
#55323=CARTESIAN_POINT('Ctrl Pts',(2.76317341453493,1.,-3.0687172484321));
#55324=CARTESIAN_POINT('Ctrl Pts',(2.76550131064852,-1.,-3.07614198408862));
#55325=CARTESIAN_POINT('Ctrl Pts',(2.76550131064852,1.,-3.07614198408862));
#55326=CARTESIAN_POINT('Ctrl Pts',(2.76779837829373,-1.,-3.08358548001504));
#55327=CARTESIAN_POINT('Ctrl Pts',(2.76779837829373,1.,-3.08358548001504));
#55328=CARTESIAN_POINT('Ctrl Pts',(2.7700647803451,-1.,-3.09104745382531));
#55329=CARTESIAN_POINT('Ctrl Pts',(2.7700647803451,1.,-3.09104745382531));
#55330=CARTESIAN_POINT('Ctrl Pts',(2.77230064796057,-1.,-3.0985276127786));
#55331=CARTESIAN_POINT('Ctrl Pts',(2.77230064796057,1.,-3.0985276127786));
#55332=CARTESIAN_POINT('Ctrl Pts',(2.77450609123362,-1.,-3.10602568032564));
#55333=CARTESIAN_POINT('Ctrl Pts',(2.77450609123362,1.,-3.10602568032564));
#55334=CARTESIAN_POINT('Ctrl Pts',(2.77668121002545,-1.,-3.11354142303921));
#55335=CARTESIAN_POINT('Ctrl Pts',(2.77668121002545,1.,-3.11354142303921));
#55336=CARTESIAN_POINT('Ctrl Pts',(2.77882610146731,-1.,-3.12107467037201));
#55337=CARTESIAN_POINT('Ctrl Pts',(2.77882610146731,1.,-3.12107467037201));
#55338=CARTESIAN_POINT('Ctrl Pts',(2.78094085161413,-1.,-3.12862530318457));
#55339=CARTESIAN_POINT('Ctrl Pts',(2.78094085161413,1.,-3.12862530318457));
#55340=CARTESIAN_POINT('Ctrl Pts',(2.78260859419319,-1.,-3.13467965833037));
#55341=CARTESIAN_POINT('Ctrl Pts',(2.78260859419319,1.,-3.13467965833037));
#55342=CARTESIAN_POINT('Ctrl Pts',(2.78384588958165,-1.,-3.13922819749279));
#55343=CARTESIAN_POINT('Ctrl Pts',(2.78384588958165,1.,-3.13922819749279));
#55344=CARTESIAN_POINT('Ctrl Pts',(2.7846647503589,-1.,-3.14226401018816));
#55345=CARTESIAN_POINT('Ctrl Pts',(2.7846647503589,1.,-3.14226401018816));
#55346=CARTESIAN_POINT('Ctrl Pts',(2.78507268004356,-1.,-3.14378277984898));
#55347=CARTESIAN_POINT('Ctrl Pts',(2.78507268004356,1.,-3.14378277984898));
#55348=CARTESIAN_POINT('',(2.58633475774921,1.,-2.71539546306948));
#55349=CARTESIAN_POINT('Ctrl Pts',(2.58633475774921,-1.,-2.71539546306948));
#55350=CARTESIAN_POINT('Ctrl Pts',(2.58633475774921,-0.666666666666667,
-2.71539546306948));
#55351=CARTESIAN_POINT('Ctrl Pts',(2.58633475774921,-0.333333333333333,
-2.71539546306948));
#55352=CARTESIAN_POINT('Ctrl Pts',(2.58633475774921,0.333333333333333,-2.71539546306948));
#55353=CARTESIAN_POINT('Ctrl Pts',(2.58633475774921,0.666666666666667,-2.71539546306948));
#55354=CARTESIAN_POINT('Ctrl Pts',(2.58633475774921,1.,-2.71539546306948));
#55355=CARTESIAN_POINT('',(2.78507268004356,1.,-3.14378277984898));
#55356=CARTESIAN_POINT('',(2.78507268004356,0.,-3.14378277984898));
#55357=CARTESIAN_POINT('Ctrl Pts',(2.58633475774921,1.,-2.71539546306948));
#55358=CARTESIAN_POINT('Ctrl Pts',(2.58638312917168,1.,-2.71540296616024));
#55359=CARTESIAN_POINT('Ctrl Pts',(2.58656037976753,1.,-2.71548946460575));
#55360=CARTESIAN_POINT('Ctrl Pts',(2.58706285424358,1.,-2.71591054189786));
#55361=CARTESIAN_POINT('Ctrl Pts',(2.58823792682672,1.,-2.71711860281815));
#55362=CARTESIAN_POINT('Ctrl Pts',(2.59056604771971,1.,-2.71974308958086));
#55363=CARTESIAN_POINT('Ctrl Pts',(2.59399625537278,1.,-2.72378896977134));
#55364=CARTESIAN_POINT('Ctrl Pts',(2.59817869034746,1.,-2.7288648348152));
#55365=CARTESIAN_POINT('Ctrl Pts',(2.60287635688728,1.,-2.73470730109615));
#55366=CARTESIAN_POINT('Ctrl Pts',(2.60782480638448,1.,-2.7410211099909));
#55367=CARTESIAN_POINT('Ctrl Pts',(2.61277170105813,1.,-2.74752219567252));
#55368=CARTESIAN_POINT('Ctrl Pts',(2.61751580407667,1.,-2.7539802502603));
#55369=CARTESIAN_POINT('Ctrl Pts',(2.62195665834605,1.,-2.76027271596686));
#55370=CARTESIAN_POINT('Ctrl Pts',(2.62609956506355,1.,-2.76639078479021));
#55371=CARTESIAN_POINT('Ctrl Pts',(2.63001305229625,1.,-2.77239433377921));
#55372=CARTESIAN_POINT('Ctrl Pts',(2.63379800904599,1.,-2.77837943466449));
#55373=CARTESIAN_POINT('Ctrl Pts',(2.637554714303,1.,-2.78444351041571));
#55374=CARTESIAN_POINT('Ctrl Pts',(2.64134450532584,1.,-2.79064495573224));
#55375=CARTESIAN_POINT('Ctrl Pts',(2.64517667799319,1.,-2.79698910670736));
#55376=CARTESIAN_POINT('Ctrl Pts',(2.64902988983337,1.,-2.80345029781152));
#55377=CARTESIAN_POINT('Ctrl Pts',(2.65286529532208,1.,-2.80998526078165));
#55378=CARTESIAN_POINT('Ctrl Pts',(2.65664198781344,1.,-2.81654896073883));
#55379=CARTESIAN_POINT('Ctrl Pts',(2.66033388273461,1.,-2.82311188135078));
#55380=CARTESIAN_POINT('Ctrl Pts',(2.6639376472693,1.,-2.82966813308998));
#55381=CARTESIAN_POINT('Ctrl Pts',(2.66746339678107,1.,-2.83622586853982));
#55382=CARTESIAN_POINT('Ctrl Pts',(2.67092916452125,1.,-2.84280157191323));
#55383=CARTESIAN_POINT('Ctrl Pts',(2.67435421039677,1.,-2.84941315703092));
#55384=CARTESIAN_POINT('Ctrl Pts',(2.67775201955724,1.,-2.85607274378018));
#55385=CARTESIAN_POINT('Ctrl Pts',(2.68112602796308,1.,-2.86278224277689));
#55386=CARTESIAN_POINT('Ctrl Pts',(2.68447353139599,1.,-2.86953736547238));
#55387=CARTESIAN_POINT('Ctrl Pts',(2.68778807801686,1.,-2.8763300724388));
#55388=CARTESIAN_POINT('Ctrl Pts',(2.69106236420198,1.,-2.88315153980466));
#55389=CARTESIAN_POINT('Ctrl Pts',(2.69429113011374,1.,-2.88999512410309));
#55390=CARTESIAN_POINT('Ctrl Pts',(2.69747340630625,1.,-2.89685866123671));
#55391=CARTESIAN_POINT('Ctrl Pts',(2.70061095078692,1.,-2.90374285605838));
#55392=CARTESIAN_POINT('Ctrl Pts',(2.70370719782113,1.,-2.91065019668329));
#55393=CARTESIAN_POINT('Ctrl Pts',(2.70676602302518,1.,-2.91758367994737));
#55394=CARTESIAN_POINT('Ctrl Pts',(2.70979055994754,1.,-2.92454558914778));
#55395=CARTESIAN_POINT('Ctrl Pts',(2.71278207520817,1.,-2.93153633192595));
#55396=CARTESIAN_POINT('Ctrl Pts',(2.7157405459259,1.,-2.93855503247266));
#55397=CARTESIAN_POINT('Ctrl Pts',(2.71866514227965,1.,-2.94560002559806));
#55398=CARTESIAN_POINT('Ctrl Pts',(2.72155475123364,1.,-2.95266939280621));
#55399=CARTESIAN_POINT('Ctrl Pts',(2.72440846811729,1.,-2.95976146492576));
#55400=CARTESIAN_POINT('Ctrl Pts',(2.72722614084076,1.,-2.96687537842451));
#55401=CARTESIAN_POINT('Ctrl Pts',(2.73000819218414,1.,-2.97401089032677));
#55402=CARTESIAN_POINT('Ctrl Pts',(2.73275539286497,1.,-2.98116814232129));
#55403=CARTESIAN_POINT('Ctrl Pts',(2.73546864694536,1.,-2.9883474369644));
#55404=CARTESIAN_POINT('Ctrl Pts',(2.73814878711641,1.,-2.99554902409778));
#55405=CARTESIAN_POINT('Ctrl Pts',(2.74079632883931,1.,-3.00277284351521));
#55406=CARTESIAN_POINT('Ctrl Pts',(2.74341150239887,1.,-3.01001855960162));
#55407=CARTESIAN_POINT('Ctrl Pts',(2.74599436193625,1.,-3.01728567646611));
#55408=CARTESIAN_POINT('Ctrl Pts',(2.7485448718414,1.,-3.02457362909245));
#55409=CARTESIAN_POINT('Ctrl Pts',(2.75106299522979,1.,-3.03188187589107));
#55410=CARTESIAN_POINT('Ctrl Pts',(2.75354880060314,1.,-3.03921001107977));
#55411=CARTESIAN_POINT('Ctrl Pts',(2.75600247455925,1.,-3.04655777351067));
#55412=CARTESIAN_POINT('Ctrl Pts',(2.75842427252931,1.,-3.05392498749847));
#55413=CARTESIAN_POINT('Ctrl Pts',(2.76081448759882,1.,-3.06131152247454));
#55414=CARTESIAN_POINT('Ctrl Pts',(2.76317341453493,1.,-3.0687172484321));
#55415=CARTESIAN_POINT('Ctrl Pts',(2.76550131064852,1.,-3.07614198408862));
#55416=CARTESIAN_POINT('Ctrl Pts',(2.76779837829373,1.,-3.08358548001504));
#55417=CARTESIAN_POINT('Ctrl Pts',(2.7700647803451,1.,-3.09104745382531));
#55418=CARTESIAN_POINT('Ctrl Pts',(2.77230064796057,1.,-3.0985276127786));
#55419=CARTESIAN_POINT('Ctrl Pts',(2.77450609123362,1.,-3.10602568032564));
#55420=CARTESIAN_POINT('Ctrl Pts',(2.77668121002545,1.,-3.11354142303921));
#55421=CARTESIAN_POINT('Ctrl Pts',(2.77882610146731,1.,-3.12107467037201));
#55422=CARTESIAN_POINT('Ctrl Pts',(2.78094085161413,1.,-3.12862530318457));
#55423=CARTESIAN_POINT('Ctrl Pts',(2.78260859419319,1.,-3.13467965833037));
#55424=CARTESIAN_POINT('Ctrl Pts',(2.78384588958165,1.,-3.13922819749279));
#55425=CARTESIAN_POINT('Ctrl Pts',(2.7846647503589,1.,-3.14226401018816));
#55426=CARTESIAN_POINT('Ctrl Pts',(2.78507268004356,1.,-3.14378277984898));
#55427=CARTESIAN_POINT('Origin',(2.78507268004356,0.,-3.14378277984898));
#55428=CARTESIAN_POINT('',(2.66939624221984,1.,-3.24257979115744));
#55429=CARTESIAN_POINT('Origin',(0.,0.,0.));
#55430=CARTESIAN_POINT('',(2.71539546306824,1.,-2.58633475775051));
#55431=CARTESIAN_POINT('Origin',(0.,1.,0.));
#55432=CARTESIAN_POINT('Ctrl Pts',(2.71539546306824,1.,-2.58633475775051));
#55433=CARTESIAN_POINT('Ctrl Pts',(2.71539546306824,0.666666666666667,-2.58633475775051));
#55434=CARTESIAN_POINT('Ctrl Pts',(2.71539546306824,0.333333333333333,-2.58633475775051));
#55435=CARTESIAN_POINT('Ctrl Pts',(2.71539546306824,-0.333333333333333,
-2.58633475775051));
#55436=CARTESIAN_POINT('Ctrl Pts',(2.71539546306824,-0.666666666666667,
-2.58633475775051));
#55437=CARTESIAN_POINT('Ctrl Pts',(2.71539546306824,-1.,-2.58633475775051));
#55438=CARTESIAN_POINT('Ctrl Pts',(3.14378277984898,-1.,-2.78507268004356));
#55439=CARTESIAN_POINT('Ctrl Pts',(3.14378277984898,1.,-2.78507268004356));
#55440=CARTESIAN_POINT('Ctrl Pts',(3.14226401019149,-1.,-2.78466475036183));
#55441=CARTESIAN_POINT('Ctrl Pts',(3.14226401019149,1.,-2.78466475036183));
#55442=CARTESIAN_POINT('Ctrl Pts',(3.13922819750185,-1.,-2.78384588958965));
#55443=CARTESIAN_POINT('Ctrl Pts',(3.13922819750185,1.,-2.78384588958965));
#55444=CARTESIAN_POINT('Ctrl Pts',(3.1346796583452,-1.,-2.78260859420629));
#55445=CARTESIAN_POINT('Ctrl Pts',(3.1346796583452,1.,-2.78260859420629));
#55446=CARTESIAN_POINT('Ctrl Pts',(3.12862530320194,-1.,-2.78094085162947));
#55447=CARTESIAN_POINT('Ctrl Pts',(3.12862530320194,1.,-2.78094085162947));
#55448=CARTESIAN_POINT('Ctrl Pts',(3.12107467038623,-1.,-2.77882610147986));
#55449=CARTESIAN_POINT('Ctrl Pts',(3.12107467038623,1.,-2.77882610147986));
#55450=CARTESIAN_POINT('Ctrl Pts',(3.11354142304692,-1.,-2.77668121003225));
#55451=CARTESIAN_POINT('Ctrl Pts',(3.11354142304692,1.,-2.77668121003225));
#55452=CARTESIAN_POINT('Ctrl Pts',(3.10602568032641,-1.,-2.7745060912343));
#55453=CARTESIAN_POINT('Ctrl Pts',(3.10602568032641,1.,-2.7745060912343));
#55454=CARTESIAN_POINT('Ctrl Pts',(3.09852761277432,-1.,-2.77230064795679));
#55455=CARTESIAN_POINT('Ctrl Pts',(3.09852761277432,1.,-2.77230064795679));
#55456=CARTESIAN_POINT('Ctrl Pts',(3.09104745381882,-1.,-2.77006478033937));
#55457=CARTESIAN_POINT('Ctrl Pts',(3.09104745381882,1.,-2.77006478033937));
#55458=CARTESIAN_POINT('Ctrl Pts',(3.08358548000904,-1.,-2.76779837828843));
#55459=CARTESIAN_POINT('Ctrl Pts',(3.08358548000904,1.,-2.76779837828843));
#55460=CARTESIAN_POINT('Ctrl Pts',(3.07614198408488,-1.,-2.76550131064522));
#55461=CARTESIAN_POINT('Ctrl Pts',(3.07614198408488,1.,-2.76550131064522));
#55462=CARTESIAN_POINT('Ctrl Pts',(3.06871724843121,-1.,-2.76317341453415));
#55463=CARTESIAN_POINT('Ctrl Pts',(3.06871724843121,1.,-2.76317341453415));
#55464=CARTESIAN_POINT('Ctrl Pts',(3.06131152247599,-1.,-2.76081448760011));
#55465=CARTESIAN_POINT('Ctrl Pts',(3.06131152247599,1.,-2.76081448760011));
#55466=CARTESIAN_POINT('Ctrl Pts',(3.05392498750112,-1.,-2.75842427253164));
#55467=CARTESIAN_POINT('Ctrl Pts',(3.05392498750112,1.,-2.75842427253164));
#55468=CARTESIAN_POINT('Ctrl Pts',(3.04655777351333,-1.,-2.7560024745616));
#55469=CARTESIAN_POINT('Ctrl Pts',(3.04655777351333,1.,-2.7560024745616));
#55470=CARTESIAN_POINT('Ctrl Pts',(3.03921001108158,-1.,-2.75354880060473));
#55471=CARTESIAN_POINT('Ctrl Pts',(3.03921001108158,1.,-2.75354880060473));
#55472=CARTESIAN_POINT('Ctrl Pts',(3.03188187589168,-1.,-2.75106299523032));
#55473=CARTESIAN_POINT('Ctrl Pts',(3.03188187589168,1.,-2.75106299523032));
#55474=CARTESIAN_POINT('Ctrl Pts',(3.02457362909199,-1.,-2.74854487184099));
#55475=CARTESIAN_POINT('Ctrl Pts',(3.02457362909199,1.,-2.74854487184099));
#55476=CARTESIAN_POINT('Ctrl Pts',(3.01728567646502,-1.,-2.74599436193528));
#55477=CARTESIAN_POINT('Ctrl Pts',(3.01728567646502,1.,-2.74599436193528));
#55478=CARTESIAN_POINT('Ctrl Pts',(3.01001855960041,-1.,-2.7434115023978));
#55479=CARTESIAN_POINT('Ctrl Pts',(3.01001855960041,1.,-2.7434115023978));
#55480=CARTESIAN_POINT('Ctrl Pts',(3.00277284351431,-1.,-2.74079632883852));
#55481=CARTESIAN_POINT('Ctrl Pts',(3.00277284351431,1.,-2.74079632883852));
#55482=CARTESIAN_POINT('Ctrl Pts',(2.99554902409741,-1.,-2.73814878711609));
#55483=CARTESIAN_POINT('Ctrl Pts',(2.99554902409741,1.,-2.73814878711609));
#55484=CARTESIAN_POINT('Ctrl Pts',(2.98834743696455,-1.,-2.73546864694548));
#55485=CARTESIAN_POINT('Ctrl Pts',(2.98834743696455,1.,-2.73546864694548));
#55486=CARTESIAN_POINT('Ctrl Pts',(2.98116814232175,-1.,-2.73275539286537));
#55487=CARTESIAN_POINT('Ctrl Pts',(2.98116814232175,1.,-2.73275539286537));
#55488=CARTESIAN_POINT('Ctrl Pts',(2.97401089032729,-1.,-2.7300081921846));
#55489=CARTESIAN_POINT('Ctrl Pts',(2.97401089032729,1.,-2.7300081921846));
#55490=CARTESIAN_POINT('Ctrl Pts',(2.96687537842492,-1.,-2.72722614084112));
#55491=CARTESIAN_POINT('Ctrl Pts',(2.96687537842492,1.,-2.72722614084112));
#55492=CARTESIAN_POINT('Ctrl Pts',(2.95976146492595,-1.,-2.72440846811745));
#55493=CARTESIAN_POINT('Ctrl Pts',(2.95976146492595,1.,-2.72440846811745));
#55494=CARTESIAN_POINT('Ctrl Pts',(2.95266939280617,-1.,-2.72155475123361));
#55495=CARTESIAN_POINT('Ctrl Pts',(2.95266939280617,1.,-2.72155475123361));
#55496=CARTESIAN_POINT('Ctrl Pts',(2.94560002559789,-1.,-2.71866514227951));
#55497=CARTESIAN_POINT('Ctrl Pts',(2.94560002559789,1.,-2.71866514227951));
#55498=CARTESIAN_POINT('Ctrl Pts',(2.93855503247248,-1.,-2.71574054592575));
#55499=CARTESIAN_POINT('Ctrl Pts',(2.93855503247248,1.,-2.71574054592575));
#55500=CARTESIAN_POINT('Ctrl Pts',(2.93153633192583,-1.,-2.71278207520807));
#55501=CARTESIAN_POINT('Ctrl Pts',(2.93153633192583,1.,-2.71278207520807));
#55502=CARTESIAN_POINT('Ctrl Pts',(2.92454558914774,-1.,-2.70979055994751));
#55503=CARTESIAN_POINT('Ctrl Pts',(2.92454558914774,1.,-2.70979055994751));
#55504=CARTESIAN_POINT('Ctrl Pts',(2.91758367994738,-1.,-2.70676602302518));
#55505=CARTESIAN_POINT('Ctrl Pts',(2.91758367994738,1.,-2.70676602302518));
#55506=CARTESIAN_POINT('Ctrl Pts',(2.91065019668331,-1.,-2.70370719782114));
#55507=CARTESIAN_POINT('Ctrl Pts',(2.91065019668331,1.,-2.70370719782114));
#55508=CARTESIAN_POINT('Ctrl Pts',(2.90374285605839,-1.,-2.70061095078692));
#55509=CARTESIAN_POINT('Ctrl Pts',(2.90374285605839,1.,-2.70061095078692));
#55510=CARTESIAN_POINT('Ctrl Pts',(2.89685866123668,-1.,-2.69747340630621));
#55511=CARTESIAN_POINT('Ctrl Pts',(2.89685866123668,1.,-2.69747340630621));
#55512=CARTESIAN_POINT('Ctrl Pts',(2.88999512410304,-1.,-2.69429113011369));
#55513=CARTESIAN_POINT('Ctrl Pts',(2.88999512410304,1.,-2.69429113011369));
#55514=CARTESIAN_POINT('Ctrl Pts',(2.88315153980464,-1.,-2.69106236420197));
#55515=CARTESIAN_POINT('Ctrl Pts',(2.88315153980464,1.,-2.69106236420197));
#55516=CARTESIAN_POINT('Ctrl Pts',(2.87633007243885,-1.,-2.68778807801691));
#55517=CARTESIAN_POINT('Ctrl Pts',(2.87633007243885,1.,-2.68778807801691));
#55518=CARTESIAN_POINT('Ctrl Pts',(2.8695373654725,-1.,-2.68447353139611));
#55519=CARTESIAN_POINT('Ctrl Pts',(2.8695373654725,1.,-2.68447353139611));
#55520=CARTESIAN_POINT('Ctrl Pts',(2.86278224277705,-1.,-2.68112602796323));
#55521=CARTESIAN_POINT('Ctrl Pts',(2.86278224277705,1.,-2.68112602796323));
#55522=CARTESIAN_POINT('Ctrl Pts',(2.85607274378031,-1.,-2.67775201955736));
#55523=CARTESIAN_POINT('Ctrl Pts',(2.85607274378031,1.,-2.67775201955736));
#55524=CARTESIAN_POINT('Ctrl Pts',(2.84941315703096,-1.,-2.67435421039682));
#55525=CARTESIAN_POINT('Ctrl Pts',(2.84941315703096,1.,-2.67435421039682));
#55526=CARTESIAN_POINT('Ctrl Pts',(2.84280157191314,-1.,-2.67092916452117));
#55527=CARTESIAN_POINT('Ctrl Pts',(2.84280157191314,1.,-2.67092916452117));
#55528=CARTESIAN_POINT('Ctrl Pts',(2.8362258685396,-1.,-2.66746339678085));
#55529=CARTESIAN_POINT('Ctrl Pts',(2.8362258685396,1.,-2.66746339678085));
#55530=CARTESIAN_POINT('Ctrl Pts',(2.82966813308969,-1.,-2.66393764726902));
#55531=CARTESIAN_POINT('Ctrl Pts',(2.82966813308969,1.,-2.66393764726902));
#55532=CARTESIAN_POINT('Ctrl Pts',(2.82311188135053,-1.,-2.66033388273437));
#55533=CARTESIAN_POINT('Ctrl Pts',(2.82311188135053,1.,-2.66033388273437));
#55534=CARTESIAN_POINT('Ctrl Pts',(2.81654896073874,-1.,-2.65664198781335));
#55535=CARTESIAN_POINT('Ctrl Pts',(2.81654896073874,1.,-2.65664198781335));
#55536=CARTESIAN_POINT('Ctrl Pts',(2.80998526078179,-1.,-2.65286529532221));
#55537=CARTESIAN_POINT('Ctrl Pts',(2.80998526078179,1.,-2.65286529532221));
#55538=CARTESIAN_POINT('Ctrl Pts',(2.80345029781191,-1.,-2.64902988983373));
#55539=CARTESIAN_POINT('Ctrl Pts',(2.80345029781191,1.,-2.64902988983373));
#55540=CARTESIAN_POINT('Ctrl Pts',(2.7969891067079,-1.,-2.6451766779937));
#55541=CARTESIAN_POINT('Ctrl Pts',(2.7969891067079,1.,-2.6451766779937));
#55542=CARTESIAN_POINT('Ctrl Pts',(2.79064495573275,-1.,-2.64134450532632));
#55543=CARTESIAN_POINT('Ctrl Pts',(2.79064495573275,1.,-2.64134450532632));
#55544=CARTESIAN_POINT('Ctrl Pts',(2.78444351041594,-1.,-2.63755471430322));
#55545=CARTESIAN_POINT('Ctrl Pts',(2.78444351041594,1.,-2.63755471430322));
#55546=CARTESIAN_POINT('Ctrl Pts',(2.77837943466423,-1.,-2.63379800904575));
#55547=CARTESIAN_POINT('Ctrl Pts',(2.77837943466423,1.,-2.63379800904575));
#55548=CARTESIAN_POINT('Ctrl Pts',(2.77239433377839,-1.,-2.63001305229548));
#55549=CARTESIAN_POINT('Ctrl Pts',(2.77239433377839,1.,-2.63001305229548));
#55550=CARTESIAN_POINT('Ctrl Pts',(2.76639078478898,-1.,-2.6260995650624));
#55551=CARTESIAN_POINT('Ctrl Pts',(2.76639078478898,1.,-2.6260995650624));
#55552=CARTESIAN_POINT('Ctrl Pts',(2.76027271596564,-1.,-2.62195665834491));
#55553=CARTESIAN_POINT('Ctrl Pts',(2.76027271596564,1.,-2.62195665834491));
#55554=CARTESIAN_POINT('Ctrl Pts',(2.75398025025967,-1.,-2.61751580407608));
#55555=CARTESIAN_POINT('Ctrl Pts',(2.75398025025967,1.,-2.61751580407608));
#55556=CARTESIAN_POINT('Ctrl Pts',(2.74752219567307,-1.,-2.61277170105864));
#55557=CARTESIAN_POINT('Ctrl Pts',(2.74752219567307,1.,-2.61277170105864));
#55558=CARTESIAN_POINT('Ctrl Pts',(2.74102110999284,-1.,-2.60782480638629));
#55559=CARTESIAN_POINT('Ctrl Pts',(2.74102110999284,1.,-2.60782480638629));
#55560=CARTESIAN_POINT('Ctrl Pts',(2.73470730109906,-1.,-2.60287635689));
#55561=CARTESIAN_POINT('Ctrl Pts',(2.73470730109906,1.,-2.60287635689));
#55562=CARTESIAN_POINT('Ctrl Pts',(2.72886483481804,-1.,-2.5981786903501));
#55563=CARTESIAN_POINT('Ctrl Pts',(2.72886483481804,1.,-2.5981786903501));
#55564=CARTESIAN_POINT('Ctrl Pts',(2.72378896977273,-1.,-2.59399625537407));
#55565=CARTESIAN_POINT('Ctrl Pts',(2.72378896977273,1.,-2.59399625537407));
#55566=CARTESIAN_POINT('Ctrl Pts',(2.7197430895797,-1.,-2.59056604771863));
#55567=CARTESIAN_POINT('Ctrl Pts',(2.7197430895797,1.,-2.59056604771863));
#55568=CARTESIAN_POINT('Ctrl Pts',(2.71690570241274,-1.,-2.58804906785077));
#55569=CARTESIAN_POINT('Ctrl Pts',(2.71690570241274,1.,-2.58804906785077));
#55570=CARTESIAN_POINT('Ctrl Pts',(2.71566956750046,-1.,-2.58682657352212));
#55571=CARTESIAN_POINT('Ctrl Pts',(2.71566956750046,1.,-2.58682657352212));
#55572=CARTESIAN_POINT('Ctrl Pts',(2.71533674140979,-1.,-2.58636629903847));
#55573=CARTESIAN_POINT('Ctrl Pts',(2.71533674140979,1.,-2.58636629903847));
#55574=CARTESIAN_POINT('Ctrl Pts',(2.71537879704999,-1.,-2.58626222935706));
#55575=CARTESIAN_POINT('Ctrl Pts',(2.71537879704999,1.,-2.58626222935706));
#55576=CARTESIAN_POINT('Ctrl Pts',(2.71546581445404,-1.,-2.58626089374824));
#55577=CARTESIAN_POINT('Ctrl Pts',(2.71546581445404,1.,-2.58626089374824));
#55578=CARTESIAN_POINT('',(3.14378277984898,1.,-2.78507268004356));
#55579=CARTESIAN_POINT('Ctrl Pts',(3.14378277984898,1.,-2.78507268004356));
#55580=CARTESIAN_POINT('Ctrl Pts',(3.14226401019149,1.,-2.78466475036183));
#55581=CARTESIAN_POINT('Ctrl Pts',(3.13922819750185,1.,-2.78384588958965));
#55582=CARTESIAN_POINT('Ctrl Pts',(3.1346796583452,1.,-2.78260859420629));
#55583=CARTESIAN_POINT('Ctrl Pts',(3.12862530320194,1.,-2.78094085162947));
#55584=CARTESIAN_POINT('Ctrl Pts',(3.12107467038623,1.,-2.77882610147986));
#55585=CARTESIAN_POINT('Ctrl Pts',(3.11354142304692,1.,-2.77668121003225));
#55586=CARTESIAN_POINT('Ctrl Pts',(3.10602568032641,1.,-2.7745060912343));
#55587=CARTESIAN_POINT('Ctrl Pts',(3.09852761277432,1.,-2.77230064795679));
#55588=CARTESIAN_POINT('Ctrl Pts',(3.09104745381882,1.,-2.77006478033937));
#55589=CARTESIAN_POINT('Ctrl Pts',(3.08358548000904,1.,-2.76779837828843));
#55590=CARTESIAN_POINT('Ctrl Pts',(3.07614198408488,1.,-2.76550131064522));
#55591=CARTESIAN_POINT('Ctrl Pts',(3.06871724843121,1.,-2.76317341453415));
#55592=CARTESIAN_POINT('Ctrl Pts',(3.06131152247599,1.,-2.76081448760011));
#55593=CARTESIAN_POINT('Ctrl Pts',(3.05392498750112,1.,-2.75842427253164));
#55594=CARTESIAN_POINT('Ctrl Pts',(3.04655777351333,1.,-2.7560024745616));
#55595=CARTESIAN_POINT('Ctrl Pts',(3.03921001108158,1.,-2.75354880060473));
#55596=CARTESIAN_POINT('Ctrl Pts',(3.03188187589168,1.,-2.75106299523032));
#55597=CARTESIAN_POINT('Ctrl Pts',(3.02457362909199,1.,-2.74854487184099));
#55598=CARTESIAN_POINT('Ctrl Pts',(3.01728567646502,1.,-2.74599436193528));
#55599=CARTESIAN_POINT('Ctrl Pts',(3.01001855960041,1.,-2.7434115023978));
#55600=CARTESIAN_POINT('Ctrl Pts',(3.00277284351431,1.,-2.74079632883852));
#55601=CARTESIAN_POINT('Ctrl Pts',(2.99554902409741,1.,-2.73814878711609));
#55602=CARTESIAN_POINT('Ctrl Pts',(2.98834743696455,1.,-2.73546864694548));
#55603=CARTESIAN_POINT('Ctrl Pts',(2.98116814232175,1.,-2.73275539286537));
#55604=CARTESIAN_POINT('Ctrl Pts',(2.97401089032729,1.,-2.7300081921846));
#55605=CARTESIAN_POINT('Ctrl Pts',(2.96687537842492,1.,-2.72722614084112));
#55606=CARTESIAN_POINT('Ctrl Pts',(2.95976146492595,1.,-2.72440846811745));
#55607=CARTESIAN_POINT('Ctrl Pts',(2.95266939280617,1.,-2.72155475123361));
#55608=CARTESIAN_POINT('Ctrl Pts',(2.94560002559789,1.,-2.71866514227951));
#55609=CARTESIAN_POINT('Ctrl Pts',(2.93855503247248,1.,-2.71574054592575));
#55610=CARTESIAN_POINT('Ctrl Pts',(2.93153633192583,1.,-2.71278207520807));
#55611=CARTESIAN_POINT('Ctrl Pts',(2.92454558914774,1.,-2.70979055994751));
#55612=CARTESIAN_POINT('Ctrl Pts',(2.91758367994738,1.,-2.70676602302518));
#55613=CARTESIAN_POINT('Ctrl Pts',(2.91065019668331,1.,-2.70370719782114));
#55614=CARTESIAN_POINT('Ctrl Pts',(2.90374285605839,1.,-2.70061095078692));
#55615=CARTESIAN_POINT('Ctrl Pts',(2.89685866123668,1.,-2.69747340630621));
#55616=CARTESIAN_POINT('Ctrl Pts',(2.88999512410304,1.,-2.69429113011369));
#55617=CARTESIAN_POINT('Ctrl Pts',(2.88315153980464,1.,-2.69106236420197));
#55618=CARTESIAN_POINT('Ctrl Pts',(2.87633007243885,1.,-2.68778807801691));
#55619=CARTESIAN_POINT('Ctrl Pts',(2.8695373654725,1.,-2.68447353139611));
#55620=CARTESIAN_POINT('Ctrl Pts',(2.86278224277705,1.,-2.68112602796323));
#55621=CARTESIAN_POINT('Ctrl Pts',(2.85607274378031,1.,-2.67775201955736));
#55622=CARTESIAN_POINT('Ctrl Pts',(2.84941315703096,1.,-2.67435421039682));
#55623=CARTESIAN_POINT('Ctrl Pts',(2.84280157191314,1.,-2.67092916452117));
#55624=CARTESIAN_POINT('Ctrl Pts',(2.8362258685396,1.,-2.66746339678085));
#55625=CARTESIAN_POINT('Ctrl Pts',(2.82966813308969,1.,-2.66393764726902));
#55626=CARTESIAN_POINT('Ctrl Pts',(2.82311188135053,1.,-2.66033388273437));
#55627=CARTESIAN_POINT('Ctrl Pts',(2.81654896073874,1.,-2.65664198781335));
#55628=CARTESIAN_POINT('Ctrl Pts',(2.80998526078179,1.,-2.65286529532221));
#55629=CARTESIAN_POINT('Ctrl Pts',(2.80345029781191,1.,-2.64902988983373));
#55630=CARTESIAN_POINT('Ctrl Pts',(2.7969891067079,1.,-2.6451766779937));
#55631=CARTESIAN_POINT('Ctrl Pts',(2.79064495573275,1.,-2.64134450532632));
#55632=CARTESIAN_POINT('Ctrl Pts',(2.78444351041594,1.,-2.63755471430322));
#55633=CARTESIAN_POINT('Ctrl Pts',(2.77837943466423,1.,-2.63379800904575));
#55634=CARTESIAN_POINT('Ctrl Pts',(2.77239433377839,1.,-2.63001305229548));
#55635=CARTESIAN_POINT('Ctrl Pts',(2.76639078478898,1.,-2.6260995650624));
#55636=CARTESIAN_POINT('Ctrl Pts',(2.76027271596564,1.,-2.62195665834491));
#55637=CARTESIAN_POINT('Ctrl Pts',(2.75398025025967,1.,-2.61751580407608));
#55638=CARTESIAN_POINT('Ctrl Pts',(2.74752219567307,1.,-2.61277170105864));
#55639=CARTESIAN_POINT('Ctrl Pts',(2.74102110999284,1.,-2.60782480638629));
#55640=CARTESIAN_POINT('Ctrl Pts',(2.73470730109906,1.,-2.60287635689));
#55641=CARTESIAN_POINT('Ctrl Pts',(2.72886483481804,1.,-2.5981786903501));
#55642=CARTESIAN_POINT('Ctrl Pts',(2.72378896977273,1.,-2.59399625537407));
#55643=CARTESIAN_POINT('Ctrl Pts',(2.7197430895797,1.,-2.59056604771863));
#55644=CARTESIAN_POINT('Ctrl Pts',(2.7171186028189,1.,-2.58823792682724));
#55645=CARTESIAN_POINT('Ctrl Pts',(2.71591054189884,1.,-2.58706285424469));
#55646=CARTESIAN_POINT('Ctrl Pts',(2.71548946460616,1.,-2.58656037976884));
#55647=CARTESIAN_POINT('Ctrl Pts',(2.71540296615967,1.,-2.58638312917291));
#55648=CARTESIAN_POINT('Ctrl Pts',(2.71539546306824,1.,-2.58633475775051));
#55649=CARTESIAN_POINT('',(3.14378277984898,0.,-2.78507268004356));
#55650=CARTESIAN_POINT('Ctrl Pts',(2.97921217251145,-1.,-2.27745358485296));
#55651=CARTESIAN_POINT('Ctrl Pts',(2.97921217251145,1.,-2.27745358485296));
#55652=CARTESIAN_POINT('Ctrl Pts',(2.97919987915678,-1.,-2.27736742984319));
#55653=CARTESIAN_POINT('Ctrl Pts',(2.97919987915678,1.,-2.27736742984319));
#55654=CARTESIAN_POINT('Ctrl Pts',(2.97929608861798,-1.,-2.2773096118942));
#55655=CARTESIAN_POINT('Ctrl Pts',(2.97929608861798,1.,-2.2773096118942));
#55656=CARTESIAN_POINT('Ctrl Pts',(2.97980276183181,-1.,-2.27756633755188));
#55657=CARTESIAN_POINT('Ctrl Pts',(2.97980276183181,1.,-2.27756633755188));
#55658=CARTESIAN_POINT('Ctrl Pts',(2.98120357932994,-1.,-2.27859601334547));
#55659=CARTESIAN_POINT('Ctrl Pts',(2.98120357932994,1.,-2.27859601334547));
#55660=CARTESIAN_POINT('Ctrl Pts',(2.98413343613983,-1.,-2.28100472516679));
#55661=CARTESIAN_POINT('Ctrl Pts',(2.98413343613983,1.,-2.28100472516679));
#55662=CARTESIAN_POINT('Ctrl Pts',(2.9881543273478,-1.,-2.28446419115919));
#55663=CARTESIAN_POINT('Ctrl Pts',(2.9881543273478,1.,-2.28446419115919));
#55664=CARTESIAN_POINT('Ctrl Pts',(2.99307930984034,-1.,-2.28882328690362));
#55665=CARTESIAN_POINT('Ctrl Pts',(2.99307930984034,1.,-2.28882328690362));
#55666=CARTESIAN_POINT('Ctrl Pts',(2.99863310339691,-1.,-2.29385894577754));
#55667=CARTESIAN_POINT('Ctrl Pts',(2.99863310339691,1.,-2.29385894577754));
#55668=CARTESIAN_POINT('Ctrl Pts',(3.00450832658613,-1.,-2.29932091315775));
#55669=CARTESIAN_POINT('Ctrl Pts',(3.00450832658613,1.,-2.29932091315775));
#55670=CARTESIAN_POINT('Ctrl Pts',(3.01041131063823,-1.,-2.30496809486482));
#55671=CARTESIAN_POINT('Ctrl Pts',(3.01041131063823,1.,-2.30496809486482));
#55672=CARTESIAN_POINT('Ctrl Pts',(3.01610726819086,-1.,-2.31060449886629));
#55673=CARTESIAN_POINT('Ctrl Pts',(3.01610726819086,1.,-2.31060449886629));
#55674=CARTESIAN_POINT('Ctrl Pts',(3.0214778066816,-1.,-2.31612479121631));
#55675=CARTESIAN_POINT('Ctrl Pts',(3.0214778066816,1.,-2.31612479121631));
#55676=CARTESIAN_POINT('Ctrl Pts',(3.02652678416611,-1.,-2.32151944306402));
#55677=CARTESIAN_POINT('Ctrl Pts',(3.02652678416611,1.,-2.32151944306402));
#55678=CARTESIAN_POINT('Ctrl Pts',(3.03133125185136,-1.,-2.32683687412097));
#55679=CARTESIAN_POINT('Ctrl Pts',(3.03133125185136,1.,-2.32683687412097));
#55680=CARTESIAN_POINT('Ctrl Pts',(3.03600588555793,-1.,-2.33215619079829));
#55681=CARTESIAN_POINT('Ctrl Pts',(3.03600588555793,1.,-2.33215619079829));
#55682=CARTESIAN_POINT('Ctrl Pts',(3.04066496998544,-1.,-2.33755792953706));
#55683=CARTESIAN_POINT('Ctrl Pts',(3.04066496998544,1.,-2.33755792953706));
#55684=CARTESIAN_POINT('Ctrl Pts',(3.04537822217256,-1.,-2.34309017083977));
#55685=CARTESIAN_POINT('Ctrl Pts',(3.04537822217256,1.,-2.34309017083977));
#55686=CARTESIAN_POINT('Ctrl Pts',(3.05015565829918,-1.,-2.34875673090771));
#55687=CARTESIAN_POINT('Ctrl Pts',(3.05015565829918,1.,-2.34875673090771));
#55688=CARTESIAN_POINT('Ctrl Pts',(3.05497218368146,-1.,-2.35453559889474));
#55689=CARTESIAN_POINT('Ctrl Pts',(3.05497218368146,1.,-2.35453559889474));
#55690=CARTESIAN_POINT('Ctrl Pts',(3.0597826624004,-1.,-2.36039011602072));
#55691=CARTESIAN_POINT('Ctrl Pts',(3.0597826624004,1.,-2.36039011602072));
#55692=CARTESIAN_POINT('Ctrl Pts',(3.06453964643162,-1.,-2.36628220107009));
#55693=CARTESIAN_POINT('Ctrl Pts',(3.06453964643162,1.,-2.36628220107009));
#55694=CARTESIAN_POINT('Ctrl Pts',(3.069212754975,-1.,-2.37218678163178));
#55695=CARTESIAN_POINT('Ctrl Pts',(3.069212754975,1.,-2.37218678163178));
#55696=CARTESIAN_POINT('Ctrl Pts',(3.07379777492165,-1.,-2.37809856205548));
#55697=CARTESIAN_POINT('Ctrl Pts',(3.07379777492165,1.,-2.37809856205548));
#55698=CARTESIAN_POINT('Ctrl Pts',(3.07830597244326,-1.,-2.38402401216126));
#55699=CARTESIAN_POINT('Ctrl Pts',(3.07830597244326,1.,-2.38402401216126));
#55700=CARTESIAN_POINT('Ctrl Pts',(3.08275773747093,-1.,-2.38997659219199));
#55701=CARTESIAN_POINT('Ctrl Pts',(3.08275773747093,1.,-2.38997659219199));
#55702=CARTESIAN_POINT('Ctrl Pts',(3.08717489512914,-1.,-2.39597098250631));
#55703=CARTESIAN_POINT('Ctrl Pts',(3.08717489512914,1.,-2.39597098250631));
#55704=CARTESIAN_POINT('Ctrl Pts',(3.091572660511,-1.,-2.40201704423341));
#55705=CARTESIAN_POINT('Ctrl Pts',(3.091572660511,1.,-2.40201704423341));
#55706=CARTESIAN_POINT('Ctrl Pts',(3.09595472616076,-1.,-2.40811612696369));
#55707=CARTESIAN_POINT('Ctrl Pts',(3.09595472616076,1.,-2.40811612696369));
#55708=CARTESIAN_POINT('Ctrl Pts',(3.1003177502767,-1.,-2.41426441798057));
#55709=CARTESIAN_POINT('Ctrl Pts',(3.1003177502767,1.,-2.41426441798057));
#55710=CARTESIAN_POINT('Ctrl Pts',(3.10465410280896,-1.,-2.42045498612489));
#55711=CARTESIAN_POINT('Ctrl Pts',(3.10465410280896,1.,-2.42045498612489));
#55712=CARTESIAN_POINT('Ctrl Pts',(3.10895518969595,-1.,-2.42668025870015));
#55713=CARTESIAN_POINT('Ctrl Pts',(3.10895518969595,1.,-2.42668025870015));
#55714=CARTESIAN_POINT('Ctrl Pts',(3.11321477659018,-1.,-2.43293449685144));
#55715=CARTESIAN_POINT('Ctrl Pts',(3.11321477659018,1.,-2.43293449685144));
#55716=CARTESIAN_POINT('Ctrl Pts',(3.11743156744186,-1.,-2.43921571477977));
#55717=CARTESIAN_POINT('Ctrl Pts',(3.11743156744186,1.,-2.43921571477977));
#55718=CARTESIAN_POINT('Ctrl Pts',(3.12160740887768,-1.,-2.44552433364715));
#55719=CARTESIAN_POINT('Ctrl Pts',(3.12160740887768,1.,-2.44552433364715));
#55720=CARTESIAN_POINT('Ctrl Pts',(3.12574608210847,-1.,-2.45186227369846));
#55721=CARTESIAN_POINT('Ctrl Pts',(3.12574608210847,1.,-2.45186227369846));
#55722=CARTESIAN_POINT('Ctrl Pts',(3.12985188384371,-1.,-2.45823188859366));
#55723=CARTESIAN_POINT('Ctrl Pts',(3.12985188384371,1.,-2.45823188859366));
#55724=CARTESIAN_POINT('Ctrl Pts',(3.13392826623906,-1.,-2.46463494332374));
#55725=CARTESIAN_POINT('Ctrl Pts',(3.13392826623906,1.,-2.46463494332374));
#55726=CARTESIAN_POINT('Ctrl Pts',(3.13797654408943,-1.,-2.47107164236838));
#55727=CARTESIAN_POINT('Ctrl Pts',(3.13797654408943,1.,-2.47107164236838));
#55728=CARTESIAN_POINT('Ctrl Pts',(3.14199655778863,-1.,-2.47754112428043));
#55729=CARTESIAN_POINT('Ctrl Pts',(3.14199655778863,1.,-2.47754112428043));
#55730=CARTESIAN_POINT('Ctrl Pts',(3.14598722723896,-1.,-2.4840418741839));
#55731=CARTESIAN_POINT('Ctrl Pts',(3.14598722723896,1.,-2.4840418741839));
#55732=CARTESIAN_POINT('Ctrl Pts',(3.14994715298907,-1.,-2.49057217131988));
#55733=CARTESIAN_POINT('Ctrl Pts',(3.14994715298907,1.,-2.49057217131988));
#55734=CARTESIAN_POINT('Ctrl Pts',(3.15387518039046,-1.,-2.49713050858896));
#55735=CARTESIAN_POINT('Ctrl Pts',(3.15387518039046,1.,-2.49713050858896));
#55736=CARTESIAN_POINT('Ctrl Pts',(3.15777102413957,-1.,-2.50371605688252));
#55737=CARTESIAN_POINT('Ctrl Pts',(3.15777102413957,1.,-2.50371605688252));
#55738=CARTESIAN_POINT('Ctrl Pts',(3.16163506380157,-1.,-2.51032851007894));
#55739=CARTESIAN_POINT('Ctrl Pts',(3.16163506380157,1.,-2.51032851007894));
#55740=CARTESIAN_POINT('Ctrl Pts',(3.16546808277023,-1.,-2.51696788755577));
#55741=CARTESIAN_POINT('Ctrl Pts',(3.16546808277023,1.,-2.51696788755577));
#55742=CARTESIAN_POINT('Ctrl Pts',(3.16927102130735,-1.,-2.52363434671788));
#55743=CARTESIAN_POINT('Ctrl Pts',(3.16927102130735,1.,-2.52363434671788));
#55744=CARTESIAN_POINT('Ctrl Pts',(3.17304474093612,-1.,-2.53032800406941));
#55745=CARTESIAN_POINT('Ctrl Pts',(3.17304474093612,1.,-2.53032800406941));
#55746=CARTESIAN_POINT('Ctrl Pts',(3.17678974135318,-1.,-2.53704871950948));
#55747=CARTESIAN_POINT('Ctrl Pts',(3.17678974135318,1.,-2.53704871950948));
#55748=CARTESIAN_POINT('Ctrl Pts',(3.18050619750639,-1.,-2.54379612553051));
#55749=CARTESIAN_POINT('Ctrl Pts',(3.18050619750639,1.,-2.54379612553051));
#55750=CARTESIAN_POINT('Ctrl Pts',(3.18419408529594,-1.,-2.55056972387731));
#55751=CARTESIAN_POINT('Ctrl Pts',(3.18419408529594,1.,-2.55056972387731));
#55752=CARTESIAN_POINT('Ctrl Pts',(3.18785328116218,-1.,-2.55736896206056));
#55753=CARTESIAN_POINT('Ctrl Pts',(3.18785328116218,1.,-2.55736896206056));
#55754=CARTESIAN_POINT('Ctrl Pts',(3.19148366395139,-1.,-2.56419331092858));
#55755=CARTESIAN_POINT('Ctrl Pts',(3.19148366395139,1.,-2.56419331092858));
#55756=CARTESIAN_POINT('Ctrl Pts',(3.19508523784363,-1.,-2.57104235897899));
#55757=CARTESIAN_POINT('Ctrl Pts',(3.19508523784363,1.,-2.57104235897899));
#55758=CARTESIAN_POINT('Ctrl Pts',(3.19865814628682,-1.,-2.57791581908875));
#55759=CARTESIAN_POINT('Ctrl Pts',(3.19865814628682,1.,-2.57791581908875));
#55760=CARTESIAN_POINT('Ctrl Pts',(3.20220261408414,-1.,-2.58481347777729));
#55761=CARTESIAN_POINT('Ctrl Pts',(3.20220261408414,1.,-2.58481347777729));
#55762=CARTESIAN_POINT('Ctrl Pts',(3.2057189102873,-1.,-2.59173516023481));
#55763=CARTESIAN_POINT('Ctrl Pts',(3.2057189102873,1.,-2.59173516023481));
#55764=CARTESIAN_POINT('Ctrl Pts',(3.20920730569681,-1.,-2.59868069194342));
#55765=CARTESIAN_POINT('Ctrl Pts',(3.20920730569681,1.,-2.59868069194342));
#55766=CARTESIAN_POINT('Ctrl Pts',(3.21266802609681,-1.,-2.60564985360017));
#55767=CARTESIAN_POINT('Ctrl Pts',(3.21266802609681,1.,-2.60564985360017));
#55768=CARTESIAN_POINT('Ctrl Pts',(3.21610123233082,-1.,-2.61264236719171));
#55769=CARTESIAN_POINT('Ctrl Pts',(3.21610123233082,1.,-2.61264236719171));
#55770=CARTESIAN_POINT('Ctrl Pts',(3.21950704109321,-1.,-2.61965792832947));
#55771=CARTESIAN_POINT('Ctrl Pts',(3.21950704109321,1.,-2.61965792832947));
#55772=CARTESIAN_POINT('Ctrl Pts',(3.2228855361324,-1.,-2.62669622735912));
#55773=CARTESIAN_POINT('Ctrl Pts',(3.2228855361324,1.,-2.62669622735912));
#55774=CARTESIAN_POINT('Ctrl Pts',(3.2262367829246,-1.,-2.63375697391372));
#55775=CARTESIAN_POINT('Ctrl Pts',(3.2262367829246,1.,-2.63375697391372));
#55776=CARTESIAN_POINT('Ctrl Pts',(3.22956084358547,-1.,-2.64083992181823));
#55777=CARTESIAN_POINT('Ctrl Pts',(3.22956084358547,1.,-2.64083992181823));
#55778=CARTESIAN_POINT('Ctrl Pts',(3.23285778737096,-1.,-2.64794488743038));
#55779=CARTESIAN_POINT('Ctrl Pts',(3.23285778737096,1.,-2.64794488743038));
#55780=CARTESIAN_POINT('Ctrl Pts',(3.236127680639,-1.,-2.65507173961555));
#55781=CARTESIAN_POINT('Ctrl Pts',(3.236127680639,1.,-2.65507173961555));
#55782=CARTESIAN_POINT('Ctrl Pts',(3.23872200034785,-1.,-2.6607906631847));
#55783=CARTESIAN_POINT('Ctrl Pts',(3.23872200034785,1.,-2.6607906631847));
#55784=CARTESIAN_POINT('Ctrl Pts',(3.24065561086749,-1.,-2.66508964663997));
#55785=CARTESIAN_POINT('Ctrl Pts',(3.24065561086749,1.,-2.66508964663997));
#55786=CARTESIAN_POINT('Ctrl Pts',(3.24193929584471,-1.,-2.66795998539579));
#55787=CARTESIAN_POINT('Ctrl Pts',(3.24193929584471,1.,-2.66795998539579));
#55788=CARTESIAN_POINT('Ctrl Pts',(3.24257979115744,-1.,-2.66939624221984));
#55789=CARTESIAN_POINT('Ctrl Pts',(3.24257979115744,1.,-2.66939624221984));
#55790=CARTESIAN_POINT('',(2.97927412174279,1.,-2.27737254473521));
#55791=CARTESIAN_POINT('Ctrl Pts',(2.97927412174279,-1.,-2.27737254473521));
#55792=CARTESIAN_POINT('Ctrl Pts',(2.97927412174279,-0.666666666666667,
-2.27737254473521));
#55793=CARTESIAN_POINT('Ctrl Pts',(2.97927412174279,-0.333333333333333,
-2.27737254473521));
#55794=CARTESIAN_POINT('Ctrl Pts',(2.97927412174279,0.333333333333333,-2.27737254473521));
#55795=CARTESIAN_POINT('Ctrl Pts',(2.97927412174279,0.666666666666667,-2.27737254473521));
#55796=CARTESIAN_POINT('Ctrl Pts',(2.97927412174279,1.,-2.27737254473521));
#55797=CARTESIAN_POINT('',(3.24257979115744,1.,-2.66939624221984));
#55798=CARTESIAN_POINT('',(3.24257979115744,0.,-2.66939624221984));
#55799=CARTESIAN_POINT('Ctrl Pts',(2.97927412174279,1.,-2.27737254473521));
#55800=CARTESIAN_POINT('Ctrl Pts',(2.97932307137476,1.,-2.27737238849287));
#55801=CARTESIAN_POINT('Ctrl Pts',(2.9795116710597,1.,-2.27743009389684));
#55802=CARTESIAN_POINT('Ctrl Pts',(2.98007383024207,1.,-2.27776738270289));
#55803=CARTESIAN_POINT('Ctrl Pts',(2.9814234180956,1.,-2.27877674853766));
#55804=CARTESIAN_POINT('Ctrl Pts',(2.98413343613983,1.,-2.28100472516679));
#55805=CARTESIAN_POINT('Ctrl Pts',(2.9881543273478,1.,-2.28446419115919));
#55806=CARTESIAN_POINT('Ctrl Pts',(2.99307930984034,1.,-2.28882328690362));
#55807=CARTESIAN_POINT('Ctrl Pts',(2.99863310339691,1.,-2.29385894577754));
#55808=CARTESIAN_POINT('Ctrl Pts',(3.00450832658613,1.,-2.29932091315775));
#55809=CARTESIAN_POINT('Ctrl Pts',(3.01041131063823,1.,-2.30496809486482));
#55810=CARTESIAN_POINT('Ctrl Pts',(3.01610726819086,1.,-2.31060449886629));
#55811=CARTESIAN_POINT('Ctrl Pts',(3.0214778066816,1.,-2.31612479121631));
#55812=CARTESIAN_POINT('Ctrl Pts',(3.02652678416611,1.,-2.32151944306402));
#55813=CARTESIAN_POINT('Ctrl Pts',(3.03133125185136,1.,-2.32683687412097));
#55814=CARTESIAN_POINT('Ctrl Pts',(3.03600588555793,1.,-2.33215619079829));
#55815=CARTESIAN_POINT('Ctrl Pts',(3.04066496998544,1.,-2.33755792953706));
#55816=CARTESIAN_POINT('Ctrl Pts',(3.04537822217256,1.,-2.34309017083977));
#55817=CARTESIAN_POINT('Ctrl Pts',(3.05015565829918,1.,-2.34875673090771));
#55818=CARTESIAN_POINT('Ctrl Pts',(3.05497218368146,1.,-2.35453559889474));
#55819=CARTESIAN_POINT('Ctrl Pts',(3.0597826624004,1.,-2.36039011602072));
#55820=CARTESIAN_POINT('Ctrl Pts',(3.06453964643162,1.,-2.36628220107009));
#55821=CARTESIAN_POINT('Ctrl Pts',(3.069212754975,1.,-2.37218678163178));
#55822=CARTESIAN_POINT('Ctrl Pts',(3.07379777492165,1.,-2.37809856205548));
#55823=CARTESIAN_POINT('Ctrl Pts',(3.07830597244326,1.,-2.38402401216126));
#55824=CARTESIAN_POINT('Ctrl Pts',(3.08275773747093,1.,-2.38997659219199));
#55825=CARTESIAN_POINT('Ctrl Pts',(3.08717489512914,1.,-2.39597098250631));
#55826=CARTESIAN_POINT('Ctrl Pts',(3.091572660511,1.,-2.40201704423341));
#55827=CARTESIAN_POINT('Ctrl Pts',(3.09595472616076,1.,-2.40811612696369));
#55828=CARTESIAN_POINT('Ctrl Pts',(3.1003177502767,1.,-2.41426441798057));
#55829=CARTESIAN_POINT('Ctrl Pts',(3.10465410280896,1.,-2.42045498612489));
#55830=CARTESIAN_POINT('Ctrl Pts',(3.10895518969595,1.,-2.42668025870015));
#55831=CARTESIAN_POINT('Ctrl Pts',(3.11321477659018,1.,-2.43293449685144));
#55832=CARTESIAN_POINT('Ctrl Pts',(3.11743156744186,1.,-2.43921571477977));
#55833=CARTESIAN_POINT('Ctrl Pts',(3.12160740887768,1.,-2.44552433364715));
#55834=CARTESIAN_POINT('Ctrl Pts',(3.12574608210847,1.,-2.45186227369846));
#55835=CARTESIAN_POINT('Ctrl Pts',(3.12985188384371,1.,-2.45823188859366));
#55836=CARTESIAN_POINT('Ctrl Pts',(3.13392826623906,1.,-2.46463494332374));
#55837=CARTESIAN_POINT('Ctrl Pts',(3.13797654408943,1.,-2.47107164236838));
#55838=CARTESIAN_POINT('Ctrl Pts',(3.14199655778863,1.,-2.47754112428043));
#55839=CARTESIAN_POINT('Ctrl Pts',(3.14598722723896,1.,-2.4840418741839));
#55840=CARTESIAN_POINT('Ctrl Pts',(3.14994715298907,1.,-2.49057217131988));
#55841=CARTESIAN_POINT('Ctrl Pts',(3.15387518039046,1.,-2.49713050858896));
#55842=CARTESIAN_POINT('Ctrl Pts',(3.15777102413957,1.,-2.50371605688252));
#55843=CARTESIAN_POINT('Ctrl Pts',(3.16163506380157,1.,-2.51032851007894));
#55844=CARTESIAN_POINT('Ctrl Pts',(3.16546808277023,1.,-2.51696788755577));
#55845=CARTESIAN_POINT('Ctrl Pts',(3.16927102130735,1.,-2.52363434671788));
#55846=CARTESIAN_POINT('Ctrl Pts',(3.17304474093612,1.,-2.53032800406941));
#55847=CARTESIAN_POINT('Ctrl Pts',(3.17678974135318,1.,-2.53704871950948));
#55848=CARTESIAN_POINT('Ctrl Pts',(3.18050619750639,1.,-2.54379612553051));
#55849=CARTESIAN_POINT('Ctrl Pts',(3.18419408529594,1.,-2.55056972387731));
#55850=CARTESIAN_POINT('Ctrl Pts',(3.18785328116218,1.,-2.55736896206056));
#55851=CARTESIAN_POINT('Ctrl Pts',(3.19148366395139,1.,-2.56419331092858));
#55852=CARTESIAN_POINT('Ctrl Pts',(3.19508523784363,1.,-2.57104235897899));
#55853=CARTESIAN_POINT('Ctrl Pts',(3.19865814628682,1.,-2.57791581908875));
#55854=CARTESIAN_POINT('Ctrl Pts',(3.20220261408414,1.,-2.58481347777729));
#55855=CARTESIAN_POINT('Ctrl Pts',(3.2057189102873,1.,-2.59173516023481));
#55856=CARTESIAN_POINT('Ctrl Pts',(3.20920730569681,1.,-2.59868069194342));
#55857=CARTESIAN_POINT('Ctrl Pts',(3.21266802609681,1.,-2.60564985360017));
#55858=CARTESIAN_POINT('Ctrl Pts',(3.21610123233082,1.,-2.61264236719171));
#55859=CARTESIAN_POINT('Ctrl Pts',(3.21950704109321,1.,-2.61965792832947));
#55860=CARTESIAN_POINT('Ctrl Pts',(3.2228855361324,1.,-2.62669622735912));
#55861=CARTESIAN_POINT('Ctrl Pts',(3.2262367829246,1.,-2.63375697391372));
#55862=CARTESIAN_POINT('Ctrl Pts',(3.22956084358547,1.,-2.64083992181823));
#55863=CARTESIAN_POINT('Ctrl Pts',(3.23285778737096,1.,-2.64794488743038));
#55864=CARTESIAN_POINT('Ctrl Pts',(3.236127680639,1.,-2.65507173961555));
#55865=CARTESIAN_POINT('Ctrl Pts',(3.23872200034785,1.,-2.6607906631847));
#55866=CARTESIAN_POINT('Ctrl Pts',(3.24065561086749,1.,-2.66508964663997));
#55867=CARTESIAN_POINT('Ctrl Pts',(3.24193929584471,1.,-2.66795998539579));
#55868=CARTESIAN_POINT('Ctrl Pts',(3.24257979115744,1.,-2.66939624221984));
#55869=CARTESIAN_POINT('Origin',(3.24257979115744,0.,-2.66939624221984));
#55870=CARTESIAN_POINT('',(3.14378277984898,1.,-2.78507268004356));
#55871=CARTESIAN_POINT('Origin',(0.,0.,0.));
#55872=CARTESIAN_POINT('',(3.08655633322109,1.,-2.12971124846838));
#55873=CARTESIAN_POINT('Origin',(0.,1.,0.));
#55874=CARTESIAN_POINT('Ctrl Pts',(3.0865563332211,1.,-2.12971124846838));
#55875=CARTESIAN_POINT('Ctrl Pts',(3.0865563332211,0.666666666666667,-2.12971124846838));
#55876=CARTESIAN_POINT('Ctrl Pts',(3.0865563332211,0.333333333333333,-2.12971124846838));
#55877=CARTESIAN_POINT('Ctrl Pts',(3.0865563332211,-0.333333333333333,-2.12971124846838));
#55878=CARTESIAN_POINT('Ctrl Pts',(3.0865563332211,-0.666666666666667,-2.12971124846838));
#55879=CARTESIAN_POINT('Ctrl Pts',(3.0865563332211,-1.,-2.12971124846838));
#55880=CARTESIAN_POINT('Ctrl Pts',(3.54075895182139,-1.,-2.25898783642071));
#55881=CARTESIAN_POINT('Ctrl Pts',(3.54075895182139,1.,-2.25898783642071));
#55882=CARTESIAN_POINT('Ctrl Pts',(3.5391950664771,-1.,-2.25882251694918));
#55883=CARTESIAN_POINT('Ctrl Pts',(3.5391950664771,1.,-2.25882251694918));
#55884=CARTESIAN_POINT('Ctrl Pts',(3.53606853163247,-1.,-2.25848864344599));
#55885=CARTESIAN_POINT('Ctrl Pts',(3.53606853163247,1.,-2.25848864344599));
#55886=CARTESIAN_POINT('Ctrl Pts',(3.53138243689932,-1.,-2.25797812951166));
#55887=CARTESIAN_POINT('Ctrl Pts',(3.53138243689932,1.,-2.25797812951166));
#55888=CARTESIAN_POINT('Ctrl Pts',(3.52514172849666,-1.,-2.25727802942142));
#55889=CARTESIAN_POINT('Ctrl Pts',(3.52514172849666,1.,-2.25727802942142));
#55890=CARTESIAN_POINT('Ctrl Pts',(3.51735323669213,-1.,-2.25637049456061));
#55891=CARTESIAN_POINT('Ctrl Pts',(3.51735323669213,1.,-2.25637049456061));
#55892=CARTESIAN_POINT('Ctrl Pts',(3.50957720118209,-1.,-2.25543046980351));
#55893=CARTESIAN_POINT('Ctrl Pts',(3.50957720118209,1.,-2.25543046980351));
#55894=CARTESIAN_POINT('Ctrl Pts',(3.50181372618058,-1.,-2.25445785151923));
#55895=CARTESIAN_POINT('Ctrl Pts',(3.50181372618058,1.,-2.25445785151923));
#55896=CARTESIAN_POINT('Ctrl Pts',(3.49406296494309,-1.,-2.25345251709453));
#55897=CARTESIAN_POINT('Ctrl Pts',(3.49406296494309,1.,-2.25345251709453));
#55898=CARTESIAN_POINT('Ctrl Pts',(3.48632513240231,-1.,-2.25241433138231));
#55899=CARTESIAN_POINT('Ctrl Pts',(3.48632513240231,1.,-2.25241433138231));
#55900=CARTESIAN_POINT('Ctrl Pts',(3.47860048448015,-1.,-2.25134314238258));
#55901=CARTESIAN_POINT('Ctrl Pts',(3.47860048448015,1.,-2.25134314238258));
#55902=CARTESIAN_POINT('Ctrl Pts',(3.47088928979467,-1.,-2.25023877475674));
#55903=CARTESIAN_POINT('Ctrl Pts',(3.47088928979467,1.,-2.25023877475674));
#55904=CARTESIAN_POINT('Ctrl Pts',(3.46319180177474,-1.,-2.24910102345977));
#55905=CARTESIAN_POINT('Ctrl Pts',(3.46319180177474,1.,-2.24910102345977));
#55906=CARTESIAN_POINT('Ctrl Pts',(3.45550823512213,-1.,-2.24792964960874));
#55907=CARTESIAN_POINT('Ctrl Pts',(3.45550823512213,1.,-2.24792964960874));
#55908=CARTESIAN_POINT('Ctrl Pts',(3.44783872863448,-1.,-2.24672437070139));
#55909=CARTESIAN_POINT('Ctrl Pts',(3.44783872863448,1.,-2.24672437070139));
#55910=CARTESIAN_POINT('Ctrl Pts',(3.44018336460619,-1.,-2.24548487526212));
#55911=CARTESIAN_POINT('Ctrl Pts',(3.44018336460619,1.,-2.24548487526212));
#55912=CARTESIAN_POINT('Ctrl Pts',(3.43254222615007,-1.,-2.24421085338856));
#55913=CARTESIAN_POINT('Ctrl Pts',(3.43254222615007,1.,-2.24421085338856));
#55914=CARTESIAN_POINT('Ctrl Pts',(3.42491544683075,-1.,-2.24290202531144));
#55915=CARTESIAN_POINT('Ctrl Pts',(3.42491544683075,1.,-2.24290202531144));
#55916=CARTESIAN_POINT('Ctrl Pts',(3.41730325539119,-1.,-2.24155816587811));
#55917=CARTESIAN_POINT('Ctrl Pts',(3.41730325539119,1.,-2.24155816587811));
#55918=CARTESIAN_POINT('Ctrl Pts',(3.40970604190205,-1.,-2.24017914395211));
#55919=CARTESIAN_POINT('Ctrl Pts',(3.40970604190205,1.,-2.24017914395211));
#55920=CARTESIAN_POINT('Ctrl Pts',(3.40212434705511,-1.,-2.23876491124064));
#55921=CARTESIAN_POINT('Ctrl Pts',(3.40212434705511,1.,-2.23876491124064));
#55922=CARTESIAN_POINT('Ctrl Pts',(3.39455873448088,-1.,-2.23731541452727));
#55923=CARTESIAN_POINT('Ctrl Pts',(3.39455873448088,1.,-2.23731541452727));
#55924=CARTESIAN_POINT('Ctrl Pts',(3.38700968549522,-1.,-2.23583052276281));
#55925=CARTESIAN_POINT('Ctrl Pts',(3.38700968549522,1.,-2.23583052276281));
#55926=CARTESIAN_POINT('Ctrl Pts',(3.37947749555649,-1.,-2.23430995599572));
#55927=CARTESIAN_POINT('Ctrl Pts',(3.37947749555649,1.,-2.23430995599572));
#55928=CARTESIAN_POINT('Ctrl Pts',(3.37196214349356,-1.,-2.23275319569253));
#55929=CARTESIAN_POINT('Ctrl Pts',(3.37196214349356,1.,-2.23275319569253));
#55930=CARTESIAN_POINT('Ctrl Pts',(3.36446325227908,-1.,-2.23115945849777));
#55931=CARTESIAN_POINT('Ctrl Pts',(3.36446325227908,1.,-2.23115945849777));
#55932=CARTESIAN_POINT('Ctrl Pts',(3.35698038165529,-1.,-2.22952789881011));
#55933=CARTESIAN_POINT('Ctrl Pts',(3.35698038165529,1.,-2.22952789881011));
#55934=CARTESIAN_POINT('Ctrl Pts',(3.34951327111117,-1.,-2.22785777756588));
#55935=CARTESIAN_POINT('Ctrl Pts',(3.34951327111117,1.,-2.22785777756588));
#55936=CARTESIAN_POINT('Ctrl Pts',(3.34206209449371,-1.,-2.22614863918044));
#55937=CARTESIAN_POINT('Ctrl Pts',(3.34206209449371,1.,-2.22614863918044));
#55938=CARTESIAN_POINT('Ctrl Pts',(3.3346277284958,-1.,-2.224400498785));
#55939=CARTESIAN_POINT('Ctrl Pts',(3.3346277284958,1.,-2.224400498785));
#55940=CARTESIAN_POINT('Ctrl Pts',(3.32721196326019,-1.,-2.22261398879623));
#55941=CARTESIAN_POINT('Ctrl Pts',(3.32721196326019,1.,-2.22261398879623));
#55942=CARTESIAN_POINT('Ctrl Pts',(3.31981686778008,-1.,-2.22078990842768));
#55943=CARTESIAN_POINT('Ctrl Pts',(3.31981686778008,1.,-2.22078990842768));
#55944=CARTESIAN_POINT('Ctrl Pts',(3.31244421655662,-1.,-2.21892881679083));
#55945=CARTESIAN_POINT('Ctrl Pts',(3.31244421655662,1.,-2.21892881679083));
#55946=CARTESIAN_POINT('Ctrl Pts',(3.3050948781957,-1.,-2.21703059947837));
#55947=CARTESIAN_POINT('Ctrl Pts',(3.3050948781957,1.,-2.21703059947837));
#55948=CARTESIAN_POINT('Ctrl Pts',(3.29776825193162,-1.,-2.2150940692337));
#55949=CARTESIAN_POINT('Ctrl Pts',(3.29776825193162,1.,-2.2150940692337));
#55950=CARTESIAN_POINT('Ctrl Pts',(3.29046159238344,-1.,-2.21311648827391));
#55951=CARTESIAN_POINT('Ctrl Pts',(3.29046159238344,1.,-2.21311648827391));
#55952=CARTESIAN_POINT('Ctrl Pts',(3.28317133333127,-1.,-2.21109449750638));
#55953=CARTESIAN_POINT('Ctrl Pts',(3.28317133333127,1.,-2.21109449750638));
#55954=CARTESIAN_POINT('Ctrl Pts',(3.27589448005534,-1.,-2.20902509417425));
#55955=CARTESIAN_POINT('Ctrl Pts',(3.27589448005534,1.,-2.20902509417425));
#55956=CARTESIAN_POINT('Ctrl Pts',(3.2686300613678,-1.,-2.20690665217741));
#55957=CARTESIAN_POINT('Ctrl Pts',(3.2686300613678,1.,-2.20690665217741));
#55958=CARTESIAN_POINT('Ctrl Pts',(3.26138036637711,-1.,-2.20473979048682));
#55959=CARTESIAN_POINT('Ctrl Pts',(3.26138036637711,1.,-2.20473979048682));
#55960=CARTESIAN_POINT('Ctrl Pts',(3.25415277957789,-1.,-2.20252866491554));
#55961=CARTESIAN_POINT('Ctrl Pts',(3.25415277957789,1.,-2.20252866491554));
#55962=CARTESIAN_POINT('Ctrl Pts',(3.24695715874356,-1.,-2.20027910880993));
#55963=CARTESIAN_POINT('Ctrl Pts',(3.24695715874356,1.,-2.20027910880993));
#55964=CARTESIAN_POINT('Ctrl Pts',(3.23980245361323,-1.,-2.19799623693263));
#55965=CARTESIAN_POINT('Ctrl Pts',(3.23980245361323,1.,-2.19799623693263));
#55966=CARTESIAN_POINT('Ctrl Pts',(3.23269332296938,-1.,-2.19568204933172));
#55967=CARTESIAN_POINT('Ctrl Pts',(3.23269332296938,1.,-2.19568204933172));
#55968=CARTESIAN_POINT('Ctrl Pts',(3.22562734221636,-1.,-2.19333345123531));
#55969=CARTESIAN_POINT('Ctrl Pts',(3.22562734221636,1.,-2.19333345123531));
#55970=CARTESIAN_POINT('Ctrl Pts',(3.21859043114069,-1.,-2.1909390194865));
#55971=CARTESIAN_POINT('Ctrl Pts',(3.21859043114069,1.,-2.1909390194865));
#55972=CARTESIAN_POINT('Ctrl Pts',(3.21156188355736,-1.,-2.18848253363878));
#55973=CARTESIAN_POINT('Ctrl Pts',(3.21156188355736,1.,-2.18848253363878));
#55974=CARTESIAN_POINT('Ctrl Pts',(3.20452259717947,-1.,-2.18594876115914));
#55975=CARTESIAN_POINT('Ctrl Pts',(3.20452259717947,1.,-2.18594876115914));
#55976=CARTESIAN_POINT('Ctrl Pts',(3.197462937404,-1.,-2.18332898656595));
#55977=CARTESIAN_POINT('Ctrl Pts',(3.197462937404,1.,-2.18332898656595));
#55978=CARTESIAN_POINT('Ctrl Pts',(3.19038924261589,-1.,-2.18062558031789));
#55979=CARTESIAN_POINT('Ctrl Pts',(3.19038924261589,1.,-2.18062558031789));
#55980=CARTESIAN_POINT('Ctrl Pts',(3.18333474627851,-1.,-2.17785968847172));
#55981=CARTESIAN_POINT('Ctrl Pts',(3.18333474627851,1.,-2.17785968847172));
#55982=CARTESIAN_POINT('Ctrl Pts',(3.17635032802584,-1.,-2.17506466903736));
#55983=CARTESIAN_POINT('Ctrl Pts',(3.17635032802584,1.,-2.17506466903736));
#55984=CARTESIAN_POINT('Ctrl Pts',(3.16948480019555,-1.,-2.17227212063857));
#55985=CARTESIAN_POINT('Ctrl Pts',(3.16948480019555,1.,-2.17227212063857));
#55986=CARTESIAN_POINT('Ctrl Pts',(3.16276685102999,-1.,-2.16949910801237));
#55987=CARTESIAN_POINT('Ctrl Pts',(3.16276685102999,1.,-2.16949910801237));
#55988=CARTESIAN_POINT('Ctrl Pts',(3.15618975593627,-1.,-2.1667372844767));
#55989=CARTESIAN_POINT('Ctrl Pts',(3.15618975593627,1.,-2.1667372844767));
#55990=CARTESIAN_POINT('Ctrl Pts',(3.14968624388961,-1.,-2.16393520288009));
#55991=CARTESIAN_POINT('Ctrl Pts',(3.14968624388961,1.,-2.16393520288009));
#55992=CARTESIAN_POINT('Ctrl Pts',(3.14314440426882,-1.,-2.16100905914341));
#55993=CARTESIAN_POINT('Ctrl Pts',(3.14314440426882,1.,-2.16100905914341));
#55994=CARTESIAN_POINT('Ctrl Pts',(3.136453565629,-1.,-2.15787423530583));
#55995=CARTESIAN_POINT('Ctrl Pts',(3.136453565629,1.,-2.15787423530583));
#55996=CARTESIAN_POINT('Ctrl Pts',(3.12954386795575,-1.,-2.15447241382872));
#55997=CARTESIAN_POINT('Ctrl Pts',(3.12954386795575,1.,-2.15447241382872));
#55998=CARTESIAN_POINT('Ctrl Pts',(3.12242318152001,-1.,-2.15079698090627));
#55999=CARTESIAN_POINT('Ctrl Pts',(3.12242318152001,1.,-2.15079698090627));
#56000=CARTESIAN_POINT('Ctrl Pts',(3.11522827017075,-1.,-2.1469279845768));
#56001=CARTESIAN_POINT('Ctrl Pts',(3.11522827017075,1.,-2.1469279845768));
#56002=CARTESIAN_POINT('Ctrl Pts',(3.10821808669189,-1.,-2.14302815602195));
#56003=CARTESIAN_POINT('Ctrl Pts',(3.10821808669189,1.,-2.14302815602195));
#56004=CARTESIAN_POINT('Ctrl Pts',(3.1017126739137,-1.,-2.13930228863968));
#56005=CARTESIAN_POINT('Ctrl Pts',(3.1017126739137,1.,-2.13930228863968));
#56006=CARTESIAN_POINT('Ctrl Pts',(3.09604502421197,-1.,-2.13596538661154));
#56007=CARTESIAN_POINT('Ctrl Pts',(3.09604502421197,1.,-2.13596538661154));
#56008=CARTESIAN_POINT('Ctrl Pts',(3.09151235281832,-1.,-2.13321032560805));
#56009=CARTESIAN_POINT('Ctrl Pts',(3.09151235281832,1.,-2.13321032560805));
#56010=CARTESIAN_POINT('Ctrl Pts',(3.08831615619661,-1.,-2.13116819908264));
#56011=CARTESIAN_POINT('Ctrl Pts',(3.08831615619661,1.,-2.13116819908264));
#56012=CARTESIAN_POINT('Ctrl Pts',(3.08690399991003,-1.,-2.1301541297915));
#56013=CARTESIAN_POINT('Ctrl Pts',(3.08690399991003,1.,-2.1301541297915));
#56014=CARTESIAN_POINT('Ctrl Pts',(3.08650326866821,-1.,-2.12975158752197));
#56015=CARTESIAN_POINT('Ctrl Pts',(3.08650326866821,1.,-2.12975158752197));
#56016=CARTESIAN_POINT('Ctrl Pts',(3.08652852644876,-1.,-2.12964222015945));
#56017=CARTESIAN_POINT('Ctrl Pts',(3.08652852644876,1.,-2.12964222015945));
#56018=CARTESIAN_POINT('Ctrl Pts',(3.08661426358891,-1.,-2.12962728847314));
#56019=CARTESIAN_POINT('Ctrl Pts',(3.08661426358891,1.,-2.12962728847314));
#56020=CARTESIAN_POINT('',(3.54075895182139,1.,-2.25898783642071));
#56021=CARTESIAN_POINT('Ctrl Pts',(3.54075895182139,1.,-2.25898783642071));
#56022=CARTESIAN_POINT('Ctrl Pts',(3.5391950664771,1.,-2.25882251694918));
#56023=CARTESIAN_POINT('Ctrl Pts',(3.53606853163247,1.,-2.25848864344599));
#56024=CARTESIAN_POINT('Ctrl Pts',(3.53138243689932,1.,-2.25797812951166));
#56025=CARTESIAN_POINT('Ctrl Pts',(3.52514172849666,1.,-2.25727802942142));
#56026=CARTESIAN_POINT('Ctrl Pts',(3.51735323669213,1.,-2.25637049456061));
#56027=CARTESIAN_POINT('Ctrl Pts',(3.50957720118209,1.,-2.25543046980351));
#56028=CARTESIAN_POINT('Ctrl Pts',(3.50181372618058,1.,-2.25445785151923));
#56029=CARTESIAN_POINT('Ctrl Pts',(3.49406296494309,1.,-2.25345251709453));
#56030=CARTESIAN_POINT('Ctrl Pts',(3.48632513240231,1.,-2.25241433138231));
#56031=CARTESIAN_POINT('Ctrl Pts',(3.47860048448015,1.,-2.25134314238258));
#56032=CARTESIAN_POINT('Ctrl Pts',(3.47088928979467,1.,-2.25023877475674));
#56033=CARTESIAN_POINT('Ctrl Pts',(3.46319180177474,1.,-2.24910102345977));
#56034=CARTESIAN_POINT('Ctrl Pts',(3.45550823512213,1.,-2.24792964960874));
#56035=CARTESIAN_POINT('Ctrl Pts',(3.44783872863448,1.,-2.24672437070139));
#56036=CARTESIAN_POINT('Ctrl Pts',(3.44018336460619,1.,-2.24548487526212));
#56037=CARTESIAN_POINT('Ctrl Pts',(3.43254222615007,1.,-2.24421085338856));
#56038=CARTESIAN_POINT('Ctrl Pts',(3.42491544683075,1.,-2.24290202531144));
#56039=CARTESIAN_POINT('Ctrl Pts',(3.41730325539119,1.,-2.24155816587811));
#56040=CARTESIAN_POINT('Ctrl Pts',(3.40970604190205,1.,-2.24017914395211));
#56041=CARTESIAN_POINT('Ctrl Pts',(3.40212434705511,1.,-2.23876491124064));
#56042=CARTESIAN_POINT('Ctrl Pts',(3.39455873448088,1.,-2.23731541452727));
#56043=CARTESIAN_POINT('Ctrl Pts',(3.38700968549522,1.,-2.23583052276281));
#56044=CARTESIAN_POINT('Ctrl Pts',(3.37947749555649,1.,-2.23430995599572));
#56045=CARTESIAN_POINT('Ctrl Pts',(3.37196214349356,1.,-2.23275319569253));
#56046=CARTESIAN_POINT('Ctrl Pts',(3.36446325227908,1.,-2.23115945849777));
#56047=CARTESIAN_POINT('Ctrl Pts',(3.35698038165529,1.,-2.22952789881011));
#56048=CARTESIAN_POINT('Ctrl Pts',(3.34951327111117,1.,-2.22785777756588));
#56049=CARTESIAN_POINT('Ctrl Pts',(3.34206209449371,1.,-2.22614863918044));
#56050=CARTESIAN_POINT('Ctrl Pts',(3.3346277284958,1.,-2.224400498785));
#56051=CARTESIAN_POINT('Ctrl Pts',(3.32721196326019,1.,-2.22261398879623));
#56052=CARTESIAN_POINT('Ctrl Pts',(3.31981686778008,1.,-2.22078990842768));
#56053=CARTESIAN_POINT('Ctrl Pts',(3.31244421655662,1.,-2.21892881679083));
#56054=CARTESIAN_POINT('Ctrl Pts',(3.3050948781957,1.,-2.21703059947837));
#56055=CARTESIAN_POINT('Ctrl Pts',(3.29776825193162,1.,-2.2150940692337));
#56056=CARTESIAN_POINT('Ctrl Pts',(3.29046159238344,1.,-2.21311648827391));
#56057=CARTESIAN_POINT('Ctrl Pts',(3.28317133333127,1.,-2.21109449750638));
#56058=CARTESIAN_POINT('Ctrl Pts',(3.27589448005534,1.,-2.20902509417425));
#56059=CARTESIAN_POINT('Ctrl Pts',(3.2686300613678,1.,-2.20690665217741));
#56060=CARTESIAN_POINT('Ctrl Pts',(3.26138036637711,1.,-2.20473979048682));
#56061=CARTESIAN_POINT('Ctrl Pts',(3.25415277957789,1.,-2.20252866491554));
#56062=CARTESIAN_POINT('Ctrl Pts',(3.24695715874356,1.,-2.20027910880993));
#56063=CARTESIAN_POINT('Ctrl Pts',(3.23980245361323,1.,-2.19799623693263));
#56064=CARTESIAN_POINT('Ctrl Pts',(3.23269332296938,1.,-2.19568204933172));
#56065=CARTESIAN_POINT('Ctrl Pts',(3.22562734221636,1.,-2.19333345123531));
#56066=CARTESIAN_POINT('Ctrl Pts',(3.21859043114069,1.,-2.1909390194865));
#56067=CARTESIAN_POINT('Ctrl Pts',(3.21156188355736,1.,-2.18848253363878));
#56068=CARTESIAN_POINT('Ctrl Pts',(3.20452259717947,1.,-2.18594876115914));
#56069=CARTESIAN_POINT('Ctrl Pts',(3.197462937404,1.,-2.18332898656595));
#56070=CARTESIAN_POINT('Ctrl Pts',(3.19038924261589,1.,-2.18062558031789));
#56071=CARTESIAN_POINT('Ctrl Pts',(3.18333474627851,1.,-2.17785968847172));
#56072=CARTESIAN_POINT('Ctrl Pts',(3.17635032802584,1.,-2.17506466903736));
#56073=CARTESIAN_POINT('Ctrl Pts',(3.16948480019555,1.,-2.17227212063857));
#56074=CARTESIAN_POINT('Ctrl Pts',(3.16276685102999,1.,-2.16949910801237));
#56075=CARTESIAN_POINT('Ctrl Pts',(3.15618975593627,1.,-2.1667372844767));
#56076=CARTESIAN_POINT('Ctrl Pts',(3.14968624388961,1.,-2.16393520288009));
#56077=CARTESIAN_POINT('Ctrl Pts',(3.14314440426882,1.,-2.16100905914341));
#56078=CARTESIAN_POINT('Ctrl Pts',(3.136453565629,1.,-2.15787423530583));
#56079=CARTESIAN_POINT('Ctrl Pts',(3.12954386795575,1.,-2.15447241382872));
#56080=CARTESIAN_POINT('Ctrl Pts',(3.12242318152001,1.,-2.15079698090627));
#56081=CARTESIAN_POINT('Ctrl Pts',(3.11522827017075,1.,-2.1469279845768));
#56082=CARTESIAN_POINT('Ctrl Pts',(3.10821808669189,1.,-2.14302815602195));
#56083=CARTESIAN_POINT('Ctrl Pts',(3.1017126739137,1.,-2.13930228863968));
#56084=CARTESIAN_POINT('Ctrl Pts',(3.09604502421197,1.,-2.13596538661154));
#56085=CARTESIAN_POINT('Ctrl Pts',(3.09151235281832,1.,-2.13321032560805));
#56086=CARTESIAN_POINT('Ctrl Pts',(3.08855597949844,1.,-2.13132142793056));
#56087=CARTESIAN_POINT('Ctrl Pts',(3.08717896996213,1.,-2.13034980480519));
#56088=CARTESIAN_POINT('Ctrl Pts',(3.08668447250383,1.,-2.12991938762497));
#56089=CARTESIAN_POINT('Ctrl Pts',(3.0865713108946,1.,-2.1297578506162));
#56090=CARTESIAN_POINT('Ctrl Pts',(3.08655633322109,1.,-2.12971124846838));
#56091=CARTESIAN_POINT('',(3.54075895182139,0.,-2.25898783642071));
#56092=CARTESIAN_POINT('Ctrl Pts',(3.2988053601491,-1.,-1.7833628895577));
#56093=CARTESIAN_POINT('Ctrl Pts',(3.2988053601491,1.,-1.7833628895577));
#56094=CARTESIAN_POINT('Ctrl Pts',(3.29877974053316,-1.,-1.78327971836342));
#56095=CARTESIAN_POINT('Ctrl Pts',(3.29877974053316,1.,-1.78327971836342));
#56096=CARTESIAN_POINT('Ctrl Pts',(3.29886572077632,-1.,-1.78320756177373));
#56097=CARTESIAN_POINT('Ctrl Pts',(3.29886572077632,1.,-1.78320756177373));
#56098=CARTESIAN_POINT('Ctrl Pts',(3.29940631674303,-1.,-1.7833818655594));
#56099=CARTESIAN_POINT('Ctrl Pts',(3.29940631674303,1.,-1.7833818655594));
#56100=CARTESIAN_POINT('Ctrl Pts',(3.30095096463517,-1.,-1.78417972819938));
#56101=CARTESIAN_POINT('Ctrl Pts',(3.30095096463517,1.,-1.78417972819938));
#56102=CARTESIAN_POINT('Ctrl Pts',(3.30422155559112,-1.,-1.78610045419846));
#56103=CARTESIAN_POINT('Ctrl Pts',(3.30422155559112,1.,-1.78610045419846));
#56104=CARTESIAN_POINT('Ctrl Pts',(3.30873412266788,-1.,-1.78888832245873));
#56105=CARTESIAN_POINT('Ctrl Pts',(3.30873412266788,1.,-1.78888832245873));
#56106=CARTESIAN_POINT('Ctrl Pts',(3.31428038326424,-1.,-1.79242331349949));
#56107=CARTESIAN_POINT('Ctrl Pts',(3.31428038326424,1.,-1.79242331349949));
#56108=CARTESIAN_POINT('Ctrl Pts',(3.3205535510082,-1.,-1.79652817033251));
#56109=CARTESIAN_POINT('Ctrl Pts',(3.3205535510082,1.,-1.79652817033251));
#56110=CARTESIAN_POINT('Ctrl Pts',(3.32721088039578,-1.,-1.80100380443406));
#56111=CARTESIAN_POINT('Ctrl Pts',(3.32721088039578,1.,-1.80100380443406));
#56112=CARTESIAN_POINT('Ctrl Pts',(3.33392460276808,-1.,-1.80565802981102));
#56113=CARTESIAN_POINT('Ctrl Pts',(3.33392460276808,1.,-1.80565802981102));
#56114=CARTESIAN_POINT('Ctrl Pts',(3.34043216147606,-1.,-1.81033399625352));
#56115=CARTESIAN_POINT('Ctrl Pts',(3.34043216147606,1.,-1.81033399625352));
#56116=CARTESIAN_POINT('Ctrl Pts',(3.34660014370673,-1.,-1.81494618732853));
#56117=CARTESIAN_POINT('Ctrl Pts',(3.34660014370673,1.,-1.81494618732853));
#56118=CARTESIAN_POINT('Ctrl Pts',(3.35243086937598,-1.,-1.81948458796829));
#56119=CARTESIAN_POINT('Ctrl Pts',(3.35243086937598,1.,-1.81948458796829));
#56120=CARTESIAN_POINT('Ctrl Pts',(3.35800801557424,-1.,-1.82398496829301));
#56121=CARTESIAN_POINT('Ctrl Pts',(3.35800801557424,1.,-1.82398496829301));
#56122=CARTESIAN_POINT('Ctrl Pts',(3.36345722124158,-1.,-1.82850752153199));
#56123=CARTESIAN_POINT('Ctrl Pts',(3.36345722124158,1.,-1.82850752153199));
#56124=CARTESIAN_POINT('Ctrl Pts',(3.36890396271836,-1.,-1.83311391452322));
#56125=CARTESIAN_POINT('Ctrl Pts',(3.36890396271836,1.,-1.83311391452322));
#56126=CARTESIAN_POINT('Ctrl Pts',(3.37442462015853,-1.,-1.83784072967077));
#56127=CARTESIAN_POINT('Ctrl Pts',(3.37442462015853,1.,-1.83784072967077));
#56128=CARTESIAN_POINT('Ctrl Pts',(3.38002968341157,-1.,-1.84269016931643));
#56129=CARTESIAN_POINT('Ctrl Pts',(3.38002968341157,1.,-1.84269016931643));
#56130=CARTESIAN_POINT('Ctrl Pts',(3.38569092349592,-1.,-1.84764441927753));
#56131=CARTESIAN_POINT('Ctrl Pts',(3.38569092349592,1.,-1.84764441927753));
#56132=CARTESIAN_POINT('Ctrl Pts',(3.39135802549398,-1.,-1.85267433291769));
#56133=CARTESIAN_POINT('Ctrl Pts',(3.39135802549398,1.,-1.85267433291769));
#56134=CARTESIAN_POINT('Ctrl Pts',(3.39697816833067,-1.,-1.85774972037062));
#56135=CARTESIAN_POINT('Ctrl Pts',(3.39697816833067,1.,-1.85774972037062));
#56136=CARTESIAN_POINT('Ctrl Pts',(3.40251742305476,-1.,-1.86285057051245));
#56137=CARTESIAN_POINT('Ctrl Pts',(3.40251742305476,1.,-1.86285057051245));
#56138=CARTESIAN_POINT('Ctrl Pts',(3.40797080000549,-1.,-1.86797231196654));
#56139=CARTESIAN_POINT('Ctrl Pts',(3.40797080000549,1.,-1.86797231196654));
#56140=CARTESIAN_POINT('Ctrl Pts',(3.41335043875209,-1.,-1.87311957248121));
#56141=CARTESIAN_POINT('Ctrl Pts',(3.41335043875209,1.,-1.87311957248121));
#56142=CARTESIAN_POINT('Ctrl Pts',(3.41867858383771,-1.,-1.87830245689344));
#56143=CARTESIAN_POINT('Ctrl Pts',(3.41867858383771,1.,-1.87830245689344));
#56144=CARTESIAN_POINT('Ctrl Pts',(3.42397908819736,-1.,-1.8835320506206));
#56145=CARTESIAN_POINT('Ctrl Pts',(3.42397908819736,1.,-1.8835320506206));
#56146=CARTESIAN_POINT('Ctrl Pts',(3.42926852222158,-1.,-1.88881571322009));
#56147=CARTESIAN_POINT('Ctrl Pts',(3.42926852222158,1.,-1.88881571322009));
#56148=CARTESIAN_POINT('Ctrl Pts',(3.43455074411571,-1.,-1.89415420002542));
#56149=CARTESIAN_POINT('Ctrl Pts',(3.43455074411571,1.,-1.89415420002542));
#56150=CARTESIAN_POINT('Ctrl Pts',(3.4398218567809,-1.,-1.89954426803384));
#56151=CARTESIAN_POINT('Ctrl Pts',(3.4398218567809,1.,-1.89954426803384));
#56152=CARTESIAN_POINT('Ctrl Pts',(3.44507323983367,-1.,-1.90498026502305));
#56153=CARTESIAN_POINT('Ctrl Pts',(3.44507323983367,1.,-1.90498026502305));
#56154=CARTESIAN_POINT('Ctrl Pts',(3.45029522038888,-1.,-1.91045605593639));
#56155=CARTESIAN_POINT('Ctrl Pts',(3.45029522038888,1.,-1.91045605593639));
#56156=CARTESIAN_POINT('Ctrl Pts',(3.4554807430995,-1.,-1.91596694784064));
#56157=CARTESIAN_POINT('Ctrl Pts',(3.4554807430995,1.,-1.91596694784064));
#56158=CARTESIAN_POINT('Ctrl Pts',(3.46062821722485,-1.,-1.92151118213212));
#56159=CARTESIAN_POINT('Ctrl Pts',(3.46062821722485,1.,-1.92151118213212));
#56160=CARTESIAN_POINT('Ctrl Pts',(3.46573953254084,-1.,-1.92708888591158));
#56161=CARTESIAN_POINT('Ctrl Pts',(3.46573953254084,1.,-1.92708888591158));
#56162=CARTESIAN_POINT('Ctrl Pts',(3.47081872409781,-1.,-1.93270136427081));
#56163=CARTESIAN_POINT('Ctrl Pts',(3.47081872409781,1.,-1.93270136427081));
#56164=CARTESIAN_POINT('Ctrl Pts',(3.47587040389915,-1.,-1.93835026973887));
#56165=CARTESIAN_POINT('Ctrl Pts',(3.47587040389915,1.,-1.93835026973887));
#56166=CARTESIAN_POINT('Ctrl Pts',(3.48089825770416,-1.,-1.94403680554065));
#56167=CARTESIAN_POINT('Ctrl Pts',(3.48089825770416,1.,-1.94403680554065));
#56168=CARTESIAN_POINT('Ctrl Pts',(3.48590361610814,-1.,-1.94976096795911));
#56169=CARTESIAN_POINT('Ctrl Pts',(3.48590361610814,1.,-1.94976096795911));
#56170=CARTESIAN_POINT('Ctrl Pts',(3.49088618670987,-1.,-1.95552193112084));
#56171=CARTESIAN_POINT('Ctrl Pts',(3.49088618670987,1.,-1.95552193112084));
#56172=CARTESIAN_POINT('Ctrl Pts',(3.49584466573064,-1.,-1.961318367765));
#56173=CARTESIAN_POINT('Ctrl Pts',(3.49584466573064,1.,-1.961318367765));
#56174=CARTESIAN_POINT('Ctrl Pts',(3.50077740176267,-1.,-1.96714879724052));
#56175=CARTESIAN_POINT('Ctrl Pts',(3.50077740176267,1.,-1.96714879724052));
#56176=CARTESIAN_POINT('Ctrl Pts',(3.5056830186108,-1.,-1.97301191162968));
#56177=CARTESIAN_POINT('Ctrl Pts',(3.5056830186108,1.,-1.97301191162968));
#56178=CARTESIAN_POINT('Ctrl Pts',(3.51056110478287,-1.,-1.97890693666288));
#56179=CARTESIAN_POINT('Ctrl Pts',(3.51056110478287,1.,-1.97890693666288));
#56180=CARTESIAN_POINT('Ctrl Pts',(3.51541198728301,-1.,-1.9848335106103));
#56181=CARTESIAN_POINT('Ctrl Pts',(3.51541198728301,1.,-1.9848335106103));
#56182=CARTESIAN_POINT('Ctrl Pts',(3.52023644289142,-1.,-1.99079153006112));
#56183=CARTESIAN_POINT('Ctrl Pts',(3.52023644289142,1.,-1.99079153006112));
#56184=CARTESIAN_POINT('Ctrl Pts',(3.52503542491728,-1.,-1.99678100339296));
#56185=CARTESIAN_POINT('Ctrl Pts',(3.52503542491728,1.,-1.99678100339296));
#56186=CARTESIAN_POINT('Ctrl Pts',(3.52980980250224,-1.,-2.00280191090366));
#56187=CARTESIAN_POINT('Ctrl Pts',(3.52980980250224,1.,-2.00280191090366));
#56188=CARTESIAN_POINT('Ctrl Pts',(3.53456004727424,-1.,-2.00885403604746));
#56189=CARTESIAN_POINT('Ctrl Pts',(3.53456004727424,1.,-2.00885403604746));
#56190=CARTESIAN_POINT('Ctrl Pts',(3.53928627453642,-1.,-2.01493698847351));
#56191=CARTESIAN_POINT('Ctrl Pts',(3.53928627453642,1.,-2.01493698847351));
#56192=CARTESIAN_POINT('Ctrl Pts',(3.54398838254136,-1.,-2.02105027983104));
#56193=CARTESIAN_POINT('Ctrl Pts',(3.54398838254136,1.,-2.02105027983104));
#56194=CARTESIAN_POINT('Ctrl Pts',(3.54866616282227,-1.,-2.02719338376175));
#56195=CARTESIAN_POINT('Ctrl Pts',(3.54866616282227,1.,-2.02719338376175));
#56196=CARTESIAN_POINT('Ctrl Pts',(3.55331941293949,-1.,-2.03336579658133));
#56197=CARTESIAN_POINT('Ctrl Pts',(3.55331941293949,1.,-2.03336579658133));
#56198=CARTESIAN_POINT('Ctrl Pts',(3.55794807264844,-1.,-2.03956711119976));
#56199=CARTESIAN_POINT('Ctrl Pts',(3.55794807264844,1.,-2.03956711119976));
#56200=CARTESIAN_POINT('Ctrl Pts',(3.56255223871505,-1.,-2.04579702158876));
#56201=CARTESIAN_POINT('Ctrl Pts',(3.56255223871505,1.,-2.04579702158876));
#56202=CARTESIAN_POINT('Ctrl Pts',(3.56713209977904,-1.,-2.05205528172911));
#56203=CARTESIAN_POINT('Ctrl Pts',(3.56713209977904,1.,-2.05205528172911));
#56204=CARTESIAN_POINT('Ctrl Pts',(3.5716878942334,-1.,-2.05834167687425));
#56205=CARTESIAN_POINT('Ctrl Pts',(3.5716878942334,1.,-2.05834167687425));
#56206=CARTESIAN_POINT('Ctrl Pts',(3.57621986224402,-1.,-2.06465599229234));
#56207=CARTESIAN_POINT('Ctrl Pts',(3.57621986224402,1.,-2.06465599229234));
#56208=CARTESIAN_POINT('Ctrl Pts',(3.58072819250872,-1.,-2.07099797606));
#56209=CARTESIAN_POINT('Ctrl Pts',(3.58072819250872,1.,-2.07099797606));
#56210=CARTESIAN_POINT('Ctrl Pts',(3.58521300039988,-1.,-2.07736732842524));
#56211=CARTESIAN_POINT('Ctrl Pts',(3.58521300039988,1.,-2.07736732842524));
#56212=CARTESIAN_POINT('Ctrl Pts',(3.58967435355834,-1.,-2.08376373049196));
#56213=CARTESIAN_POINT('Ctrl Pts',(3.58967435355834,1.,-2.08376373049196));
#56214=CARTESIAN_POINT('Ctrl Pts',(3.5941122862608,-1.,-2.09018686331706));
#56215=CARTESIAN_POINT('Ctrl Pts',(3.5941122862608,1.,-2.09018686331706));
#56216=CARTESIAN_POINT('Ctrl Pts',(3.59852681775396,-1.,-2.09663642986579));
#56217=CARTESIAN_POINT('Ctrl Pts',(3.59852681775396,1.,-2.09663642986579));
#56218=CARTESIAN_POINT('Ctrl Pts',(3.60291797087849,-1.,-2.10311217727687));
#56219=CARTESIAN_POINT('Ctrl Pts',(3.60291797087849,1.,-2.10311217727687));
#56220=CARTESIAN_POINT('Ctrl Pts',(3.60728578530968,-1.,-2.10961391333497));
#56221=CARTESIAN_POINT('Ctrl Pts',(3.60728578530968,1.,-2.10961391333497));
#56222=CARTESIAN_POINT('Ctrl Pts',(3.61163030607452,-1.,-2.11614149813928));
#56223=CARTESIAN_POINT('Ctrl Pts',(3.61163030607452,1.,-2.11614149813928));
#56224=CARTESIAN_POINT('Ctrl Pts',(3.61508732215187,-1.,-2.12138417125349));
#56225=CARTESIAN_POINT('Ctrl Pts',(3.61508732215187,1.,-2.12138417125349));
#56226=CARTESIAN_POINT('Ctrl Pts',(3.61766963589442,-1.,-2.12532774376144));
#56227=CARTESIAN_POINT('Ctrl Pts',(3.61766963589442,1.,-2.12532774376144));
#56228=CARTESIAN_POINT('Ctrl Pts',(3.61938653648716,-1.,-2.12796193131142));
#56229=CARTESIAN_POINT('Ctrl Pts',(3.61938653648716,1.,-2.12796193131142));
#56230=CARTESIAN_POINT('Ctrl Pts',(3.62024382630768,-1.,-2.12928030988903));
#56231=CARTESIAN_POINT('Ctrl Pts',(3.62024382630768,1.,-2.12928030988903));
#56232=CARTESIAN_POINT('',(3.29885386921514,1.,-1.78327315618341));
#56233=CARTESIAN_POINT('Ctrl Pts',(3.29885386921513,-1.,-1.78327315618341));
#56234=CARTESIAN_POINT('Ctrl Pts',(3.29885386921513,-0.666666666666667,
-1.78327315618341));
#56235=CARTESIAN_POINT('Ctrl Pts',(3.29885386921513,-0.333333333333333,
-1.78327315618341));
#56236=CARTESIAN_POINT('Ctrl Pts',(3.29885386921513,0.333333333333333,-1.78327315618341));
#56237=CARTESIAN_POINT('Ctrl Pts',(3.29885386921513,0.666666666666667,-1.78327315618341));
#56238=CARTESIAN_POINT('Ctrl Pts',(3.29885386921513,1.,-1.78327315618341));
#56239=CARTESIAN_POINT('',(3.62024382630768,1.,-2.12928030988903));
#56240=CARTESIAN_POINT('',(3.62024382630768,0.,-2.12928030988903));
#56241=CARTESIAN_POINT('Ctrl Pts',(3.29885386921514,1.,-1.78327315618341));
#56242=CARTESIAN_POINT('Ctrl Pts',(3.29890219175423,1.,-1.78326534445518));
#56243=CARTESIAN_POINT('Ctrl Pts',(3.29909749657808,1.,-1.78329283591905));
#56244=CARTESIAN_POINT('Ctrl Pts',(3.299705498242,1.,-1.78353803106924));
#56245=CARTESIAN_POINT('Ctrl Pts',(3.30119637003394,1.,-1.78432384788174));
#56246=CARTESIAN_POINT('Ctrl Pts',(3.30422155559112,1.,-1.78610045419846));
#56247=CARTESIAN_POINT('Ctrl Pts',(3.30873412266788,1.,-1.78888832245873));
#56248=CARTESIAN_POINT('Ctrl Pts',(3.31428038326424,1.,-1.79242331349949));
#56249=CARTESIAN_POINT('Ctrl Pts',(3.3205535510082,1.,-1.79652817033251));
#56250=CARTESIAN_POINT('Ctrl Pts',(3.32721088039578,1.,-1.80100380443406));
#56251=CARTESIAN_POINT('Ctrl Pts',(3.33392460276808,1.,-1.80565802981102));
#56252=CARTESIAN_POINT('Ctrl Pts',(3.34043216147606,1.,-1.81033399625352));
#56253=CARTESIAN_POINT('Ctrl Pts',(3.34660014370673,1.,-1.81494618732853));
#56254=CARTESIAN_POINT('Ctrl Pts',(3.35243086937598,1.,-1.81948458796829));
#56255=CARTESIAN_POINT('Ctrl Pts',(3.35800801557424,1.,-1.82398496829301));
#56256=CARTESIAN_POINT('Ctrl Pts',(3.36345722124158,1.,-1.82850752153199));
#56257=CARTESIAN_POINT('Ctrl Pts',(3.36890396271836,1.,-1.83311391452322));
#56258=CARTESIAN_POINT('Ctrl Pts',(3.37442462015853,1.,-1.83784072967077));
#56259=CARTESIAN_POINT('Ctrl Pts',(3.38002968341157,1.,-1.84269016931643));
#56260=CARTESIAN_POINT('Ctrl Pts',(3.38569092349592,1.,-1.84764441927753));
#56261=CARTESIAN_POINT('Ctrl Pts',(3.39135802549398,1.,-1.85267433291769));
#56262=CARTESIAN_POINT('Ctrl Pts',(3.39697816833067,1.,-1.85774972037062));
#56263=CARTESIAN_POINT('Ctrl Pts',(3.40251742305476,1.,-1.86285057051245));
#56264=CARTESIAN_POINT('Ctrl Pts',(3.40797080000549,1.,-1.86797231196654));
#56265=CARTESIAN_POINT('Ctrl Pts',(3.41335043875209,1.,-1.87311957248121));
#56266=CARTESIAN_POINT('Ctrl Pts',(3.41867858383771,1.,-1.87830245689344));
#56267=CARTESIAN_POINT('Ctrl Pts',(3.42397908819736,1.,-1.8835320506206));
#56268=CARTESIAN_POINT('Ctrl Pts',(3.42926852222158,1.,-1.88881571322009));
#56269=CARTESIAN_POINT('Ctrl Pts',(3.43455074411571,1.,-1.89415420002542));
#56270=CARTESIAN_POINT('Ctrl Pts',(3.4398218567809,1.,-1.89954426803384));
#56271=CARTESIAN_POINT('Ctrl Pts',(3.44507323983367,1.,-1.90498026502305));
#56272=CARTESIAN_POINT('Ctrl Pts',(3.45029522038888,1.,-1.91045605593639));
#56273=CARTESIAN_POINT('Ctrl Pts',(3.4554807430995,1.,-1.91596694784064));
#56274=CARTESIAN_POINT('Ctrl Pts',(3.46062821722485,1.,-1.92151118213212));
#56275=CARTESIAN_POINT('Ctrl Pts',(3.46573953254084,1.,-1.92708888591158));
#56276=CARTESIAN_POINT('Ctrl Pts',(3.47081872409781,1.,-1.93270136427081));
#56277=CARTESIAN_POINT('Ctrl Pts',(3.47587040389915,1.,-1.93835026973887));
#56278=CARTESIAN_POINT('Ctrl Pts',(3.48089825770416,1.,-1.94403680554065));
#56279=CARTESIAN_POINT('Ctrl Pts',(3.48590361610814,1.,-1.94976096795911));
#56280=CARTESIAN_POINT('Ctrl Pts',(3.49088618670987,1.,-1.95552193112084));
#56281=CARTESIAN_POINT('Ctrl Pts',(3.49584466573064,1.,-1.961318367765));
#56282=CARTESIAN_POINT('Ctrl Pts',(3.50077740176267,1.,-1.96714879724052));
#56283=CARTESIAN_POINT('Ctrl Pts',(3.5056830186108,1.,-1.97301191162968));
#56284=CARTESIAN_POINT('Ctrl Pts',(3.51056110478287,1.,-1.97890693666288));
#56285=CARTESIAN_POINT('Ctrl Pts',(3.51541198728301,1.,-1.9848335106103));
#56286=CARTESIAN_POINT('Ctrl Pts',(3.52023644289142,1.,-1.99079153006112));
#56287=CARTESIAN_POINT('Ctrl Pts',(3.52503542491728,1.,-1.99678100339296));
#56288=CARTESIAN_POINT('Ctrl Pts',(3.52980980250224,1.,-2.00280191090366));
#56289=CARTESIAN_POINT('Ctrl Pts',(3.53456004727424,1.,-2.00885403604746));
#56290=CARTESIAN_POINT('Ctrl Pts',(3.53928627453642,1.,-2.01493698847351));
#56291=CARTESIAN_POINT('Ctrl Pts',(3.54398838254136,1.,-2.02105027983104));
#56292=CARTESIAN_POINT('Ctrl Pts',(3.54866616282227,1.,-2.02719338376175));
#56293=CARTESIAN_POINT('Ctrl Pts',(3.55331941293949,1.,-2.03336579658133));
#56294=CARTESIAN_POINT('Ctrl Pts',(3.55794807264844,1.,-2.03956711119976));
#56295=CARTESIAN_POINT('Ctrl Pts',(3.56255223871505,1.,-2.04579702158876));
#56296=CARTESIAN_POINT('Ctrl Pts',(3.56713209977904,1.,-2.05205528172911));
#56297=CARTESIAN_POINT('Ctrl Pts',(3.5716878942334,1.,-2.05834167687425));
#56298=CARTESIAN_POINT('Ctrl Pts',(3.57621986224402,1.,-2.06465599229234));
#56299=CARTESIAN_POINT('Ctrl Pts',(3.58072819250872,1.,-2.07099797606));
#56300=CARTESIAN_POINT('Ctrl Pts',(3.58521300039988,1.,-2.07736732842524));
#56301=CARTESIAN_POINT('Ctrl Pts',(3.58967435355834,1.,-2.08376373049196));
#56302=CARTESIAN_POINT('Ctrl Pts',(3.5941122862608,1.,-2.09018686331706));
#56303=CARTESIAN_POINT('Ctrl Pts',(3.59852681775396,1.,-2.09663642986579));
#56304=CARTESIAN_POINT('Ctrl Pts',(3.60291797087849,1.,-2.10311217727687));
#56305=CARTESIAN_POINT('Ctrl Pts',(3.60728578530968,1.,-2.10961391333497));
#56306=CARTESIAN_POINT('Ctrl Pts',(3.61163030607452,1.,-2.11614149813928));
#56307=CARTESIAN_POINT('Ctrl Pts',(3.61508732215187,1.,-2.12138417125349));
#56308=CARTESIAN_POINT('Ctrl Pts',(3.61766963589442,1.,-2.12532774376144));
#56309=CARTESIAN_POINT('Ctrl Pts',(3.61938653648716,1.,-2.12796193131142));
#56310=CARTESIAN_POINT('Ctrl Pts',(3.62024382630768,1.,-2.12928030988903));
#56311=CARTESIAN_POINT('Origin',(3.62024382630768,0.,-2.12928030988903));
#56312=CARTESIAN_POINT('',(3.54075895182139,1.,-2.25898783642071));
#56313=CARTESIAN_POINT('Origin',(0.,0.,0.));
#56314=CARTESIAN_POINT('',(3.38171594275687,1.,-1.62064718014256));
#56315=CARTESIAN_POINT('Origin',(0.,1.,0.));
#56316=CARTESIAN_POINT('Ctrl Pts',(3.38171594275687,1.,-1.62064718014256));
#56317=CARTESIAN_POINT('Ctrl Pts',(3.38171594275687,0.666666666666667,-1.62064718014256));
#56318=CARTESIAN_POINT('Ctrl Pts',(3.38171594275687,0.333333333333333,-1.62064718014256));
#56319=CARTESIAN_POINT('Ctrl Pts',(3.38171594275687,-0.333333333333333,
-1.62064718014256));
#56320=CARTESIAN_POINT('Ctrl Pts',(3.38171594275687,-0.666666666666667,
-1.62064718014255));
#56321=CARTESIAN_POINT('Ctrl Pts',(3.38171594275687,-1.,-1.62064718014255));
#56322=CARTESIAN_POINT('Ctrl Pts',(3.85054988729471,-1.,-1.67727921511438));
#56323=CARTESIAN_POINT('Ctrl Pts',(3.85054988729471,1.,-1.67727921511438));
#56324=CARTESIAN_POINT('Ctrl Pts',(3.84897939431104,-1.,-1.6773605765671));
#56325=CARTESIAN_POINT('Ctrl Pts',(3.84897939431104,1.,-1.6773605765671));
#56326=CARTESIAN_POINT('Ctrl Pts',(3.84583912297567,-1.,-1.67751991140661));
#56327=CARTESIAN_POINT('Ctrl Pts',(3.84583912297567,1.,-1.67751991140661));
#56328=CARTESIAN_POINT('Ctrl Pts',(3.8411308598706,-1.,-1.67774874946867));
#56329=CARTESIAN_POINT('Ctrl Pts',(3.8411308598706,1.,-1.67774874946867));
#56330=CARTESIAN_POINT('Ctrl Pts',(3.83485746516115,-1.,-1.67803353065273));
#56331=CARTESIAN_POINT('Ctrl Pts',(3.83485746516115,1.,-1.67803353065273));
#56332=CARTESIAN_POINT('Ctrl Pts',(3.82702289288453,-1.,-1.67835555760094));
#56333=CARTESIAN_POINT('Ctrl Pts',(3.82702289288453,1.,-1.67835555760094));
#56334=CARTESIAN_POINT('Ctrl Pts',(3.81919554100522,-1.,-1.67864354606363));
#56335=CARTESIAN_POINT('Ctrl Pts',(3.81919554100522,1.,-1.67864354606363));
#56336=CARTESIAN_POINT('Ctrl Pts',(3.81137549624273,-1.,-1.67889737738311));
#56337=CARTESIAN_POINT('Ctrl Pts',(3.81137549624273,1.,-1.67889737738311));
#56338=CARTESIAN_POINT('Ctrl Pts',(3.80356289078481,-1.,-1.67911690648128));
#56339=CARTESIAN_POINT('Ctrl Pts',(3.80356289078481,1.,-1.67911690648128));
#56340=CARTESIAN_POINT('Ctrl Pts',(3.7957579157763,-1.,-1.67930196625204));
#56341=CARTESIAN_POINT('Ctrl Pts',(3.7957579157763,1.,-1.67930196625204));
#56342=CARTESIAN_POINT('Ctrl Pts',(3.78796080021026,-1.,-1.67945236653175));
#56343=CARTESIAN_POINT('Ctrl Pts',(3.78796080021026,1.,-1.67945236653175));
#56344=CARTESIAN_POINT('Ctrl Pts',(3.78017178196859,-1.,-1.67956789211943));
#56345=CARTESIAN_POINT('Ctrl Pts',(3.78017178196859,1.,-1.67956789211943));
#56346=CARTESIAN_POINT('Ctrl Pts',(3.77239107928394,-1.,-1.67964830084946));
#56347=CARTESIAN_POINT('Ctrl Pts',(3.77239107928394,1.,-1.67964830084946));
#56348=CARTESIAN_POINT('Ctrl Pts',(3.76461886684523,-1.,-1.67969332319322));
#56349=CARTESIAN_POINT('Ctrl Pts',(3.76461886684523,1.,-1.67969332319322));
#56350=CARTESIAN_POINT('Ctrl Pts',(3.75685523754816,-1.,-1.67970265841379));
#56351=CARTESIAN_POINT('Ctrl Pts',(3.75685523754816,1.,-1.67970265841379));
#56352=CARTESIAN_POINT('Ctrl Pts',(3.74910022394845,-1.,-1.67967598599665));
#56353=CARTESIAN_POINT('Ctrl Pts',(3.74910022394845,1.,-1.67967598599665));
#56354=CARTESIAN_POINT('Ctrl Pts',(3.74135385965622,-1.,-1.67961298685316));
#56355=CARTESIAN_POINT('Ctrl Pts',(3.74135385965622,1.,-1.67961298685316));
#56356=CARTESIAN_POINT('Ctrl Pts',(3.73361623282617,-1.,-1.67951336376434));
#56357=CARTESIAN_POINT('Ctrl Pts',(3.73361623282617,1.,-1.67951336376434));
#56358=CARTESIAN_POINT('Ctrl Pts',(3.72588753416339,-1.,-1.67937685856627));
#56359=CARTESIAN_POINT('Ctrl Pts',(3.72588753416339,1.,-1.67937685856627));
#56360=CARTESIAN_POINT('Ctrl Pts',(3.71816812842188,-1.,-1.6792032807165));
#56361=CARTESIAN_POINT('Ctrl Pts',(3.71816812842188,1.,-1.6792032807165));
#56362=CARTESIAN_POINT('Ctrl Pts',(3.71045854208195,-1.,-1.67899249793398));
#56363=CARTESIAN_POINT('Ctrl Pts',(3.71045854208195,1.,-1.67899249793398));
#56364=CARTESIAN_POINT('Ctrl Pts',(3.70275932350998,-1.,-1.6787443694862));
#56365=CARTESIAN_POINT('Ctrl Pts',(3.70275932350998,1.,-1.6787443694862));
#56366=CARTESIAN_POINT('Ctrl Pts',(3.69507092759545,-1.,-1.67845869064304));
#56367=CARTESIAN_POINT('Ctrl Pts',(3.69507092759545,1.,-1.67845869064304));
#56368=CARTESIAN_POINT('Ctrl Pts',(3.68739360236505,-1.,-1.67813513867973));
#56369=CARTESIAN_POINT('Ctrl Pts',(3.68739360236505,1.,-1.67813513867973));
#56370=CARTESIAN_POINT('Ctrl Pts',(3.6797272457918,-1.,-1.67777320475872));
#56371=CARTESIAN_POINT('Ctrl Pts',(3.6797272457918,1.,-1.67777320475872));
#56372=CARTESIAN_POINT('Ctrl Pts',(3.67207136294639,-1.,-1.67737217414901));
#56373=CARTESIAN_POINT('Ctrl Pts',(3.67207136294639,1.,-1.67737217414901));
#56374=CARTESIAN_POINT('Ctrl Pts',(3.66442538671018,-1.,-1.67693128053153));
#56375=CARTESIAN_POINT('Ctrl Pts',(3.66442538671018,1.,-1.67693128053153));
#56376=CARTESIAN_POINT('Ctrl Pts',(3.65678894416442,-1.,-1.67644983469459));
#56377=CARTESIAN_POINT('Ctrl Pts',(3.65678894416442,1.,-1.67644983469459));
#56378=CARTESIAN_POINT('Ctrl Pts',(3.64916213574663,-1.,-1.6759273594669));
#56379=CARTESIAN_POINT('Ctrl Pts',(3.64916213574663,1.,-1.6759273594669));
#56380=CARTESIAN_POINT('Ctrl Pts',(3.6415458297232,-1.,-1.6753637326484));
#56381=CARTESIAN_POINT('Ctrl Pts',(3.6415458297232,1.,-1.6753637326484));
#56382=CARTESIAN_POINT('Ctrl Pts',(3.63394189312902,-1.,-1.67475929882962));
#56383=CARTESIAN_POINT('Ctrl Pts',(3.63394189312902,1.,-1.67475929882962));
#56384=CARTESIAN_POINT('Ctrl Pts',(3.62635249450908,-1.,-1.67411452372265));
#56385=CARTESIAN_POINT('Ctrl Pts',(3.62635249450908,1.,-1.67411452372265));
#56386=CARTESIAN_POINT('Ctrl Pts',(3.61877947398179,-1.,-1.67342968196223));
#56387=CARTESIAN_POINT('Ctrl Pts',(3.61877947398179,1.,-1.67342968196223));
#56388=CARTESIAN_POINT('Ctrl Pts',(3.61122367156182,-1.,-1.67270452466968));
#56389=CARTESIAN_POINT('Ctrl Pts',(3.61122367156182,1.,-1.67270452466968));
#56390=CARTESIAN_POINT('Ctrl Pts',(3.60368430815203,-1.,-1.67193797318598));
#56391=CARTESIAN_POINT('Ctrl Pts',(3.60368430815203,1.,-1.67193797318598));
#56392=CARTESIAN_POINT('Ctrl Pts',(3.59615824388808,-1.,-1.67112775290706));
#56393=CARTESIAN_POINT('Ctrl Pts',(3.59615824388808,1.,-1.67112775290706));
#56394=CARTESIAN_POINT('Ctrl Pts',(3.5886414309783,-1.,-1.67027110397602));
#56395=CARTESIAN_POINT('Ctrl Pts',(3.5886414309783,1.,-1.67027110397602));
#56396=CARTESIAN_POINT('Ctrl Pts',(3.58113044183823,-1.,-1.66936552908228));
#56397=CARTESIAN_POINT('Ctrl Pts',(3.58113044183823,1.,-1.66936552908228));
#56398=CARTESIAN_POINT('Ctrl Pts',(3.57362406285884,-1.,-1.66840957407299));
#56399=CARTESIAN_POINT('Ctrl Pts',(3.57362406285884,1.,-1.66840957407299));
#56400=CARTESIAN_POINT('Ctrl Pts',(3.56612465179429,-1.,-1.66740349220308));
#56401=CARTESIAN_POINT('Ctrl Pts',(3.56612465179429,1.,-1.66740349220308));
#56402=CARTESIAN_POINT('Ctrl Pts',(3.55864015233617,-1.,-1.66635023293121));
#56403=CARTESIAN_POINT('Ctrl Pts',(3.55864015233617,1.,-1.66635023293121));
#56404=CARTESIAN_POINT('Ctrl Pts',(3.5511812134288,-1.,-1.66525401569004));
#56405=CARTESIAN_POINT('Ctrl Pts',(3.5511812134288,1.,-1.66525401569004));
#56406=CARTESIAN_POINT('Ctrl Pts',(3.5437574747503,-1.,-1.66411849222334));
#56407=CARTESIAN_POINT('Ctrl Pts',(3.5437574747503,1.,-1.66411849222334));
#56408=CARTESIAN_POINT('Ctrl Pts',(3.53637385060225,-1.,-1.66294490916113));
#56409=CARTESIAN_POINT('Ctrl Pts',(3.53637385060225,1.,-1.66294490916113));
#56410=CARTESIAN_POINT('Ctrl Pts',(3.52902746211081,-1.,-1.66173058912365));
#56411=CARTESIAN_POINT('Ctrl Pts',(3.52902746211081,1.,-1.66173058912365));
#56412=CARTESIAN_POINT('Ctrl Pts',(3.52170261543787,-1.,-1.66046645222266));
#56413=CARTESIAN_POINT('Ctrl Pts',(3.52170261543787,1.,-1.66046645222266));
#56414=CARTESIAN_POINT('Ctrl Pts',(3.51437632188903,-1.,-1.65913971687324));
#56415=CARTESIAN_POINT('Ctrl Pts',(3.51437632188903,1.,-1.65913971687324));
#56416=CARTESIAN_POINT('Ctrl Pts',(3.5070273314651,-1.,-1.65773832633617));
#56417=CARTESIAN_POINT('Ctrl Pts',(3.5070273314651,1.,-1.65773832633617));
#56418=CARTESIAN_POINT('Ctrl Pts',(3.49964476477929,-1.,-1.65625517961583));
#56419=CARTESIAN_POINT('Ctrl Pts',(3.49964476477929,1.,-1.65625517961583));
#56420=CARTESIAN_POINT('Ctrl Pts',(3.49223525300194,-1.,-1.65469162644476));
#56421=CARTESIAN_POINT('Ctrl Pts',(3.49223525300194,1.,-1.65469162644476));
#56422=CARTESIAN_POINT('Ctrl Pts',(3.48483492840942,-1.,-1.65306335367762));
#56423=CARTESIAN_POINT('Ctrl Pts',(3.48483492840942,1.,-1.65306335367762));
#56424=CARTESIAN_POINT('Ctrl Pts',(3.47749926256543,-1.,-1.65139534930353));
#56425=CARTESIAN_POINT('Ctrl Pts',(3.47749926256543,1.,-1.65139534930353));
#56426=CARTESIAN_POINT('Ctrl Pts',(3.47028140996055,-1.,-1.64971118698285));
#56427=CARTESIAN_POINT('Ctrl Pts',(3.47028140996055,1.,-1.64971118698285));
#56428=CARTESIAN_POINT('Ctrl Pts',(3.46321237515029,-1.,-1.64802323352752));
#56429=CARTESIAN_POINT('Ctrl Pts',(3.46321237515029,1.,-1.64802323352752));
#56430=CARTESIAN_POINT('Ctrl Pts',(3.4562842106239,-1.,-1.64632429697506));
#56431=CARTESIAN_POINT('Ctrl Pts',(3.4562842106239,1.,-1.64632429697506));
#56432=CARTESIAN_POINT('Ctrl Pts',(3.44942242546693,-1.,-1.64457408708059));
#56433=CARTESIAN_POINT('Ctrl Pts',(3.44942242546693,1.,-1.64457408708059));
#56434=CARTESIAN_POINT('Ctrl Pts',(3.44250337701736,-1.,-1.64270733821042));
#56435=CARTESIAN_POINT('Ctrl Pts',(3.44250337701736,1.,-1.64270733821042));
#56436=CARTESIAN_POINT('Ctrl Pts',(3.43540451921397,-1.,-1.64065778701952));
#56437=CARTESIAN_POINT('Ctrl Pts',(3.43540451921397,1.,-1.64065778701952));
#56438=CARTESIAN_POINT('Ctrl Pts',(3.42804772926213,-1.,-1.6383787624689));
#56439=CARTESIAN_POINT('Ctrl Pts',(3.42804772926213,1.,-1.6383787624689));
#56440=CARTESIAN_POINT('Ctrl Pts',(3.4204397459095,-1.,-1.63586250099804));
#56441=CARTESIAN_POINT('Ctrl Pts',(3.4204397459095,1.,-1.63586250099804));
#56442=CARTESIAN_POINT('Ctrl Pts',(3.41272817148719,-1.,-1.63316667054156));
#56443=CARTESIAN_POINT('Ctrl Pts',(3.41272817148719,1.,-1.63316667054156));
#56444=CARTESIAN_POINT('Ctrl Pts',(3.40519422740596,-1.,-1.63041148964996));
#56445=CARTESIAN_POINT('Ctrl Pts',(3.40519422740596,1.,-1.63041148964996));
#56446=CARTESIAN_POINT('Ctrl Pts',(3.39818605298342,-1.,-1.62774916464571));
#56447=CARTESIAN_POINT('Ctrl Pts',(3.39818605298342,1.,-1.62774916464571));
#56448=CARTESIAN_POINT('Ctrl Pts',(3.39206617497078,-1.,-1.62533996116793));
#56449=CARTESIAN_POINT('Ctrl Pts',(3.39206617497078,1.,-1.62533996116793));
#56450=CARTESIAN_POINT('Ctrl Pts',(3.38715832178929,-1.,-1.62332788556183));
#56451=CARTESIAN_POINT('Ctrl Pts',(3.38715832178929,1.,-1.62332788556183));
#56452=CARTESIAN_POINT('Ctrl Pts',(3.38368201668123,-1.,-1.62181089631134));
#56453=CARTESIAN_POINT('Ctrl Pts',(3.38368201668123,1.,-1.62181089631134));
#56454=CARTESIAN_POINT('Ctrl Pts',(3.38212861099481,-1.,-1.62103022180917));
#56455=CARTESIAN_POINT('Ctrl Pts',(3.38212861099481,1.,-1.62103022180917));
#56456=CARTESIAN_POINT('Ctrl Pts',(3.38166984193496,-1.,-1.6206953236804));
#56457=CARTESIAN_POINT('Ctrl Pts',(3.38166984193496,1.,-1.6206953236804));
#56458=CARTESIAN_POINT('Ctrl Pts',(3.38167767992546,-1.,-1.62058335162421));
#56459=CARTESIAN_POINT('Ctrl Pts',(3.38167767992546,1.,-1.62058335162421));
#56460=CARTESIAN_POINT('Ctrl Pts',(3.38176002566879,-1.,-1.62055519152809));
#56461=CARTESIAN_POINT('Ctrl Pts',(3.38176002566879,1.,-1.62055519152809));
#56462=CARTESIAN_POINT('',(3.85054988729471,1.,-1.67727921511438));
#56463=CARTESIAN_POINT('Ctrl Pts',(3.85054988729471,1.,-1.67727921511438));
#56464=CARTESIAN_POINT('Ctrl Pts',(3.84897939431104,1.,-1.6773605765671));
#56465=CARTESIAN_POINT('Ctrl Pts',(3.84583912297567,1.,-1.67751991140661));
#56466=CARTESIAN_POINT('Ctrl Pts',(3.8411308598706,1.,-1.67774874946867));
#56467=CARTESIAN_POINT('Ctrl Pts',(3.83485746516115,1.,-1.67803353065273));
#56468=CARTESIAN_POINT('Ctrl Pts',(3.82702289288453,1.,-1.67835555760094));
#56469=CARTESIAN_POINT('Ctrl Pts',(3.81919554100522,1.,-1.67864354606363));
#56470=CARTESIAN_POINT('Ctrl Pts',(3.81137549624273,1.,-1.67889737738311));
#56471=CARTESIAN_POINT('Ctrl Pts',(3.80356289078481,1.,-1.67911690648128));
#56472=CARTESIAN_POINT('Ctrl Pts',(3.7957579157763,1.,-1.67930196625204));
#56473=CARTESIAN_POINT('Ctrl Pts',(3.78796080021026,1.,-1.67945236653175));
#56474=CARTESIAN_POINT('Ctrl Pts',(3.78017178196859,1.,-1.67956789211943));
#56475=CARTESIAN_POINT('Ctrl Pts',(3.77239107928394,1.,-1.67964830084946));
#56476=CARTESIAN_POINT('Ctrl Pts',(3.76461886684523,1.,-1.67969332319322));
#56477=CARTESIAN_POINT('Ctrl Pts',(3.75685523754816,1.,-1.67970265841379));
#56478=CARTESIAN_POINT('Ctrl Pts',(3.74910022394845,1.,-1.67967598599665));
#56479=CARTESIAN_POINT('Ctrl Pts',(3.74135385965622,1.,-1.67961298685316));
#56480=CARTESIAN_POINT('Ctrl Pts',(3.73361623282617,1.,-1.67951336376434));
#56481=CARTESIAN_POINT('Ctrl Pts',(3.72588753416339,1.,-1.67937685856627));
#56482=CARTESIAN_POINT('Ctrl Pts',(3.71816812842188,1.,-1.6792032807165));
#56483=CARTESIAN_POINT('Ctrl Pts',(3.71045854208195,1.,-1.67899249793398));
#56484=CARTESIAN_POINT('Ctrl Pts',(3.70275932350998,1.,-1.6787443694862));
#56485=CARTESIAN_POINT('Ctrl Pts',(3.69507092759545,1.,-1.67845869064304));
#56486=CARTESIAN_POINT('Ctrl Pts',(3.68739360236505,1.,-1.67813513867973));
#56487=CARTESIAN_POINT('Ctrl Pts',(3.6797272457918,1.,-1.67777320475872));
#56488=CARTESIAN_POINT('Ctrl Pts',(3.67207136294639,1.,-1.67737217414901));
#56489=CARTESIAN_POINT('Ctrl Pts',(3.66442538671018,1.,-1.67693128053153));
#56490=CARTESIAN_POINT('Ctrl Pts',(3.65678894416442,1.,-1.67644983469459));
#56491=CARTESIAN_POINT('Ctrl Pts',(3.64916213574663,1.,-1.6759273594669));
#56492=CARTESIAN_POINT('Ctrl Pts',(3.6415458297232,1.,-1.6753637326484));
#56493=CARTESIAN_POINT('Ctrl Pts',(3.63394189312902,1.,-1.67475929882962));
#56494=CARTESIAN_POINT('Ctrl Pts',(3.62635249450908,1.,-1.67411452372265));
#56495=CARTESIAN_POINT('Ctrl Pts',(3.61877947398179,1.,-1.67342968196223));
#56496=CARTESIAN_POINT('Ctrl Pts',(3.61122367156182,1.,-1.67270452466968));
#56497=CARTESIAN_POINT('Ctrl Pts',(3.60368430815203,1.,-1.67193797318598));
#56498=CARTESIAN_POINT('Ctrl Pts',(3.59615824388808,1.,-1.67112775290706));
#56499=CARTESIAN_POINT('Ctrl Pts',(3.5886414309783,1.,-1.67027110397602));
#56500=CARTESIAN_POINT('Ctrl Pts',(3.58113044183823,1.,-1.66936552908228));
#56501=CARTESIAN_POINT('Ctrl Pts',(3.57362406285884,1.,-1.66840957407299));
#56502=CARTESIAN_POINT('Ctrl Pts',(3.56612465179429,1.,-1.66740349220308));
#56503=CARTESIAN_POINT('Ctrl Pts',(3.55864015233617,1.,-1.66635023293121));
#56504=CARTESIAN_POINT('Ctrl Pts',(3.5511812134288,1.,-1.66525401569004));
#56505=CARTESIAN_POINT('Ctrl Pts',(3.5437574747503,1.,-1.66411849222334));
#56506=CARTESIAN_POINT('Ctrl Pts',(3.53637385060225,1.,-1.66294490916113));
#56507=CARTESIAN_POINT('Ctrl Pts',(3.52902746211081,1.,-1.66173058912365));
#56508=CARTESIAN_POINT('Ctrl Pts',(3.52170261543787,1.,-1.66046645222266));
#56509=CARTESIAN_POINT('Ctrl Pts',(3.51437632188903,1.,-1.65913971687324));
#56510=CARTESIAN_POINT('Ctrl Pts',(3.5070273314651,1.,-1.65773832633617));
#56511=CARTESIAN_POINT('Ctrl Pts',(3.49964476477929,1.,-1.65625517961583));
#56512=CARTESIAN_POINT('Ctrl Pts',(3.49223525300194,1.,-1.65469162644476));
#56513=CARTESIAN_POINT('Ctrl Pts',(3.48483492840942,1.,-1.65306335367762));
#56514=CARTESIAN_POINT('Ctrl Pts',(3.47749926256543,1.,-1.65139534930353));
#56515=CARTESIAN_POINT('Ctrl Pts',(3.47028140996055,1.,-1.64971118698285));
#56516=CARTESIAN_POINT('Ctrl Pts',(3.46321237515029,1.,-1.64802323352752));
#56517=CARTESIAN_POINT('Ctrl Pts',(3.4562842106239,1.,-1.64632429697506));
#56518=CARTESIAN_POINT('Ctrl Pts',(3.44942242546693,1.,-1.64457408708059));
#56519=CARTESIAN_POINT('Ctrl Pts',(3.44250337701736,1.,-1.64270733821042));
#56520=CARTESIAN_POINT('Ctrl Pts',(3.43540451921397,1.,-1.64065778701952));
#56521=CARTESIAN_POINT('Ctrl Pts',(3.42804772926213,1.,-1.6383787624689));
#56522=CARTESIAN_POINT('Ctrl Pts',(3.4204397459095,1.,-1.63586250099804));
#56523=CARTESIAN_POINT('Ctrl Pts',(3.41272817148719,1.,-1.63316667054156));
#56524=CARTESIAN_POINT('Ctrl Pts',(3.40519422740596,1.,-1.63041148964996));
#56525=CARTESIAN_POINT('Ctrl Pts',(3.39818605298342,1.,-1.62774916464571));
#56526=CARTESIAN_POINT('Ctrl Pts',(3.39206617497078,1.,-1.62533996116793));
#56527=CARTESIAN_POINT('Ctrl Pts',(3.38715832178929,1.,-1.62332788556183));
#56528=CARTESIAN_POINT('Ctrl Pts',(3.3839428576331,1.,-1.62192472202795));
#56529=CARTESIAN_POINT('Ctrl Pts',(3.38243080602536,1.,-1.62118047294574));
#56530=CARTESIAN_POINT('Ctrl Pts',(3.38187506457001,1.,-1.62083271136059));
#56531=CARTESIAN_POINT('Ctrl Pts',(3.38173802621242,1.,-1.62069086551627));
#56532=CARTESIAN_POINT('Ctrl Pts',(3.38171594275687,1.,-1.62064718014256));
#56533=CARTESIAN_POINT('',(3.85054988729471,0.,-1.67727921511438));
#56534=CARTESIAN_POINT('Ctrl Pts',(3.53717101171257,-1.,-1.24535988127942));
#56535=CARTESIAN_POINT('Ctrl Pts',(3.53717101171257,1.,-1.24535988127942));
#56536=CARTESIAN_POINT('Ctrl Pts',(3.53713269667534,-1.,-1.24528174185147));
#56537=CARTESIAN_POINT('Ctrl Pts',(3.53713269667534,1.,-1.24528174185147));
#56538=CARTESIAN_POINT('Ctrl Pts',(3.53720633058152,-1.,-1.2451970233558));
#56539=CARTESIAN_POINT('Ctrl Pts',(3.53720633058152,1.,-1.2451970233558));
#56540=CARTESIAN_POINT('Ctrl Pts',(3.53776753803428,-1.,-1.24528461333177));
#56541=CARTESIAN_POINT('Ctrl Pts',(3.53776753803428,1.,-1.24528461333177));
#56542=CARTESIAN_POINT('Ctrl Pts',(3.53941798196293,-1.,-1.24583101679199));
#56543=CARTESIAN_POINT('Ctrl Pts',(3.53941798196293,1.,-1.24583101679199));
#56544=CARTESIAN_POINT('Ctrl Pts',(3.54294877426113,-1.,-1.2472164623202));
#56545=CARTESIAN_POINT('Ctrl Pts',(3.54294877426113,1.,-1.2472164623202));
#56546=CARTESIAN_POINT('Ctrl Pts',(3.54784190282889,-1.,-1.24926408627938));
#56547=CARTESIAN_POINT('Ctrl Pts',(3.54784190282889,1.,-1.24926408627938));
#56548=CARTESIAN_POINT('Ctrl Pts',(3.5538728741862,-1.,-1.25188792940508));
#56549=CARTESIAN_POINT('Ctrl Pts',(3.5538728741862,1.,-1.25188792940508));
#56550=CARTESIAN_POINT('Ctrl Pts',(3.56071094990825,-1.,-1.25496090899873));
#56551=CARTESIAN_POINT('Ctrl Pts',(3.56071094990825,1.,-1.25496090899873));
#56552=CARTESIAN_POINT('Ctrl Pts',(3.56798645995025,-1.,-1.25834000485626));
#56553=CARTESIAN_POINT('Ctrl Pts',(3.56798645995025,1.,-1.25834000485626));
#56554=CARTESIAN_POINT('Ctrl Pts',(3.5753456065164,-1.,-1.26188667142784));
#56555=CARTESIAN_POINT('Ctrl Pts',(3.5753456065164,1.,-1.26188667142784));
#56556=CARTESIAN_POINT('Ctrl Pts',(3.58250452868699,-1.,-1.26548706249891));
#56557=CARTESIAN_POINT('Ctrl Pts',(3.58250452868699,1.,-1.26548706249891));
#56558=CARTESIAN_POINT('Ctrl Pts',(3.5893180784647,-1.,-1.26907758484766));
#56559=CARTESIAN_POINT('Ctrl Pts',(3.5893180784647,1.,-1.26907758484766));
#56560=CARTESIAN_POINT('Ctrl Pts',(3.59578698050164,-1.,-1.27264798379365));
#56561=CARTESIAN_POINT('Ctrl Pts',(3.59578698050164,1.,-1.27264798379365));
#56562=CARTESIAN_POINT('Ctrl Pts',(3.60199947736404,-1.,-1.27622049908664));
#56563=CARTESIAN_POINT('Ctrl Pts',(3.60199947736404,1.,-1.27622049908664));
#56564=CARTESIAN_POINT('Ctrl Pts',(3.60808907746372,-1.,-1.27983492861703));
#56565=CARTESIAN_POINT('Ctrl Pts',(3.60808907746372,1.,-1.27983492861703));
#56566=CARTESIAN_POINT('Ctrl Pts',(3.61418935913793,-1.,-1.28353255117754));
#56567=CARTESIAN_POINT('Ctrl Pts',(3.61418935913793,1.,-1.28353255117754));
#56568=CARTESIAN_POINT('Ctrl Pts',(3.62038148492295,-1.,-1.2873375502936));
#56569=CARTESIAN_POINT('Ctrl Pts',(3.62038148492295,1.,-1.2873375502936));
#56570=CARTESIAN_POINT('Ctrl Pts',(3.62667616004299,-1.,-1.29125046021853));
#56571=CARTESIAN_POINT('Ctrl Pts',(3.62667616004299,1.,-1.29125046021853));
#56572=CARTESIAN_POINT('Ctrl Pts',(3.63304271630995,-1.,-1.29525810207744));
#56573=CARTESIAN_POINT('Ctrl Pts',(3.63304271630995,1.,-1.29525810207744));
#56574=CARTESIAN_POINT('Ctrl Pts',(3.6394268987279,-1.,-1.29933955906463));
#56575=CARTESIAN_POINT('Ctrl Pts',(3.6394268987279,1.,-1.29933955906463));
#56576=CARTESIAN_POINT('Ctrl Pts',(3.64577181380125,-1.,-1.30347327603778));
#56577=CARTESIAN_POINT('Ctrl Pts',(3.64577181380125,1.,-1.30347327603778));
#56578=CARTESIAN_POINT('Ctrl Pts',(3.65204081987101,-1.,-1.30764479590051));
#56579=CARTESIAN_POINT('Ctrl Pts',(3.65204081987101,1.,-1.30764479590051));
#56580=CARTESIAN_POINT('Ctrl Pts',(3.65822827358655,-1.,-1.31185038411231));
#56581=CARTESIAN_POINT('Ctrl Pts',(3.65822827358655,1.,-1.31185038411231));
#56582=CARTESIAN_POINT('Ctrl Pts',(3.66434688899822,-1.,-1.31609271239922));
#56583=CARTESIAN_POINT('Ctrl Pts',(3.66434688899822,1.,-1.31609271239922));
#56584=CARTESIAN_POINT('Ctrl Pts',(3.67042021752668,-1.,-1.3203782813777));
#56585=CARTESIAN_POINT('Ctrl Pts',(3.67042021752668,1.,-1.3203782813777));
#56586=CARTESIAN_POINT('Ctrl Pts',(3.67647355257906,-1.,-1.32471430856413));
#56587=CARTESIAN_POINT('Ctrl Pts',(3.67647355257906,1.,-1.32471430856413));
#56588=CARTESIAN_POINT('Ctrl Pts',(3.68252441182534,-1.,-1.32910547072734));
#56589=CARTESIAN_POINT('Ctrl Pts',(3.68252441182534,1.,-1.32910547072734));
#56590=CARTESIAN_POINT('Ctrl Pts',(3.68857672413013,-1.,-1.33355191034515));
#56591=CARTESIAN_POINT('Ctrl Pts',(3.68857672413013,1.,-1.33355191034515));
#56592=CARTESIAN_POINT('Ctrl Pts',(3.69462613305692,-1.,-1.33805103398214));
#56593=CARTESIAN_POINT('Ctrl Pts',(3.69462613305692,1.,-1.33805103398214));
#56594=CARTESIAN_POINT('Ctrl Pts',(3.70066324015112,-1.,-1.3425986075293));
#56595=CARTESIAN_POINT('Ctrl Pts',(3.70066324015112,1.,-1.3425986075293));
#56596=CARTESIAN_POINT('Ctrl Pts',(3.7066775318825,-1.,-1.34719008463535));
#56597=CARTESIAN_POINT('Ctrl Pts',(3.7066775318825,1.,-1.34719008463535));
#56598=CARTESIAN_POINT('Ctrl Pts',(3.71266130563061,-1.,-1.35182193384426));
#56599=CARTESIAN_POINT('Ctrl Pts',(3.71266130563061,1.,-1.35182193384426));
#56600=CARTESIAN_POINT('Ctrl Pts',(3.71861271513318,-1.,-1.35649266705038));
#56601=CARTESIAN_POINT('Ctrl Pts',(3.71861271513318,1.,-1.35649266705038));
#56602=CARTESIAN_POINT('Ctrl Pts',(3.72453364678279,-1.,-1.36120211416354));
#56603=CARTESIAN_POINT('Ctrl Pts',(3.72453364678279,1.,-1.36120211416354));
#56604=CARTESIAN_POINT('Ctrl Pts',(3.73042829011293,-1.,-1.36595093298674));
#56605=CARTESIAN_POINT('Ctrl Pts',(3.73042829011293,1.,-1.36595093298674));
#56606=CARTESIAN_POINT('Ctrl Pts',(3.73630145885809,-1.,-1.37074003422739));
#56607=CARTESIAN_POINT('Ctrl Pts',(3.73630145885809,1.,-1.37074003422739));
#56608=CARTESIAN_POINT('Ctrl Pts',(3.7421569816256,-1.,-1.3755700297169));
#56609=CARTESIAN_POINT('Ctrl Pts',(3.7421569816256,1.,-1.3755700297169));
#56610=CARTESIAN_POINT('Ctrl Pts',(3.74799617204744,-1.,-1.38044070763302));
#56611=CARTESIAN_POINT('Ctrl Pts',(3.74799617204744,1.,-1.38044070763302));
#56612=CARTESIAN_POINT('Ctrl Pts',(3.75381861212728,-1.,-1.38535129801185));
#56613=CARTESIAN_POINT('Ctrl Pts',(3.75381861212728,1.,-1.38535129801185));
#56614=CARTESIAN_POINT('Ctrl Pts',(3.75962280650875,-1.,-1.39030069388926));
#56615=CARTESIAN_POINT('Ctrl Pts',(3.75962280650875,1.,-1.39030069388926));
#56616=CARTESIAN_POINT('Ctrl Pts',(3.76540689249078,-1.,-1.39528769118054));
#56617=CARTESIAN_POINT('Ctrl Pts',(3.76540689249078,1.,-1.39528769118054));
#56618=CARTESIAN_POINT('Ctrl Pts',(3.77116930621804,-1.,-1.40031121335495));
#56619=CARTESIAN_POINT('Ctrl Pts',(3.77116930621804,1.,-1.40031121335495));
#56620=CARTESIAN_POINT('Ctrl Pts',(3.77690952014209,-1.,-1.40537056004702));
#56621=CARTESIAN_POINT('Ctrl Pts',(3.77690952014209,1.,-1.40537056004702));
#56622=CARTESIAN_POINT('Ctrl Pts',(3.78262780065406,-1.,-1.41046532282567));
#56623=CARTESIAN_POINT('Ctrl Pts',(3.78262780065406,1.,-1.41046532282567));
#56624=CARTESIAN_POINT('Ctrl Pts',(3.78832489879369,-1.,-1.41559527803808));
#56625=CARTESIAN_POINT('Ctrl Pts',(3.78832489879369,1.,-1.41559527803808));
#56626=CARTESIAN_POINT('Ctrl Pts',(3.7940017574439,-1.,-1.42076028482828));
#56627=CARTESIAN_POINT('Ctrl Pts',(3.7940017574439,1.,-1.42076028482828));
#56628=CARTESIAN_POINT('Ctrl Pts',(3.79965923196365,-1.,-1.42596018777301));
#56629=CARTESIAN_POINT('Ctrl Pts',(3.79965923196365,1.,-1.42596018777301));
#56630=CARTESIAN_POINT('Ctrl Pts',(3.80529775429916,-1.,-1.43119469921364));
#56631=CARTESIAN_POINT('Ctrl Pts',(3.80529775429916,1.,-1.43119469921364));
#56632=CARTESIAN_POINT('Ctrl Pts',(3.81091737726965,-1.,-1.43646341556783));
#56633=CARTESIAN_POINT('Ctrl Pts',(3.81091737726965,1.,-1.43646341556783));
#56634=CARTESIAN_POINT('Ctrl Pts',(3.8165179239855,-1.,-1.44176587041401));
#56635=CARTESIAN_POINT('Ctrl Pts',(3.8165179239855,1.,-1.44176587041401));
#56636=CARTESIAN_POINT('Ctrl Pts',(3.82209910620591,-1.,-1.44710157648562));
#56637=CARTESIAN_POINT('Ctrl Pts',(3.82209910620591,1.,-1.44710157648562));
#56638=CARTESIAN_POINT('Ctrl Pts',(3.82766064519,-1.,-1.45247006796807));
#56639=CARTESIAN_POINT('Ctrl Pts',(3.82766064519,1.,-1.45247006796807));
#56640=CARTESIAN_POINT('Ctrl Pts',(3.83320241775199,-1.,-1.45787095220763));
#56641=CARTESIAN_POINT('Ctrl Pts',(3.83320241775199,1.,-1.45787095220763));
#56642=CARTESIAN_POINT('Ctrl Pts',(3.83872447159309,-1.,-1.46330391180621));
#56643=CARTESIAN_POINT('Ctrl Pts',(3.83872447159309,1.,-1.46330391180621));
#56644=CARTESIAN_POINT('Ctrl Pts',(3.84422695454469,-1.,-1.46876867426375));
#56645=CARTESIAN_POINT('Ctrl Pts',(3.84422695454469,1.,-1.46876867426375));
#56646=CARTESIAN_POINT('Ctrl Pts',(3.84971006847096,-1.,-1.47426499018467));
#56647=CARTESIAN_POINT('Ctrl Pts',(3.84971006847096,1.,-1.47426499018467));
#56648=CARTESIAN_POINT('Ctrl Pts',(3.85517401698952,-1.,-1.47979260991063));
#56649=CARTESIAN_POINT('Ctrl Pts',(3.85517401698952,1.,-1.47979260991063));
#56650=CARTESIAN_POINT('Ctrl Pts',(3.86061894706551,-1.,-1.48535125510102));
#56651=CARTESIAN_POINT('Ctrl Pts',(3.86061894706551,1.,-1.48535125510102));
#56652=CARTESIAN_POINT('Ctrl Pts',(3.86604492575933,-1.,-1.49094061164604));
#56653=CARTESIAN_POINT('Ctrl Pts',(3.86604492575933,1.,-1.49094061164604));
#56654=CARTESIAN_POINT('Ctrl Pts',(3.8714519699927,-1.,-1.4965603539944));
#56655=CARTESIAN_POINT('Ctrl Pts',(3.8714519699927,1.,-1.4965603539944));
#56656=CARTESIAN_POINT('Ctrl Pts',(3.87684006372665,-1.,-1.50221016176766));
#56657=CARTESIAN_POINT('Ctrl Pts',(3.87684006372665,1.,-1.50221016176766));
#56658=CARTESIAN_POINT('Ctrl Pts',(3.88220917950443,-1.,-1.50788973857719));
#56659=CARTESIAN_POINT('Ctrl Pts',(3.88220917950443,1.,-1.50788973857719));
#56660=CARTESIAN_POINT('Ctrl Pts',(3.88755930032927,-1.,-1.51359883110181));
#56661=CARTESIAN_POINT('Ctrl Pts',(3.88755930032927,1.,-1.51359883110181));
#56662=CARTESIAN_POINT('Ctrl Pts',(3.89289043531893,-1.,-1.51933724328609));
#56663=CARTESIAN_POINT('Ctrl Pts',(3.89289043531893,1.,-1.51933724328609));
#56664=CARTESIAN_POINT('Ctrl Pts',(3.8982026070607,-1.,-1.52510482990784));
#56665=CARTESIAN_POINT('Ctrl Pts',(3.8982026070607,1.,-1.52510482990784));
#56666=CARTESIAN_POINT('Ctrl Pts',(3.90243719629755,-1.,-1.5297421605556));
#56667=CARTESIAN_POINT('Ctrl Pts',(3.90243719629755,1.,-1.5297421605556));
#56668=CARTESIAN_POINT('Ctrl Pts',(3.90560462812846,-1.,-1.53323321827311));
#56669=CARTESIAN_POINT('Ctrl Pts',(3.90560462812846,1.,-1.53323321827311));
#56670=CARTESIAN_POINT('Ctrl Pts',(3.90771246854607,-1.,-1.53556639217742));
#56671=CARTESIAN_POINT('Ctrl Pts',(3.90771246854607,1.,-1.53556639217742));
#56672=CARTESIAN_POINT('Ctrl Pts',(3.90876544355381,-1.,-1.53673442965256));
#56673=CARTESIAN_POINT('Ctrl Pts',(3.90876544355381,1.,-1.53673442965256));
#56674=CARTESIAN_POINT('',(3.5372048861591,1.,-1.24526366418208));
#56675=CARTESIAN_POINT('Ctrl Pts',(3.5372048861591,-1.,-1.24526366418208));
#56676=CARTESIAN_POINT('Ctrl Pts',(3.5372048861591,-0.666666666666667,-1.24526366418208));
#56677=CARTESIAN_POINT('Ctrl Pts',(3.5372048861591,-0.333333333333333,-1.24526366418208));
#56678=CARTESIAN_POINT('Ctrl Pts',(3.5372048861591,0.333333333333333,-1.24526366418208));
#56679=CARTESIAN_POINT('Ctrl Pts',(3.5372048861591,0.666666666666667,-1.24526366418208));
#56680=CARTESIAN_POINT('Ctrl Pts',(3.5372048861591,1.,-1.24526366418208));
#56681=CARTESIAN_POINT('',(3.90876544355381,1.,-1.53673442965256));
#56682=CARTESIAN_POINT('',(3.90876544355381,0.,-1.53673442965256));
#56683=CARTESIAN_POINT('Ctrl Pts',(3.5372048861591,1.,-1.24526366418208));
#56684=CARTESIAN_POINT('Ctrl Pts',(3.53725139174402,1.,-1.24524838931864));
#56685=CARTESIAN_POINT('Ctrl Pts',(3.53744859265385,1.,-1.24524498991133));
#56686=CARTESIAN_POINT('Ctrl Pts',(3.53808746578052,1.,-1.2453920538873));
#56687=CARTESIAN_POINT('Ctrl Pts',(3.53968291129942,1.,-1.24593497225964));
#56688=CARTESIAN_POINT('Ctrl Pts',(3.54294877426113,1.,-1.2472164623202));
#56689=CARTESIAN_POINT('Ctrl Pts',(3.54784190282889,1.,-1.24926408627938));
#56690=CARTESIAN_POINT('Ctrl Pts',(3.5538728741862,1.,-1.25188792940508));
#56691=CARTESIAN_POINT('Ctrl Pts',(3.56071094990825,1.,-1.25496090899873));
#56692=CARTESIAN_POINT('Ctrl Pts',(3.56798645995025,1.,-1.25834000485626));
#56693=CARTESIAN_POINT('Ctrl Pts',(3.5753456065164,1.,-1.26188667142784));
#56694=CARTESIAN_POINT('Ctrl Pts',(3.58250452868699,1.,-1.26548706249891));
#56695=CARTESIAN_POINT('Ctrl Pts',(3.5893180784647,1.,-1.26907758484766));
#56696=CARTESIAN_POINT('Ctrl Pts',(3.59578698050164,1.,-1.27264798379365));
#56697=CARTESIAN_POINT('Ctrl Pts',(3.60199947736404,1.,-1.27622049908664));
#56698=CARTESIAN_POINT('Ctrl Pts',(3.60808907746372,1.,-1.27983492861703));
#56699=CARTESIAN_POINT('Ctrl Pts',(3.61418935913793,1.,-1.28353255117754));
#56700=CARTESIAN_POINT('Ctrl Pts',(3.62038148492295,1.,-1.2873375502936));
#56701=CARTESIAN_POINT('Ctrl Pts',(3.62667616004299,1.,-1.29125046021853));
#56702=CARTESIAN_POINT('Ctrl Pts',(3.63304271630995,1.,-1.29525810207744));
#56703=CARTESIAN_POINT('Ctrl Pts',(3.6394268987279,1.,-1.29933955906463));
#56704=CARTESIAN_POINT('Ctrl Pts',(3.64577181380125,1.,-1.30347327603778));
#56705=CARTESIAN_POINT('Ctrl Pts',(3.65204081987101,1.,-1.30764479590051));
#56706=CARTESIAN_POINT('Ctrl Pts',(3.65822827358655,1.,-1.31185038411231));
#56707=CARTESIAN_POINT('Ctrl Pts',(3.66434688899822,1.,-1.31609271239922));
#56708=CARTESIAN_POINT('Ctrl Pts',(3.67042021752668,1.,-1.3203782813777));
#56709=CARTESIAN_POINT('Ctrl Pts',(3.67647355257906,1.,-1.32471430856413));
#56710=CARTESIAN_POINT('Ctrl Pts',(3.68252441182534,1.,-1.32910547072734));
#56711=CARTESIAN_POINT('Ctrl Pts',(3.68857672413013,1.,-1.33355191034515));
#56712=CARTESIAN_POINT('Ctrl Pts',(3.69462613305692,1.,-1.33805103398214));
#56713=CARTESIAN_POINT('Ctrl Pts',(3.70066324015112,1.,-1.3425986075293));
#56714=CARTESIAN_POINT('Ctrl Pts',(3.7066775318825,1.,-1.34719008463535));
#56715=CARTESIAN_POINT('Ctrl Pts',(3.71266130563061,1.,-1.35182193384426));
#56716=CARTESIAN_POINT('Ctrl Pts',(3.71861271513318,1.,-1.35649266705038));
#56717=CARTESIAN_POINT('Ctrl Pts',(3.72453364678279,1.,-1.36120211416354));
#56718=CARTESIAN_POINT('Ctrl Pts',(3.73042829011293,1.,-1.36595093298674));
#56719=CARTESIAN_POINT('Ctrl Pts',(3.73630145885809,1.,-1.37074003422739));
#56720=CARTESIAN_POINT('Ctrl Pts',(3.7421569816256,1.,-1.3755700297169));
#56721=CARTESIAN_POINT('Ctrl Pts',(3.74799617204744,1.,-1.38044070763302));
#56722=CARTESIAN_POINT('Ctrl Pts',(3.75381861212728,1.,-1.38535129801185));
#56723=CARTESIAN_POINT('Ctrl Pts',(3.75962280650875,1.,-1.39030069388926));
#56724=CARTESIAN_POINT('Ctrl Pts',(3.76540689249078,1.,-1.39528769118054));
#56725=CARTESIAN_POINT('Ctrl Pts',(3.77116930621804,1.,-1.40031121335495));
#56726=CARTESIAN_POINT('Ctrl Pts',(3.77690952014209,1.,-1.40537056004702));
#56727=CARTESIAN_POINT('Ctrl Pts',(3.78262780065406,1.,-1.41046532282567));
#56728=CARTESIAN_POINT('Ctrl Pts',(3.78832489879369,1.,-1.41559527803808));
#56729=CARTESIAN_POINT('Ctrl Pts',(3.7940017574439,1.,-1.42076028482828));
#56730=CARTESIAN_POINT('Ctrl Pts',(3.79965923196365,1.,-1.42596018777301));
#56731=CARTESIAN_POINT('Ctrl Pts',(3.80529775429916,1.,-1.43119469921364));
#56732=CARTESIAN_POINT('Ctrl Pts',(3.81091737726965,1.,-1.43646341556783));
#56733=CARTESIAN_POINT('Ctrl Pts',(3.8165179239855,1.,-1.44176587041401));
#56734=CARTESIAN_POINT('Ctrl Pts',(3.82209910620591,1.,-1.44710157648562));
#56735=CARTESIAN_POINT('Ctrl Pts',(3.82766064519,1.,-1.45247006796807));
#56736=CARTESIAN_POINT('Ctrl Pts',(3.83320241775199,1.,-1.45787095220763));
#56737=CARTESIAN_POINT('Ctrl Pts',(3.83872447159309,1.,-1.46330391180621));
#56738=CARTESIAN_POINT('Ctrl Pts',(3.84422695454469,1.,-1.46876867426375));
#56739=CARTESIAN_POINT('Ctrl Pts',(3.84971006847096,1.,-1.47426499018467));
#56740=CARTESIAN_POINT('Ctrl Pts',(3.85517401698952,1.,-1.47979260991063));
#56741=CARTESIAN_POINT('Ctrl Pts',(3.86061894706551,1.,-1.48535125510102));
#56742=CARTESIAN_POINT('Ctrl Pts',(3.86604492575933,1.,-1.49094061164604));
#56743=CARTESIAN_POINT('Ctrl Pts',(3.8714519699927,1.,-1.4965603539944));
#56744=CARTESIAN_POINT('Ctrl Pts',(3.87684006372665,1.,-1.50221016176766));
#56745=CARTESIAN_POINT('Ctrl Pts',(3.88220917950443,1.,-1.50788973857719));
#56746=CARTESIAN_POINT('Ctrl Pts',(3.88755930032927,1.,-1.51359883110181));
#56747=CARTESIAN_POINT('Ctrl Pts',(3.89289043531893,1.,-1.51933724328609));
#56748=CARTESIAN_POINT('Ctrl Pts',(3.8982026070607,1.,-1.52510482990784));
#56749=CARTESIAN_POINT('Ctrl Pts',(3.90243719629755,1.,-1.5297421605556));
#56750=CARTESIAN_POINT('Ctrl Pts',(3.90560462812846,1.,-1.53323321827311));
#56751=CARTESIAN_POINT('Ctrl Pts',(3.90771246854607,1.,-1.53556639217742));
#56752=CARTESIAN_POINT('Ctrl Pts',(3.90876544355381,1.,-1.53673442965256));
#56753=CARTESIAN_POINT('Origin',(3.90876544355381,0.,-1.53673442965256));
#56754=CARTESIAN_POINT('',(3.85054988729471,1.,-1.67727921511438));
#56755=CARTESIAN_POINT('Origin',(0.,0.,0.));
#56756=CARTESIAN_POINT('',(3.59360648251021,1.,-1.071677399622));
#56757=CARTESIAN_POINT('Origin',(0.,1.,0.));
#56758=CARTESIAN_POINT('Ctrl Pts',(3.59360648251021,1.,-1.071677399622));
#56759=CARTESIAN_POINT('Ctrl Pts',(3.59360648251021,0.666666666666667,-1.071677399622));
#56760=CARTESIAN_POINT('Ctrl Pts',(3.59360648251021,0.333333333333333,-1.071677399622));
#56761=CARTESIAN_POINT('Ctrl Pts',(3.59360648251021,-0.333333333333333,
-1.071677399622));
#56762=CARTESIAN_POINT('Ctrl Pts',(3.59360648251021,-0.666666666666667,
-1.071677399622));
#56763=CARTESIAN_POINT('Ctrl Pts',(3.59360648251021,-1.,-1.071677399622));
#56764=CARTESIAN_POINT('Ctrl Pts',(4.06552750530042,-1.,-1.05427041296137));
#56765=CARTESIAN_POINT('Ctrl Pts',(4.06552750530042,1.,-1.05427041296137));
#56766=CARTESIAN_POINT('Ctrl Pts',(4.06398907542679,-1.,-1.05459645194934));
#56767=CARTESIAN_POINT('Ctrl Pts',(4.06398907542679,1.,-1.05459645194934));
#56768=CARTESIAN_POINT('Ctrl Pts',(4.06091239150293,-1.,-1.05524507177901));
#56769=CARTESIAN_POINT('Ctrl Pts',(4.06091239150293,1.,-1.05524507177901));
#56770=CARTESIAN_POINT('Ctrl Pts',(4.05629789308941,-1.,-1.0562076270849));
#56771=CARTESIAN_POINT('Ctrl Pts',(4.05629789308941,1.,-1.0562076270849));
#56772=CARTESIAN_POINT('Ctrl Pts',(4.05014628387112,-1.,-1.05747027728537));
#56773=CARTESIAN_POINT('Ctrl Pts',(4.05014628387112,1.,-1.05747027728537));
#56774=CARTESIAN_POINT('Ctrl Pts',(4.04245854429333,-1.,-1.0590139366704));
#56775=CARTESIAN_POINT('Ctrl Pts',(4.04245854429333,1.,-1.0590139366704));
#56776=CARTESIAN_POINT('Ctrl Pts',(4.03477261142549,-1.,-1.06052284712114));
#56777=CARTESIAN_POINT('Ctrl Pts',(4.03477261142549,1.,-1.06052284712114));
#56778=CARTESIAN_POINT('Ctrl Pts',(4.02708855235732,-1.,-1.06199687787488));
#56779=CARTESIAN_POINT('Ctrl Pts',(4.02708855235732,1.,-1.06199687787488));
#56780=CARTESIAN_POINT('Ctrl Pts',(4.0194064749539,-1.,-1.06343586496094));
#56781=CARTESIAN_POINT('Ctrl Pts',(4.0194064749539,1.,-1.06343586496094));
#56782=CARTESIAN_POINT('Ctrl Pts',(4.0117265418656,-1.,-1.06483961342894));
#56783=CARTESIAN_POINT('Ctrl Pts',(4.0117265418656,1.,-1.06483961342894));
#56784=CARTESIAN_POINT('Ctrl Pts',(4.00404894951804,-1.,-1.06620789963406));
#56785=CARTESIAN_POINT('Ctrl Pts',(4.00404894951804,1.,-1.06620789963406));
#56786=CARTESIAN_POINT('Ctrl Pts',(3.99637389919958,-1.,-1.06754047381188));
#56787=CARTESIAN_POINT('Ctrl Pts',(3.99637389919958,1.,-1.06754047381188));
#56788=CARTESIAN_POINT('Ctrl Pts',(3.98870156857298,-1.,-1.06883706263912));
#56789=CARTESIAN_POINT('Ctrl Pts',(3.98870156857298,1.,-1.06883706263912));
#56790=CARTESIAN_POINT('Ctrl Pts',(3.98103208801289,-1.,-1.07009737257815));
#56791=CARTESIAN_POINT('Ctrl Pts',(3.98103208801289,1.,-1.07009737257815));
#56792=CARTESIAN_POINT('Ctrl Pts',(3.97336550222571,-1.,-1.07132109206252));
#56793=CARTESIAN_POINT('Ctrl Pts',(3.97336550222571,1.,-1.07132109206252));
#56794=CARTESIAN_POINT('Ctrl Pts',(3.96570179322681,-1.,-1.07250789943095));
#56795=CARTESIAN_POINT('Ctrl Pts',(3.96570179322681,1.,-1.07250789943095));
#56796=CARTESIAN_POINT('Ctrl Pts',(3.95804094429606,-1.,-1.07365747426551));
#56797=CARTESIAN_POINT('Ctrl Pts',(3.95804094429606,1.,-1.07365747426551));
#56798=CARTESIAN_POINT('Ctrl Pts',(3.95038299600754,-1.,-1.07476950921607));
#56799=CARTESIAN_POINT('Ctrl Pts',(3.95038299600754,1.,-1.07476950921607));
#56800=CARTESIAN_POINT('Ctrl Pts',(3.94272809633271,-1.,-1.07584371946428));
#56801=CARTESIAN_POINT('Ctrl Pts',(3.94272809633271,1.,-1.07584371946428));
#56802=CARTESIAN_POINT('Ctrl Pts',(3.93507657572743,-1.,-1.07687985975348));
#56803=CARTESIAN_POINT('Ctrl Pts',(3.93507657572743,1.,-1.07687985975348));
#56804=CARTESIAN_POINT('Ctrl Pts',(3.92742893349684,-1.,-1.07787771707155));
#56805=CARTESIAN_POINT('Ctrl Pts',(3.92742893349684,1.,-1.07787771707155));
#56806=CARTESIAN_POINT('Ctrl Pts',(3.91978568924062,-1.,-1.07883706663524));
#56807=CARTESIAN_POINT('Ctrl Pts',(3.91978568924062,1.,-1.07883706663524));
#56808=CARTESIAN_POINT('Ctrl Pts',(3.91214726022096,-1.,-1.0797576350746));
#56809=CARTESIAN_POINT('Ctrl Pts',(3.91214726022096,1.,-1.0797576350746));
#56810=CARTESIAN_POINT('Ctrl Pts',(3.90451384092564,-1.,-1.08063906483823));
#56811=CARTESIAN_POINT('Ctrl Pts',(3.90451384092564,1.,-1.08063906483823));
#56812=CARTESIAN_POINT('Ctrl Pts',(3.89688525098408,-1.,-1.08148086931373));
#56813=CARTESIAN_POINT('Ctrl Pts',(3.89688525098408,1.,-1.08148086931373));
#56814=CARTESIAN_POINT('Ctrl Pts',(3.88926088975182,-1.,-1.08228241999363));
#56815=CARTESIAN_POINT('Ctrl Pts',(3.88926088975182,1.,-1.08228241999363));
#56816=CARTESIAN_POINT('Ctrl Pts',(3.88164007721365,-1.,-1.08304304871042));
#56817=CARTESIAN_POINT('Ctrl Pts',(3.88164007721365,1.,-1.08304304871042));
#56818=CARTESIAN_POINT('Ctrl Pts',(3.87402233722563,-1.,-1.0837621330751));
#56819=CARTESIAN_POINT('Ctrl Pts',(3.87402233722563,1.,-1.0837621330751));
#56820=CARTESIAN_POINT('Ctrl Pts',(3.86640769434269,-1.,-1.08443918607926));
#56821=CARTESIAN_POINT('Ctrl Pts',(3.86640769434269,1.,-1.08443918607926));
#56822=CARTESIAN_POINT('Ctrl Pts',(3.85879698702511,-1.,-1.08507395120054));
#56823=CARTESIAN_POINT('Ctrl Pts',(3.85879698702511,1.,-1.08507395120054));
#56824=CARTESIAN_POINT('Ctrl Pts',(3.85119211322732,-1.,-1.08566647671838));
#56825=CARTESIAN_POINT('Ctrl Pts',(3.85119211322732,1.,-1.08566647671838));
#56826=CARTESIAN_POINT('Ctrl Pts',(3.84359528764934,-1.,-1.08621688337601));
#56827=CARTESIAN_POINT('Ctrl Pts',(3.84359528764934,1.,-1.08621688337601));
#56828=CARTESIAN_POINT('Ctrl Pts',(3.83600837071702,-1.,-1.08672515456901));
#56829=CARTESIAN_POINT('Ctrl Pts',(3.83600837071702,1.,-1.08672515456901));
#56830=CARTESIAN_POINT('Ctrl Pts',(3.82843215316985,-1.,-1.08719091307558));
#56831=CARTESIAN_POINT('Ctrl Pts',(3.82843215316985,1.,-1.08719091307558));
#56832=CARTESIAN_POINT('Ctrl Pts',(3.82086569676321,-1.,-1.08761321539442));
#56833=CARTESIAN_POINT('Ctrl Pts',(3.82086569676321,1.,-1.08761321539442));
#56834=CARTESIAN_POINT('Ctrl Pts',(3.81330554446324,-1.,-1.08799030610861));
#56835=CARTESIAN_POINT('Ctrl Pts',(3.81330554446324,1.,-1.08799030610861));
#56836=CARTESIAN_POINT('Ctrl Pts',(3.80574726657656,-1.,-1.08832009255378));
#56837=CARTESIAN_POINT('Ctrl Pts',(3.80574726657656,1.,-1.08832009255378));
#56838=CARTESIAN_POINT('Ctrl Pts',(3.79818708705252,-1.,-1.08860064435776));
#56839=CARTESIAN_POINT('Ctrl Pts',(3.79818708705252,1.,-1.08860064435776));
#56840=CARTESIAN_POINT('Ctrl Pts',(3.79062357974401,-1.,-1.08883071512097));
#56841=CARTESIAN_POINT('Ctrl Pts',(3.79062357974401,1.,-1.08883071512097));
#56842=CARTESIAN_POINT('Ctrl Pts',(3.78305911299511,-1.,-1.08901018614638));
#56843=CARTESIAN_POINT('Ctrl Pts',(3.78305911299511,1.,-1.08901018614638));
#56844=CARTESIAN_POINT('Ctrl Pts',(3.7755019940944,-1.,-1.08914072791275));
#56845=CARTESIAN_POINT('Ctrl Pts',(3.7755019940944,1.,-1.08914072791275));
#56846=CARTESIAN_POINT('Ctrl Pts',(3.76796340094469,-1.,-1.08922484204263));
#56847=CARTESIAN_POINT('Ctrl Pts',(3.76796340094469,1.,-1.08922484204263));
#56848=CARTESIAN_POINT('Ctrl Pts',(3.76045342580226,-1.,-1.08926462734287));
#56849=CARTESIAN_POINT('Ctrl Pts',(3.76045342580226,1.,-1.08926462734287));
#56850=CARTESIAN_POINT('Ctrl Pts',(3.75297711748138,-1.,-1.08926054632927));
#56851=CARTESIAN_POINT('Ctrl Pts',(3.75297711748138,1.,-1.08926054632927));
#56852=CARTESIAN_POINT('Ctrl Pts',(3.74553121371745,-1.,-1.08921040494013));
#56853=CARTESIAN_POINT('Ctrl Pts',(3.74553121371745,1.,-1.08921040494013));
#56854=CARTESIAN_POINT('Ctrl Pts',(3.73809879348209,-1.,-1.08910769013288));
#56855=CARTESIAN_POINT('Ctrl Pts',(3.73809879348209,1.,-1.08910769013288));
#56856=CARTESIAN_POINT('Ctrl Pts',(3.73065515162949,-1.,-1.08894337390925));
#56857=CARTESIAN_POINT('Ctrl Pts',(3.73065515162949,1.,-1.08894337390925));
#56858=CARTESIAN_POINT('Ctrl Pts',(3.72317741369364,-1.,-1.08870887220072));
#56859=CARTESIAN_POINT('Ctrl Pts',(3.72317741369364,1.,-1.08870887220072));
#56860=CARTESIAN_POINT('Ctrl Pts',(3.71565372339063,-1.,-1.08839887334777));
#56861=CARTESIAN_POINT('Ctrl Pts',(3.71565372339063,1.,-1.08839887334777));
#56862=CARTESIAN_POINT('Ctrl Pts',(3.70809084139476,-1.,-1.0880136731219));
#56863=CARTESIAN_POINT('Ctrl Pts',(3.70809084139476,1.,-1.0880136731219));
#56864=CARTESIAN_POINT('Ctrl Pts',(3.70052690909884,-1.,-1.08756311291324));
#56865=CARTESIAN_POINT('Ctrl Pts',(3.70052690909884,1.,-1.08756311291324));
#56866=CARTESIAN_POINT('Ctrl Pts',(3.69302062410229,-1.,-1.08706319540292));
#56867=CARTESIAN_POINT('Ctrl Pts',(3.69302062410229,1.,-1.08706319540292));
#56868=CARTESIAN_POINT('Ctrl Pts',(3.68562817420864,-1.,-1.08652888882609));
#56869=CARTESIAN_POINT('Ctrl Pts',(3.68562817420864,1.,-1.08652888882609));
#56870=CARTESIAN_POINT('Ctrl Pts',(3.67838211685148,-1.,-1.08596755755768));
#56871=CARTESIAN_POINT('Ctrl Pts',(3.67838211685148,1.,-1.08596755755768));
#56872=CARTESIAN_POINT('Ctrl Pts',(3.67127347729632,-1.,-1.0853733414448));
#56873=CARTESIAN_POINT('Ctrl Pts',(3.67127347729632,1.,-1.0853733414448));
#56874=CARTESIAN_POINT('Ctrl Pts',(3.66422237895256,-1.,-1.0847180992287));
#56875=CARTESIAN_POINT('Ctrl Pts',(3.66422237895256,1.,-1.0847180992287));
#56876=CARTESIAN_POINT('Ctrl Pts',(3.65709649161004,-1.,-1.08395671077761));
#56877=CARTESIAN_POINT('Ctrl Pts',(3.65709649161004,1.,-1.08395671077761));
#56878=CARTESIAN_POINT('Ctrl Pts',(3.64976441208197,-1.,-1.08304289898577));
#56879=CARTESIAN_POINT('Ctrl Pts',(3.64976441208197,1.,-1.08304289898577));
#56880=CARTESIAN_POINT('Ctrl Pts',(3.64214167843595,-1.,-1.08194278850972));
#56881=CARTESIAN_POINT('Ctrl Pts',(3.64214167843595,1.,-1.08194278850972));
#56882=CARTESIAN_POINT('Ctrl Pts',(3.63423373196602,-1.,-1.08064765719887));
#56883=CARTESIAN_POINT('Ctrl Pts',(3.63423373196602,1.,-1.08064765719887));
#56884=CARTESIAN_POINT('Ctrl Pts',(3.62619537902616,-1.,-1.07919137290816));
#56885=CARTESIAN_POINT('Ctrl Pts',(3.62619537902616,1.,-1.07919137290816));
#56886=CARTESIAN_POINT('Ctrl Pts',(3.61832318504957,-1.,-1.07764868137729));
#56887=CARTESIAN_POINT('Ctrl Pts',(3.61832318504957,1.,-1.07764868137729));
#56888=CARTESIAN_POINT('Ctrl Pts',(3.61098481349577,-1.,-1.07611545402841));
#56889=CARTESIAN_POINT('Ctrl Pts',(3.61098481349577,1.,-1.07611545402841));
#56890=CARTESIAN_POINT('Ctrl Pts',(3.6045633988796,-1.,-1.0746932716863));
#56891=CARTESIAN_POINT('Ctrl Pts',(3.6045633988796,1.,-1.0746932716863));
#56892=CARTESIAN_POINT('Ctrl Pts',(3.59940121154383,-1.,-1.0734737254567));
#56893=CARTESIAN_POINT('Ctrl Pts',(3.59940121154383,1.,-1.0734737254567));
#56894=CARTESIAN_POINT('Ctrl Pts',(3.59573039611837,-1.,-1.07251922679108));
#56895=CARTESIAN_POINT('Ctrl Pts',(3.59573039611837,1.,-1.07251922679108));
#56896=CARTESIAN_POINT('Ctrl Pts',(3.59407399103556,-1.,-1.07199116987503));
#56897=CARTESIAN_POINT('Ctrl Pts',(3.59407399103556,1.,-1.07199116987503));
#56898=CARTESIAN_POINT('Ctrl Pts',(3.59356848057451,-1.,-1.07173216219041));
#56899=CARTESIAN_POINT('Ctrl Pts',(3.59356848057451,1.,-1.07173216219041));
#56900=CARTESIAN_POINT('Ctrl Pts',(3.59355870577763,-1.,-1.07162034256419));
#56901=CARTESIAN_POINT('Ctrl Pts',(3.59355870577763,1.,-1.07162034256419));
#56902=CARTESIAN_POINT('Ctrl Pts',(3.59363563249864,-1.,-1.07157964745328));
#56903=CARTESIAN_POINT('Ctrl Pts',(3.59363563249864,1.,-1.07157964745328));
#56904=CARTESIAN_POINT('',(4.06552750530042,1.,-1.05427041296137));
#56905=CARTESIAN_POINT('Ctrl Pts',(4.06552750530042,1.,-1.05427041296137));
#56906=CARTESIAN_POINT('Ctrl Pts',(4.06398907542679,1.,-1.05459645194934));
#56907=CARTESIAN_POINT('Ctrl Pts',(4.06091239150293,1.,-1.05524507177901));
#56908=CARTESIAN_POINT('Ctrl Pts',(4.05629789308941,1.,-1.0562076270849));
#56909=CARTESIAN_POINT('Ctrl Pts',(4.05014628387112,1.,-1.05747027728537));
#56910=CARTESIAN_POINT('Ctrl Pts',(4.04245854429333,1.,-1.0590139366704));
#56911=CARTESIAN_POINT('Ctrl Pts',(4.03477261142549,1.,-1.06052284712114));
#56912=CARTESIAN_POINT('Ctrl Pts',(4.02708855235732,1.,-1.06199687787488));
#56913=CARTESIAN_POINT('Ctrl Pts',(4.0194064749539,1.,-1.06343586496094));
#56914=CARTESIAN_POINT('Ctrl Pts',(4.0117265418656,1.,-1.06483961342894));
#56915=CARTESIAN_POINT('Ctrl Pts',(4.00404894951804,1.,-1.06620789963406));
#56916=CARTESIAN_POINT('Ctrl Pts',(3.99637389919958,1.,-1.06754047381188));
#56917=CARTESIAN_POINT('Ctrl Pts',(3.98870156857298,1.,-1.06883706263912));
#56918=CARTESIAN_POINT('Ctrl Pts',(3.98103208801289,1.,-1.07009737257815));
#56919=CARTESIAN_POINT('Ctrl Pts',(3.97336550222571,1.,-1.07132109206252));
#56920=CARTESIAN_POINT('Ctrl Pts',(3.96570179322681,1.,-1.07250789943095));
#56921=CARTESIAN_POINT('Ctrl Pts',(3.95804094429606,1.,-1.07365747426551));
#56922=CARTESIAN_POINT('Ctrl Pts',(3.95038299600754,1.,-1.07476950921607));
#56923=CARTESIAN_POINT('Ctrl Pts',(3.94272809633271,1.,-1.07584371946428));
#56924=CARTESIAN_POINT('Ctrl Pts',(3.93507657572743,1.,-1.07687985975348));
#56925=CARTESIAN_POINT('Ctrl Pts',(3.92742893349684,1.,-1.07787771707155));
#56926=CARTESIAN_POINT('Ctrl Pts',(3.91978568924062,1.,-1.07883706663524));
#56927=CARTESIAN_POINT('Ctrl Pts',(3.91214726022096,1.,-1.0797576350746));
#56928=CARTESIAN_POINT('Ctrl Pts',(3.90451384092564,1.,-1.08063906483823));
#56929=CARTESIAN_POINT('Ctrl Pts',(3.89688525098408,1.,-1.08148086931373));
#56930=CARTESIAN_POINT('Ctrl Pts',(3.88926088975182,1.,-1.08228241999363));
#56931=CARTESIAN_POINT('Ctrl Pts',(3.88164007721365,1.,-1.08304304871042));
#56932=CARTESIAN_POINT('Ctrl Pts',(3.87402233722563,1.,-1.0837621330751));
#56933=CARTESIAN_POINT('Ctrl Pts',(3.86640769434269,1.,-1.08443918607926));
#56934=CARTESIAN_POINT('Ctrl Pts',(3.85879698702511,1.,-1.08507395120054));
#56935=CARTESIAN_POINT('Ctrl Pts',(3.85119211322732,1.,-1.08566647671838));
#56936=CARTESIAN_POINT('Ctrl Pts',(3.84359528764934,1.,-1.08621688337601));
#56937=CARTESIAN_POINT('Ctrl Pts',(3.83600837071702,1.,-1.08672515456901));
#56938=CARTESIAN_POINT('Ctrl Pts',(3.82843215316985,1.,-1.08719091307558));
#56939=CARTESIAN_POINT('Ctrl Pts',(3.82086569676321,1.,-1.08761321539442));
#56940=CARTESIAN_POINT('Ctrl Pts',(3.81330554446324,1.,-1.08799030610861));
#56941=CARTESIAN_POINT('Ctrl Pts',(3.80574726657656,1.,-1.08832009255378));
#56942=CARTESIAN_POINT('Ctrl Pts',(3.79818708705252,1.,-1.08860064435776));
#56943=CARTESIAN_POINT('Ctrl Pts',(3.79062357974401,1.,-1.08883071512097));
#56944=CARTESIAN_POINT('Ctrl Pts',(3.78305911299511,1.,-1.08901018614638));
#56945=CARTESIAN_POINT('Ctrl Pts',(3.7755019940944,1.,-1.08914072791275));
#56946=CARTESIAN_POINT('Ctrl Pts',(3.76796340094469,1.,-1.08922484204263));
#56947=CARTESIAN_POINT('Ctrl Pts',(3.76045342580226,1.,-1.08926462734287));
#56948=CARTESIAN_POINT('Ctrl Pts',(3.75297711748138,1.,-1.08926054632927));
#56949=CARTESIAN_POINT('Ctrl Pts',(3.74553121371745,1.,-1.08921040494013));
#56950=CARTESIAN_POINT('Ctrl Pts',(3.73809879348209,1.,-1.08910769013288));
#56951=CARTESIAN_POINT('Ctrl Pts',(3.73065515162949,1.,-1.08894337390925));
#56952=CARTESIAN_POINT('Ctrl Pts',(3.72317741369364,1.,-1.08870887220072));
#56953=CARTESIAN_POINT('Ctrl Pts',(3.71565372339063,1.,-1.08839887334777));
#56954=CARTESIAN_POINT('Ctrl Pts',(3.70809084139476,1.,-1.0880136731219));
#56955=CARTESIAN_POINT('Ctrl Pts',(3.70052690909884,1.,-1.08756311291324));
#56956=CARTESIAN_POINT('Ctrl Pts',(3.69302062410229,1.,-1.08706319540292));
#56957=CARTESIAN_POINT('Ctrl Pts',(3.68562817420864,1.,-1.08652888882609));
#56958=CARTESIAN_POINT('Ctrl Pts',(3.67838211685148,1.,-1.08596755755768));
#56959=CARTESIAN_POINT('Ctrl Pts',(3.67127347729632,1.,-1.0853733414448));
#56960=CARTESIAN_POINT('Ctrl Pts',(3.66422237895256,1.,-1.0847180992287));
#56961=CARTESIAN_POINT('Ctrl Pts',(3.65709649161004,1.,-1.08395671077761));
#56962=CARTESIAN_POINT('Ctrl Pts',(3.64976441208197,1.,-1.08304289898577));
#56963=CARTESIAN_POINT('Ctrl Pts',(3.64214167843595,1.,-1.08194278850972));
#56964=CARTESIAN_POINT('Ctrl Pts',(3.63423373196602,1.,-1.08064765719887));
#56965=CARTESIAN_POINT('Ctrl Pts',(3.62619537902616,1.,-1.07919137290816));
#56966=CARTESIAN_POINT('Ctrl Pts',(3.61832318504957,1.,-1.07764868137729));
#56967=CARTESIAN_POINT('Ctrl Pts',(3.61098481349577,1.,-1.07611545402841));
#56968=CARTESIAN_POINT('Ctrl Pts',(3.6045633988796,1.,-1.0746932716863));
#56969=CARTESIAN_POINT('Ctrl Pts',(3.59940121154383,1.,-1.0734737254567));
#56970=CARTESIAN_POINT('Ctrl Pts',(3.59600583195037,1.,-1.07259084660947));
#56971=CARTESIAN_POINT('Ctrl Pts',(3.59439597,1.,-1.07209229745284));
#56972=CARTESIAN_POINT('Ctrl Pts',(3.59379266874663,1.,-1.07183575450716));
#56973=CARTESIAN_POINT('Ctrl Pts',(3.59363512797985,1.,-1.07171709254271));
#56974=CARTESIAN_POINT('Ctrl Pts',(3.59360648251021,1.,-1.071677399622));
#56975=CARTESIAN_POINT('',(4.06552750530042,0.,-1.05427041296137));
#56976=CARTESIAN_POINT('Origin',(4.10104028313088,0.,-0.906349047628866));
#56977=CARTESIAN_POINT('',(4.10104028313088,1.,-0.906349047628866));
#56978=CARTESIAN_POINT('',(4.06552750530042,1.,-1.05427041296137));
#56979=CARTESIAN_POINT('',(4.10104028313088,0.,-0.906349047628866));
#56980=CARTESIAN_POINT('Ctrl Pts',(3.68843977377012,-1.,-0.676691979611561));
#56981=CARTESIAN_POINT('Ctrl Pts',(3.68843977377012,1.,-0.676691979611561));
#56982=CARTESIAN_POINT('Ctrl Pts',(3.68838970675497,-1.,-0.67662079600199));
#56983=CARTESIAN_POINT('Ctrl Pts',(3.68838970675497,1.,-0.67662079600199));
#56984=CARTESIAN_POINT('Ctrl Pts',(3.68844918121303,-1.,-0.676525601650856));
#56985=CARTESIAN_POINT('Ctrl Pts',(3.68844918121303,1.,-0.676525601650856));
#56986=CARTESIAN_POINT('Ctrl Pts',(3.68901718136181,-1.,-0.676524321061226));
#56987=CARTESIAN_POINT('Ctrl Pts',(3.68901718136181,1.,-0.676524321061226));
#56988=CARTESIAN_POINT('Ctrl Pts',(3.69073278191994,-1.,-0.676805811075091));
#56989=CARTESIAN_POINT('Ctrl Pts',(3.69073278191994,1.,-0.676805811075091));
#56990=CARTESIAN_POINT('Ctrl Pts',(3.69443683573598,-1.,-0.677621861865498));
#56991=CARTESIAN_POINT('Ctrl Pts',(3.69443683573598,1.,-0.677621861865498));
#56992=CARTESIAN_POINT('Ctrl Pts',(3.69959004073005,-1.,-0.678878822226027));
#56993=CARTESIAN_POINT('Ctrl Pts',(3.69959004073005,1.,-0.678878822226027));
#56994=CARTESIAN_POINT('Ctrl Pts',(3.70595722031785,-1.,-0.680526909710877));
#56995=CARTESIAN_POINT('Ctrl Pts',(3.70595722031785,1.,-0.680526909710877));
#56996=CARTESIAN_POINT('Ctrl Pts',(3.71319182789943,-1.,-0.68249234510893));
#56997=CARTESIAN_POINT('Ctrl Pts',(3.71319182789943,1.,-0.68249234510893));
#56998=CARTESIAN_POINT('Ctrl Pts',(3.7209063713926,-1.,-0.684691698167848));
#56999=CARTESIAN_POINT('Ctrl Pts',(3.7209063713926,1.,-0.684691698167848));
#57000=CARTESIAN_POINT('Ctrl Pts',(3.72872973554051,-1.,-0.687043475232355));
#57001=CARTESIAN_POINT('Ctrl Pts',(3.72872973554051,1.,-0.687043475232355));
#57002=CARTESIAN_POINT('Ctrl Pts',(3.73636374475077,-1.,-0.689479637354814));
#57003=CARTESIAN_POINT('Ctrl Pts',(3.73636374475077,1.,-0.689479637354814));
#57004=CARTESIAN_POINT('Ctrl Pts',(3.74365508986712,-1.,-0.69196008040082));
#57005=CARTESIAN_POINT('Ctrl Pts',(3.74365508986712,1.,-0.69196008040082));
#57006=CARTESIAN_POINT('Ctrl Pts',(3.75060288243455,-1.,-0.694474562581493));
#57007=CARTESIAN_POINT('Ctrl Pts',(3.75060288243455,1.,-0.694474562581493));
#57008=CARTESIAN_POINT('Ctrl Pts',(3.75729775767023,-1.,-0.697031245659744));
#57009=CARTESIAN_POINT('Ctrl Pts',(3.75729775767023,1.,-0.697031245659744));
#57010=CARTESIAN_POINT('Ctrl Pts',(3.76387780603759,-1.,-0.699648552230917));
#57011=CARTESIAN_POINT('Ctrl Pts',(3.76387780603759,1.,-0.699648552230917));
#57012=CARTESIAN_POINT('Ctrl Pts',(3.77048141872872,-1.,-0.702346356621552));
#57013=CARTESIAN_POINT('Ctrl Pts',(3.77048141872872,1.,-0.702346356621552));
#57014=CARTESIAN_POINT('Ctrl Pts',(3.77719254217129,-1.,-0.705135847999817));
#57015=CARTESIAN_POINT('Ctrl Pts',(3.77719254217129,1.,-0.705135847999817));
#57016=CARTESIAN_POINT('Ctrl Pts',(3.78402183336605,-1.,-0.708015879375459));
#57017=CARTESIAN_POINT('Ctrl Pts',(3.78402183336605,1.,-0.708015879375459));
#57018=CARTESIAN_POINT('Ctrl Pts',(3.79093694007094,-1.,-0.710978231689017));
#57019=CARTESIAN_POINT('Ctrl Pts',(3.79093694007094,1.,-0.710978231689017));
#57020=CARTESIAN_POINT('Ctrl Pts',(3.79788100314975,-1.,-0.714010733006641));
#57021=CARTESIAN_POINT('Ctrl Pts',(3.79788100314975,1.,-0.714010733006641));
#57022=CARTESIAN_POINT('Ctrl Pts',(3.80479445759309,-1.,-0.717100993669115));
#57023=CARTESIAN_POINT('Ctrl Pts',(3.80479445759309,1.,-0.717100993669115));
#57024=CARTESIAN_POINT('Ctrl Pts',(3.81163885127344,-1.,-0.720240466589236));
#57025=CARTESIAN_POINT('Ctrl Pts',(3.81163885127344,1.,-0.720240466589236));
#57026=CARTESIAN_POINT('Ctrl Pts',(3.81840802610835,-1.,-0.723426346019423));
#57027=CARTESIAN_POINT('Ctrl Pts',(3.81840802610835,1.,-0.723426346019423));
#57028=CARTESIAN_POINT('Ctrl Pts',(3.82511495756713,-1.,-0.726659281876664));
#57029=CARTESIAN_POINT('Ctrl Pts',(3.82511495756713,1.,-0.726659281876664));
#57030=CARTESIAN_POINT('Ctrl Pts',(3.83178392403383,-1.,-0.729942010490168));
#57031=CARTESIAN_POINT('Ctrl Pts',(3.83178392403383,1.,-0.729942010490168));
#57032=CARTESIAN_POINT('Ctrl Pts',(3.83844103658009,-1.,-0.733277703756078));
#57033=CARTESIAN_POINT('Ctrl Pts',(3.83844103658009,1.,-0.733277703756078));
#57034=CARTESIAN_POINT('Ctrl Pts',(3.84510432881213,-1.,-0.736668240497118));
#57035=CARTESIAN_POINT('Ctrl Pts',(3.84510432881213,1.,-0.736668240497118));
#57036=CARTESIAN_POINT('Ctrl Pts',(3.85177770351215,-1.,-0.740113146827137));
#57037=CARTESIAN_POINT('Ctrl Pts',(3.85177770351215,1.,-0.740113146827137));
#57038=CARTESIAN_POINT('Ctrl Pts',(3.85845645217594,-1.,-0.743610542737013));
#57039=CARTESIAN_POINT('Ctrl Pts',(3.85845645217594,1.,-0.743610542737013));
#57040=CARTESIAN_POINT('Ctrl Pts',(3.86513062969889,-1.,-0.747157716488871));
#57041=CARTESIAN_POINT('Ctrl Pts',(3.86513062969889,1.,-0.747157716488871));
#57042=CARTESIAN_POINT('Ctrl Pts',(3.87178914078374,-1.,-0.750751822383028));
#57043=CARTESIAN_POINT('Ctrl Pts',(3.87178914078374,1.,-0.750751822383028));
#57044=CARTESIAN_POINT('Ctrl Pts',(3.87842382520065,-1.,-0.754390577396857));
#57045=CARTESIAN_POINT('Ctrl Pts',(3.87842382520065,1.,-0.754390577396857));
#57046=CARTESIAN_POINT('Ctrl Pts',(3.88503262662689,-1.,-0.758072800564801));
#57047=CARTESIAN_POINT('Ctrl Pts',(3.88503262662689,1.,-0.758072800564801));
#57048=CARTESIAN_POINT('Ctrl Pts',(3.89161738162245,-1.,-0.76179802879397));
#57049=CARTESIAN_POINT('Ctrl Pts',(3.89161738162245,1.,-0.76179802879397));
#57050=CARTESIAN_POINT('Ctrl Pts',(3.89818233104378,-1.,-0.765566256401296));
#57051=CARTESIAN_POINT('Ctrl Pts',(3.89818233104378,1.,-0.765566256401296));
#57052=CARTESIAN_POINT('Ctrl Pts',(3.90473237182633,-1.,-0.769377629847874));
#57053=CARTESIAN_POINT('Ctrl Pts',(3.90473237182633,1.,-0.769377629847874));
#57054=CARTESIAN_POINT('Ctrl Pts',(3.91127138115243,-1.,-0.773232154506321));
#57055=CARTESIAN_POINT('Ctrl Pts',(3.91127138115243,1.,-0.773232154506321));
#57056=CARTESIAN_POINT('Ctrl Pts',(3.9178006233448,-1.,-0.777129415664956));
#57057=CARTESIAN_POINT('Ctrl Pts',(3.9178006233448,1.,-0.777129415664956));
#57058=CARTESIAN_POINT('Ctrl Pts',(3.92431956510441,-1.,-0.781068718228451));
#57059=CARTESIAN_POINT('Ctrl Pts',(3.92431956510441,1.,-0.781068718228451));
#57060=CARTESIAN_POINT('Ctrl Pts',(3.93082655631789,-1.,-0.785049202786508));
#57061=CARTESIAN_POINT('Ctrl Pts',(3.93082655631789,1.,-0.785049202786508));
#57062=CARTESIAN_POINT('Ctrl Pts',(3.93731956885676,-1.,-0.789069971469333));
#57063=CARTESIAN_POINT('Ctrl Pts',(3.93731956885676,1.,-0.789069971469333));
#57064=CARTESIAN_POINT('Ctrl Pts',(3.94379688971283,-1.,-0.793130205640961));
#57065=CARTESIAN_POINT('Ctrl Pts',(3.94379688971283,1.,-0.793130205640961));
#57066=CARTESIAN_POINT('Ctrl Pts',(3.95025788827136,-1.,-0.797229296085316));
#57067=CARTESIAN_POINT('Ctrl Pts',(3.95025788827136,1.,-0.797229296085316));
#57068=CARTESIAN_POINT('Ctrl Pts',(3.95670276375108,-1.,-0.80136679772705));
#57069=CARTESIAN_POINT('Ctrl Pts',(3.95670276375108,1.,-0.80136679772705));
#57070=CARTESIAN_POINT('Ctrl Pts',(3.96313222295815,-1.,-0.805542372178362));
#57071=CARTESIAN_POINT('Ctrl Pts',(3.96313222295815,1.,-0.805542372178362));
#57072=CARTESIAN_POINT('Ctrl Pts',(3.96954717513232,-1.,-0.809755732818091));
#57073=CARTESIAN_POINT('Ctrl Pts',(3.96954717513232,1.,-0.809755732818091));
#57074=CARTESIAN_POINT('Ctrl Pts',(3.97594844078811,-1.,-0.814006592328844));
#57075=CARTESIAN_POINT('Ctrl Pts',(3.97594844078811,1.,-0.814006592328844));
#57076=CARTESIAN_POINT('Ctrl Pts',(3.98233640155404,-1.,-0.818294599022294));
#57077=CARTESIAN_POINT('Ctrl Pts',(3.98233640155404,1.,-0.818294599022294));
#57078=CARTESIAN_POINT('Ctrl Pts',(3.98871104646485,-1.,-0.822619346022119));
#57079=CARTESIAN_POINT('Ctrl Pts',(3.98871104646485,1.,-0.822619346022119));
#57080=CARTESIAN_POINT('Ctrl Pts',(3.99507212784431,-1.,-0.82698040032079));
#57081=CARTESIAN_POINT('Ctrl Pts',(3.99507212784431,1.,-0.82698040032079));
#57082=CARTESIAN_POINT('Ctrl Pts',(4.00141928477507,-1.,-0.831377325741623));
#57083=CARTESIAN_POINT('Ctrl Pts',(4.00141928477507,1.,-0.831377325741623));
#57084=CARTESIAN_POINT('Ctrl Pts',(4.00775216907856,-1.,-0.835809705809646));
#57085=CARTESIAN_POINT('Ctrl Pts',(4.00775216907856,1.,-0.835809705809646));
#57086=CARTESIAN_POINT('Ctrl Pts',(4.01407059766103,-1.,-0.840277171975855));
#57087=CARTESIAN_POINT('Ctrl Pts',(4.01407059766103,1.,-0.840277171975855));
#57088=CARTESIAN_POINT('Ctrl Pts',(4.02037456798441,-1.,-0.844779403287746));
#57089=CARTESIAN_POINT('Ctrl Pts',(4.02037456798441,1.,-0.844779403287746));
#57090=CARTESIAN_POINT('Ctrl Pts',(4.02666418343164,-1.,-0.849316107474245));
#57091=CARTESIAN_POINT('Ctrl Pts',(4.02666418343164,1.,-0.849316107474245));
#57092=CARTESIAN_POINT('Ctrl Pts',(4.03293960436756,-1.,-0.853887006631755));
#57093=CARTESIAN_POINT('Ctrl Pts',(4.03293960436756,1.,-0.853887006631755));
#57094=CARTESIAN_POINT('Ctrl Pts',(4.03920099284773,-1.,-0.858491822322828));
#57095=CARTESIAN_POINT('Ctrl Pts',(4.03920099284773,1.,-0.858491822322828));
#57096=CARTESIAN_POINT('Ctrl Pts',(4.04544845048584,-1.,-0.863130256643259));
#57097=CARTESIAN_POINT('Ctrl Pts',(4.04544845048584,1.,-0.863130256643259));
#57098=CARTESIAN_POINT('Ctrl Pts',(4.05168199437909,-1.,-0.867801988859918));
#57099=CARTESIAN_POINT('Ctrl Pts',(4.05168199437909,1.,-0.867801988859918));
#57100=CARTESIAN_POINT('Ctrl Pts',(4.0579015903134,-1.,-0.872506694782446));
#57101=CARTESIAN_POINT('Ctrl Pts',(4.0579015903134,1.,-0.872506694782446));
#57102=CARTESIAN_POINT('Ctrl Pts',(4.06410717232905,-1.,-0.877244060485838));
#57103=CARTESIAN_POINT('Ctrl Pts',(4.06410717232905,1.,-0.877244060485838));
#57104=CARTESIAN_POINT('Ctrl Pts',(4.07029866694192,-1.,-0.882013797525692));
#57105=CARTESIAN_POINT('Ctrl Pts',(4.07029866694192,1.,-0.882013797525692));
#57106=CARTESIAN_POINT('Ctrl Pts',(4.07647601773635,-1.,-0.886815658358501));
#57107=CARTESIAN_POINT('Ctrl Pts',(4.07647601773635,1.,-0.886815658358501));
#57108=CARTESIAN_POINT('Ctrl Pts',(4.08263920304799,-1.,-0.891649447916278));
#57109=CARTESIAN_POINT('Ctrl Pts',(4.08263920304799,1.,-0.891649447916278));
#57110=CARTESIAN_POINT('Ctrl Pts',(4.08878822246833,-1.,-0.896515019231334));
#57111=CARTESIAN_POINT('Ctrl Pts',(4.08878822246833,1.,-0.896515019231334));
#57112=CARTESIAN_POINT('Ctrl Pts',(4.09369611522387,-1.,-0.900432820941675));
#57113=CARTESIAN_POINT('Ctrl Pts',(4.09369611522387,1.,-0.900432820941675));
#57114=CARTESIAN_POINT('Ctrl Pts',(4.09737067245935,-1.,-0.903385402441588));
#57115=CARTESIAN_POINT('Ctrl Pts',(4.09737067245935,1.,-0.903385402441588));
#57116=CARTESIAN_POINT('Ctrl Pts',(4.09981755067523,-1.,-0.905360112215337));
#57117=CARTESIAN_POINT('Ctrl Pts',(4.09981755067523,1.,-0.905360112215337));
#57118=CARTESIAN_POINT('Ctrl Pts',(4.10104028313088,-1.,-0.906349047628866));
#57119=CARTESIAN_POINT('Ctrl Pts',(4.10104028313088,1.,-0.906349047628866));
#57120=CARTESIAN_POINT('',(3.68845817949586,1.,-0.676591647975427));
#57121=CARTESIAN_POINT('Ctrl Pts',(3.68845817949586,-1.,-0.676591647975429));
#57122=CARTESIAN_POINT('Ctrl Pts',(3.68845817949586,-0.666666666666667,
-0.676591647975429));
#57123=CARTESIAN_POINT('Ctrl Pts',(3.68845817949586,-0.333333333333333,
-0.676591647975429));
#57124=CARTESIAN_POINT('Ctrl Pts',(3.68845817949586,0.333333333333333,-0.676591647975429));
#57125=CARTESIAN_POINT('Ctrl Pts',(3.68845817949586,0.666666666666667,-0.676591647975429));
#57126=CARTESIAN_POINT('Ctrl Pts',(3.68845817949586,1.,-0.676591647975429));
#57127=CARTESIAN_POINT('Ctrl Pts',(3.68845817949586,1.,-0.676591647975428));
#57128=CARTESIAN_POINT('Ctrl Pts',(3.68850172300477,1.,-0.676569286094606));
#57129=CARTESIAN_POINT('Ctrl Pts',(3.68869596425969,1.,-0.676535079520807));
#57130=CARTESIAN_POINT('Ctrl Pts',(3.68934997767243,1.,-0.676580391119397));
#57131=CARTESIAN_POINT('Ctrl Pts',(3.69101071175464,1.,-0.676867042599402));
#57132=CARTESIAN_POINT('Ctrl Pts',(3.69443683573598,1.,-0.677621861865498));
#57133=CARTESIAN_POINT('Ctrl Pts',(3.69959004073005,1.,-0.678878822226027));
#57134=CARTESIAN_POINT('Ctrl Pts',(3.70595722031785,1.,-0.680526909710877));
#57135=CARTESIAN_POINT('Ctrl Pts',(3.71319182789943,1.,-0.68249234510893));
#57136=CARTESIAN_POINT('Ctrl Pts',(3.7209063713926,1.,-0.684691698167848));
#57137=CARTESIAN_POINT('Ctrl Pts',(3.72872973554051,1.,-0.687043475232355));
#57138=CARTESIAN_POINT('Ctrl Pts',(3.73636374475077,1.,-0.689479637354814));
#57139=CARTESIAN_POINT('Ctrl Pts',(3.74365508986712,1.,-0.69196008040082));
#57140=CARTESIAN_POINT('Ctrl Pts',(3.75060288243455,1.,-0.694474562581493));
#57141=CARTESIAN_POINT('Ctrl Pts',(3.75729775767023,1.,-0.697031245659744));
#57142=CARTESIAN_POINT('Ctrl Pts',(3.76387780603759,1.,-0.699648552230917));
#57143=CARTESIAN_POINT('Ctrl Pts',(3.77048141872872,1.,-0.702346356621552));
#57144=CARTESIAN_POINT('Ctrl Pts',(3.77719254217129,1.,-0.705135847999817));
#57145=CARTESIAN_POINT('Ctrl Pts',(3.78402183336605,1.,-0.708015879375459));
#57146=CARTESIAN_POINT('Ctrl Pts',(3.79093694007094,1.,-0.710978231689017));
#57147=CARTESIAN_POINT('Ctrl Pts',(3.79788100314975,1.,-0.714010733006641));
#57148=CARTESIAN_POINT('Ctrl Pts',(3.80479445759309,1.,-0.717100993669115));
#57149=CARTESIAN_POINT('Ctrl Pts',(3.81163885127344,1.,-0.720240466589236));
#57150=CARTESIAN_POINT('Ctrl Pts',(3.81840802610835,1.,-0.723426346019423));
#57151=CARTESIAN_POINT('Ctrl Pts',(3.82511495756713,1.,-0.726659281876664));
#57152=CARTESIAN_POINT('Ctrl Pts',(3.83178392403383,1.,-0.729942010490168));
#57153=CARTESIAN_POINT('Ctrl Pts',(3.83844103658009,1.,-0.733277703756078));
#57154=CARTESIAN_POINT('Ctrl Pts',(3.84510432881213,1.,-0.736668240497118));
#57155=CARTESIAN_POINT('Ctrl Pts',(3.85177770351215,1.,-0.740113146827137));
#57156=CARTESIAN_POINT('Ctrl Pts',(3.85845645217594,1.,-0.743610542737013));
#57157=CARTESIAN_POINT('Ctrl Pts',(3.86513062969889,1.,-0.747157716488871));
#57158=CARTESIAN_POINT('Ctrl Pts',(3.87178914078374,1.,-0.750751822383028));
#57159=CARTESIAN_POINT('Ctrl Pts',(3.87842382520065,1.,-0.754390577396857));
#57160=CARTESIAN_POINT('Ctrl Pts',(3.88503262662689,1.,-0.758072800564801));
#57161=CARTESIAN_POINT('Ctrl Pts',(3.89161738162245,1.,-0.76179802879397));
#57162=CARTESIAN_POINT('Ctrl Pts',(3.89818233104378,1.,-0.765566256401296));
#57163=CARTESIAN_POINT('Ctrl Pts',(3.90473237182633,1.,-0.769377629847874));
#57164=CARTESIAN_POINT('Ctrl Pts',(3.91127138115243,1.,-0.773232154506321));
#57165=CARTESIAN_POINT('Ctrl Pts',(3.9178006233448,1.,-0.777129415664956));
#57166=CARTESIAN_POINT('Ctrl Pts',(3.92431956510441,1.,-0.781068718228451));
#57167=CARTESIAN_POINT('Ctrl Pts',(3.93082655631789,1.,-0.785049202786508));
#57168=CARTESIAN_POINT('Ctrl Pts',(3.93731956885676,1.,-0.789069971469333));
#57169=CARTESIAN_POINT('Ctrl Pts',(3.94379688971283,1.,-0.793130205640961));
#57170=CARTESIAN_POINT('Ctrl Pts',(3.95025788827136,1.,-0.797229296085316));
#57171=CARTESIAN_POINT('Ctrl Pts',(3.95670276375108,1.,-0.80136679772705));
#57172=CARTESIAN_POINT('Ctrl Pts',(3.96313222295815,1.,-0.805542372178362));
#57173=CARTESIAN_POINT('Ctrl Pts',(3.96954717513232,1.,-0.809755732818091));
#57174=CARTESIAN_POINT('Ctrl Pts',(3.97594844078811,1.,-0.814006592328844));
#57175=CARTESIAN_POINT('Ctrl Pts',(3.98233640155404,1.,-0.818294599022294));
#57176=CARTESIAN_POINT('Ctrl Pts',(3.98871104646485,1.,-0.822619346022119));
#57177=CARTESIAN_POINT('Ctrl Pts',(3.99507212784431,1.,-0.82698040032079));
#57178=CARTESIAN_POINT('Ctrl Pts',(4.00141928477507,1.,-0.831377325741623));
#57179=CARTESIAN_POINT('Ctrl Pts',(4.00775216907856,1.,-0.835809705809646));
#57180=CARTESIAN_POINT('Ctrl Pts',(4.01407059766103,1.,-0.840277171975855));
#57181=CARTESIAN_POINT('Ctrl Pts',(4.02037456798441,1.,-0.844779403287746));
#57182=CARTESIAN_POINT('Ctrl Pts',(4.02666418343164,1.,-0.849316107474245));
#57183=CARTESIAN_POINT('Ctrl Pts',(4.03293960436756,1.,-0.853887006631755));
#57184=CARTESIAN_POINT('Ctrl Pts',(4.03920099284773,1.,-0.858491822322828));
#57185=CARTESIAN_POINT('Ctrl Pts',(4.04544845048584,1.,-0.863130256643259));
#57186=CARTESIAN_POINT('Ctrl Pts',(4.05168199437909,1.,-0.867801988859918));
#57187=CARTESIAN_POINT('Ctrl Pts',(4.0579015903134,1.,-0.872506694782446));
#57188=CARTESIAN_POINT('Ctrl Pts',(4.06410717232905,1.,-0.877244060485838));
#57189=CARTESIAN_POINT('Ctrl Pts',(4.07029866694192,1.,-0.882013797525692));
#57190=CARTESIAN_POINT('Ctrl Pts',(4.07647601773635,1.,-0.886815658358501));
#57191=CARTESIAN_POINT('Ctrl Pts',(4.08263920304799,1.,-0.891649447916278));
#57192=CARTESIAN_POINT('Ctrl Pts',(4.08878822246833,1.,-0.896515019231334));
#57193=CARTESIAN_POINT('Ctrl Pts',(4.09369611522387,1.,-0.900432820941675));
#57194=CARTESIAN_POINT('Ctrl Pts',(4.09737067245935,1.,-0.903385402441588));
#57195=CARTESIAN_POINT('Ctrl Pts',(4.09981755067523,1.,-0.905360112215337));
#57196=CARTESIAN_POINT('Ctrl Pts',(4.10104028313088,1.,-0.906349047628866));
#57197=CARTESIAN_POINT('Origin',(0.,0.,0.));
#57198=CARTESIAN_POINT('',(3.71701050416802,1.,-0.496319364829374));
#57199=CARTESIAN_POINT('Origin',(0.,1.,0.));
#57200=CARTESIAN_POINT('Ctrl Pts',(3.71701050416802,1.,-0.496319364829374));
#57201=CARTESIAN_POINT('Ctrl Pts',(3.71701050416802,0.666666666666667,-0.496319364829374));
#57202=CARTESIAN_POINT('Ctrl Pts',(3.71701050416802,0.333333333333333,-0.496319364829374));
#57203=CARTESIAN_POINT('Ctrl Pts',(3.71701050416802,-0.333333333333333,
-0.496319364829374));
#57204=CARTESIAN_POINT('Ctrl Pts',(3.71701050416802,-0.666666666666667,
-0.496319364829374));
#57205=CARTESIAN_POINT('Ctrl Pts',(3.71701050416802,-1.,-0.496319364829374));
#57206=CARTESIAN_POINT('Ctrl Pts',(3.74888690736767,-1.,-0.0913616755937424));
#57207=CARTESIAN_POINT('Ctrl Pts',(3.74888690736767,1.,-0.0913616755937424));
#57208=CARTESIAN_POINT('Ctrl Pts',(3.74882632119067,-1.,-0.0912992005792589));
#57209=CARTESIAN_POINT('Ctrl Pts',(3.74882632119067,1.,-0.0912992005792589));
#57210=CARTESIAN_POINT('Ctrl Pts',(3.74887017174206,-1.,-0.0911958743735238));
#57211=CARTESIAN_POINT('Ctrl Pts',(3.74887017174206,1.,-0.0911958743735238));
#57212=CARTESIAN_POINT('Ctrl Pts',(3.74943097853811,-1.,-0.0911057547506604));
#57213=CARTESIAN_POINT('Ctrl Pts',(3.74943097853811,1.,-0.0911057547506604));
#57214=CARTESIAN_POINT('Ctrl Pts',(3.75116949194623,-1.,-0.0911154000998146));
#57215=CARTESIAN_POINT('Ctrl Pts',(3.75116949194623,1.,-0.0911154000998146));
#57216=CARTESIAN_POINT('Ctrl Pts',(3.75495560118212,-1.,-0.0913419622736402));
#57217=CARTESIAN_POINT('Ctrl Pts',(3.75495560118212,1.,-0.0913419622736402));
#57218=CARTESIAN_POINT('Ctrl Pts',(3.76024199359303,-1.,-0.0917773084998339));
#57219=CARTESIAN_POINT('Ctrl Pts',(3.76024199359303,1.,-0.0917773084998339));
#57220=CARTESIAN_POINT('Ctrl Pts',(3.76678860031841,-1.,-0.0924090589602695));
#57221=CARTESIAN_POINT('Ctrl Pts',(3.76678860031841,1.,-0.0924090589602695));
#57222=CARTESIAN_POINT('Ctrl Pts',(3.77424159971059,-1.,-0.0932185546203182));
#57223=CARTESIAN_POINT('Ctrl Pts',(3.77424159971059,1.,-0.0932185546203182));
#57224=CARTESIAN_POINT('Ctrl Pts',(3.782205218991,-1.,-0.0941840095090818));
#57225=CARTESIAN_POINT('Ctrl Pts',(3.782205218991,1.,-0.0941840095090818));
#57226=CARTESIAN_POINT('Ctrl Pts',(3.79030016353111,-1.,-0.0952829885100805));
#57227=CARTESIAN_POINT('Ctrl Pts',(3.79030016353111,1.,-0.0952829885100805));
#57228=CARTESIAN_POINT('Ctrl Pts',(3.79822128513845,-1.,-0.0964949352873135));
#57229=CARTESIAN_POINT('Ctrl Pts',(3.79822128513845,1.,-0.0964949352873135));
#57230=CARTESIAN_POINT('Ctrl Pts',(3.80581088847809,-1.,-0.0978042222906647));
#57231=CARTESIAN_POINT('Ctrl Pts',(3.80581088847809,1.,-0.0978042222906647));
#57232=CARTESIAN_POINT('Ctrl Pts',(3.81306649386461,-1.,-0.0992008728096518));
#57233=CARTESIAN_POINT('Ctrl Pts',(3.81306649386461,1.,-0.0992008728096518));
#57234=CARTESIAN_POINT('Ctrl Pts',(3.82007889742625,-1.,-0.100678769650632));
#57235=CARTESIAN_POINT('Ctrl Pts',(3.82007889742625,1.,-0.100678769650632));
#57236=CARTESIAN_POINT('Ctrl Pts',(3.82698737143255,-1.,-0.102234506488457));
#57237=CARTESIAN_POINT('Ctrl Pts',(3.82698737143255,1.,-0.102234506488457));
#57238=CARTESIAN_POINT('Ctrl Pts',(3.83393171228002,-1.,-0.103866063811623));
#57239=CARTESIAN_POINT('Ctrl Pts',(3.83393171228002,1.,-0.103866063811623));
#57240=CARTESIAN_POINT('Ctrl Pts',(3.84099658324803,-1.,-0.105571360916569));
#57241=CARTESIAN_POINT('Ctrl Pts',(3.84099658324803,1.,-0.105571360916569));
#57242=CARTESIAN_POINT('Ctrl Pts',(3.84819233070317,-1.,-0.107347597812184));
#57243=CARTESIAN_POINT('Ctrl Pts',(3.84819233070317,1.,-0.107347597812184));
#57244=CARTESIAN_POINT('Ctrl Pts',(3.855485714969,-1.,-0.109191717634944));
#57245=CARTESIAN_POINT('Ctrl Pts',(3.855485714969,1.,-0.109191717634944));
#57246=CARTESIAN_POINT('Ctrl Pts',(3.86281867282965,-1.,-0.111100593036261));
#57247=CARTESIAN_POINT('Ctrl Pts',(3.86281867282965,1.,-0.111100593036261));
#57248=CARTESIAN_POINT('Ctrl Pts',(3.87013043445014,-1.,-0.113071304914562));
#57249=CARTESIAN_POINT('Ctrl Pts',(3.87013043445014,1.,-0.113071304914562));
#57250=CARTESIAN_POINT('Ctrl Pts',(3.87738168405343,-1.,-0.11510142664947));
#57251=CARTESIAN_POINT('Ctrl Pts',(3.87738168405343,1.,-0.11510142664947));
#57252=CARTESIAN_POINT('Ctrl Pts',(3.88456590045767,-1.,-0.117189150373144));
#57253=CARTESIAN_POINT('Ctrl Pts',(3.88456590045767,1.,-0.117189150373144));
#57254=CARTESIAN_POINT('Ctrl Pts',(3.89169600105201,-1.,-0.119333088190418));
#57255=CARTESIAN_POINT('Ctrl Pts',(3.89169600105201,1.,-0.119333088190418));
#57256=CARTESIAN_POINT('Ctrl Pts',(3.89879639336952,-1.,-0.121532144765723));
#57257=CARTESIAN_POINT('Ctrl Pts',(3.89879639336952,1.,-0.121532144765723));
#57258=CARTESIAN_POINT('Ctrl Pts',(3.90589336320508,-1.,-0.123785368272378));
#57259=CARTESIAN_POINT('Ctrl Pts',(3.90589336320508,1.,-0.123785368272378));
#57260=CARTESIAN_POINT('Ctrl Pts',(3.91300501605392,-1.,-0.126091793324137));
#57261=CARTESIAN_POINT('Ctrl Pts',(3.91300501605392,1.,-0.126091793324137));
#57262=CARTESIAN_POINT('Ctrl Pts',(3.92013513251642,-1.,-0.128450341339528));
#57263=CARTESIAN_POINT('Ctrl Pts',(3.92013513251642,1.,-0.128450341339528));
#57264=CARTESIAN_POINT('Ctrl Pts',(3.9272787679596,-1.,-0.130859892027799));
#57265=CARTESIAN_POINT('Ctrl Pts',(3.9272787679596,1.,-0.130859892027799));
#57266=CARTESIAN_POINT('Ctrl Pts',(3.93442567551035,-1.,-0.13331932279419));
#57267=CARTESIAN_POINT('Ctrl Pts',(3.93442567551035,1.,-0.13331932279419));
#57268=CARTESIAN_POINT('Ctrl Pts',(3.94156445130744,-1.,-0.135827558661188));
#57269=CARTESIAN_POINT('Ctrl Pts',(3.94156445130744,1.,-0.135827558661188));
#57270=CARTESIAN_POINT('Ctrl Pts',(3.94868667844355,-1.,-0.138383621255159));
#57271=CARTESIAN_POINT('Ctrl Pts',(3.94868667844355,1.,-0.138383621255159));
#57272=CARTESIAN_POINT('Ctrl Pts',(3.95579014116899,-1.,-0.140986665829937));
#57273=CARTESIAN_POINT('Ctrl Pts',(3.95579014116899,1.,-0.140986665829937));
#57274=CARTESIAN_POINT('Ctrl Pts',(3.96287658098896,-1.,-0.143635947692791));
#57275=CARTESIAN_POINT('Ctrl Pts',(3.96287658098896,1.,-0.143635947692791));
#57276=CARTESIAN_POINT('Ctrl Pts',(3.96995018565891,-1.,-0.146330797814514));
#57277=CARTESIAN_POINT('Ctrl Pts',(3.96995018565891,1.,-0.146330797814514));
#57278=CARTESIAN_POINT('Ctrl Pts',(3.97701581473643,-1.,-0.149070594803544));
#57279=CARTESIAN_POINT('Ctrl Pts',(3.97701581473643,1.,-0.149070594803544));
#57280=CARTESIAN_POINT('Ctrl Pts',(3.9840772985098,-1.,-0.151854737441406));
#57281=CARTESIAN_POINT('Ctrl Pts',(3.9840772985098,1.,-0.151854737441406));
#57282=CARTESIAN_POINT('Ctrl Pts',(3.99113582086059,-1.,-0.154682618338563));
#57283=CARTESIAN_POINT('Ctrl Pts',(3.99113582086059,1.,-0.154682618338563));
#57284=CARTESIAN_POINT('Ctrl Pts',(3.99819074631874,-1.,-0.15755363438381));
#57285=CARTESIAN_POINT('Ctrl Pts',(3.99819074631874,1.,-0.15755363438381));
#57286=CARTESIAN_POINT('Ctrl Pts',(4.00524031064509,-1.,-0.160467194882219));
#57287=CARTESIAN_POINT('Ctrl Pts',(4.00524031064509,1.,-0.160467194882219));
#57288=CARTESIAN_POINT('Ctrl Pts',(4.01228237022301,-1.,-0.163422730287459));
#57289=CARTESIAN_POINT('Ctrl Pts',(4.01228237022301,1.,-0.163422730287459));
#57290=CARTESIAN_POINT('Ctrl Pts',(4.01931510507143,-1.,-0.166419700015848));
#57291=CARTESIAN_POINT('Ctrl Pts',(4.01931510507143,1.,-0.166419700015848));
#57292=CARTESIAN_POINT('Ctrl Pts',(4.0263377970371,-1.,-0.169457601001653));
#57293=CARTESIAN_POINT('Ctrl Pts',(4.0263377970371,1.,-0.169457601001653));
#57294=CARTESIAN_POINT('Ctrl Pts',(4.03335057326093,-1.,-0.172535962484467));
#57295=CARTESIAN_POINT('Ctrl Pts',(4.03335057326093,1.,-0.172535962484467));
#57296=CARTESIAN_POINT('Ctrl Pts',(4.04035407891161,-1.,-0.175654339673758));
#57297=CARTESIAN_POINT('Ctrl Pts',(4.04035407891161,1.,-0.175654339673758));
#57298=CARTESIAN_POINT('Ctrl Pts',(4.04734916719722,-1.,-0.178812307240716));
#57299=CARTESIAN_POINT('Ctrl Pts',(4.04734916719722,1.,-0.178812307240716));
#57300=CARTESIAN_POINT('Ctrl Pts',(4.05433660358402,-1.,-0.18200945304855));
#57301=CARTESIAN_POINT('Ctrl Pts',(4.05433660358402,1.,-0.18200945304855));
#57302=CARTESIAN_POINT('Ctrl Pts',(4.06131670998589,-1.,-0.185245370038948));
#57303=CARTESIAN_POINT('Ctrl Pts',(4.06131670998589,1.,-0.185245370038948));
#57304=CARTESIAN_POINT('Ctrl Pts',(4.06828941192308,-1.,-0.188519658060256));
#57305=CARTESIAN_POINT('Ctrl Pts',(4.06828941192308,1.,-0.188519658060256));
#57306=CARTESIAN_POINT('Ctrl Pts',(4.07525439703137,-1.,-0.191831928181081));
#57307=CARTESIAN_POINT('Ctrl Pts',(4.07525439703137,1.,-0.191831928181081));
#57308=CARTESIAN_POINT('Ctrl Pts',(4.08221124060385,-1.,-0.195181806054714));
#57309=CARTESIAN_POINT('Ctrl Pts',(4.08221124060385,1.,-0.195181806054714));
#57310=CARTESIAN_POINT('Ctrl Pts',(4.08915953359753,-1.,-0.198568934800811));
#57311=CARTESIAN_POINT('Ctrl Pts',(4.08915953359753,1.,-0.198568934800811));
#57312=CARTESIAN_POINT('Ctrl Pts',(4.09609903751912,-1.,-0.201992979049985));
#57313=CARTESIAN_POINT('Ctrl Pts',(4.09609903751912,1.,-0.201992979049985));
#57314=CARTESIAN_POINT('Ctrl Pts',(4.10302969965374,-1.,-0.205453622198233));
#57315=CARTESIAN_POINT('Ctrl Pts',(4.10302969965374,1.,-0.205453622198233));
#57316=CARTESIAN_POINT('Ctrl Pts',(4.10995157639026,-1.,-0.208950559400172));
#57317=CARTESIAN_POINT('Ctrl Pts',(4.10995157639026,1.,-0.208950559400172));
#57318=CARTESIAN_POINT('Ctrl Pts',(4.11686478264545,-1.,-0.212483491087068));
#57319=CARTESIAN_POINT('Ctrl Pts',(4.11686478264545,1.,-0.212483491087068));
#57320=CARTESIAN_POINT('Ctrl Pts',(4.12376943492249,-1.,-0.216052116898425));
#57321=CARTESIAN_POINT('Ctrl Pts',(4.12376943492249,1.,-0.216052116898425));
#57322=CARTESIAN_POINT('Ctrl Pts',(4.13066558698156,-1.,-0.219656126701852));
#57323=CARTESIAN_POINT('Ctrl Pts',(4.13066558698156,1.,-0.219656126701852));
#57324=CARTESIAN_POINT('Ctrl Pts',(4.13755320553563,-1.,-0.223295201038384));
#57325=CARTESIAN_POINT('Ctrl Pts',(4.13755320553563,1.,-0.223295201038384));
#57326=CARTESIAN_POINT('Ctrl Pts',(4.14443220607733,-1.,-0.226969025061244));
#57327=CARTESIAN_POINT('Ctrl Pts',(4.14443220607733,1.,-0.226969025061244));
#57328=CARTESIAN_POINT('Ctrl Pts',(4.15130247435029,-1.,-0.230677299028738));
#57329=CARTESIAN_POINT('Ctrl Pts',(4.15130247435029,1.,-0.230677299028738));
#57330=CARTESIAN_POINT('Ctrl Pts',(4.1581638926525,-1.,-0.234419749543143));
#57331=CARTESIAN_POINT('Ctrl Pts',(4.1581638926525,1.,-0.234419749543143));
#57332=CARTESIAN_POINT('Ctrl Pts',(4.1650163665385,-1.,-0.238196140933977));
#57333=CARTESIAN_POINT('Ctrl Pts',(4.1650163665385,1.,-0.238196140933977));
#57334=CARTESIAN_POINT('Ctrl Pts',(4.17185984409533,-1.,-0.242006283923912));
#57335=CARTESIAN_POINT('Ctrl Pts',(4.17185984409533,1.,-0.242006283923912));
#57336=CARTESIAN_POINT('Ctrl Pts',(4.17869430192868,-1.,-0.245850033418584));
#57337=CARTESIAN_POINT('Ctrl Pts',(4.17869430192868,1.,-0.245850033418584));
#57338=CARTESIAN_POINT('Ctrl Pts',(4.18415464959491,-1.,-0.248951836910964));
#57339=CARTESIAN_POINT('Ctrl Pts',(4.18415464959491,1.,-0.248951836910964));
#57340=CARTESIAN_POINT('Ctrl Pts',(4.18824585244066,-1.,-0.251293239837693));
#57341=CARTESIAN_POINT('Ctrl Pts',(4.18824585244066,1.,-0.251293239837693));
#57342=CARTESIAN_POINT('Ctrl Pts',(4.19097151819241,-1.,-0.252860861572566));
#57343=CARTESIAN_POINT('Ctrl Pts',(4.19097151819241,1.,-0.252860861572566));
#57344=CARTESIAN_POINT('Ctrl Pts',(4.1923339003649,-1.,-0.253646344052521));
#57345=CARTESIAN_POINT('Ctrl Pts',(4.1923339003649,1.,-0.253646344052521));
#57346=CARTESIAN_POINT('',(3.74888939116255,1.,-0.0912596999166826));
#57347=CARTESIAN_POINT('Ctrl Pts',(3.74888939116255,-1.,-0.0912596999166829));
#57348=CARTESIAN_POINT('Ctrl Pts',(3.74888939116255,-0.666666666666667,
-0.0912596999166829));
#57349=CARTESIAN_POINT('Ctrl Pts',(3.74888939116255,-0.333333333333333,
-0.0912596999166829));
#57350=CARTESIAN_POINT('Ctrl Pts',(3.74888939116255,0.333333333333333,-0.0912596999166829));
#57351=CARTESIAN_POINT('Ctrl Pts',(3.74888939116255,0.666666666666667,-0.0912596999166829));
#57352=CARTESIAN_POINT('Ctrl Pts',(3.74888939116255,1.,-0.0912596999166829));
#57353=CARTESIAN_POINT('',(4.1923339003649,1.,-0.253646344052521));
#57354=CARTESIAN_POINT('',(4.1923339003649,0.,-0.253646344052521));
#57355=CARTESIAN_POINT('Ctrl Pts',(3.74888939116255,1.,-0.0912596999166826));
#57356=CARTESIAN_POINT('Ctrl Pts',(3.74892890040974,1.,-0.0912308016421984));
#57357=CARTESIAN_POINT('Ctrl Pts',(3.74911539914542,1.,-0.0911666301812821));
#57358=CARTESIAN_POINT('Ctrl Pts',(3.74976844886346,1.,-0.0911090736805514));
#57359=CARTESIAN_POINT('Ctrl Pts',(3.75145357872422,1.,-0.091132399957443));
#57360=CARTESIAN_POINT('Ctrl Pts',(3.75495560118212,1.,-0.0913419622736402));
#57361=CARTESIAN_POINT('Ctrl Pts',(3.76024199359303,1.,-0.0917773084998339));
#57362=CARTESIAN_POINT('Ctrl Pts',(3.76678860031841,1.,-0.0924090589602695));
#57363=CARTESIAN_POINT('Ctrl Pts',(3.77424159971059,1.,-0.0932185546203182));
#57364=CARTESIAN_POINT('Ctrl Pts',(3.782205218991,1.,-0.0941840095090818));
#57365=CARTESIAN_POINT('Ctrl Pts',(3.79030016353111,1.,-0.0952829885100805));
#57366=CARTESIAN_POINT('Ctrl Pts',(3.79822128513845,1.,-0.0964949352873135));
#57367=CARTESIAN_POINT('Ctrl Pts',(3.80581088847809,1.,-0.0978042222906647));
#57368=CARTESIAN_POINT('Ctrl Pts',(3.81306649386461,1.,-0.0992008728096518));
#57369=CARTESIAN_POINT('Ctrl Pts',(3.82007889742625,1.,-0.100678769650632));
#57370=CARTESIAN_POINT('Ctrl Pts',(3.82698737143255,1.,-0.102234506488457));
#57371=CARTESIAN_POINT('Ctrl Pts',(3.83393171228002,1.,-0.103866063811623));
#57372=CARTESIAN_POINT('Ctrl Pts',(3.84099658324803,1.,-0.105571360916569));
#57373=CARTESIAN_POINT('Ctrl Pts',(3.84819233070317,1.,-0.107347597812184));
#57374=CARTESIAN_POINT('Ctrl Pts',(3.855485714969,1.,-0.109191717634944));
#57375=CARTESIAN_POINT('Ctrl Pts',(3.86281867282965,1.,-0.111100593036261));
#57376=CARTESIAN_POINT('Ctrl Pts',(3.87013043445014,1.,-0.113071304914562));
#57377=CARTESIAN_POINT('Ctrl Pts',(3.87738168405343,1.,-0.11510142664947));
#57378=CARTESIAN_POINT('Ctrl Pts',(3.88456590045767,1.,-0.117189150373144));
#57379=CARTESIAN_POINT('Ctrl Pts',(3.89169600105201,1.,-0.119333088190418));
#57380=CARTESIAN_POINT('Ctrl Pts',(3.89879639336952,1.,-0.121532144765723));
#57381=CARTESIAN_POINT('Ctrl Pts',(3.90589336320508,1.,-0.123785368272378));
#57382=CARTESIAN_POINT('Ctrl Pts',(3.91300501605392,1.,-0.126091793324137));
#57383=CARTESIAN_POINT('Ctrl Pts',(3.92013513251642,1.,-0.128450341339528));
#57384=CARTESIAN_POINT('Ctrl Pts',(3.9272787679596,1.,-0.130859892027799));
#57385=CARTESIAN_POINT('Ctrl Pts',(3.93442567551035,1.,-0.13331932279419));
#57386=CARTESIAN_POINT('Ctrl Pts',(3.94156445130744,1.,-0.135827558661188));
#57387=CARTESIAN_POINT('Ctrl Pts',(3.94868667844355,1.,-0.138383621255159));
#57388=CARTESIAN_POINT('Ctrl Pts',(3.95579014116899,1.,-0.140986665829937));
#57389=CARTESIAN_POINT('Ctrl Pts',(3.96287658098896,1.,-0.143635947692791));
#57390=CARTESIAN_POINT('Ctrl Pts',(3.96995018565891,1.,-0.146330797814514));
#57391=CARTESIAN_POINT('Ctrl Pts',(3.97701581473643,1.,-0.149070594803544));
#57392=CARTESIAN_POINT('Ctrl Pts',(3.9840772985098,1.,-0.151854737441406));
#57393=CARTESIAN_POINT('Ctrl Pts',(3.99113582086059,1.,-0.154682618338563));
#57394=CARTESIAN_POINT('Ctrl Pts',(3.99819074631874,1.,-0.15755363438381));
#57395=CARTESIAN_POINT('Ctrl Pts',(4.00524031064509,1.,-0.160467194882219));
#57396=CARTESIAN_POINT('Ctrl Pts',(4.01228237022301,1.,-0.163422730287459));
#57397=CARTESIAN_POINT('Ctrl Pts',(4.01931510507143,1.,-0.166419700015848));
#57398=CARTESIAN_POINT('Ctrl Pts',(4.0263377970371,1.,-0.169457601001653));
#57399=CARTESIAN_POINT('Ctrl Pts',(4.03335057326093,1.,-0.172535962484467));
#57400=CARTESIAN_POINT('Ctrl Pts',(4.04035407891161,1.,-0.175654339673758));
#57401=CARTESIAN_POINT('Ctrl Pts',(4.04734916719722,1.,-0.178812307240716));
#57402=CARTESIAN_POINT('Ctrl Pts',(4.05433660358402,1.,-0.18200945304855));
#57403=CARTESIAN_POINT('Ctrl Pts',(4.06131670998589,1.,-0.185245370038948));
#57404=CARTESIAN_POINT('Ctrl Pts',(4.06828941192308,1.,-0.188519658060256));
#57405=CARTESIAN_POINT('Ctrl Pts',(4.07525439703137,1.,-0.191831928181081));
#57406=CARTESIAN_POINT('Ctrl Pts',(4.08221124060385,1.,-0.195181806054714));
#57407=CARTESIAN_POINT('Ctrl Pts',(4.08915953359753,1.,-0.198568934800811));
#57408=CARTESIAN_POINT('Ctrl Pts',(4.09609903751912,1.,-0.201992979049985));
#57409=CARTESIAN_POINT('Ctrl Pts',(4.10302969965374,1.,-0.205453622198233));
#57410=CARTESIAN_POINT('Ctrl Pts',(4.10995157639026,1.,-0.208950559400172));
#57411=CARTESIAN_POINT('Ctrl Pts',(4.11686478264545,1.,-0.212483491087068));
#57412=CARTESIAN_POINT('Ctrl Pts',(4.12376943492249,1.,-0.216052116898425));
#57413=CARTESIAN_POINT('Ctrl Pts',(4.13066558698156,1.,-0.219656126701852));
#57414=CARTESIAN_POINT('Ctrl Pts',(4.13755320553563,1.,-0.223295201038384));
#57415=CARTESIAN_POINT('Ctrl Pts',(4.14443220607733,1.,-0.226969025061244));
#57416=CARTESIAN_POINT('Ctrl Pts',(4.15130247435029,1.,-0.230677299028738));
#57417=CARTESIAN_POINT('Ctrl Pts',(4.1581638926525,1.,-0.234419749543143));
#57418=CARTESIAN_POINT('Ctrl Pts',(4.1650163665385,1.,-0.238196140933977));
#57419=CARTESIAN_POINT('Ctrl Pts',(4.17185984409533,1.,-0.242006283923912));
#57420=CARTESIAN_POINT('Ctrl Pts',(4.17869430192868,1.,-0.245850033418584));
#57421=CARTESIAN_POINT('Ctrl Pts',(4.18415464959491,1.,-0.248951836910964));
#57422=CARTESIAN_POINT('Ctrl Pts',(4.18824585244066,1.,-0.251293239837693));
#57423=CARTESIAN_POINT('Ctrl Pts',(4.19097151819241,1.,-0.252860861572566));
#57424=CARTESIAN_POINT('Ctrl Pts',(4.1923339003649,1.,-0.253646344052521));
#57425=CARTESIAN_POINT('Ctrl Pts',(4.18039834341342,-1.,-0.40530197431835));
#57426=CARTESIAN_POINT('Ctrl Pts',(4.18039834341342,1.,-0.40530197431835));
#57427=CARTESIAN_POINT('Ctrl Pts',(4.17892985789908,-1.,-0.405864662679631));
#57428=CARTESIAN_POINT('Ctrl Pts',(4.17892985789908,1.,-0.405864662679631));
#57429=CARTESIAN_POINT('Ctrl Pts',(4.17599251955585,-1.,-0.406986596326603));
#57430=CARTESIAN_POINT('Ctrl Pts',(4.17599251955585,1.,-0.406986596326603));
#57431=CARTESIAN_POINT('Ctrl Pts',(4.17158541009947,-1.,-0.408659167570153));
#57432=CARTESIAN_POINT('Ctrl Pts',(4.17158541009947,1.,-0.408659167570153));
#57433=CARTESIAN_POINT('Ctrl Pts',(4.16570705940731,-1.,-0.410868596148614));
#57434=CARTESIAN_POINT('Ctrl Pts',(4.16570705940731,1.,-0.410868596148614));
#57435=CARTESIAN_POINT('Ctrl Pts',(4.1583554501909,-1.,-0.413595877953269));
#57436=CARTESIAN_POINT('Ctrl Pts',(4.1583554501909,1.,-0.413595877953269));
#57437=CARTESIAN_POINT('Ctrl Pts',(4.15100018950989,-1.,-0.416288556008986));
#57438=CARTESIAN_POINT('Ctrl Pts',(4.15100018950989,1.,-0.416288556008986));
#57439=CARTESIAN_POINT('Ctrl Pts',(4.14364132317223,-1.,-0.4189464906678));
#57440=CARTESIAN_POINT('Ctrl Pts',(4.14364132317223,1.,-0.4189464906678));
#57441=CARTESIAN_POINT('Ctrl Pts',(4.13627893206433,-1.,-0.421569503103971));
#57442=CARTESIAN_POINT('Ctrl Pts',(4.13627893206433,1.,-0.421569503103971));
#57443=CARTESIAN_POINT('Ctrl Pts',(4.1289131463371,-1.,-0.424157375323155));
#57444=CARTESIAN_POINT('Ctrl Pts',(4.1289131463371,1.,-0.424157375323155));
#57445=CARTESIAN_POINT('Ctrl Pts',(4.1215441250121,-1.,-0.426709855706243));
#57446=CARTESIAN_POINT('Ctrl Pts',(4.1215441250121,1.,-0.426709855706243));
#57447=CARTESIAN_POINT('Ctrl Pts',(4.1141720278277,-1.,-0.429226666075373));
#57448=CARTESIAN_POINT('Ctrl Pts',(4.1141720278277,1.,-0.429226666075373));
#57449=CARTESIAN_POINT('Ctrl Pts',(4.10679698750219,-1.,-0.431707508679772));
#57450=CARTESIAN_POINT('Ctrl Pts',(4.10679698750219,1.,-0.431707508679772));
#57451=CARTESIAN_POINT('Ctrl Pts',(4.09941908688567,-1.,-0.434152073200643));
#57452=CARTESIAN_POINT('Ctrl Pts',(4.09941908688567,1.,-0.434152073200643));
#57453=CARTESIAN_POINT('Ctrl Pts',(4.09203832139439,-1.,-0.436560044913814));
#57454=CARTESIAN_POINT('Ctrl Pts',(4.09203832139439,1.,-0.436560044913814));
#57455=CARTESIAN_POINT('Ctrl Pts',(4.08465462294625,-1.,-0.438931108931614));
#57456=CARTESIAN_POINT('Ctrl Pts',(4.08465462294625,1.,-0.438931108931614));
#57457=CARTESIAN_POINT('Ctrl Pts',(4.07726792490256,-1.,-0.441264951396587));
#57458=CARTESIAN_POINT('Ctrl Pts',(4.07726792490256,1.,-0.441264951396587));
#57459=CARTESIAN_POINT('Ctrl Pts',(4.0698782192577,-1.,-0.443561262395408));
#57460=CARTESIAN_POINT('Ctrl Pts',(4.0698782192577,1.,-0.443561262395408));
#57461=CARTESIAN_POINT('Ctrl Pts',(4.06248560760596,-1.,-0.445819737468478));
#57462=CARTESIAN_POINT('Ctrl Pts',(4.06248560760596,1.,-0.445819737468478));
#57463=CARTESIAN_POINT('Ctrl Pts',(4.05509037796815,-1.,-0.448040082683977));
#57464=CARTESIAN_POINT('Ctrl Pts',(4.05509037796815,1.,-0.448040082683977));
#57465=CARTESIAN_POINT('Ctrl Pts',(4.0476929901797,-1.,-0.450222009543774));
#57466=CARTESIAN_POINT('Ctrl Pts',(4.0476929901797,1.,-0.450222009543774));
#57467=CARTESIAN_POINT('Ctrl Pts',(4.0402939222793,-1.,-0.452365214748779));
#57468=CARTESIAN_POINT('Ctrl Pts',(4.0402939222793,1.,-0.452365214748779));
#57469=CARTESIAN_POINT('Ctrl Pts',(4.03289354362745,-1.,-0.454469363020496));
#57470=CARTESIAN_POINT('Ctrl Pts',(4.03289354362745,1.,-0.454469363020496));
#57471=CARTESIAN_POINT('Ctrl Pts',(4.02549199038414,-1.,-0.456534070784968));
#57472=CARTESIAN_POINT('Ctrl Pts',(4.02549199038414,1.,-0.456534070784968));
#57473=CARTESIAN_POINT('Ctrl Pts',(4.01808900827647,-1.,-0.458558885637001));
#57474=CARTESIAN_POINT('Ctrl Pts',(4.01808900827647,1.,-0.458558885637001));
#57475=CARTESIAN_POINT('Ctrl Pts',(4.01068390573469,-1.,-0.460543280768577));
#57476=CARTESIAN_POINT('Ctrl Pts',(4.01068390573469,1.,-0.460543280768577));
#57477=CARTESIAN_POINT('Ctrl Pts',(4.00327590659129,-1.,-0.462486702616252));
#57478=CARTESIAN_POINT('Ctrl Pts',(4.00327590659129,1.,-0.462486702616252));
#57479=CARTESIAN_POINT('Ctrl Pts',(3.99586444320134,-1.,-0.464388610938995));
#57480=CARTESIAN_POINT('Ctrl Pts',(3.99586444320134,1.,-0.464388610938995));
#57481=CARTESIAN_POINT('Ctrl Pts',(3.98844946363258,-1.,-0.466248520883035));
#57482=CARTESIAN_POINT('Ctrl Pts',(3.98844946363258,1.,-0.466248520883035));
#57483=CARTESIAN_POINT('Ctrl Pts',(3.98103175589349,-1.,-0.46806604792014));
#57484=CARTESIAN_POINT('Ctrl Pts',(3.98103175589349,1.,-0.46806604792014));
#57485=CARTESIAN_POINT('Ctrl Pts',(3.97361320212413,-1.,-0.469840942829878));
#57486=CARTESIAN_POINT('Ctrl Pts',(3.97361320212413,1.,-0.469840942829878));
#57487=CARTESIAN_POINT('Ctrl Pts',(3.96619600864626,-1.,-0.471572978413494));
#57488=CARTESIAN_POINT('Ctrl Pts',(3.96619600864626,1.,-0.471572978413494));
#57489=CARTESIAN_POINT('Ctrl Pts',(3.95878201038332,-1.,-0.473261847236296));
#57490=CARTESIAN_POINT('Ctrl Pts',(3.95878201038332,1.,-0.473261847236296));
#57491=CARTESIAN_POINT('Ctrl Pts',(3.95137192932898,-1.,-0.474907053021791));
#57492=CARTESIAN_POINT('Ctrl Pts',(3.95137192932898,1.,-0.474907053021791));
#57493=CARTESIAN_POINT('Ctrl Pts',(3.94396469119385,-1.,-0.476507810658535));
#57494=CARTESIAN_POINT('Ctrl Pts',(3.94396469119385,1.,-0.476507810658535));
#57495=CARTESIAN_POINT('Ctrl Pts',(3.93655660689819,-1.,-0.478062927140957));
#57496=CARTESIAN_POINT('Ctrl Pts',(3.93655660689819,1.,-0.478062927140957));
#57497=CARTESIAN_POINT('Ctrl Pts',(3.92914297392067,-1.,-0.479571028525566));
#57498=CARTESIAN_POINT('Ctrl Pts',(3.92914297392067,1.,-0.479571028525566));
#57499=CARTESIAN_POINT('Ctrl Pts',(3.92171976072334,-1.,-0.481030798910735));
#57500=CARTESIAN_POINT('Ctrl Pts',(3.92171976072334,1.,-0.481030798910735));
#57501=CARTESIAN_POINT('Ctrl Pts',(3.91428536373749,-1.,-0.482441230340709));
#57502=CARTESIAN_POINT('Ctrl Pts',(3.91428536373749,1.,-0.482441230340709));
#57503=CARTESIAN_POINT('Ctrl Pts',(3.90684210358063,-1.,-0.483801835089161));
#57504=CARTESIAN_POINT('Ctrl Pts',(3.90684210358063,1.,-0.483801835089161));
#57505=CARTESIAN_POINT('Ctrl Pts',(3.89939844658529,-1.,-0.485112963522246));
#57506=CARTESIAN_POINT('Ctrl Pts',(3.89939844658529,1.,-0.485112963522246));
#57507=CARTESIAN_POINT('Ctrl Pts',(3.89196582437574,-1.,-0.486375337854134));
#57508=CARTESIAN_POINT('Ctrl Pts',(3.89196582437574,1.,-0.486375337854134));
#57509=CARTESIAN_POINT('Ctrl Pts',(3.88455453328156,-1.,-0.487589452275179));
#57510=CARTESIAN_POINT('Ctrl Pts',(3.88455453328156,1.,-0.487589452275179));
#57511=CARTESIAN_POINT('Ctrl Pts',(3.87716963231115,-1.,-0.488754973798281));
#57512=CARTESIAN_POINT('Ctrl Pts',(3.87716963231115,1.,-0.488754973798281));
#57513=CARTESIAN_POINT('Ctrl Pts',(3.86980755613694,-1.,-0.4898702457049));
#57514=CARTESIAN_POINT('Ctrl Pts',(3.86980755613694,1.,-0.4898702457049));
#57515=CARTESIAN_POINT('Ctrl Pts',(3.86245057319215,-1.,-0.490931482170849));
#57516=CARTESIAN_POINT('Ctrl Pts',(3.86245057319215,1.,-0.490931482170849));
#57517=CARTESIAN_POINT('Ctrl Pts',(3.85507287020223,-1.,-0.49193363108376));
#57518=CARTESIAN_POINT('Ctrl Pts',(3.85507287020223,1.,-0.49193363108376));
#57519=CARTESIAN_POINT('Ctrl Pts',(3.84765051147965,-1.,-0.492871792414095));
#57520=CARTESIAN_POINT('Ctrl Pts',(3.84765051147965,1.,-0.492871792414095));
#57521=CARTESIAN_POINT('Ctrl Pts',(3.84017095578438,-1.,-0.493742574629117));
#57522=CARTESIAN_POINT('Ctrl Pts',(3.84017095578438,1.,-0.493742574629117));
#57523=CARTESIAN_POINT('Ctrl Pts',(3.8326409268245,-1.,-0.494545212256426));
#57524=CARTESIAN_POINT('Ctrl Pts',(3.8326409268245,1.,-0.494545212256426));
#57525=CARTESIAN_POINT('Ctrl Pts',(3.82509963594156,-1.,-0.495283458893903));
#57526=CARTESIAN_POINT('Ctrl Pts',(3.82509963594156,1.,-0.495283458893903));
#57527=CARTESIAN_POINT('Ctrl Pts',(3.81760756144099,-1.,-0.495963937875572));
#57528=CARTESIAN_POINT('Ctrl Pts',(3.81760756144099,1.,-0.495963937875572));
#57529=CARTESIAN_POINT('Ctrl Pts',(3.81022254090909,-1.,-0.496592643443789));
#57530=CARTESIAN_POINT('Ctrl Pts',(3.81022254090909,1.,-0.496592643443789));
#57531=CARTESIAN_POINT('Ctrl Pts',(3.80297788298545,-1.,-0.497171756201091));
#57532=CARTESIAN_POINT('Ctrl Pts',(3.80297788298545,1.,-0.497171756201091));
#57533=CARTESIAN_POINT('Ctrl Pts',(3.79586380669959,-1.,-0.497696892100581));
#57534=CARTESIAN_POINT('Ctrl Pts',(3.79586380669959,1.,-0.497696892100581));
#57535=CARTESIAN_POINT('Ctrl Pts',(3.78879701661152,-1.,-0.498152751800819));
#57536=CARTESIAN_POINT('Ctrl Pts',(3.78879701661152,1.,-0.498152751800819));
#57537=CARTESIAN_POINT('Ctrl Pts',(3.78163975337189,-1.,-0.498515471679379));
#57538=CARTESIAN_POINT('Ctrl Pts',(3.78163975337189,1.,-0.498515471679379));
#57539=CARTESIAN_POINT('Ctrl Pts',(3.77425499225089,-1.,-0.498759900365687));
#57540=CARTESIAN_POINT('Ctrl Pts',(3.77425499225089,1.,-0.498759900365687));
#57541=CARTESIAN_POINT('Ctrl Pts',(3.76655401191144,-1.,-0.498865792335185));
#57542=CARTESIAN_POINT('Ctrl Pts',(3.76655401191144,1.,-0.498865792335185));
#57543=CARTESIAN_POINT('Ctrl Pts',(3.75854082221127,-1.,-0.498823681615513));
#57544=CARTESIAN_POINT('Ctrl Pts',(3.75854082221127,1.,-0.498823681615513));
#57545=CARTESIAN_POINT('Ctrl Pts',(3.75037362168103,-1.,-0.498642802042929));
#57546=CARTESIAN_POINT('Ctrl Pts',(3.75037362168103,1.,-0.498642802042929));
#57547=CARTESIAN_POINT('Ctrl Pts',(3.74235701735109,-1.,-0.498350586058176));
#57548=CARTESIAN_POINT('Ctrl Pts',(3.74235701735109,1.,-0.498350586058176));
#57549=CARTESIAN_POINT('Ctrl Pts',(3.73486914372834,-1.,-0.497984209510496));
#57550=CARTESIAN_POINT('Ctrl Pts',(3.73486914372834,1.,-0.497984209510496));
#57551=CARTESIAN_POINT('Ctrl Pts',(3.72830430904794,-1.,-0.49758406715328));
#57552=CARTESIAN_POINT('Ctrl Pts',(3.72830430904794,1.,-0.49758406715328));
#57553=CARTESIAN_POINT('Ctrl Pts',(3.72301489774241,-1.,-0.497187079575795));
#57554=CARTESIAN_POINT('Ctrl Pts',(3.72301489774241,1.,-0.497187079575795));
#57555=CARTESIAN_POINT('Ctrl Pts',(3.71923995965807,-1.,-0.496818574419989));
#57556=CARTESIAN_POINT('Ctrl Pts',(3.71923995965807,1.,-0.496818574419989));
#57557=CARTESIAN_POINT('Ctrl Pts',(3.71752134136931,-1.,-0.496556137603856));
#57558=CARTESIAN_POINT('Ctrl Pts',(3.71752134136931,1.,-0.496556137603856));
#57559=CARTESIAN_POINT('Ctrl Pts',(3.71698153685229,-1.,-0.496379397992182));
#57560=CARTESIAN_POINT('Ctrl Pts',(3.71698153685229,1.,-0.496379397992182));
#57561=CARTESIAN_POINT('Ctrl Pts',(3.71695438995598,-1.,-0.496270484166233));
#57562=CARTESIAN_POINT('Ctrl Pts',(3.71695438995598,1.,-0.496270484166233));
#57563=CARTESIAN_POINT('Ctrl Pts',(3.71702400346349,-1.,-0.496218256089212));
#57564=CARTESIAN_POINT('Ctrl Pts',(3.71702400346349,1.,-0.496218256089212));
#57565=CARTESIAN_POINT('',(4.18039834341342,1.,-0.40530197431835));
#57566=CARTESIAN_POINT('Ctrl Pts',(4.18039834341342,1.,-0.40530197431835));
#57567=CARTESIAN_POINT('Ctrl Pts',(4.17892985789908,1.,-0.405864662679631));
#57568=CARTESIAN_POINT('Ctrl Pts',(4.17599251955585,1.,-0.406986596326603));
#57569=CARTESIAN_POINT('Ctrl Pts',(4.17158541009947,1.,-0.408659167570153));
#57570=CARTESIAN_POINT('Ctrl Pts',(4.16570705940731,1.,-0.410868596148614));
#57571=CARTESIAN_POINT('Ctrl Pts',(4.1583554501909,1.,-0.413595877953269));
#57572=CARTESIAN_POINT('Ctrl Pts',(4.15100018950989,1.,-0.416288556008986));
#57573=CARTESIAN_POINT('Ctrl Pts',(4.14364132317223,1.,-0.4189464906678));
#57574=CARTESIAN_POINT('Ctrl Pts',(4.13627893206433,1.,-0.421569503103971));
#57575=CARTESIAN_POINT('Ctrl Pts',(4.1289131463371,1.,-0.424157375323155));
#57576=CARTESIAN_POINT('Ctrl Pts',(4.1215441250121,1.,-0.426709855706243));
#57577=CARTESIAN_POINT('Ctrl Pts',(4.1141720278277,1.,-0.429226666075373));
#57578=CARTESIAN_POINT('Ctrl Pts',(4.10679698750219,1.,-0.431707508679772));
#57579=CARTESIAN_POINT('Ctrl Pts',(4.09941908688567,1.,-0.434152073200643));
#57580=CARTESIAN_POINT('Ctrl Pts',(4.09203832139439,1.,-0.436560044913814));
#57581=CARTESIAN_POINT('Ctrl Pts',(4.08465462294625,1.,-0.438931108931614));
#57582=CARTESIAN_POINT('Ctrl Pts',(4.07726792490256,1.,-0.441264951396587));
#57583=CARTESIAN_POINT('Ctrl Pts',(4.0698782192577,1.,-0.443561262395408));
#57584=CARTESIAN_POINT('Ctrl Pts',(4.06248560760596,1.,-0.445819737468478));
#57585=CARTESIAN_POINT('Ctrl Pts',(4.05509037796815,1.,-0.448040082683977));
#57586=CARTESIAN_POINT('Ctrl Pts',(4.0476929901797,1.,-0.450222009543774));
#57587=CARTESIAN_POINT('Ctrl Pts',(4.0402939222793,1.,-0.452365214748779));
#57588=CARTESIAN_POINT('Ctrl Pts',(4.03289354362745,1.,-0.454469363020496));
#57589=CARTESIAN_POINT('Ctrl Pts',(4.02549199038414,1.,-0.456534070784968));
#57590=CARTESIAN_POINT('Ctrl Pts',(4.01808900827647,1.,-0.458558885637001));
#57591=CARTESIAN_POINT('Ctrl Pts',(4.01068390573469,1.,-0.460543280768577));
#57592=CARTESIAN_POINT('Ctrl Pts',(4.00327590659129,1.,-0.462486702616252));
#57593=CARTESIAN_POINT('Ctrl Pts',(3.99586444320134,1.,-0.464388610938995));
#57594=CARTESIAN_POINT('Ctrl Pts',(3.98844946363258,1.,-0.466248520883035));
#57595=CARTESIAN_POINT('Ctrl Pts',(3.98103175589349,1.,-0.46806604792014));
#57596=CARTESIAN_POINT('Ctrl Pts',(3.97361320212413,1.,-0.469840942829878));
#57597=CARTESIAN_POINT('Ctrl Pts',(3.96619600864626,1.,-0.471572978413494));
#57598=CARTESIAN_POINT('Ctrl Pts',(3.95878201038332,1.,-0.473261847236296));
#57599=CARTESIAN_POINT('Ctrl Pts',(3.95137192932898,1.,-0.474907053021791));
#57600=CARTESIAN_POINT('Ctrl Pts',(3.94396469119385,1.,-0.476507810658535));
#57601=CARTESIAN_POINT('Ctrl Pts',(3.93655660689819,1.,-0.478062927140957));
#57602=CARTESIAN_POINT('Ctrl Pts',(3.92914297392067,1.,-0.479571028525566));
#57603=CARTESIAN_POINT('Ctrl Pts',(3.92171976072334,1.,-0.481030798910735));
#57604=CARTESIAN_POINT('Ctrl Pts',(3.91428536373749,1.,-0.482441230340709));
#57605=CARTESIAN_POINT('Ctrl Pts',(3.90684210358063,1.,-0.483801835089161));
#57606=CARTESIAN_POINT('Ctrl Pts',(3.89939844658529,1.,-0.485112963522246));
#57607=CARTESIAN_POINT('Ctrl Pts',(3.89196582437574,1.,-0.486375337854134));
#57608=CARTESIAN_POINT('Ctrl Pts',(3.88455453328156,1.,-0.487589452275179));
#57609=CARTESIAN_POINT('Ctrl Pts',(3.87716963231115,1.,-0.488754973798281));
#57610=CARTESIAN_POINT('Ctrl Pts',(3.86980755613694,1.,-0.4898702457049));
#57611=CARTESIAN_POINT('Ctrl Pts',(3.86245057319215,1.,-0.490931482170849));
#57612=CARTESIAN_POINT('Ctrl Pts',(3.85507287020223,1.,-0.49193363108376));
#57613=CARTESIAN_POINT('Ctrl Pts',(3.84765051147965,1.,-0.492871792414095));
#57614=CARTESIAN_POINT('Ctrl Pts',(3.84017095578438,1.,-0.493742574629117));
#57615=CARTESIAN_POINT('Ctrl Pts',(3.8326409268245,1.,-0.494545212256426));
#57616=CARTESIAN_POINT('Ctrl Pts',(3.82509963594156,1.,-0.495283458893903));
#57617=CARTESIAN_POINT('Ctrl Pts',(3.81760756144099,1.,-0.495963937875572));
#57618=CARTESIAN_POINT('Ctrl Pts',(3.81022254090909,1.,-0.496592643443789));
#57619=CARTESIAN_POINT('Ctrl Pts',(3.80297788298545,1.,-0.497171756201091));
#57620=CARTESIAN_POINT('Ctrl Pts',(3.79586380669959,1.,-0.497696892100581));
#57621=CARTESIAN_POINT('Ctrl Pts',(3.78879701661152,1.,-0.498152751800819));
#57622=CARTESIAN_POINT('Ctrl Pts',(3.78163975337189,1.,-0.498515471679379));
#57623=CARTESIAN_POINT('Ctrl Pts',(3.77425499225089,1.,-0.498759900365687));
#57624=CARTESIAN_POINT('Ctrl Pts',(3.76655401191144,1.,-0.498865792335185));
#57625=CARTESIAN_POINT('Ctrl Pts',(3.75854082221127,1.,-0.498823681615513));
#57626=CARTESIAN_POINT('Ctrl Pts',(3.75037362168103,1.,-0.498642802042929));
#57627=CARTESIAN_POINT('Ctrl Pts',(3.74235701735109,1.,-0.498350586058176));
#57628=CARTESIAN_POINT('Ctrl Pts',(3.73486914372834,1.,-0.497984209510496));
#57629=CARTESIAN_POINT('Ctrl Pts',(3.72830430904794,1.,-0.49758406715328));
#57630=CARTESIAN_POINT('Ctrl Pts',(3.72301489774241,1.,-0.497187079575795));
#57631=CARTESIAN_POINT('Ctrl Pts',(3.7195232082259,1.,-0.496846224822535));
#57632=CARTESIAN_POINT('Ctrl Pts',(3.71785517607694,1.,-0.496605651526314));
#57633=CARTESIAN_POINT('Ctrl Pts',(3.71721917030465,1.,-0.496446644158827));
#57634=CARTESIAN_POINT('Ctrl Pts',(3.71704500630521,1.,-0.496354087925646));
#57635=CARTESIAN_POINT('Ctrl Pts',(3.71701050416802,1.,-0.496319364829374));
#57636=CARTESIAN_POINT('',(4.18039834341342,0.,-0.40530197431835));
#57637=CARTESIAN_POINT('Origin',(4.1923339003649,0.,-0.253646344052521));
#57638=CARTESIAN_POINT('',(4.18039834341342,1.,-0.40530197431835));
#57639=CARTESIAN_POINT('Origin',(0.,1.,0.));
#57640=CARTESIAN_POINT('Origin',(0.,1.,0.));
#57641=CARTESIAN_POINT('Origin',(0.,0.,0.));
#57839=UNCERTAINTY_MEASURE_WITH_UNIT(LENGTH_MEASURE(0.001),#57901,
'DISTANCE_ACCURACY_VALUE',
'Maximum model space distance between geometric entities at asserted c
onnectivities');
#57841=UNCERTAINTY_MEASURE_WITH_UNIT(LENGTH_MEASURE(0.001),#57901,
'DISTANCE_ACCURACY_VALUE',
'Maximum model space distance between geometric entities at asserted c
onnectivities');
#57898=(
GEOMETRIC_REPRESENTATION_CONTEXT(3)
GLOBAL_UNCERTAINTY_ASSIGNED_CONTEXT((#57839))
GLOBAL_UNIT_ASSIGNED_CONTEXT((#57901,#57903,#57904))
REPRESENTATION_CONTEXT('','3D')
);
#57900=(
GEOMETRIC_REPRESENTATION_CONTEXT(3)
GLOBAL_UNCERTAINTY_ASSIGNED_CONTEXT((#57841))
GLOBAL_UNIT_ASSIGNED_CONTEXT((#57901,#57903,#57904))
REPRESENTATION_CONTEXT('','3D')
);
#57901=(
LENGTH_UNIT()
NAMED_UNIT(*)
SI_UNIT(.CENTI.,.METRE.)
);
#57903=(
NAMED_UNIT(*)
PLANE_ANGLE_UNIT()
SI_UNIT($,.RADIAN.)
);
#57904=(
NAMED_UNIT(*)
SI_UNIT($,.STERADIAN.)
SOLID_ANGLE_UNIT()
);
#57961=SHAPE_DEFINITION_REPRESENTATION(#58032,#58165);
#58032=PRODUCT_DEFINITION_SHAPE('',$,#58224);
#58165=SHAPE_REPRESENTATION('',(#15306),#57898);
#58167=PRODUCT_DEFINITION_CONTEXT('part definition',#58343,'design');
#58224=PRODUCT_DEFINITION('Spur Gear - Module 2, 40 Teeth, 20 mm Bore',
'Spur Gear - Module 2, 40 Teeth, 20 mm Bore',#58282,#58167);
#58282=PRODUCT_DEFINITION_FORMATION('',$,#58401);
#58343=APPLICATION_CONTEXT(
'Core Data for Automotive Mechanical Design Process');
#58344=PRODUCT_CONTEXT('part definition',#58343,'mechanical');
#58401=PRODUCT('Spur Gear - Module 2, 40 Teeth, 20 mm Bore',
'Spur Gear - Module 2, 40 Teeth, 20 mm Bore',
'Spur Gear - Module 2, 40 Teeth, 20 mm Bore',(#58344));
#58452=COLOUR_RGB('Sky Blue',0.24,0.69,0.87);
#58453=FILL_AREA_STYLE_COLOUR('',#58452);
#58454=FILL_AREA_STYLE('',(#58453));
#58455=SURFACE_STYLE_FILL_AREA(#58454);
#58456=SURFACE_SIDE_STYLE('',(#58455));
#58457=SURFACE_STYLE_USAGE(.BOTH.,#58456);
#58458=PRESENTATION_STYLE_ASSIGNMENT((#58457));
ENDSEC;
END-ISO-10303-21;
